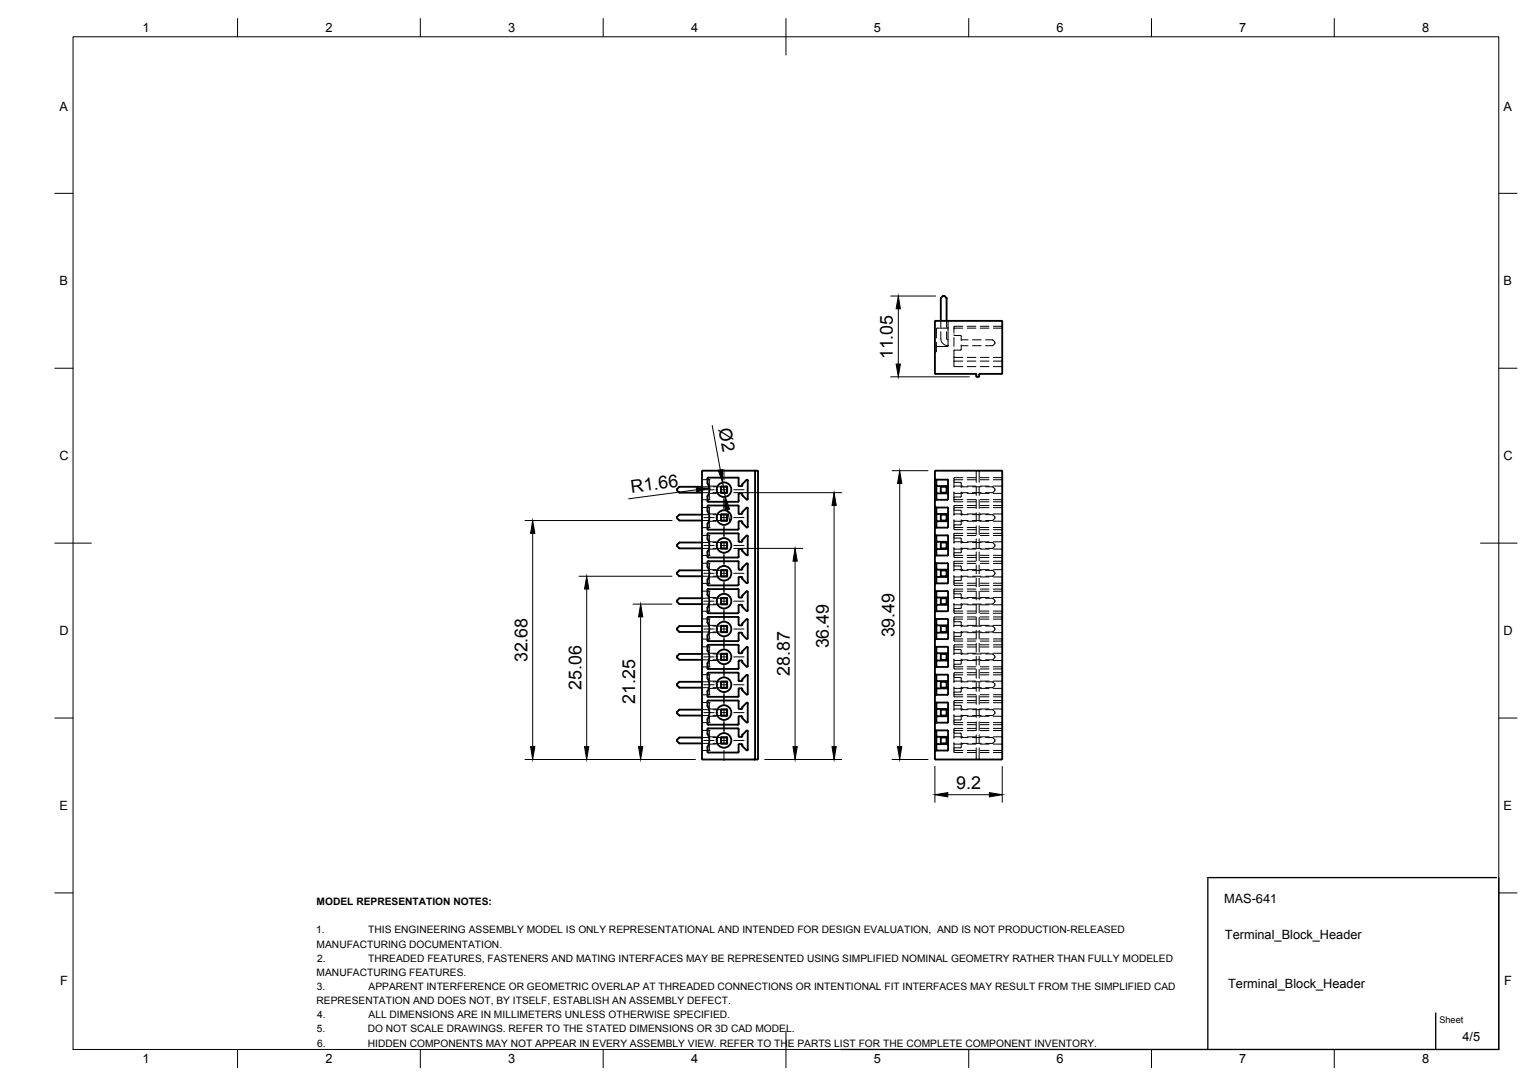
ISO-10303-21;
HEADER;
FILE_DESCRIPTION((''),'2;1');
FILE_NAME('Terminal_Block_Header.step','2026-10-09T09:55:32-07:00',(''),(''),'','','');
FILE_SCHEMA (('AUTOMOTIVE_DESIGN { 1 0 10303 214 3 1 1 }'));
ENDSEC;
DATA;
#10=MECHANICAL_DESIGN_GEOMETRIC_PRESENTATION_REPRESENTATION('',(#80780,#80781,#80782,#80783,#80784,#80785,#80786,#80787,#80788,#80789,#80790,#80791,#80792,#80793,#80794,#80795,#80796,#80797,#80798,#80799,#80800,#80801,#80802,#80803,#80804,#80805,#80806,#80807,#80808,#80809,#80810,#80811,#80812,#80813,#80814,#80815,#80816,#80817,#80818,#80819,#80820,#80821,#80822,#80823,#80824,#80825,#80826,#80827,#80828,#80829,#80830,#80831,#80832,#80833,#80834,#80835,#80836,#80837,#80838,#80839,#80840,#80841,#80842,#80843,#80844,#80845,#80846,#80847,#80848,#80849,#80850,#80851,#80852,#80853,#80854,#80855,#80856,#80857,#80858,#80859,#80860,#80861,#80862,#80863,#80864,#80865,#80866,#80867,#80868,#80869,#80870,#80871,#80872,#80873,#80874,#80875,#80876,#80877,#80878,#80879,#80880,#80881,#80882,#80883,#80884,#80885,#80886,#80887,#80888,#80889,#80890,#80891,#80892,#80893,#80894,#80895,#80896,#80897,#80898,#80899,#80900,#80901,#80902,#80903,#80904,#80905,#80906,#80907,#80908,#80909,#80910,#80911,#80912,#80913,#80914,#80915,#80916,#80917,#80918,#80919,#80920,#80921,#80922,#80923,#80924,#80925,#80926,#80927,#80928,#80929,#80930,#80931,#80932,#80933,#80934,#80935,#80936,#80937,#80938,#80939,#80940,#80941,#80942,#80943,#80944,#80945,#80946,#80947,#80948,#80949,#80950,#80951,#80952,#80953,#80954,#80955,#80956,#80957,#80958,#80959,#80960,#80961,#80962,#80963,#80964,#80965,#80966,#80967,#80968,#80969,#80970,#80971,#80972,#80973,#80974,#80975,#80976,#80977,#80978,#80979,#80980,#80981,#80982,#80983,#80984,#80985,#80986,#80987,#80988,#80989,#80990,#80991,#80992,#80993,#80994,#80995,#80996,#80997,#80998,#80999,#81000,#81001,#81002,#81003,#81004,#81005,#81006,#81007,#81008,#81009,#81010,#81011,#81012,#81013,#81014,#81015,#81016,#81017,#81018,#81019,#81020,#81021,#81022,#81023,#81024,#81025,#81026,#81027,#81028,#81029,#81030,#81031,#81032,#81033,#81034,#81035,#81036,#81037,#81038,#81039,#81040,#81041,#81042,#81043,#81044,#81045,#81046,#81047,#81048,#81049,#81050,#81051,#81052,#81053,#81054,#81055,#81056,#81057,#81058,#81059,#81060,#81061,#81062,#81063,#81064,#81065,#81066,#81067,#81068,#81069,#81070,#81071,#81072,#81073,#81074,#81075,#81076,#81077,#81078,#81079,#81080,#81081,#81082,#81083,#81084,#81085,#81086,#81087,#81088,#81089,#81090,#81091,#81092,#81093,#81094,#81095,#81096,#81097,#81098,#81099,#81100,#81101,#81102,#81103,#81104,#81105,#81106,#81107,#81108,#81109,#81110,#81111,#81112,#81113,#81114,#81115,#81116,#81117,#81118,#81119,#81120,#81121,#81122,#81123,#81124,#81125,#81126,#81127,#81128,#81129,#81130,#81131,#81132,#81133,#81134,#81135,#81136,#81137,#81138,#81139,#81140,#81141,#81142,#81143,#81144,#81145,#81146,#81147,#81148,#81149,#81150,#81151,#81152,#81153,#81154,#81155,#81156,#81157,#81158,#81159,#81160,#81161,#81162,#81163,#81164,#81165,#81166,#81167,#81168,#81169,#81170,#81171,#81172,#81173,#81174,#81175,#81176,#81177,#81178,#81179,#81180,#81181,#81182,#81183,#81184,#81185,#81186,#81187,#81188,#81189,#81190,#81191,#81192,#81193,#81194,#81195,#81196,#81197,#81198,#81199,#81200,#81201,#81202,#81203,#81204,#81205,#81206,#81207,#81208,#81209,#81210,#81211,#81212,#81213,#81214,#81215,#81216,#81217,#81218,#81219,#81220,#81221,#81222,#81223,#81224,#81225,#81226,#81227,#81228,#81229,#81230,#81231,#81232,#81233,#81234,#81235,#81236,#81237,#81238,#81239,#81240,#81241,#81242,#81243,#81244,#81245,#81246,#81247,#81248,#81249,#81250,#81251,#81252,#81253,#81254,#81255,#81256,#81257,#81258,#81259,#81260,#81261,#81262,#81263,#81264,#81265,#81266,#81267,#81268,#81269,#81270,#81271,#81272,#81273,#81274,#81275,#81276,#81277,#81278,#81279,#81280,#81281,#81282,#81283,#81284,#81285,#81286,#81287,#81288,#81289,#81290,#81291,#81292,#81293,#81294,#81295,#81296,#81297,#81298,#81299,#81300,#81301,#81302,#81303,#81304,#81305,#81306,#81307,#81308,#81309,#81310,#81311,#81312,#81313,#81314,#81315,#81316,#81317,#81318,#81319,#81320,#81321,#81322,#81323,#81324,#81325,#81326,#81327,#81328,#81329,#81330,#81331,#81332,#81333,#81334,#81335,#81336,#81337,#81338,#81339,#81340,#81341,#81342,#81343,#81344,#81345,#81346,#81347,#81348,#81349,#81350,#81351,#81352,#81353,#81354,#81355,#81356,#81357,#81358,#81359,#81360,#81361,#81362,#81363,#81364,#81365,#81366,#81367,#81368,#81369,#81370,#81371,#81372,#81373,#81374,#81375,#81376,#81377,#81378,#81379,#81380,#81381,#81382,#81383,#81384,#81385,#81386,#81387,#81388,#81389,#81390,#81391,#81392,#81393,#81394,#81395,#81396,#81397,#81398,#81399,#81400,#81401,#81402,#81403,#81404,#81405,#81406,#81407,#81408,#81409,#81410,#81411,#81412,#81413,#81414,#81415,#81416,#81417,#81418,#81419,#81420,#81421,#81422,#81423,#81424,#81425,#81426,#81427,#81428,#81429,#81430,#81431,#81432,#81433,#81434,#81435,#81436,#81437,#81438,#81439,#81440,#81441,#81442,#81443,#81444,#81445,#81446,#81447,#81448,#81449,#81450,#81451,#81452,#81453,#81454,#81455,#81456,#81457,#81458,#81459,#81460,#81461,#81462,#81463,#81464,#81465,#81466,#81467,#81468,#81469,#81470,#81471,#81472,#81473,#81474,#81475,#81476,#81477,#81478,#81479,#81480,#81481,#81482,#81483,#81484,#81485,#81486,#81487,#81488,#81489,#81490,#81491,#81492,#81493,#81494,#81495,#81496,#81497,#81498,#81499,#81500,#81501,#81502,#81503,#81504,#81505,#81506,#81507,#81508,#81509,#81510,#81511,#81512,#81513,#81514,#81515,#81516,#81517,#81518,#81519,#81520,#81521,#81522,#81523,#81524,#81525,#81526,#81527,#81528,#81529,#81530,#81531,#81532,#81533,#81534,#81535,#81536,#81537,#81538,#81539,#81540,#81541,#81542,#81543,#81544,#81545,#81546,#81547,#81548,#81549,#81550,#81551,#81552,#81553,#81554,#81555,#81556,#81557,#81558,#81559,#81560,#81561,#81562,#81563,#81564,#81565,#81566,#81567,#81568,#81569,#81570,#81571,#81572,#81573,#81574,#81575,#81576,#81577,#81578,#81579,#81580,#81581,#81582,#81583,#81584,#81585,#81586,#81587,#81588,#81589,#81590,#81591,#81592,#81593,#81594,#81595,#81596,#81597,#81598,#81599,#81600,#81601,#81602,#81603,#81604,#81605,#81606,#81607,#81608,#81609,#81610,#81611,#81612,#81613,#81614,#81615,#81616,#81617,#81618,#81619,#81620,#81621,#81622,#81623,#81624,#81625,#81626,#81627,#81628,#81629,#81630,#81631,#81632,#81633,#81634,#81635,#81636,#81637,#81638,#81639,#81640,#81641,#81642,#81643,#81644,#81645,#81646,#81647,#81648,#81649,#81650,#81651,#81652,#81653,#81654,#81655,#81656,#81657,#81658,#81659,#81660,#81661,#81662,#81663,#81664,#81665,#81666,#81667,#81668,#81669,#81670,#81671,#81672,#81673,#81674,#81675,#81676,#81677,#81678,#81679,#81680,#81681,#81682,#81683,#81684,#81685,#81686,#81687,#81688,#81689,#81690,#81691,#81692,#81693,#81694,#81695,#81696,#81697,#81698,#81699,#81700,#81701,#81702,#81703,#81704,#81705,#81706,#81707,#81708,#81709,#81710,#81711,#81712,#81713,#81714,#81715,#81716,#81717,#81718,#81719,#81720,#81721,#81722,#81723,#81724,#81725,#81726,#81727,#81728,#81729,#81730,#81731,#81732,#81733,#81734,#81735,#81736,#81737,#81738,#81739,#81740,#81741,#81742,#81743,#81744,#81745,#81746,#81747,#81748,#81749,#81750,#81751,#81752,#81753,#81754,#81755,#81756,#81757,#81758,#81759,#81760,#81761,#81762,#81763,#81764,#81765,#81766,#81767,#81768,#81769,#81770,#81771,#81772,#81773,#81774,#81775,#81776,#81777,#81778,#81779,#81780,#81781,#81782,#81783,#81784,#81785,#81786,#81787,#81788,#81789,#81790,#81791,#81792,#81793,#81794,#81795,#81796,#81797,#81798,#81799,#81800,#81801,#81802,#81803,#81804,#81805,#81806,#81807,#81808,#81809,#81810,#81811,#81812,#81813,#81814,#81815,#81816,#81817,#81818,#81819,#81820,#81821,#81822,#81823,#81824,#81825,#81826,#81827,#81828,#81829,#81830,#81831,#81832,#81833,#81834,#81835,#81836,#81837,#81838,#81839,#81840,#81841,#81842,#81843,#81844,#81845,#81846,#81847,#81848,#81849,#81850,#81851,#81852,#81853,#81854,#81855,#81856,#81857,#81858,#81859,#81860,#81861,#81862,#81863,#81864,#81865,#81866,#81867,#81868,#81869,#81870,#81871,#81872,#81873,#81874,#81875,#81876,#81877,#81878,#81879,#81880,#81881,#81882,#81883,#81884,#81885,#81886,#81887,#81888,#81889,#81890,#81891,#81892,#81893,#81894,#81895,#81896,#81897,#81898,#81899,#81900,#81901,#81902,#81903,#81904,#81905,#81906,#81907,#81908,#81909,#81910,#81911,#81912,#81913,#81914,#81915,#81916,#81917,#81918,#81919,#81920,#81921,#81922,#81923,#81924,#81925,#81926,#81927,#81928,#81929,#81930,#81931,#81932,#81933,#81934,#81935,#81936,#81937,#81938,#81939,#81940,#81941,#81942,#81943,#81944,#81945,#81946,#81947,#81948,#81949,#81950,#81951,#81952,#81953,#81954,#81955,#81956,#81957,#81958,#81959,#81960,#81961,#81962,#81963,#81964,#81965,#81966,#81967,#81968,#81969,#81970,#81971,#81972,#81973,#81974,#81975,#81976,#81977,#81978,#81979,#81980,#81981,#81982,#81983,#81984,#81985,#81986,#81987,#81988,#81989,#81990,#81991,#81992,#81993,#81994,#81995,#81996,#81997,#81998,#81999,#82000,#82001,#82002,#82003,#82004,#82005,#82006,#82007,#82008,#82009,#82010,#82011,#82012,#82013,#82014,#82015,#82016,#82017,#82018,#82019,#82020,#82021,#82022,#82023,#82024,#82025,#82026,#82027,#82028,#82029,#82030,#82031,#82032,#82033,#82034,#82035,#82036,#82037,#82038,#82039,#82040,#82041,#82042,#82043,#82044,#82045,#82046,#82047,#82048,#82049,#82050,#82051,#82052,#82053,#82054,#82055,#82056,#82057,#82058,#82059,#82060,#82061,#82062,#82063,#82064,#82065,#82066,#82067,#82068,#82069,#82070,#82071,#82072,#82073,#82074,#82075,#82076,#82077,#82078,#82079,#82080,#82081,#82082,#82083,#82084,#82085,#82086,#82087,#82088,#82089,#82090,#82091,#82092,#82093,#82094,#82095,#82096,#82097,#82098,#82099,#82100,#82101,#82102,#82103,#82104,#82105,#82106,#82107,#82108,#82109,#82110,#82111,#82112,#82113,#82114,#82115,#82116,#82117,#82118,#82119,#82120,#82121,#82122,#82123,#82124,#82125,#82126,#82127,#82128,#82129,#82130,#82131,#82132,#82133,#82134,#82135,#82136,#82137,#82138,#82139,#82140,#82141,#82142,#82143,#82144,#82145,#82146,#82147,#82148,#82149,#82150,#82151,#82152,#82153,#82154,#82155,#82156,#82157,#82158,#82159,#82160,#82161,#82162,#82163,#82164,#82165,#82166,#82167,#82168,#82169,#82170,#82171,#82172,#82173,#82174,#82175,#82176,#82177,#82178,#82179,#82180,#82181,#82182,#82183,#82184,#82185,#82186,#82187,#82188,#82189,#82190,#82191,#82192,#82193,#82194,#82195,#82196,#82197,#82198,#82199,#82200,#82201,#82202,#82203,#82204,#82205,#82206,#82207,#82208,#82209,#82210,#82211,#82212,#82213,#82214,#82215,#82216,#82217,#82218,#82219,#82220,#82221,#82222,#82223,#82224,#82225,#82226,#82227,#82228,#82229,#82230,#82231,#82232,#82233,#82234,#82235,#82236,#82237,#82238,#82239,#82240,#82241,#82242,#82243,#82244,#82245,#82246,#82247,#82248,#82249,#82250,#82251,#82252,#82253,#82254,#82255,#82256,#82257,#82258,#82259,#82260,#82261,#82262,#82263,#82264,#82265,#82266,#82267,#82268,#82269,#82270,#82271,#82272,#82273,#82274,#82275,#82276,#82277,#82278,#82279,#82280,#82281,#82282,#82283,#82284,#82285,#82286,#82287,#82288,#82289,#82290,#82291,#82292,#82293,#82294,#82295,#82296,#82297,#82298,#82299,#82300,#82301,#82302,#82303,#82304,#82305,#82306,#82307,#82308,#82309,#82310,#82311,#82312,#82313,#82314,#82315,#82316,#82317,#82318,#82319,#82320,#82321,#82322,#82323,#82324,#82325,#82326,#82327,#82328,#82329,#82330,#82331,#82332,#82333,#82334,#82335,#82336,#82337,#82338,#82339,#82340,#82341,#82342,#82343,#82344,#82345,#82346,#82347,#82348,#82349,#82350,#82351,#82352,#82353,#82354,#82355,#82356,#82357,#82358,#82359,#82360,#82361,#82362,#82363,#82364,#82365,#82366,#82367,#82368,#82369,#82370,#82371,#82372,#82373,#82374,#82375,#82376,#82377,#82378,#82379,#82380,#82381,#82382,#82383,#82384,#82385,#82386,#82387,#82388,#82389,#82390,#82391,#82392,#82393,#82394,#82395,#82396,#82397,#82398,#82399,#82400,#82401,#82402,#82403,#82404,#82405,#82406,#82407,#82408,#82409,#82410,#82411,#82412,#82413,#82414,#82415,#82416,#82417,#82418,#82419,#82420,#82421,#82422,#82423,#82424,#82425,#82426,#82427,#82428,#82429,#82430,#82431,#82432,#82433,#82434,#82435,#82436,#82437,#82438,#82439,#82440,#82441,#82442,#82443,#82444,#82445,#82446,#82447,#82448,#82449,#82450,#82451,#82452,#82453,#82454,#82455,#82456,#82457,#82458,#82459,#82460,#82461,#82462,#82463,#82464,#82465,#82466,#82467,#82468,#82469,#82470,#82471,#82472,#82473,#82474,#82475,#82476,#82477,#82478,#82479,#82480,#82481,#82482,#82483,#82484,#82485,#82486,#82487,#82488,#82489,#82490,#82491,#82492,#82493,#82494,#82495,#82496,#82497,#82498,#82499,#82500,#82501,#82502,#82503,#82504,#82505,#82506,#82507,#82508,#82509,#82510,#82511,#82512,#82513,#82514,#82515,#82516,#82517,#82518,#82519,#82520,#82521,#82522,#82523,#82524,#82525,#82526,#82527,#82528,#82529,#82530,#82531,#82532,#82533,#82534,#82535,#82536,#82537,#82538,#82539,#82540,#82541,#82542,#82543,#82544,#82545,#82546,#82547,#82548,#82549,#82550,#82551,#82552,#82553,#82554,#82555,#82556,#82557,#82558,#82559,#82560,#82561,#82562,#82563,#82564,#82565,#82566,#82567,#82568,#82569,#82570,#82571,#82572,#82573,#82574,#82575,#82576,#82577,#82578,#82579,#82580,#82581,#82582,#82583,#82584,#82585,#82586,#82587,#82588,#82589,#82590,#82591,#82592,#82593,#82594,#82595,#82596,#82597,#82598,#82599,#82600,#82601,#82602,#82603,#82604,#82605,#82606,#82607,#82608,#82609,#82610,#82611,#82612,#82613,#82614,#82615,#82616,#82617,#82618,#82619,#82620,#82621,#82622,#82623,#82624,#82625,#82626,#82627,#82628,#82629,#82630,#82631,#82632,#82633,#82634,#82635,#82636,#82637,#82638,#82639,#82640,#82641,#82642,#82643,#82644,#82645,#82646,#82647,#82648,#82649,#82650,#82651,#82652,#82653,#82654,#82655,#82656,#82657,#82658,#82659,#82660,#82661,#82662,#82663,#82664,#82665,#82666,#82667,#82668,#82669,#82670,#82671,#82672,#82673,#82674,#82675,#82676,#82677,#82678,#82679,#82680,#82681,#82682,#82683,#82684,#82685,#82686,#82687,#82688,#82689,#82690,#82691,#82692,#82693,#82694,#82695,#82696,#82697,#82698,#82699,#82700,#82701,#82702,#82703,#82704,#82705,#82706,#82707,#82708,#82709,#82710,#82711,#82712,#82713,#82714,#82715,#82716,#82717,#82718,#82719,#82720,#82721,#82722,#82723,#82724,#82725,#82726,#82727,#82728,#82729,#82730,#82731,#82732,#82733,#82734,#82735,#82736,#82737,#82738,#82739,#82740,#82741,#82742,#82743,#82744,#82745,#82746,#82747,#82748,#82749,#82750,#82751,#82752,#82753,#82754,#82755,#82756,#82757,#82758,#82759,#82760,#82761,#82762,#82763,#82764,#82765,#82766,#82767,#82768,#82769,#82770,#82771,#82772,#82773,#82774,#82775,#82776,#82777,#82778,#82779,#82780,#82781,#82782,#82783,#82784,#82785,#82786,#82787,#82788,#82789,#82790,#82791,#82792,#82793,#82794,#82795,#82796,#82797,#82798,#82799,#82800,#82801,#82802,#82803,#82804,#82805,#82806,#82807,#82808,#82809,#82810,#82811,#82812,#82813,#82814,#82815,#82816,#82817,#82818,#82819,#82820,#82821,#82822,#82823,#82824,#82825,#82826,#82827,#82828,#82829,#82830,#82831,#82832,#82833,#82834,#82835,#82836,#82837,#82838,#82839,#82840,#82841,#82842,#82843,#82844,#82845,#82846,#82847,#82848,#82849,#82850,#82851,#82852,#82853,#82854,#82855,#82856,#82857,#82858,#82859,#82860,#82861,#82862,#82863,#82864,#82865,#82866,#82867,#82868,#82869,#82870,#82871,#82872,#82873,#82874,#82875,#82876,#82877,#82878,#82879,#82880,#82881,#82882,#82883,#82884,#82885,#82886,#82887,#82888,#82889,#82890,#82891,#82892,#82893,#82894,#82895,#82896,#82897,#82898,#82899,#82900,#82901,#82902,#82903,#82904,#82905,#82906,#82907,#82908,#82909,#82910,#82911,#82912,#82913,#82914,#82915,#82916,#82917,#82918,#82919,#82920,#82921,#82922,#82923,#82924,#82925,#82926,#82927,#82928,#82929,#82930,#82931,#82932,#82933,#82934,#82935,#82936,#82937,#82938,#82939,#82940,#82941,#82942,#82943,#82944,#82945,#82946,#82947,#82948,#82949,#82950,#82951,#82952,#82953,#82954,#82955,#82956,#82957,#82958,#82959,#82960,#82961,#82962,#82963,#82964,#82965,#82966,#82967,#82968,#82969,#82970,#82971,#82972,#82973,#82974,#82975,#82976,#82977,#82978,#82979,#82980,#82981,#82982,#82983,#82984,#82985,#82986,#82987,#82988,#82989,#82990,#82991,#82992,#82993,#82994,#82995,#82996,#82997,#82998,#82999,#83000,#83001,#83002,#83003,#83004,#83005,#83006,#83007,#83008,#83009,#83010),#170127);
#24=SHAPE_REPRESENTATION_RELATIONSHIP('SRR','None',#170145,#27) ;
#27=ADVANCED_BREP_SHAPE_REPRESENTATION('',(#32),#170125) ;
#32=MANIFOLD_SOLID_BREP('Body1',#91086) ;
#357=ELLIPSE('',#93363,0.141421356226833,0.0999999999854714) ;
#358=ELLIPSE('',#93380,0.141421356205715,0.0999999999561054) ;
#359=ELLIPSE('',#93397,0.141421356206211,0.0999999999568741) ;
#360=ELLIPSE('',#93414,0.14142135619891,0.0999999999469108) ;
#361=ELLIPSE('',#93431,0.14142135620716,0.0999999999583245) ;
#362=ELLIPSE('',#93448,0.141421356264666,0.100000000037862) ;
#363=ELLIPSE('',#93465,0.141421356235352,0.0999999999972513) ;
#364=ELLIPSE('',#93482,0.141421356240128,0.100000000003844) ;
#365=ELLIPSE('',#93544,0.141421356242718,0.100000000007393) ;
#366=ELLIPSE('',#93593,0.141421356244824,0.100000000010334) ;
#684=FACE_BOUND('',#24047,.T.) ;
#685=FACE_BOUND('',#24048,.T.) ;
#686=FACE_BOUND('',#24049,.T.) ;
#687=FACE_BOUND('',#24050,.T.) ;
#688=FACE_BOUND('',#24051,.T.) ;
#689=FACE_BOUND('',#24052,.T.) ;
#690=FACE_BOUND('',#24053,.T.) ;
#691=FACE_BOUND('',#24054,.T.) ;
#692=FACE_BOUND('',#24055,.T.) ;
#693=FACE_BOUND('',#24056,.T.) ;
#694=FACE_BOUND('',#24093,.T.) ;
#695=FACE_BOUND('',#24095,.T.) ;
#696=FACE_BOUND('',#24382,.T.) ;
#697=FACE_BOUND('',#24411,.T.) ;
#698=FACE_BOUND('',#24440,.T.) ;
#699=FACE_BOUND('',#24469,.T.) ;
#700=FACE_BOUND('',#24498,.T.) ;
#701=FACE_BOUND('',#24527,.T.) ;
#702=FACE_BOUND('',#24556,.T.) ;
#703=FACE_BOUND('',#24585,.T.) ;
#704=FACE_BOUND('',#24614,.T.) ;
#705=FACE_BOUND('',#24616,.T.) ;
#706=FACE_BOUND('',#24618,.T.) ;
#707=FACE_BOUND('',#24620,.T.) ;
#708=FACE_BOUND('',#24622,.T.) ;
#709=FACE_BOUND('',#24624,.T.) ;
#710=FACE_BOUND('',#24626,.T.) ;
#711=FACE_BOUND('',#24628,.T.) ;
#712=FACE_BOUND('',#24630,.T.) ;
#713=FACE_BOUND('',#24632,.T.) ;
#1083=PLANE('',#93599) ;
#1084=PLANE('',#93604) ;
#1085=PLANE('',#93609) ;
#1086=PLANE('',#93614) ;
#1087=PLANE('',#93619) ;
#1088=PLANE('',#93624) ;
#1089=PLANE('',#93629) ;
#1090=PLANE('',#93634) ;
#1091=PLANE('',#93639) ;
#1092=PLANE('',#93644) ;
#1093=PLANE('',#93646) ;
#1094=PLANE('',#93648) ;
#1095=PLANE('',#93650) ;
#1096=PLANE('',#93652) ;
#1097=PLANE('',#93654) ;
#1098=PLANE('',#93656) ;
#1099=PLANE('',#93658) ;
#1100=PLANE('',#93660) ;
#1101=PLANE('',#93662) ;
#1102=PLANE('',#93664) ;
#1103=PLANE('',#93666) ;
#1104=PLANE('',#93668) ;
#1105=PLANE('',#93670) ;
#1106=PLANE('',#93672) ;
#1107=PLANE('',#93674) ;
#1108=PLANE('',#93676) ;
#1109=PLANE('',#93678) ;
#1110=PLANE('',#93707) ;
#1111=PLANE('',#93712) ;
#1112=PLANE('',#93714) ;
#1113=PLANE('',#93722) ;
#1114=PLANE('',#93746) ;
#1115=PLANE('',#93770) ;
#1116=PLANE('',#93774) ;
#1117=PLANE('',#93778) ;
#1118=PLANE('',#93782) ;
#1119=PLANE('',#93786) ;
#1120=PLANE('',#93790) ;
#1121=PLANE('',#93891) ;
#1122=PLANE('',#93894) ;
#1123=PLANE('',#93897) ;
#1124=PLANE('',#93900) ;
#1125=PLANE('',#93901) ;
#1126=PLANE('',#93902) ;
#1127=PLANE('',#93903) ;
#1128=PLANE('',#93904) ;
#1129=PLANE('',#93908) ;
#1130=PLANE('',#93912) ;
#1131=PLANE('',#93916) ;
#1132=PLANE('',#93919) ;
#1133=PLANE('',#93920) ;
#1134=PLANE('',#93924) ;
#1135=PLANE('',#93928) ;
#1136=PLANE('',#93932) ;
#1137=PLANE('',#93936) ;
#1138=PLANE('',#93940) ;
#1139=PLANE('',#93950) ;
#1140=PLANE('',#93954) ;
#1141=PLANE('',#93958) ;
#1142=PLANE('',#93959) ;
#1143=PLANE('',#93965) ;
#1144=PLANE('',#94240) ;
#1145=PLANE('',#94241) ;
#1146=PLANE('',#94242) ;
#1147=PLANE('',#94243) ;
#1148=PLANE('',#94244) ;
#1149=PLANE('',#94245) ;
#1150=PLANE('',#94248) ;
#1151=PLANE('',#94257) ;
#1152=PLANE('',#94258) ;
#1153=PLANE('',#94259) ;
#1154=PLANE('',#94260) ;
#1155=PLANE('',#94261) ;
#1156=PLANE('',#94262) ;
#1157=PLANE('',#94263) ;
#1158=PLANE('',#94264) ;
#1159=PLANE('',#94265) ;
#1160=PLANE('',#94266) ;
#1161=PLANE('',#94267) ;
#1162=PLANE('',#94380) ;
#1163=PLANE('',#94383) ;
#1164=PLANE('',#94386) ;
#1165=PLANE('',#94389) ;
#1166=PLANE('',#94392) ;
#1167=PLANE('',#94395) ;
#1168=PLANE('',#94398) ;
#1169=PLANE('',#94401) ;
#1170=PLANE('',#94404) ;
#1171=PLANE('',#94407) ;
#1172=PLANE('',#94408) ;
#1173=PLANE('',#94409) ;
#1174=PLANE('',#94410) ;
#1175=PLANE('',#94411) ;
#1176=PLANE('',#94412) ;
#1177=PLANE('',#94413) ;
#1178=PLANE('',#94414) ;
#1179=PLANE('',#94415) ;
#1180=PLANE('',#94416) ;
#1181=PLANE('',#94417) ;
#1182=PLANE('',#94418) ;
#1183=PLANE('',#94419) ;
#1184=PLANE('',#94420) ;
#1185=PLANE('',#94421) ;
#1186=PLANE('',#94422) ;
#1187=PLANE('',#94423) ;
#1188=PLANE('',#94424) ;
#1189=PLANE('',#94425) ;
#1190=PLANE('',#94426) ;
#1191=PLANE('',#94427) ;
#1192=PLANE('',#94428) ;
#1193=PLANE('',#94429) ;
#1194=PLANE('',#94430) ;
#1195=PLANE('',#94431) ;
#1196=PLANE('',#94432) ;
#1197=PLANE('',#94433) ;
#1198=PLANE('',#94434) ;
#1199=PLANE('',#94435) ;
#1200=PLANE('',#94436) ;
#1201=PLANE('',#94437) ;
#1202=PLANE('',#94438) ;
#1203=PLANE('',#94439) ;
#1204=PLANE('',#94440) ;
#1205=PLANE('',#94441) ;
#1206=PLANE('',#94442) ;
#1207=PLANE('',#94443) ;
#1208=PLANE('',#94444) ;
#1209=PLANE('',#94445) ;
#1210=PLANE('',#94446) ;
#1211=PLANE('',#94447) ;
#1212=PLANE('',#94448) ;
#1213=PLANE('',#94449) ;
#1214=PLANE('',#94450) ;
#1215=PLANE('',#94451) ;
#1216=PLANE('',#94455) ;
#1217=PLANE('',#94459) ;
#1218=PLANE('',#94463) ;
#1219=PLANE('',#94466) ;
#1220=PLANE('',#94467) ;
#1221=PLANE('',#94471) ;
#1222=PLANE('',#94475) ;
#1223=PLANE('',#94479) ;
#1224=PLANE('',#94483) ;
#1225=PLANE('',#94487) ;
#1226=PLANE('',#94497) ;
#1227=PLANE('',#94501) ;
#1228=PLANE('',#94505) ;
#1229=PLANE('',#94506) ;
#1230=PLANE('',#94515) ;
#1231=PLANE('',#94519) ;
#1232=PLANE('',#94523) ;
#1233=PLANE('',#94526) ;
#1234=PLANE('',#94527) ;
#1235=PLANE('',#94531) ;
#1236=PLANE('',#94535) ;
#1237=PLANE('',#94539) ;
#1238=PLANE('',#94543) ;
#1239=PLANE('',#94547) ;
#1240=PLANE('',#94557) ;
#1241=PLANE('',#94561) ;
#1242=PLANE('',#94565) ;
#1243=PLANE('',#94566) ;
#1244=PLANE('',#94575) ;
#1245=PLANE('',#94579) ;
#1246=PLANE('',#94583) ;
#1247=PLANE('',#94586) ;
#1248=PLANE('',#94587) ;
#1249=PLANE('',#94591) ;
#1250=PLANE('',#94595) ;
#1251=PLANE('',#94599) ;
#1252=PLANE('',#94603) ;
#1253=PLANE('',#94607) ;
#1254=PLANE('',#94617) ;
#1255=PLANE('',#94621) ;
#1256=PLANE('',#94625) ;
#1257=PLANE('',#94626) ;
#1258=PLANE('',#94635) ;
#1259=PLANE('',#94639) ;
#1260=PLANE('',#94643) ;
#1261=PLANE('',#94646) ;
#1262=PLANE('',#94647) ;
#1263=PLANE('',#94651) ;
#1264=PLANE('',#94655) ;
#1265=PLANE('',#94659) ;
#1266=PLANE('',#94663) ;
#1267=PLANE('',#94667) ;
#1268=PLANE('',#94677) ;
#1269=PLANE('',#94681) ;
#1270=PLANE('',#94685) ;
#1271=PLANE('',#94686) ;
#1272=PLANE('',#94695) ;
#1273=PLANE('',#94699) ;
#1274=PLANE('',#94703) ;
#1275=PLANE('',#94706) ;
#1276=PLANE('',#94707) ;
#1277=PLANE('',#94711) ;
#1278=PLANE('',#94715) ;
#1279=PLANE('',#94719) ;
#1280=PLANE('',#94723) ;
#1281=PLANE('',#94727) ;
#1282=PLANE('',#94737) ;
#1283=PLANE('',#94741) ;
#1284=PLANE('',#94745) ;
#1285=PLANE('',#94746) ;
#1286=PLANE('',#94755) ;
#1287=PLANE('',#94759) ;
#1288=PLANE('',#94763) ;
#1289=PLANE('',#94766) ;
#1290=PLANE('',#94767) ;
#1291=PLANE('',#94771) ;
#1292=PLANE('',#94775) ;
#1293=PLANE('',#94779) ;
#1294=PLANE('',#94783) ;
#1295=PLANE('',#94787) ;
#1296=PLANE('',#94797) ;
#1297=PLANE('',#94801) ;
#1298=PLANE('',#94805) ;
#1299=PLANE('',#94806) ;
#1300=PLANE('',#94815) ;
#1301=PLANE('',#94819) ;
#1302=PLANE('',#94823) ;
#1303=PLANE('',#94826) ;
#1304=PLANE('',#94827) ;
#1305=PLANE('',#94831) ;
#1306=PLANE('',#94835) ;
#1307=PLANE('',#94839) ;
#1308=PLANE('',#94843) ;
#1309=PLANE('',#94847) ;
#1310=PLANE('',#94857) ;
#1311=PLANE('',#94861) ;
#1312=PLANE('',#94865) ;
#1313=PLANE('',#94866) ;
#1314=PLANE('',#94875) ;
#1315=PLANE('',#94879) ;
#1316=PLANE('',#94883) ;
#1317=PLANE('',#94886) ;
#1318=PLANE('',#94887) ;
#1319=PLANE('',#94891) ;
#1320=PLANE('',#94895) ;
#1321=PLANE('',#94899) ;
#1322=PLANE('',#94903) ;
#1323=PLANE('',#94907) ;
#1324=PLANE('',#94917) ;
#1325=PLANE('',#94921) ;
#1326=PLANE('',#94925) ;
#1327=PLANE('',#94926) ;
#1328=PLANE('',#94935) ;
#1329=PLANE('',#94939) ;
#1330=PLANE('',#94943) ;
#1331=PLANE('',#94946) ;
#1332=PLANE('',#94947) ;
#1333=PLANE('',#94951) ;
#1334=PLANE('',#94955) ;
#1335=PLANE('',#94959) ;
#1336=PLANE('',#94963) ;
#1337=PLANE('',#94967) ;
#1338=PLANE('',#94977) ;
#1339=PLANE('',#94981) ;
#1340=PLANE('',#94985) ;
#1341=PLANE('',#94986) ;
#1342=PLANE('',#94992) ;
#1343=PLANE('',#94997) ;
#1344=PLANE('',#95002) ;
#1345=PLANE('',#95007) ;
#1346=PLANE('',#95012) ;
#1347=PLANE('',#95017) ;
#1348=PLANE('',#95022) ;
#1349=PLANE('',#95027) ;
#1350=PLANE('',#95032) ;
#1351=PLANE('',#96891) ;
#1352=PLANE('',#96892) ;
#1353=PLANE('',#96893) ;
#1354=PLANE('',#96894) ;
#1355=PLANE('',#96895) ;
#1356=PLANE('',#96896) ;
#1357=PLANE('',#96899) ;
#1358=PLANE('',#96908) ;
#1359=PLANE('',#96909) ;
#1360=PLANE('',#96910) ;
#1361=PLANE('',#96911) ;
#1362=PLANE('',#96912) ;
#1363=PLANE('',#96913) ;
#1364=PLANE('',#96914) ;
#1365=PLANE('',#96915) ;
#1366=PLANE('',#96916) ;
#1367=PLANE('',#96917) ;
#1368=PLANE('',#96918) ;
#1369=PLANE('',#96919) ;
#1370=PLANE('',#96920) ;
#1371=PLANE('',#96923) ;
#1372=PLANE('',#96932) ;
#1373=PLANE('',#96933) ;
#1374=PLANE('',#96934) ;
#1375=PLANE('',#96935) ;
#1376=PLANE('',#96936) ;
#1377=PLANE('',#96937) ;
#1378=PLANE('',#96938) ;
#1379=PLANE('',#96939) ;
#1380=PLANE('',#96940) ;
#1381=PLANE('',#96941) ;
#1382=PLANE('',#96942) ;
#1383=PLANE('',#96943) ;
#1384=PLANE('',#96944) ;
#1385=PLANE('',#96947) ;
#1386=PLANE('',#96956) ;
#1387=PLANE('',#96957) ;
#1388=PLANE('',#96958) ;
#1389=PLANE('',#96959) ;
#1390=PLANE('',#96960) ;
#1391=PLANE('',#96961) ;
#1392=PLANE('',#96962) ;
#1393=PLANE('',#96963) ;
#1394=PLANE('',#96964) ;
#1395=PLANE('',#96965) ;
#1396=PLANE('',#96966) ;
#1397=PLANE('',#96967) ;
#1398=PLANE('',#96968) ;
#1399=PLANE('',#96971) ;
#1400=PLANE('',#96980) ;
#1401=PLANE('',#96981) ;
#1402=PLANE('',#96982) ;
#1403=PLANE('',#96983) ;
#1404=PLANE('',#96984) ;
#1405=PLANE('',#96985) ;
#1406=PLANE('',#96986) ;
#1407=PLANE('',#96987) ;
#1408=PLANE('',#96988) ;
#1409=PLANE('',#96989) ;
#1410=PLANE('',#96990) ;
#1411=PLANE('',#96991) ;
#1412=PLANE('',#96992) ;
#1413=PLANE('',#96995) ;
#1414=PLANE('',#97004) ;
#1415=PLANE('',#97005) ;
#1416=PLANE('',#97006) ;
#1417=PLANE('',#97007) ;
#1418=PLANE('',#97008) ;
#1419=PLANE('',#97009) ;
#1420=PLANE('',#97010) ;
#1421=PLANE('',#97011) ;
#1422=PLANE('',#97012) ;
#1423=PLANE('',#97013) ;
#1424=PLANE('',#97014) ;
#1425=PLANE('',#97015) ;
#1426=PLANE('',#97016) ;
#1427=PLANE('',#97019) ;
#1428=PLANE('',#97028) ;
#1429=PLANE('',#97029) ;
#1430=PLANE('',#97030) ;
#1431=PLANE('',#97031) ;
#1432=PLANE('',#97032) ;
#1433=PLANE('',#97033) ;
#1434=PLANE('',#97034) ;
#1435=PLANE('',#97035) ;
#1436=PLANE('',#97036) ;
#1437=PLANE('',#97037) ;
#1438=PLANE('',#97038) ;
#1439=PLANE('',#97039) ;
#1440=PLANE('',#97040) ;
#1441=PLANE('',#97043) ;
#1442=PLANE('',#97052) ;
#1443=PLANE('',#97053) ;
#1444=PLANE('',#97054) ;
#1445=PLANE('',#97055) ;
#1446=PLANE('',#97056) ;
#1447=PLANE('',#97057) ;
#1448=PLANE('',#97058) ;
#1449=PLANE('',#97059) ;
#1450=PLANE('',#97060) ;
#1451=PLANE('',#97061) ;
#1452=PLANE('',#97062) ;
#1453=PLANE('',#97063) ;
#1454=PLANE('',#97064) ;
#1455=PLANE('',#97067) ;
#1456=PLANE('',#97076) ;
#1457=PLANE('',#97077) ;
#1458=PLANE('',#97078) ;
#1459=PLANE('',#97079) ;
#1460=PLANE('',#97080) ;
#1461=PLANE('',#97081) ;
#1462=PLANE('',#97082) ;
#1463=PLANE('',#97083) ;
#1464=PLANE('',#97084) ;
#1465=PLANE('',#97085) ;
#1466=PLANE('',#97086) ;
#1467=PLANE('',#97087) ;
#1468=PLANE('',#97088) ;
#1469=PLANE('',#97091) ;
#1470=PLANE('',#97100) ;
#1471=PLANE('',#97101) ;
#1472=PLANE('',#97102) ;
#1473=PLANE('',#97103) ;
#1474=PLANE('',#97104) ;
#1475=PLANE('',#97105) ;
#1476=PLANE('',#97106) ;
#1477=PLANE('',#97107) ;
#1478=PLANE('',#97108) ;
#1479=PLANE('',#97109) ;
#1480=PLANE('',#97110) ;
#1481=PLANE('',#97111) ;
#1482=PLANE('',#97112) ;
#1483=PLANE('',#97113) ;
#1484=PLANE('',#97114) ;
#1485=PLANE('',#97115) ;
#1486=PLANE('',#97116) ;
#1487=PLANE('',#97117) ;
#1488=PLANE('',#97118) ;
#1489=PLANE('',#97119) ;
#1490=PLANE('',#97120) ;
#1491=PLANE('',#97121) ;
#1492=PLANE('',#97122) ;
#1493=PLANE('',#97123) ;
#1494=PLANE('',#97124) ;
#1495=PLANE('',#97125) ;
#1496=PLANE('',#97126) ;
#1497=PLANE('',#97127) ;
#1498=PLANE('',#97128) ;
#1499=PLANE('',#97129) ;
#1500=PLANE('',#97130) ;
#1501=PLANE('',#97131) ;
#1502=PLANE('',#97132) ;
#1503=PLANE('',#97133) ;
#1504=PLANE('',#97134) ;
#1505=PLANE('',#97135) ;
#1506=PLANE('',#97136) ;
#1507=PLANE('',#97137) ;
#1508=PLANE('',#97138) ;
#1509=PLANE('',#97139) ;
#1510=PLANE('',#97140) ;
#1511=PLANE('',#97141) ;
#1512=PLANE('',#97142) ;
#2157=B_SPLINE_CURVE_WITH_KNOTS('',3,(#141862,#141863,#141864,#141865,#141866,
#141867,#141868,#141869),.UNSPECIFIED.,.F.,.F.,(4,2,2,4),(-0.0212593174733862,
-0.0176486602253693,-0.0143243289552082,-0.0134403252720105),
 .UNSPECIFIED.) ;
#2158=B_SPLINE_CURVE_WITH_KNOTS('',3,(#141905,#141906,#141907,#141908,#141909,
#141910,#141911,#141912),.UNSPECIFIED.,.F.,.F.,(4,2,2,4),(-0.021259317482921,
-0.0176486602328459,-0.0143243289609224,-0.0134403252772803),
 .UNSPECIFIED.) ;
#2159=B_SPLINE_CURVE_WITH_KNOTS('',3,(#141948,#141949,#141950,#141951,#141952,
#141953,#141954,#141955),.UNSPECIFIED.,.F.,.F.,(4,2,2,4),(-0.0212593174877944,
-0.0176486602368674,-0.0143243289641644,-0.0134403252803157),
 .UNSPECIFIED.) ;
#2160=B_SPLINE_CURVE_WITH_KNOTS('',3,(#141991,#141992,#141993,#141994,#141995,
#141996,#141997,#141998),.UNSPECIFIED.,.F.,.F.,(4,2,2,4),(-0.0212593174829433,
-0.0176486602328601,-0.014324328960934,-0.0134403252772914),
 .UNSPECIFIED.) ;
#2161=B_SPLINE_CURVE_WITH_KNOTS('',3,(#142034,#142035,#142036,#142037,#142038,
#142039,#142040,#142041),.UNSPECIFIED.,.F.,.F.,(4,2,2,4),(-0.0212593174732112,
-0.0176486602254681,-0.0143243289554829,-0.0134403252723181),
 .UNSPECIFIED.) ;
#2162=B_SPLINE_CURVE_WITH_KNOTS('',3,(#142077,#142078,#142079,#142080,#142081,
#142082,#142083,#142084),.UNSPECIFIED.,.F.,.F.,(4,2,2,4),(-0.0212593174781932,
-0.0176486602293651,-0.0143243289584549,-0.0134403252750573),
 .UNSPECIFIED.) ;
#2163=B_SPLINE_CURVE_WITH_KNOTS('',3,(#142120,#142121,#142122,#142123,#142124,
#142125,#142126,#142127),.UNSPECIFIED.,.F.,.F.,(4,2,2,4),(-0.0212593174830444,
-0.0176486602331658,-0.0143243289613579,-0.0134403252777338),
 .UNSPECIFIED.) ;
#2164=B_SPLINE_CURVE_WITH_KNOTS('',3,(#142163,#142164,#142165,#142166,#142167,
#142168,#142169,#142170),.UNSPECIFIED.,.F.,.F.,(4,2,2,4),(-0.021259317485983,
-0.017648660235379,-0.0143243289629727,-0.0134403252792024),
 .UNSPECIFIED.) ;
#2165=B_SPLINE_CURVE_WITH_KNOTS('',3,(#142287,#142288,#142289,#142290,#142291,
#142292,#142293,#142294),.UNSPECIFIED.,.F.,.F.,(4,2,2,4),(-0.0212593174838741,
-0.0176486602337396,-0.0143243289617316,-0.0134403252780616),
 .UNSPECIFIED.) ;
#2166=B_SPLINE_CURVE_WITH_KNOTS('',3,(#142411,#142412,#142413,#142414,#142415,
#142416,#142417,#142418),.UNSPECIFIED.,.F.,.F.,(4,2,2,4),(-0.021259317485706,
-0.0176486602351398,-0.0143243289627718,-0.013440325279013),
 .UNSPECIFIED.) ;
#2167=B_SPLINE_CURVE_WITH_KNOTS('',3,(#144015,#144016,#144017,#144018,#144019,
#144020,#144021,#144022),.UNSPECIFIED.,.F.,.F.,(4,2,2,4),(-0.052701717162025,
-0.0518504523811948,-0.0480303917439054,-0.04467544736819),
 .UNSPECIFIED.) ;
#2168=B_SPLINE_CURVE_WITH_KNOTS('',3,(#144026,#144027,#144028,#144029,#144030,
#144031,#144032,#144033,#144034,#144035,#144036,#144037,#144038,#144039,
#144040,#144041,#144042,#144043,#144044,#144045,#144046,#144047,#144048,
#144049,#144050,#144051,#144052,#144053,#144054,#144055,#144056),
 .UNSPECIFIED.,.F.,.F.,(4,3,3,3,3,3,3,3,3,3,4),(0.,1.7911486298437E-5,3.35636550441565E-5,
5.14128838689559E-5,6.71346369544057E-5,8.50076921954425E-5,0.000100614915215922,
0.000118595988596762,0.000134133865285036,0.000151845157316713,0.0001565184788544),
 .UNSPECIFIED.) ;
#2169=B_SPLINE_CURVE_WITH_KNOTS('',3,(#144058,#144059,#144060,#144061,#144062,
#144063,#144064,#144065,#144066,#144067,#144068,#144069,#144070,#144071,
#144072,#144073,#144074,#144075,#144076,#144077,#144078,#144079),
 .UNSPECIFIED.,.F.,.F.,(4,2,2,2,2,2,2,2,2,2,4),(-0.0842935807175857,-0.0841564124762399,
-0.0836958438579189,-0.0829341784875174,-0.0805923611130053,-0.0773601159115686,
-0.0742136752654363,-0.071123820447877,-0.0675672289498007,-0.0637829215046486,
-0.0629274139192696),.UNSPECIFIED.) ;
#2170=B_SPLINE_CURVE_WITH_KNOTS('',3,(#147077,#147078,#147079,#147080,#147081,
#147082,#147083,#147084),.UNSPECIFIED.,.F.,.F.,(4,2,2,4),(-0.0527017171620382,
-0.0518504523812081,-0.0480303917439178,-0.0446754473682008),
 .UNSPECIFIED.) ;
#2171=B_SPLINE_CURVE_WITH_KNOTS('',3,(#147088,#147089,#147090,#147091,#147092,
#147093,#147094,#147095,#147096,#147097,#147098,#147099,#147100,#147101,
#147102,#147103,#147104,#147105,#147106,#147107,#147108,#147109,#147110,
#147111,#147112,#147113,#147114,#147115,#147116,#147117,#147118),
 .UNSPECIFIED.,.F.,.F.,(4,3,3,3,3,3,3,3,3,3,4),(0.,1.79114862984415E-5,
3.35636550441565E-5,5.14128838689557E-5,6.7134636954406E-5,8.50076921954395E-5,
0.000100614915215921,0.000118595988596772,0.000134133865285036,0.000151845157316653,
0.0001565184788544),.UNSPECIFIED.) ;
#2172=B_SPLINE_CURVE_WITH_KNOTS('',3,(#147120,#147121,#147122,#147123,#147124,
#147125,#147126,#147127,#147128,#147129,#147130,#147131,#147132,#147133,
#147134,#147135,#147136,#147137,#147138,#147139,#147140,#147141),
 .UNSPECIFIED.,.F.,.F.,(4,2,2,2,2,2,2,2,2,2,4),(-0.0842935807153196,-0.0841564124739783,
-0.0836958438556783,-0.0829341784853091,-0.0805923611108952,-0.0773601159095917,
-0.0742136752635866,-0.0711238204461505,-0.0675672289482145,-0.0637829215032092,
-0.062927413917864),.UNSPECIFIED.) ;
#2173=B_SPLINE_CURVE_WITH_KNOTS('',3,(#147781,#147782,#147783,#147784,#147785,
#147786,#147787,#147788),.UNSPECIFIED.,.F.,.F.,(4,2,2,4),(-0.0527017171621304,
-0.0518504523813015,-0.0480303917440028,-0.0446754473682719),
 .UNSPECIFIED.) ;
#2174=B_SPLINE_CURVE_WITH_KNOTS('',3,(#147792,#147793,#147794,#147795,#147796,
#147797,#147798,#147799,#147800,#147801,#147802,#147803,#147804,#147805,
#147806,#147807,#147808,#147809,#147810,#147811,#147812,#147813,#147814,
#147815,#147816,#147817,#147818,#147819,#147820,#147821,#147822),
 .UNSPECIFIED.,.F.,.F.,(4,3,3,3,3,3,3,3,3,3,4),(0.,1.79114862984384E-5,
3.35636550441566E-5,5.14128838689606E-5,6.7134636954406E-5,8.50076921954722E-5,
0.000100614915215922,0.000118595988596755,0.000134133865285036,0.00015184515731678,
0.0001565184788544),.UNSPECIFIED.) ;
#2175=B_SPLINE_CURVE_WITH_KNOTS('',3,(#147824,#147825,#147826,#147827,#147828,
#147829,#147830,#147831,#147832,#147833,#147834,#147835,#147836,#147837,
#147838,#147839,#147840,#147841,#147842,#147843,#147844,#147845),
 .UNSPECIFIED.,.F.,.F.,(4,2,2,2,2,2,2,2,2,2,4),(-0.0842935807419127,-0.0841564125005222,
-0.0836958438819682,-0.082934178511186,-0.0805923611355419,-0.0773601159325885,
-0.0742136752850249,-0.0711238204661043,-0.0675672289665108,-0.0637829215197928,
-0.0629274139340661),.UNSPECIFIED.) ;
#2176=B_SPLINE_CURVE_WITH_KNOTS('',3,(#148008,#148009,#148010,#148011,#148012,
#148013,#148014,#148015),.UNSPECIFIED.,.F.,.F.,(4,2,2,4),(-0.0527017171621393,
-0.0518504523813096,-0.0480303917440155,-0.0446754473682944),
 .UNSPECIFIED.) ;
#2177=B_SPLINE_CURVE_WITH_KNOTS('',3,(#148019,#148020,#148021,#148022,#148023,
#148024,#148025,#148026,#148027,#148028,#148029,#148030,#148031,#148032,
#148033,#148034,#148035,#148036,#148037,#148038,#148039,#148040,#148041,
#148042,#148043,#148044,#148045,#148046,#148047,#148048,#148049),
 .UNSPECIFIED.,.F.,.F.,(4,3,3,3,3,3,3,3,3,3,4),(0.,1.7911486298444E-5,3.35636550441567E-5,
5.14128838689174E-5,6.71346369544062E-5,8.50076921954515E-5,0.000100614915215921,
0.000118595988596814,0.000134133865285036,0.000151845157316771,0.0001565184788544),
 .UNSPECIFIED.) ;
#2178=B_SPLINE_CURVE_WITH_KNOTS('',3,(#148051,#148052,#148053,#148054,#148055,
#148056,#148057,#148058,#148059,#148060,#148061,#148062,#148063,#148064,
#148065,#148066,#148067,#148068,#148069,#148070,#148071,#148072),
 .UNSPECIFIED.,.F.,.F.,(4,2,2,2,2,2,2,2,2,2,4),(-0.0842935808351552,-0.0841564125935704,
-0.0836958439740798,-0.0829341786018125,-0.0805923612217205,-0.077360116012801,
-0.0742136753596006,-0.0711238205353107,-0.0675672290297288,-0.0637829215768355,
-0.0629274139897445),.UNSPECIFIED.) ;
#2179=B_SPLINE_CURVE_WITH_KNOTS('',3,(#148235,#148236,#148237,#148238,#148239,
#148240,#148241,#148242),.UNSPECIFIED.,.F.,.F.,(4,2,2,4),(-0.0527017171620452,
-0.0518504523812172,-0.0480303917439374,-0.04467544736823),
 .UNSPECIFIED.) ;
#2180=B_SPLINE_CURVE_WITH_KNOTS('',3,(#148246,#148247,#148248,#148249,#148250,
#148251,#148252,#148253,#148254,#148255,#148256,#148257,#148258,#148259,
#148260,#148261,#148262,#148263,#148264,#148265,#148266,#148267,#148268,
#148269,#148270,#148271,#148272,#148273,#148274,#148275,#148276),
 .UNSPECIFIED.,.F.,.F.,(4,3,3,3,3,3,3,3,3,3,4),(0.,1.79114862984569E-5,
3.35636550441567E-5,5.14128838689565E-5,6.71346369544062E-5,8.50076921954284E-5,
0.000100614915215921,0.000118595988596684,0.000134133865285036,0.000151845157316633,
0.0001565184788544),.UNSPECIFIED.) ;
#2181=B_SPLINE_CURVE_WITH_KNOTS('',3,(#148278,#148279,#148280,#148281,#148282,
#148283,#148284,#148285,#148286,#148287,#148288,#148289,#148290,#148291,
#148292,#148293,#148294,#148295,#148296,#148297,#148298,#148299),
 .UNSPECIFIED.,.F.,.F.,(4,2,2,2,2,2,2,2,2,2,4),(-0.0842935807861705,-0.0841564125446822,
-0.08369584392567,-0.0829341785541707,-0.0805923611763772,-0.0773601159705437,
-0.0742136753202586,-0.0711238204987475,-0.0675672289962676,-0.0637829215465878,
-0.0629274139602073),.UNSPECIFIED.) ;
#2182=B_SPLINE_CURVE_WITH_KNOTS('',3,(#148462,#148463,#148464,#148465,#148466,
#148467,#148468,#148469),.UNSPECIFIED.,.F.,.F.,(4,2,2,4),(-0.0527017171621833,
-0.0518504523813524,-0.0480303917440445,-0.044675447368305),
 .UNSPECIFIED.) ;
#2183=B_SPLINE_CURVE_WITH_KNOTS('',3,(#148473,#148474,#148475,#148476,#148477,
#148478,#148479,#148480,#148481,#148482,#148483,#148484,#148485,#148486,
#148487,#148488,#148489,#148490,#148491,#148492,#148493,#148494,#148495,
#148496,#148497,#148498,#148499,#148500,#148501,#148502,#148503),
 .UNSPECIFIED.,.F.,.F.,(4,3,3,3,3,3,3,3,3,3,4),(0.,1.791148629847E-5,3.35636550441561E-5,
5.14128838689644E-5,6.71346369544058E-5,8.50076921954764E-5,0.000100614915215921,
0.000118595988596817,0.000134133865285032,0.000151845157316703,0.000156518478854398),
 .UNSPECIFIED.) ;
#2184=B_SPLINE_CURVE_WITH_KNOTS('',3,(#148505,#148506,#148507,#148508,#148509,
#148510,#148511,#148512,#148513,#148514,#148515,#148516,#148517,#148518,
#148519,#148520,#148521,#148522,#148523,#148524,#148525,#148526),
 .UNSPECIFIED.,.F.,.F.,(4,2,2,2,2,2,2,2,2,2,4),(-0.0842935807861705,-0.0841564125446822,
-0.08369584392567,-0.0829341785541707,-0.0805923611763772,-0.0773601159705437,
-0.0742136753202586,-0.0711238204987475,-0.0675672289962676,-0.0637829215465878,
-0.0629274139602073),.UNSPECIFIED.) ;
#2185=B_SPLINE_CURVE_WITH_KNOTS('',3,(#148689,#148690,#148691,#148692,#148693,
#148694,#148695,#148696),.UNSPECIFIED.,.F.,.F.,(4,2,2,4),(-0.0527017171619057,
-0.0518504523810739,-0.0480303917437878,-0.0446754473680843),
 .UNSPECIFIED.) ;
#2186=B_SPLINE_CURVE_WITH_KNOTS('',3,(#148700,#148701,#148702,#148703,#148704,
#148705,#148706,#148707,#148708,#148709,#148710,#148711,#148712,#148713,
#148714,#148715,#148716,#148717,#148718,#148719,#148720,#148721,#148722,
#148723,#148724,#148725,#148726,#148727,#148728,#148729,#148730),
 .UNSPECIFIED.,.F.,.F.,(4,3,3,3,3,3,3,3,3,3,4),(0.,1.79114862984022E-5,
3.35636550441561E-5,5.14128838690747E-5,6.71346369544058E-5,8.50076921955029E-5,
0.000100614915215921,0.000118595988596949,0.000134133865285032,0.000151845157316721,
0.000156518478854398),.UNSPECIFIED.) ;
#2187=B_SPLINE_CURVE_WITH_KNOTS('',3,(#148732,#148733,#148734,#148735,#148736,
#148737,#148738,#148739,#148740,#148741,#148742,#148743,#148744,#148745,
#148746,#148747,#148748,#148749,#148750,#148751,#148752,#148753),
 .UNSPECIFIED.,.F.,.F.,(4,2,2,2,2,2,2,2,2,2,4),(-0.0842935806846017,-0.0841564124433096,
-0.0836958438252493,-0.0829341784552694,-0.0805923610820353,-0.0773601158823278,
-0.0742136752378489,-0.07112382042188,-0.0675672289255957,-0.0637829214823062,
-0.0629274138973503),.UNSPECIFIED.) ;
#2188=B_SPLINE_CURVE_WITH_KNOTS('',3,(#148916,#148917,#148918,#148919,#148920,
#148921,#148922,#148923),.UNSPECIFIED.,.F.,.F.,(4,2,2,4),(-0.0527017171620534,
-0.0518504523812236,-0.0480303917439217,-0.0446754473681886),
 .UNSPECIFIED.) ;
#2189=B_SPLINE_CURVE_WITH_KNOTS('',3,(#148927,#148928,#148929,#148930,#148931,
#148932,#148933,#148934,#148935,#148936,#148937,#148938,#148939,#148940,
#148941,#148942,#148943,#148944,#148945,#148946,#148947,#148948,#148949,
#148950,#148951,#148952,#148953,#148954,#148955,#148956,#148957),
 .UNSPECIFIED.,.F.,.F.,(4,3,3,3,3,3,3,3,3,3,4),(0.,1.79114862984111E-5,
3.35636550441561E-5,5.1412883869035E-5,6.71346369544058E-5,8.50076921954072E-5,
0.000100614915215921,0.000118595988596959,0.000134133865285032,0.000151845157317271,
0.000156518478854398),.UNSPECIFIED.) ;
#2190=B_SPLINE_CURVE_WITH_KNOTS('',3,(#148959,#148960,#148961,#148962,#148963,
#148964,#148965,#148966,#148967,#148968,#148969,#148970,#148971,#148972,
#148973,#148974,#148975,#148976,#148977,#148978,#148979,#148980),
 .UNSPECIFIED.,.F.,.F.,(4,2,2,2,2,2,2,2,2,2,4),(-0.0842935807784001,-0.0841564125369118,
-0.0836958439179285,-0.0829341785465007,-0.080592361168928,-0.0773601159633862,
-0.0742136753133782,-0.071123820492143,-0.0675672289899856,-0.063782921540619,
-0.0629274139542864),.UNSPECIFIED.) ;
#2191=B_SPLINE_CURVE_WITH_KNOTS('',3,(#149143,#149144,#149145,#149146,#149147,
#149148,#149149,#149150),.UNSPECIFIED.,.F.,.F.,(4,2,2,4),(-0.0527017171619366,
-0.0518504523811075,-0.0480303917438238,-0.0446754473681228),
 .UNSPECIFIED.) ;
#2192=B_SPLINE_CURVE_WITH_KNOTS('',3,(#149154,#149155,#149156,#149157,#149158,
#149159,#149160,#149161,#149162,#149163,#149164,#149165,#149166,#149167,
#149168,#149169,#149170,#149171,#149172,#149173,#149174,#149175,#149176,
#149177,#149178,#149179,#149180,#149181,#149182,#149183,#149184),
 .UNSPECIFIED.,.F.,.F.,(4,3,3,3,3,3,3,3,3,3,4),(0.,1.7911486298388E-5,3.35636550441561E-5,
5.14128838690249E-5,6.71346369544058E-5,8.50076921954834E-5,0.000100614915215921,
0.000118595988596784,0.000134133865285032,0.000151845157317113,0.000156518478854398),
 .UNSPECIFIED.) ;
#2193=B_SPLINE_CURVE_WITH_KNOTS('',3,(#149186,#149187,#149188,#149189,#149190,
#149191,#149192,#149193,#149194,#149195,#149196,#149197,#149198,#149199,
#149200,#149201,#149202,#149203,#149204,#149205,#149206,#149207),
 .UNSPECIFIED.,.F.,.F.,(4,2,2,2,2,2,2,2,2,2,4),(-0.0842935807784001,-0.0841564125369118,
-0.0836958439179285,-0.0829341785465007,-0.080592361168928,-0.0773601159633862,
-0.0742136753133782,-0.071123820492143,-0.0675672289899856,-0.063782921540619,
-0.0629274139542864),.UNSPECIFIED.) ;
#2194=B_SPLINE_CURVE_WITH_KNOTS('',3,(#149370,#149371,#149372,#149373,#149374,
#149375,#149376,#149377),.UNSPECIFIED.,.F.,.F.,(4,2,2,4),(-0.0527017171617456,
-0.0518504523809185,-0.0480303917436524,-0.0446754473679689),
 .UNSPECIFIED.) ;
#2195=B_SPLINE_CURVE_WITH_KNOTS('',3,(#149381,#149382,#149383,#149384,#149385,
#149386,#149387,#149388,#149389,#149390,#149391,#149392,#149393,#149394,
#149395,#149396,#149397,#149398,#149399,#149400,#149401,#149402,#149403,
#149404,#149405,#149406,#149407,#149408,#149409,#149410,#149411),
 .UNSPECIFIED.,.F.,.F.,(4,3,3,3,3,3,3,3,3,3,4),(0.,1.79114862983986E-5,
3.35636550441583E-5,5.14128838688763E-5,6.71346369544075E-5,8.5007692195462E-5,
0.000100614915215918,0.000118595988596873,0.000134133865285036,0.000151845157315814,
0.000156518478854401),.UNSPECIFIED.) ;
#2196=B_SPLINE_CURVE_WITH_KNOTS('',3,(#149413,#149414,#149415,#149416,#149417,
#149418,#149419,#149420,#149421,#149422,#149423,#149424,#149425,#149426,
#149427,#149428,#149429,#149430,#149431,#149432,#149433,#149434),
 .UNSPECIFIED.,.F.,.F.,(4,2,2,2,2,2,2,2,2,2,4),(-0.0842935807784001,-0.0841564125369118,
-0.0836958439179285,-0.0829341785465007,-0.080592361168928,-0.0773601159633862,
-0.0742136753133782,-0.071123820492143,-0.0675672289899856,-0.063782921540619,
-0.0629274139542864),.UNSPECIFIED.) ;
#3629=LINE('',#141855,#9183) ;
#3630=LINE('',#141859,#9184) ;
#3631=LINE('',#141861,#9185) ;
#3632=LINE('',#141898,#9186) ;
#3633=LINE('',#141902,#9187) ;
#3634=LINE('',#141904,#9188) ;
#3635=LINE('',#141941,#9189) ;
#3636=LINE('',#141945,#9190) ;
#3637=LINE('',#141947,#9191) ;
#3638=LINE('',#141984,#9192) ;
#3639=LINE('',#141988,#9193) ;
#3640=LINE('',#141990,#9194) ;
#3641=LINE('',#142027,#9195) ;
#3642=LINE('',#142031,#9196) ;
#3643=LINE('',#142033,#9197) ;
#3644=LINE('',#142070,#9198) ;
#3645=LINE('',#142074,#9199) ;
#3646=LINE('',#142076,#9200) ;
#3647=LINE('',#142113,#9201) ;
#3648=LINE('',#142117,#9202) ;
#3649=LINE('',#142119,#9203) ;
#3650=LINE('',#142156,#9204) ;
#3651=LINE('',#142160,#9205) ;
#3652=LINE('',#142162,#9206) ;
#3653=LINE('',#142280,#9207) ;
#3654=LINE('',#142284,#9208) ;
#3655=LINE('',#142286,#9209) ;
#3656=LINE('',#142296,#9210) ;
#3657=LINE('',#142298,#9211) ;
#3658=LINE('',#142300,#9212) ;
#3659=LINE('',#142302,#9213) ;
#3660=LINE('',#142304,#9214) ;
#3661=LINE('',#142306,#9215) ;
#3662=LINE('',#142308,#9216) ;
#3663=LINE('',#142310,#9217) ;
#3664=LINE('',#142312,#9218) ;
#3665=LINE('',#142317,#9219) ;
#3666=LINE('',#142318,#9220) ;
#3667=LINE('',#142323,#9221) ;
#3668=LINE('',#142324,#9222) ;
#3669=LINE('',#142329,#9223) ;
#3670=LINE('',#142330,#9224) ;
#3671=LINE('',#142335,#9225) ;
#3672=LINE('',#142336,#9226) ;
#3673=LINE('',#142341,#9227) ;
#3674=LINE('',#142342,#9228) ;
#3675=LINE('',#142347,#9229) ;
#3676=LINE('',#142348,#9230) ;
#3677=LINE('',#142353,#9231) ;
#3678=LINE('',#142354,#9232) ;
#3679=LINE('',#142359,#9233) ;
#3680=LINE('',#142360,#9234) ;
#3681=LINE('',#142365,#9235) ;
#3682=LINE('',#142366,#9236) ;
#3683=LINE('',#142404,#9237) ;
#3684=LINE('',#142408,#9238) ;
#3685=LINE('',#142410,#9239) ;
#3686=LINE('',#142420,#9240) ;
#3687=LINE('',#142425,#9241) ;
#3688=LINE('',#142426,#9242) ;
#3689=LINE('',#142430,#9243) ;
#3690=LINE('',#142434,#9244) ;
#3691=LINE('',#142439,#9245) ;
#3692=LINE('',#142441,#9246) ;
#3693=LINE('',#142443,#9247) ;
#3694=LINE('',#142445,#9248) ;
#3695=LINE('',#142447,#9249) ;
#3696=LINE('',#142452,#9250) ;
#3697=LINE('',#142456,#9251) ;
#3698=LINE('',#142461,#9252) ;
#3699=LINE('',#142463,#9253) ;
#3700=LINE('',#142465,#9254) ;
#3701=LINE('',#142467,#9255) ;
#3702=LINE('',#142469,#9256) ;
#3703=LINE('',#142474,#9257) ;
#3704=LINE('',#142478,#9258) ;
#3705=LINE('',#142483,#9259) ;
#3706=LINE('',#142485,#9260) ;
#3707=LINE('',#142487,#9261) ;
#3708=LINE('',#142489,#9262) ;
#3709=LINE('',#142491,#9263) ;
#3710=LINE('',#142496,#9264) ;
#3711=LINE('',#142500,#9265) ;
#3712=LINE('',#142505,#9266) ;
#3713=LINE('',#142507,#9267) ;
#3714=LINE('',#142509,#9268) ;
#3715=LINE('',#142511,#9269) ;
#3716=LINE('',#142513,#9270) ;
#3717=LINE('',#142518,#9271) ;
#3718=LINE('',#142522,#9272) ;
#3719=LINE('',#142527,#9273) ;
#3720=LINE('',#142529,#9274) ;
#3721=LINE('',#142531,#9275) ;
#3722=LINE('',#142533,#9276) ;
#3723=LINE('',#142535,#9277) ;
#3724=LINE('',#142540,#9278) ;
#3725=LINE('',#142544,#9279) ;
#3726=LINE('',#142549,#9280) ;
#3727=LINE('',#142551,#9281) ;
#3728=LINE('',#142553,#9282) ;
#3729=LINE('',#142555,#9283) ;
#3730=LINE('',#142557,#9284) ;
#3731=LINE('',#142562,#9285) ;
#3732=LINE('',#142566,#9286) ;
#3733=LINE('',#142571,#9287) ;
#3734=LINE('',#142573,#9288) ;
#3735=LINE('',#142575,#9289) ;
#3736=LINE('',#142577,#9290) ;
#3737=LINE('',#142579,#9291) ;
#3738=LINE('',#142584,#9292) ;
#3739=LINE('',#142588,#9293) ;
#3740=LINE('',#142593,#9294) ;
#3741=LINE('',#142595,#9295) ;
#3742=LINE('',#142597,#9296) ;
#3743=LINE('',#142599,#9297) ;
#3744=LINE('',#142601,#9298) ;
#3745=LINE('',#142606,#9299) ;
#3746=LINE('',#142610,#9300) ;
#3747=LINE('',#142615,#9301) ;
#3748=LINE('',#142617,#9302) ;
#3749=LINE('',#142619,#9303) ;
#3750=LINE('',#142621,#9304) ;
#3751=LINE('',#142623,#9305) ;
#3752=LINE('',#142630,#9306) ;
#3753=LINE('',#142632,#9307) ;
#3754=LINE('',#142634,#9308) ;
#3755=LINE('',#142635,#9309) ;
#3756=LINE('',#142641,#9310) ;
#3757=LINE('',#142643,#9311) ;
#3758=LINE('',#142645,#9312) ;
#3759=LINE('',#142646,#9313) ;
#3760=LINE('',#142652,#9314) ;
#3761=LINE('',#142654,#9315) ;
#3762=LINE('',#142656,#9316) ;
#3763=LINE('',#142657,#9317) ;
#3764=LINE('',#142663,#9318) ;
#3765=LINE('',#142665,#9319) ;
#3766=LINE('',#142667,#9320) ;
#3767=LINE('',#142668,#9321) ;
#3768=LINE('',#142674,#9322) ;
#3769=LINE('',#142676,#9323) ;
#3770=LINE('',#142678,#9324) ;
#3771=LINE('',#142679,#9325) ;
#3772=LINE('',#142685,#9326) ;
#3773=LINE('',#142687,#9327) ;
#3774=LINE('',#142689,#9328) ;
#3775=LINE('',#142690,#9329) ;
#3776=LINE('',#142696,#9330) ;
#3777=LINE('',#142698,#9331) ;
#3778=LINE('',#142700,#9332) ;
#3779=LINE('',#142701,#9333) ;
#3780=LINE('',#142707,#9334) ;
#3781=LINE('',#142709,#9335) ;
#3782=LINE('',#142711,#9336) ;
#3783=LINE('',#142712,#9337) ;
#3784=LINE('',#142718,#9338) ;
#3785=LINE('',#142720,#9339) ;
#3786=LINE('',#142722,#9340) ;
#3787=LINE('',#142723,#9341) ;
#3788=LINE('',#142729,#9342) ;
#3789=LINE('',#142731,#9343) ;
#3790=LINE('',#142733,#9344) ;
#3791=LINE('',#142734,#9345) ;
#3792=LINE('',#142740,#9346) ;
#3793=LINE('',#142742,#9347) ;
#3794=LINE('',#142744,#9348) ;
#3795=LINE('',#142745,#9349) ;
#3796=LINE('',#142751,#9350) ;
#3797=LINE('',#142753,#9351) ;
#3798=LINE('',#142755,#9352) ;
#3799=LINE('',#142756,#9353) ;
#3800=LINE('',#142762,#9354) ;
#3801=LINE('',#142764,#9355) ;
#3802=LINE('',#142766,#9356) ;
#3803=LINE('',#142767,#9357) ;
#3804=LINE('',#142773,#9358) ;
#3805=LINE('',#142775,#9359) ;
#3806=LINE('',#142777,#9360) ;
#3807=LINE('',#142778,#9361) ;
#3808=LINE('',#142784,#9362) ;
#3809=LINE('',#142786,#9363) ;
#3810=LINE('',#142788,#9364) ;
#3811=LINE('',#142789,#9365) ;
#3812=LINE('',#142795,#9366) ;
#3813=LINE('',#142797,#9367) ;
#3814=LINE('',#142799,#9368) ;
#3815=LINE('',#142800,#9369) ;
#3816=LINE('',#142806,#9370) ;
#3817=LINE('',#142808,#9371) ;
#3818=LINE('',#142810,#9372) ;
#3819=LINE('',#142811,#9373) ;
#3820=LINE('',#142817,#9374) ;
#3821=LINE('',#142819,#9375) ;
#3822=LINE('',#142821,#9376) ;
#3823=LINE('',#142822,#9377) ;
#3824=LINE('',#142826,#9378) ;
#3825=LINE('',#142830,#9379) ;
#3826=LINE('',#142835,#9380) ;
#3827=LINE('',#142839,#9381) ;
#3828=LINE('',#142844,#9382) ;
#3829=LINE('',#142848,#9383) ;
#3830=LINE('',#142853,#9384) ;
#3831=LINE('',#142857,#9385) ;
#3832=LINE('',#142862,#9386) ;
#3833=LINE('',#142866,#9387) ;
#3834=LINE('',#142871,#9388) ;
#3835=LINE('',#142875,#9389) ;
#3836=LINE('',#142880,#9390) ;
#3837=LINE('',#142884,#9391) ;
#3838=LINE('',#142889,#9392) ;
#3839=LINE('',#142893,#9393) ;
#3840=LINE('',#142898,#9394) ;
#3841=LINE('',#142902,#9395) ;
#3842=LINE('',#142907,#9396) ;
#3843=LINE('',#142911,#9397) ;
#3844=LINE('',#142916,#9398) ;
#3845=LINE('',#142918,#9399) ;
#3846=LINE('',#142920,#9400) ;
#3847=LINE('',#142922,#9401) ;
#3848=LINE('',#142924,#9402) ;
#3849=LINE('',#142931,#9403) ;
#3850=LINE('',#142933,#9404) ;
#3851=LINE('',#142935,#9405) ;
#3852=LINE('',#142936,#9406) ;
#3853=LINE('',#142942,#9407) ;
#3854=LINE('',#142944,#9408) ;
#3855=LINE('',#142946,#9409) ;
#3856=LINE('',#142947,#9410) ;
#3857=LINE('',#142951,#9411) ;
#3858=LINE('',#142955,#9412) ;
#3859=LINE('',#142960,#9413) ;
#3860=LINE('',#142964,#9414) ;
#3861=LINE('',#142971,#9415) ;
#3862=LINE('',#142973,#9416) ;
#3863=LINE('',#142974,#9417) ;
#3864=LINE('',#142975,#9418) ;
#3865=LINE('',#142977,#9419) ;
#3866=LINE('',#142981,#9420) ;
#3867=LINE('',#142984,#9421) ;
#3868=LINE('',#142986,#9422) ;
#3869=LINE('',#142990,#9423) ;
#3870=LINE('',#142993,#9424) ;
#3871=LINE('',#142995,#9425) ;
#3872=LINE('',#142999,#9426) ;
#3873=LINE('',#143002,#9427) ;
#3874=LINE('',#143004,#9428) ;
#3875=LINE('',#143008,#9429) ;
#3876=LINE('',#143011,#9430) ;
#3877=LINE('',#143013,#9431) ;
#3878=LINE('',#143017,#9432) ;
#3879=LINE('',#143020,#9433) ;
#3880=LINE('',#143022,#9434) ;
#3881=LINE('',#143026,#9435) ;
#3882=LINE('',#143029,#9436) ;
#3883=LINE('',#143031,#9437) ;
#3884=LINE('',#143035,#9438) ;
#3885=LINE('',#143038,#9439) ;
#3886=LINE('',#143040,#9440) ;
#3887=LINE('',#143044,#9441) ;
#3888=LINE('',#143047,#9442) ;
#3889=LINE('',#143049,#9443) ;
#3890=LINE('',#143053,#9444) ;
#3891=LINE('',#143056,#9445) ;
#3892=LINE('',#143058,#9446) ;
#3893=LINE('',#143061,#9447) ;
#3894=LINE('',#143066,#9448) ;
#3895=LINE('',#143072,#9449) ;
#3896=LINE('',#143074,#9450) ;
#3897=LINE('',#143078,#9451) ;
#3898=LINE('',#143081,#9452) ;
#3899=LINE('',#143083,#9453) ;
#3900=LINE('',#143087,#9454) ;
#3901=LINE('',#143090,#9455) ;
#3902=LINE('',#143092,#9456) ;
#3903=LINE('',#143096,#9457) ;
#3904=LINE('',#143099,#9458) ;
#3905=LINE('',#143101,#9459) ;
#3906=LINE('',#143105,#9460) ;
#3907=LINE('',#143108,#9461) ;
#3908=LINE('',#143110,#9462) ;
#3909=LINE('',#143114,#9463) ;
#3910=LINE('',#143117,#9464) ;
#3911=LINE('',#143119,#9465) ;
#3912=LINE('',#143123,#9466) ;
#3913=LINE('',#143126,#9467) ;
#3914=LINE('',#143128,#9468) ;
#3915=LINE('',#143132,#9469) ;
#3916=LINE('',#143135,#9470) ;
#3917=LINE('',#143137,#9471) ;
#3918=LINE('',#143141,#9472) ;
#3919=LINE('',#143144,#9473) ;
#3920=LINE('',#143146,#9474) ;
#3921=LINE('',#143150,#9475) ;
#3922=LINE('',#143153,#9476) ;
#3923=LINE('',#143155,#9477) ;
#3924=LINE('',#143157,#9478) ;
#3925=LINE('',#143158,#9479) ;
#3926=LINE('',#143160,#9480) ;
#3927=LINE('',#143163,#9481) ;
#3928=LINE('',#143167,#9482) ;
#3929=LINE('',#143173,#9483) ;
#3930=LINE('',#143174,#9484) ;
#3931=LINE('',#143175,#9485) ;
#3932=LINE('',#143179,#9486) ;
#3933=LINE('',#143185,#9487) ;
#3934=LINE('',#143186,#9488) ;
#3935=LINE('',#143187,#9489) ;
#3936=LINE('',#143191,#9490) ;
#3937=LINE('',#143197,#9491) ;
#3938=LINE('',#143198,#9492) ;
#3939=LINE('',#143199,#9493) ;
#3940=LINE('',#143203,#9494) ;
#3941=LINE('',#143209,#9495) ;
#3942=LINE('',#143210,#9496) ;
#3943=LINE('',#143211,#9497) ;
#3944=LINE('',#143215,#9498) ;
#3945=LINE('',#143221,#9499) ;
#3946=LINE('',#143222,#9500) ;
#3947=LINE('',#143223,#9501) ;
#3948=LINE('',#143227,#9502) ;
#3949=LINE('',#143231,#9503) ;
#3950=LINE('',#143232,#9504) ;
#3951=LINE('',#143237,#9505) ;
#3952=LINE('',#143239,#9506) ;
#3953=LINE('',#143241,#9507) ;
#3954=LINE('',#143245,#9508) ;
#3955=LINE('',#143248,#9509) ;
#3956=LINE('',#143250,#9510) ;
#3957=LINE('',#143254,#9511) ;
#3958=LINE('',#143256,#9512) ;
#3959=LINE('',#143258,#9513) ;
#3960=LINE('',#143262,#9514) ;
#3961=LINE('',#143266,#9515) ;
#3962=LINE('',#143274,#9516) ;
#3963=LINE('',#143277,#9517) ;
#3964=LINE('',#143282,#9518) ;
#3965=LINE('',#143284,#9519) ;
#3966=LINE('',#143286,#9520) ;
#3967=LINE('',#143290,#9521) ;
#3968=LINE('',#143293,#9522) ;
#3969=LINE('',#143295,#9523) ;
#3970=LINE('',#143299,#9524) ;
#3971=LINE('',#143301,#9525) ;
#3972=LINE('',#143303,#9526) ;
#3973=LINE('',#143307,#9527) ;
#3974=LINE('',#143311,#9528) ;
#3975=LINE('',#143319,#9529) ;
#3976=LINE('',#143322,#9530) ;
#3977=LINE('',#143327,#9531) ;
#3978=LINE('',#143329,#9532) ;
#3979=LINE('',#143331,#9533) ;
#3980=LINE('',#143335,#9534) ;
#3981=LINE('',#143338,#9535) ;
#3982=LINE('',#143340,#9536) ;
#3983=LINE('',#143344,#9537) ;
#3984=LINE('',#143346,#9538) ;
#3985=LINE('',#143348,#9539) ;
#3986=LINE('',#143352,#9540) ;
#3987=LINE('',#143356,#9541) ;
#3988=LINE('',#143364,#9542) ;
#3989=LINE('',#143367,#9543) ;
#3990=LINE('',#143372,#9544) ;
#3991=LINE('',#143374,#9545) ;
#3992=LINE('',#143376,#9546) ;
#3993=LINE('',#143380,#9547) ;
#3994=LINE('',#143383,#9548) ;
#3995=LINE('',#143385,#9549) ;
#3996=LINE('',#143389,#9550) ;
#3997=LINE('',#143391,#9551) ;
#3998=LINE('',#143393,#9552) ;
#3999=LINE('',#143397,#9553) ;
#4000=LINE('',#143401,#9554) ;
#4001=LINE('',#143409,#9555) ;
#4002=LINE('',#143412,#9556) ;
#4003=LINE('',#143417,#9557) ;
#4004=LINE('',#143419,#9558) ;
#4005=LINE('',#143421,#9559) ;
#4006=LINE('',#143425,#9560) ;
#4007=LINE('',#143428,#9561) ;
#4008=LINE('',#143430,#9562) ;
#4009=LINE('',#143434,#9563) ;
#4010=LINE('',#143436,#9564) ;
#4011=LINE('',#143438,#9565) ;
#4012=LINE('',#143442,#9566) ;
#4013=LINE('',#143446,#9567) ;
#4014=LINE('',#143454,#9568) ;
#4015=LINE('',#143457,#9569) ;
#4016=LINE('',#143462,#9570) ;
#4017=LINE('',#143464,#9571) ;
#4018=LINE('',#143466,#9572) ;
#4019=LINE('',#143470,#9573) ;
#4020=LINE('',#143473,#9574) ;
#4021=LINE('',#143475,#9575) ;
#4022=LINE('',#143479,#9576) ;
#4023=LINE('',#143481,#9577) ;
#4024=LINE('',#143483,#9578) ;
#4025=LINE('',#143487,#9579) ;
#4026=LINE('',#143491,#9580) ;
#4027=LINE('',#143499,#9581) ;
#4028=LINE('',#143502,#9582) ;
#4029=LINE('',#143507,#9583) ;
#4030=LINE('',#143509,#9584) ;
#4031=LINE('',#143511,#9585) ;
#4032=LINE('',#143515,#9586) ;
#4033=LINE('',#143518,#9587) ;
#4034=LINE('',#143520,#9588) ;
#4035=LINE('',#143524,#9589) ;
#4036=LINE('',#143526,#9590) ;
#4037=LINE('',#143528,#9591) ;
#4038=LINE('',#143532,#9592) ;
#4039=LINE('',#143536,#9593) ;
#4040=LINE('',#143544,#9594) ;
#4041=LINE('',#143547,#9595) ;
#4042=LINE('',#143552,#9596) ;
#4043=LINE('',#143554,#9597) ;
#4044=LINE('',#143556,#9598) ;
#4045=LINE('',#143560,#9599) ;
#4046=LINE('',#143563,#9600) ;
#4047=LINE('',#143565,#9601) ;
#4048=LINE('',#143569,#9602) ;
#4049=LINE('',#143571,#9603) ;
#4050=LINE('',#143573,#9604) ;
#4051=LINE('',#143577,#9605) ;
#4052=LINE('',#143581,#9606) ;
#4053=LINE('',#143589,#9607) ;
#4054=LINE('',#143592,#9608) ;
#4055=LINE('',#143597,#9609) ;
#4056=LINE('',#143599,#9610) ;
#4057=LINE('',#143601,#9611) ;
#4058=LINE('',#143605,#9612) ;
#4059=LINE('',#143608,#9613) ;
#4060=LINE('',#143610,#9614) ;
#4061=LINE('',#143614,#9615) ;
#4062=LINE('',#143616,#9616) ;
#4063=LINE('',#143618,#9617) ;
#4064=LINE('',#143622,#9618) ;
#4065=LINE('',#143626,#9619) ;
#4066=LINE('',#143634,#9620) ;
#4067=LINE('',#143637,#9621) ;
#4068=LINE('',#143642,#9622) ;
#4069=LINE('',#143644,#9623) ;
#4070=LINE('',#143646,#9624) ;
#4071=LINE('',#143650,#9625) ;
#4072=LINE('',#143653,#9626) ;
#4073=LINE('',#143655,#9627) ;
#4074=LINE('',#143659,#9628) ;
#4075=LINE('',#143661,#9629) ;
#4076=LINE('',#143663,#9630) ;
#4077=LINE('',#143667,#9631) ;
#4078=LINE('',#143671,#9632) ;
#4079=LINE('',#143679,#9633) ;
#4080=LINE('',#143682,#9634) ;
#4081=LINE('',#143686,#9635) ;
#4082=LINE('',#143688,#9636) ;
#4083=LINE('',#143690,#9637) ;
#4084=LINE('',#143692,#9638) ;
#4085=LINE('',#143696,#9639) ;
#4086=LINE('',#143698,#9640) ;
#4087=LINE('',#143700,#9641) ;
#4088=LINE('',#143703,#9642) ;
#4089=LINE('',#143707,#9643) ;
#4090=LINE('',#143709,#9644) ;
#4091=LINE('',#143711,#9645) ;
#4092=LINE('',#143713,#9646) ;
#4093=LINE('',#143717,#9647) ;
#4094=LINE('',#143719,#9648) ;
#4095=LINE('',#143721,#9649) ;
#4096=LINE('',#143724,#9650) ;
#4097=LINE('',#143728,#9651) ;
#4098=LINE('',#143730,#9652) ;
#4099=LINE('',#143732,#9653) ;
#4100=LINE('',#143734,#9654) ;
#4101=LINE('',#143736,#9655) ;
#4102=LINE('',#143738,#9656) ;
#4103=LINE('',#143742,#9657) ;
#4104=LINE('',#143745,#9658) ;
#4105=LINE('',#143749,#9659) ;
#4106=LINE('',#143751,#9660) ;
#4107=LINE('',#143753,#9661) ;
#4108=LINE('',#143754,#9662) ;
#4109=LINE('',#143757,#9663) ;
#4110=LINE('',#143759,#9664) ;
#4111=LINE('',#143760,#9665) ;
#4112=LINE('',#143764,#9666) ;
#4113=LINE('',#143766,#9667) ;
#4114=LINE('',#143768,#9668) ;
#4115=LINE('',#143769,#9669) ;
#4116=LINE('',#143773,#9670) ;
#4117=LINE('',#143775,#9671) ;
#4118=LINE('',#143777,#9672) ;
#4119=LINE('',#143778,#9673) ;
#4120=LINE('',#143782,#9674) ;
#4121=LINE('',#143784,#9675) ;
#4122=LINE('',#143786,#9676) ;
#4123=LINE('',#143787,#9677) ;
#4124=LINE('',#143791,#9678) ;
#4125=LINE('',#143795,#9679) ;
#4126=LINE('',#143799,#9680) ;
#4127=LINE('',#143801,#9681) ;
#4128=LINE('',#143802,#9682) ;
#4129=LINE('',#143807,#9683) ;
#4130=LINE('',#143811,#9684) ;
#4131=LINE('',#143813,#9685) ;
#4132=LINE('',#143814,#9686) ;
#4133=LINE('',#143819,#9687) ;
#4134=LINE('',#143822,#9688) ;
#4135=LINE('',#143824,#9689) ;
#4136=LINE('',#143825,#9690) ;
#4137=LINE('',#143828,#9691) ;
#4138=LINE('',#143831,#9692) ;
#4139=LINE('',#143832,#9693) ;
#4140=LINE('',#143835,#9694) ;
#4141=LINE('',#143837,#9695) ;
#4142=LINE('',#143838,#9696) ;
#4143=LINE('',#143843,#9697) ;
#4144=LINE('',#143847,#9698) ;
#4145=LINE('',#143849,#9699) ;
#4146=LINE('',#143850,#9700) ;
#4147=LINE('',#143855,#9701) ;
#4148=LINE('',#143859,#9702) ;
#4149=LINE('',#143861,#9703) ;
#4150=LINE('',#143862,#9704) ;
#4151=LINE('',#143867,#9705) ;
#4152=LINE('',#143871,#9706) ;
#4153=LINE('',#143873,#9707) ;
#4154=LINE('',#143874,#9708) ;
#4155=LINE('',#143879,#9709) ;
#4156=LINE('',#143883,#9710) ;
#4157=LINE('',#143885,#9711) ;
#4158=LINE('',#143886,#9712) ;
#4159=LINE('',#143891,#9713) ;
#4160=LINE('',#143895,#9714) ;
#4161=LINE('',#143897,#9715) ;
#4162=LINE('',#143898,#9716) ;
#4163=LINE('',#143903,#9717) ;
#4164=LINE('',#143909,#9718) ;
#4165=LINE('',#143915,#9719) ;
#4166=LINE('',#143919,#9720) ;
#4167=LINE('',#143921,#9721) ;
#4168=LINE('',#143922,#9722) ;
#4169=LINE('',#143927,#9723) ;
#4170=LINE('',#143931,#9724) ;
#4171=LINE('',#143933,#9725) ;
#4172=LINE('',#143934,#9726) ;
#4173=LINE('',#143939,#9727) ;
#4174=LINE('',#143942,#9728) ;
#4175=LINE('',#143943,#9729) ;
#4176=LINE('',#143949,#9730) ;
#4177=LINE('',#143953,#9731) ;
#4178=LINE('',#143955,#9732) ;
#4179=LINE('',#143957,#9733) ;
#4180=LINE('',#143961,#9734) ;
#4181=LINE('',#143963,#9735) ;
#4182=LINE('',#143965,#9736) ;
#4183=LINE('',#143969,#9737) ;
#4184=LINE('',#143973,#9738) ;
#4185=LINE('',#143975,#9739) ;
#4186=LINE('',#143976,#9740) ;
#4187=LINE('',#143978,#9741) ;
#4188=LINE('',#143979,#9742) ;
#4189=LINE('',#143983,#9743) ;
#4190=LINE('',#143987,#9744) ;
#4191=LINE('',#143991,#9745) ;
#4192=LINE('',#143995,#9746) ;
#4193=LINE('',#144023,#9747) ;
#4194=LINE('',#144080,#9748) ;
#4195=LINE('',#144105,#9749) ;
#4196=LINE('',#144137,#9750) ;
#4197=LINE('',#144163,#9751) ;
#4198=LINE('',#144344,#9752) ;
#4199=LINE('',#144346,#9753) ;
#4200=LINE('',#144348,#9754) ;
#4201=LINE('',#144349,#9755) ;
#4202=LINE('',#144353,#9756) ;
#4203=LINE('',#144355,#9757) ;
#4204=LINE('',#144357,#9758) ;
#4205=LINE('',#144358,#9759) ;
#4206=LINE('',#144362,#9760) ;
#4207=LINE('',#144364,#9761) ;
#4208=LINE('',#144366,#9762) ;
#4209=LINE('',#144367,#9763) ;
#4210=LINE('',#144371,#9764) ;
#4211=LINE('',#144373,#9765) ;
#4212=LINE('',#144375,#9766) ;
#4213=LINE('',#144376,#9767) ;
#4214=LINE('',#144380,#9768) ;
#4215=LINE('',#144382,#9769) ;
#4216=LINE('',#144384,#9770) ;
#4217=LINE('',#144385,#9771) ;
#4218=LINE('',#144389,#9772) ;
#4219=LINE('',#144394,#9773) ;
#4220=LINE('',#144395,#9774) ;
#4221=LINE('',#144399,#9775) ;
#4222=LINE('',#144404,#9776) ;
#4223=LINE('',#144405,#9777) ;
#4224=LINE('',#144415,#9778) ;
#4225=LINE('',#144417,#9779) ;
#4226=LINE('',#144419,#9780) ;
#4227=LINE('',#144420,#9781) ;
#4228=LINE('',#144424,#9782) ;
#4229=LINE('',#144425,#9783) ;
#4230=LINE('',#144426,#9784) ;
#4231=LINE('',#144429,#9785) ;
#4232=LINE('',#144431,#9786) ;
#4233=LINE('',#144432,#9787) ;
#4234=LINE('',#144436,#9788) ;
#4235=LINE('',#144438,#9789) ;
#4236=LINE('',#144440,#9790) ;
#4237=LINE('',#144441,#9791) ;
#4238=LINE('',#144445,#9792) ;
#4239=LINE('',#144447,#9793) ;
#4240=LINE('',#144449,#9794) ;
#4241=LINE('',#144450,#9795) ;
#4242=LINE('',#144454,#9796) ;
#4243=LINE('',#144455,#9797) ;
#4244=LINE('',#144456,#9798) ;
#4245=LINE('',#144459,#9799) ;
#4246=LINE('',#144461,#9800) ;
#4247=LINE('',#144462,#9801) ;
#4248=LINE('',#144466,#9802) ;
#4249=LINE('',#144468,#9803) ;
#4250=LINE('',#144470,#9804) ;
#4251=LINE('',#144471,#9805) ;
#4252=LINE('',#144475,#9806) ;
#4253=LINE('',#144477,#9807) ;
#4254=LINE('',#144479,#9808) ;
#4255=LINE('',#144480,#9809) ;
#4256=LINE('',#144484,#9810) ;
#4257=LINE('',#144486,#9811) ;
#4258=LINE('',#144488,#9812) ;
#4259=LINE('',#144489,#9813) ;
#4260=LINE('',#144493,#9814) ;
#4261=LINE('',#144495,#9815) ;
#4262=LINE('',#144497,#9816) ;
#4263=LINE('',#144498,#9817) ;
#4264=LINE('',#144614,#9818) ;
#4265=LINE('',#144616,#9819) ;
#4266=LINE('',#144618,#9820) ;
#4267=LINE('',#144620,#9821) ;
#4268=LINE('',#144622,#9822) ;
#4269=LINE('',#144624,#9823) ;
#4270=LINE('',#144628,#9824) ;
#4271=LINE('',#144631,#9825) ;
#4272=LINE('',#144635,#9826) ;
#4273=LINE('',#144637,#9827) ;
#4274=LINE('',#144639,#9828) ;
#4275=LINE('',#144641,#9829) ;
#4276=LINE('',#144643,#9830) ;
#4277=LINE('',#144645,#9831) ;
#4278=LINE('',#144649,#9832) ;
#4279=LINE('',#144652,#9833) ;
#4280=LINE('',#144656,#9834) ;
#4281=LINE('',#144658,#9835) ;
#4282=LINE('',#144660,#9836) ;
#4283=LINE('',#144662,#9837) ;
#4284=LINE('',#144664,#9838) ;
#4285=LINE('',#144666,#9839) ;
#4286=LINE('',#144670,#9840) ;
#4287=LINE('',#144673,#9841) ;
#4288=LINE('',#144677,#9842) ;
#4289=LINE('',#144679,#9843) ;
#4290=LINE('',#144681,#9844) ;
#4291=LINE('',#144683,#9845) ;
#4292=LINE('',#144685,#9846) ;
#4293=LINE('',#144687,#9847) ;
#4294=LINE('',#144691,#9848) ;
#4295=LINE('',#144694,#9849) ;
#4296=LINE('',#144698,#9850) ;
#4297=LINE('',#144700,#9851) ;
#4298=LINE('',#144702,#9852) ;
#4299=LINE('',#144704,#9853) ;
#4300=LINE('',#144706,#9854) ;
#4301=LINE('',#144708,#9855) ;
#4302=LINE('',#144712,#9856) ;
#4303=LINE('',#144715,#9857) ;
#4304=LINE('',#144719,#9858) ;
#4305=LINE('',#144721,#9859) ;
#4306=LINE('',#144723,#9860) ;
#4307=LINE('',#144725,#9861) ;
#4308=LINE('',#144727,#9862) ;
#4309=LINE('',#144729,#9863) ;
#4310=LINE('',#144733,#9864) ;
#4311=LINE('',#144736,#9865) ;
#4312=LINE('',#144740,#9866) ;
#4313=LINE('',#144742,#9867) ;
#4314=LINE('',#144744,#9868) ;
#4315=LINE('',#144746,#9869) ;
#4316=LINE('',#144748,#9870) ;
#4317=LINE('',#144750,#9871) ;
#4318=LINE('',#144754,#9872) ;
#4319=LINE('',#144757,#9873) ;
#4320=LINE('',#144761,#9874) ;
#4321=LINE('',#144763,#9875) ;
#4322=LINE('',#144765,#9876) ;
#4323=LINE('',#144767,#9877) ;
#4324=LINE('',#144769,#9878) ;
#4325=LINE('',#144771,#9879) ;
#4326=LINE('',#144775,#9880) ;
#4327=LINE('',#144778,#9881) ;
#4328=LINE('',#144782,#9882) ;
#4329=LINE('',#144784,#9883) ;
#4330=LINE('',#144786,#9884) ;
#4331=LINE('',#144788,#9885) ;
#4332=LINE('',#144790,#9886) ;
#4333=LINE('',#144792,#9887) ;
#4334=LINE('',#144796,#9888) ;
#4335=LINE('',#144799,#9889) ;
#4336=LINE('',#144803,#9890) ;
#4337=LINE('',#144805,#9891) ;
#4338=LINE('',#144807,#9892) ;
#4339=LINE('',#144808,#9893) ;
#4340=LINE('',#144811,#9894) ;
#4341=LINE('',#144813,#9895) ;
#4342=LINE('',#144814,#9896) ;
#4343=LINE('',#144818,#9897) ;
#4344=LINE('',#144820,#9898) ;
#4345=LINE('',#144822,#9899) ;
#4346=LINE('',#144823,#9900) ;
#4347=LINE('',#144827,#9901) ;
#4348=LINE('',#144829,#9902) ;
#4349=LINE('',#144831,#9903) ;
#4350=LINE('',#144832,#9904) ;
#4351=LINE('',#144836,#9905) ;
#4352=LINE('',#144838,#9906) ;
#4353=LINE('',#144840,#9907) ;
#4354=LINE('',#144841,#9908) ;
#4355=LINE('',#144845,#9909) ;
#4356=LINE('',#144847,#9910) ;
#4357=LINE('',#144849,#9911) ;
#4358=LINE('',#144850,#9912) ;
#4359=LINE('',#144853,#9913) ;
#4360=LINE('',#144855,#9914) ;
#4361=LINE('',#144856,#9915) ;
#4362=LINE('',#144860,#9916) ;
#4363=LINE('',#144862,#9917) ;
#4364=LINE('',#144864,#9918) ;
#4365=LINE('',#144865,#9919) ;
#4366=LINE('',#144869,#9920) ;
#4367=LINE('',#144871,#9921) ;
#4368=LINE('',#144873,#9922) ;
#4369=LINE('',#144874,#9923) ;
#4370=LINE('',#144878,#9924) ;
#4371=LINE('',#144880,#9925) ;
#4372=LINE('',#144882,#9926) ;
#4373=LINE('',#144883,#9927) ;
#4374=LINE('',#144887,#9928) ;
#4375=LINE('',#144889,#9929) ;
#4376=LINE('',#144891,#9930) ;
#4377=LINE('',#144892,#9931) ;
#4378=LINE('',#144895,#9932) ;
#4379=LINE('',#144897,#9933) ;
#4380=LINE('',#144898,#9934) ;
#4381=LINE('',#144902,#9935) ;
#4382=LINE('',#144904,#9936) ;
#4383=LINE('',#144906,#9937) ;
#4384=LINE('',#144907,#9938) ;
#4385=LINE('',#144911,#9939) ;
#4386=LINE('',#144913,#9940) ;
#4387=LINE('',#144915,#9941) ;
#4388=LINE('',#144916,#9942) ;
#4389=LINE('',#144920,#9943) ;
#4390=LINE('',#144922,#9944) ;
#4391=LINE('',#144924,#9945) ;
#4392=LINE('',#144925,#9946) ;
#4393=LINE('',#144929,#9947) ;
#4394=LINE('',#144931,#9948) ;
#4395=LINE('',#144933,#9949) ;
#4396=LINE('',#144934,#9950) ;
#4397=LINE('',#144937,#9951) ;
#4398=LINE('',#144939,#9952) ;
#4399=LINE('',#144940,#9953) ;
#4400=LINE('',#144944,#9954) ;
#4401=LINE('',#144946,#9955) ;
#4402=LINE('',#144948,#9956) ;
#4403=LINE('',#144949,#9957) ;
#4404=LINE('',#144953,#9958) ;
#4405=LINE('',#144955,#9959) ;
#4406=LINE('',#144957,#9960) ;
#4407=LINE('',#144958,#9961) ;
#4408=LINE('',#144962,#9962) ;
#4409=LINE('',#144964,#9963) ;
#4410=LINE('',#144966,#9964) ;
#4411=LINE('',#144967,#9965) ;
#4412=LINE('',#144971,#9966) ;
#4413=LINE('',#144973,#9967) ;
#4414=LINE('',#144975,#9968) ;
#4415=LINE('',#144976,#9969) ;
#4416=LINE('',#144979,#9970) ;
#4417=LINE('',#144981,#9971) ;
#4418=LINE('',#144982,#9972) ;
#4419=LINE('',#144986,#9973) ;
#4420=LINE('',#144988,#9974) ;
#4421=LINE('',#144990,#9975) ;
#4422=LINE('',#144991,#9976) ;
#4423=LINE('',#144995,#9977) ;
#4424=LINE('',#144997,#9978) ;
#4425=LINE('',#144999,#9979) ;
#4426=LINE('',#145000,#9980) ;
#4427=LINE('',#145004,#9981) ;
#4428=LINE('',#145006,#9982) ;
#4429=LINE('',#145008,#9983) ;
#4430=LINE('',#145009,#9984) ;
#4431=LINE('',#145013,#9985) ;
#4432=LINE('',#145015,#9986) ;
#4433=LINE('',#145017,#9987) ;
#4434=LINE('',#145018,#9988) ;
#4435=LINE('',#145021,#9989) ;
#4436=LINE('',#145023,#9990) ;
#4437=LINE('',#145024,#9991) ;
#4438=LINE('',#145028,#9992) ;
#4439=LINE('',#145030,#9993) ;
#4440=LINE('',#145032,#9994) ;
#4441=LINE('',#145033,#9995) ;
#4442=LINE('',#145037,#9996) ;
#4443=LINE('',#145039,#9997) ;
#4444=LINE('',#145041,#9998) ;
#4445=LINE('',#145042,#9999) ;
#4446=LINE('',#145046,#10000) ;
#4447=LINE('',#145048,#10001) ;
#4448=LINE('',#145050,#10002) ;
#4449=LINE('',#145051,#10003) ;
#4450=LINE('',#145055,#10004) ;
#4451=LINE('',#145057,#10005) ;
#4452=LINE('',#145059,#10006) ;
#4453=LINE('',#145060,#10007) ;
#4454=LINE('',#145063,#10008) ;
#4455=LINE('',#145065,#10009) ;
#4456=LINE('',#145066,#10010) ;
#4457=LINE('',#145070,#10011) ;
#4458=LINE('',#145072,#10012) ;
#4459=LINE('',#145074,#10013) ;
#4460=LINE('',#145075,#10014) ;
#4461=LINE('',#145079,#10015) ;
#4462=LINE('',#145081,#10016) ;
#4463=LINE('',#145083,#10017) ;
#4464=LINE('',#145084,#10018) ;
#4465=LINE('',#145088,#10019) ;
#4466=LINE('',#145090,#10020) ;
#4467=LINE('',#145092,#10021) ;
#4468=LINE('',#145093,#10022) ;
#4469=LINE('',#145097,#10023) ;
#4470=LINE('',#145099,#10024) ;
#4471=LINE('',#145101,#10025) ;
#4472=LINE('',#145102,#10026) ;
#4473=LINE('',#145105,#10027) ;
#4474=LINE('',#145107,#10028) ;
#4475=LINE('',#145108,#10029) ;
#4476=LINE('',#145112,#10030) ;
#4477=LINE('',#145114,#10031) ;
#4478=LINE('',#145116,#10032) ;
#4479=LINE('',#145117,#10033) ;
#4480=LINE('',#145121,#10034) ;
#4481=LINE('',#145123,#10035) ;
#4482=LINE('',#145125,#10036) ;
#4483=LINE('',#145126,#10037) ;
#4484=LINE('',#145130,#10038) ;
#4485=LINE('',#145132,#10039) ;
#4486=LINE('',#145134,#10040) ;
#4487=LINE('',#145135,#10041) ;
#4488=LINE('',#145139,#10042) ;
#4489=LINE('',#145141,#10043) ;
#4490=LINE('',#145143,#10044) ;
#4491=LINE('',#145144,#10045) ;
#4492=LINE('',#145147,#10046) ;
#4493=LINE('',#145149,#10047) ;
#4494=LINE('',#145150,#10048) ;
#4495=LINE('',#145154,#10049) ;
#4496=LINE('',#145156,#10050) ;
#4497=LINE('',#145158,#10051) ;
#4498=LINE('',#145159,#10052) ;
#4499=LINE('',#145163,#10053) ;
#4500=LINE('',#145165,#10054) ;
#4501=LINE('',#145167,#10055) ;
#4502=LINE('',#145168,#10056) ;
#4503=LINE('',#145172,#10057) ;
#4504=LINE('',#145174,#10058) ;
#4505=LINE('',#145176,#10059) ;
#4506=LINE('',#145177,#10060) ;
#4507=LINE('',#145181,#10061) ;
#4508=LINE('',#145185,#10062) ;
#4509=LINE('',#145189,#10063) ;
#4510=LINE('',#145191,#10064) ;
#4511=LINE('',#145192,#10065) ;
#4512=LINE('',#145197,#10066) ;
#4513=LINE('',#145201,#10067) ;
#4514=LINE('',#145203,#10068) ;
#4515=LINE('',#145204,#10069) ;
#4516=LINE('',#145209,#10070) ;
#4517=LINE('',#145212,#10071) ;
#4518=LINE('',#145214,#10072) ;
#4519=LINE('',#145215,#10073) ;
#4520=LINE('',#145218,#10074) ;
#4521=LINE('',#145221,#10075) ;
#4522=LINE('',#145222,#10076) ;
#4523=LINE('',#145225,#10077) ;
#4524=LINE('',#145227,#10078) ;
#4525=LINE('',#145228,#10079) ;
#4526=LINE('',#145233,#10080) ;
#4527=LINE('',#145237,#10081) ;
#4528=LINE('',#145239,#10082) ;
#4529=LINE('',#145240,#10083) ;
#4530=LINE('',#145245,#10084) ;
#4531=LINE('',#145249,#10085) ;
#4532=LINE('',#145251,#10086) ;
#4533=LINE('',#145252,#10087) ;
#4534=LINE('',#145257,#10088) ;
#4535=LINE('',#145261,#10089) ;
#4536=LINE('',#145263,#10090) ;
#4537=LINE('',#145264,#10091) ;
#4538=LINE('',#145269,#10092) ;
#4539=LINE('',#145273,#10093) ;
#4540=LINE('',#145275,#10094) ;
#4541=LINE('',#145276,#10095) ;
#4542=LINE('',#145281,#10096) ;
#4543=LINE('',#145285,#10097) ;
#4544=LINE('',#145287,#10098) ;
#4545=LINE('',#145288,#10099) ;
#4546=LINE('',#145293,#10100) ;
#4547=LINE('',#145299,#10101) ;
#4548=LINE('',#145305,#10102) ;
#4549=LINE('',#145309,#10103) ;
#4550=LINE('',#145311,#10104) ;
#4551=LINE('',#145312,#10105) ;
#4552=LINE('',#145317,#10106) ;
#4553=LINE('',#145321,#10107) ;
#4554=LINE('',#145323,#10108) ;
#4555=LINE('',#145324,#10109) ;
#4556=LINE('',#145329,#10110) ;
#4557=LINE('',#145332,#10111) ;
#4558=LINE('',#145333,#10112) ;
#4559=LINE('',#145339,#10113) ;
#4560=LINE('',#145343,#10114) ;
#4561=LINE('',#145345,#10115) ;
#4562=LINE('',#145347,#10116) ;
#4563=LINE('',#145351,#10117) ;
#4564=LINE('',#145353,#10118) ;
#4565=LINE('',#145355,#10119) ;
#4566=LINE('',#145359,#10120) ;
#4567=LINE('',#145363,#10121) ;
#4568=LINE('',#145365,#10122) ;
#4569=LINE('',#145366,#10123) ;
#4570=LINE('',#145368,#10124) ;
#4571=LINE('',#145369,#10125) ;
#4572=LINE('',#145373,#10126) ;
#4573=LINE('',#145377,#10127) ;
#4574=LINE('',#145381,#10128) ;
#4575=LINE('',#145383,#10129) ;
#4576=LINE('',#145384,#10130) ;
#4577=LINE('',#145389,#10131) ;
#4578=LINE('',#145393,#10132) ;
#4579=LINE('',#145395,#10133) ;
#4580=LINE('',#145396,#10134) ;
#4581=LINE('',#145401,#10135) ;
#4582=LINE('',#145404,#10136) ;
#4583=LINE('',#145406,#10137) ;
#4584=LINE('',#145407,#10138) ;
#4585=LINE('',#145410,#10139) ;
#4586=LINE('',#145413,#10140) ;
#4587=LINE('',#145414,#10141) ;
#4588=LINE('',#145417,#10142) ;
#4589=LINE('',#145419,#10143) ;
#4590=LINE('',#145420,#10144) ;
#4591=LINE('',#145425,#10145) ;
#4592=LINE('',#145429,#10146) ;
#4593=LINE('',#145431,#10147) ;
#4594=LINE('',#145432,#10148) ;
#4595=LINE('',#145437,#10149) ;
#4596=LINE('',#145441,#10150) ;
#4597=LINE('',#145443,#10151) ;
#4598=LINE('',#145444,#10152) ;
#4599=LINE('',#145449,#10153) ;
#4600=LINE('',#145453,#10154) ;
#4601=LINE('',#145455,#10155) ;
#4602=LINE('',#145456,#10156) ;
#4603=LINE('',#145461,#10157) ;
#4604=LINE('',#145465,#10158) ;
#4605=LINE('',#145467,#10159) ;
#4606=LINE('',#145468,#10160) ;
#4607=LINE('',#145473,#10161) ;
#4608=LINE('',#145477,#10162) ;
#4609=LINE('',#145479,#10163) ;
#4610=LINE('',#145480,#10164) ;
#4611=LINE('',#145485,#10165) ;
#4612=LINE('',#145491,#10166) ;
#4613=LINE('',#145497,#10167) ;
#4614=LINE('',#145501,#10168) ;
#4615=LINE('',#145503,#10169) ;
#4616=LINE('',#145504,#10170) ;
#4617=LINE('',#145509,#10171) ;
#4618=LINE('',#145513,#10172) ;
#4619=LINE('',#145515,#10173) ;
#4620=LINE('',#145516,#10174) ;
#4621=LINE('',#145521,#10175) ;
#4622=LINE('',#145524,#10176) ;
#4623=LINE('',#145525,#10177) ;
#4624=LINE('',#145531,#10178) ;
#4625=LINE('',#145535,#10179) ;
#4626=LINE('',#145537,#10180) ;
#4627=LINE('',#145539,#10181) ;
#4628=LINE('',#145543,#10182) ;
#4629=LINE('',#145545,#10183) ;
#4630=LINE('',#145547,#10184) ;
#4631=LINE('',#145551,#10185) ;
#4632=LINE('',#145555,#10186) ;
#4633=LINE('',#145557,#10187) ;
#4634=LINE('',#145558,#10188) ;
#4635=LINE('',#145560,#10189) ;
#4636=LINE('',#145561,#10190) ;
#4637=LINE('',#145565,#10191) ;
#4638=LINE('',#145569,#10192) ;
#4639=LINE('',#145573,#10193) ;
#4640=LINE('',#145575,#10194) ;
#4641=LINE('',#145576,#10195) ;
#4642=LINE('',#145581,#10196) ;
#4643=LINE('',#145585,#10197) ;
#4644=LINE('',#145587,#10198) ;
#4645=LINE('',#145588,#10199) ;
#4646=LINE('',#145593,#10200) ;
#4647=LINE('',#145596,#10201) ;
#4648=LINE('',#145598,#10202) ;
#4649=LINE('',#145599,#10203) ;
#4650=LINE('',#145602,#10204) ;
#4651=LINE('',#145605,#10205) ;
#4652=LINE('',#145606,#10206) ;
#4653=LINE('',#145609,#10207) ;
#4654=LINE('',#145611,#10208) ;
#4655=LINE('',#145612,#10209) ;
#4656=LINE('',#145617,#10210) ;
#4657=LINE('',#145621,#10211) ;
#4658=LINE('',#145623,#10212) ;
#4659=LINE('',#145624,#10213) ;
#4660=LINE('',#145629,#10214) ;
#4661=LINE('',#145633,#10215) ;
#4662=LINE('',#145635,#10216) ;
#4663=LINE('',#145636,#10217) ;
#4664=LINE('',#145641,#10218) ;
#4665=LINE('',#145645,#10219) ;
#4666=LINE('',#145647,#10220) ;
#4667=LINE('',#145648,#10221) ;
#4668=LINE('',#145653,#10222) ;
#4669=LINE('',#145657,#10223) ;
#4670=LINE('',#145659,#10224) ;
#4671=LINE('',#145660,#10225) ;
#4672=LINE('',#145665,#10226) ;
#4673=LINE('',#145669,#10227) ;
#4674=LINE('',#145671,#10228) ;
#4675=LINE('',#145672,#10229) ;
#4676=LINE('',#145677,#10230) ;
#4677=LINE('',#145683,#10231) ;
#4678=LINE('',#145689,#10232) ;
#4679=LINE('',#145693,#10233) ;
#4680=LINE('',#145695,#10234) ;
#4681=LINE('',#145696,#10235) ;
#4682=LINE('',#145701,#10236) ;
#4683=LINE('',#145705,#10237) ;
#4684=LINE('',#145707,#10238) ;
#4685=LINE('',#145708,#10239) ;
#4686=LINE('',#145713,#10240) ;
#4687=LINE('',#145716,#10241) ;
#4688=LINE('',#145717,#10242) ;
#4689=LINE('',#145723,#10243) ;
#4690=LINE('',#145727,#10244) ;
#4691=LINE('',#145729,#10245) ;
#4692=LINE('',#145731,#10246) ;
#4693=LINE('',#145735,#10247) ;
#4694=LINE('',#145737,#10248) ;
#4695=LINE('',#145739,#10249) ;
#4696=LINE('',#145743,#10250) ;
#4697=LINE('',#145747,#10251) ;
#4698=LINE('',#145749,#10252) ;
#4699=LINE('',#145750,#10253) ;
#4700=LINE('',#145752,#10254) ;
#4701=LINE('',#145753,#10255) ;
#4702=LINE('',#145757,#10256) ;
#4703=LINE('',#145761,#10257) ;
#4704=LINE('',#145765,#10258) ;
#4705=LINE('',#145767,#10259) ;
#4706=LINE('',#145768,#10260) ;
#4707=LINE('',#145773,#10261) ;
#4708=LINE('',#145777,#10262) ;
#4709=LINE('',#145779,#10263) ;
#4710=LINE('',#145780,#10264) ;
#4711=LINE('',#145785,#10265) ;
#4712=LINE('',#145788,#10266) ;
#4713=LINE('',#145790,#10267) ;
#4714=LINE('',#145791,#10268) ;
#4715=LINE('',#145794,#10269) ;
#4716=LINE('',#145797,#10270) ;
#4717=LINE('',#145798,#10271) ;
#4718=LINE('',#145801,#10272) ;
#4719=LINE('',#145803,#10273) ;
#4720=LINE('',#145804,#10274) ;
#4721=LINE('',#145809,#10275) ;
#4722=LINE('',#145813,#10276) ;
#4723=LINE('',#145815,#10277) ;
#4724=LINE('',#145816,#10278) ;
#4725=LINE('',#145821,#10279) ;
#4726=LINE('',#145825,#10280) ;
#4727=LINE('',#145827,#10281) ;
#4728=LINE('',#145828,#10282) ;
#4729=LINE('',#145833,#10283) ;
#4730=LINE('',#145837,#10284) ;
#4731=LINE('',#145839,#10285) ;
#4732=LINE('',#145840,#10286) ;
#4733=LINE('',#145845,#10287) ;
#4734=LINE('',#145849,#10288) ;
#4735=LINE('',#145851,#10289) ;
#4736=LINE('',#145852,#10290) ;
#4737=LINE('',#145857,#10291) ;
#4738=LINE('',#145861,#10292) ;
#4739=LINE('',#145863,#10293) ;
#4740=LINE('',#145864,#10294) ;
#4741=LINE('',#145869,#10295) ;
#4742=LINE('',#145875,#10296) ;
#4743=LINE('',#145881,#10297) ;
#4744=LINE('',#145885,#10298) ;
#4745=LINE('',#145887,#10299) ;
#4746=LINE('',#145888,#10300) ;
#4747=LINE('',#145893,#10301) ;
#4748=LINE('',#145897,#10302) ;
#4749=LINE('',#145899,#10303) ;
#4750=LINE('',#145900,#10304) ;
#4751=LINE('',#145905,#10305) ;
#4752=LINE('',#145908,#10306) ;
#4753=LINE('',#145909,#10307) ;
#4754=LINE('',#145915,#10308) ;
#4755=LINE('',#145919,#10309) ;
#4756=LINE('',#145921,#10310) ;
#4757=LINE('',#145923,#10311) ;
#4758=LINE('',#145927,#10312) ;
#4759=LINE('',#145929,#10313) ;
#4760=LINE('',#145931,#10314) ;
#4761=LINE('',#145935,#10315) ;
#4762=LINE('',#145939,#10316) ;
#4763=LINE('',#145941,#10317) ;
#4764=LINE('',#145942,#10318) ;
#4765=LINE('',#145944,#10319) ;
#4766=LINE('',#145945,#10320) ;
#4767=LINE('',#145949,#10321) ;
#4768=LINE('',#145953,#10322) ;
#4769=LINE('',#145957,#10323) ;
#4770=LINE('',#145959,#10324) ;
#4771=LINE('',#145960,#10325) ;
#4772=LINE('',#145965,#10326) ;
#4773=LINE('',#145969,#10327) ;
#4774=LINE('',#145971,#10328) ;
#4775=LINE('',#145972,#10329) ;
#4776=LINE('',#145977,#10330) ;
#4777=LINE('',#145980,#10331) ;
#4778=LINE('',#145982,#10332) ;
#4779=LINE('',#145983,#10333) ;
#4780=LINE('',#145986,#10334) ;
#4781=LINE('',#145989,#10335) ;
#4782=LINE('',#145990,#10336) ;
#4783=LINE('',#145993,#10337) ;
#4784=LINE('',#145995,#10338) ;
#4785=LINE('',#145996,#10339) ;
#4786=LINE('',#146001,#10340) ;
#4787=LINE('',#146005,#10341) ;
#4788=LINE('',#146007,#10342) ;
#4789=LINE('',#146008,#10343) ;
#4790=LINE('',#146013,#10344) ;
#4791=LINE('',#146017,#10345) ;
#4792=LINE('',#146019,#10346) ;
#4793=LINE('',#146020,#10347) ;
#4794=LINE('',#146025,#10348) ;
#4795=LINE('',#146029,#10349) ;
#4796=LINE('',#146031,#10350) ;
#4797=LINE('',#146032,#10351) ;
#4798=LINE('',#146037,#10352) ;
#4799=LINE('',#146041,#10353) ;
#4800=LINE('',#146043,#10354) ;
#4801=LINE('',#146044,#10355) ;
#4802=LINE('',#146049,#10356) ;
#4803=LINE('',#146053,#10357) ;
#4804=LINE('',#146055,#10358) ;
#4805=LINE('',#146056,#10359) ;
#4806=LINE('',#146061,#10360) ;
#4807=LINE('',#146067,#10361) ;
#4808=LINE('',#146073,#10362) ;
#4809=LINE('',#146077,#10363) ;
#4810=LINE('',#146079,#10364) ;
#4811=LINE('',#146080,#10365) ;
#4812=LINE('',#146085,#10366) ;
#4813=LINE('',#146089,#10367) ;
#4814=LINE('',#146091,#10368) ;
#4815=LINE('',#146092,#10369) ;
#4816=LINE('',#146097,#10370) ;
#4817=LINE('',#146100,#10371) ;
#4818=LINE('',#146101,#10372) ;
#4819=LINE('',#146107,#10373) ;
#4820=LINE('',#146111,#10374) ;
#4821=LINE('',#146113,#10375) ;
#4822=LINE('',#146115,#10376) ;
#4823=LINE('',#146119,#10377) ;
#4824=LINE('',#146121,#10378) ;
#4825=LINE('',#146123,#10379) ;
#4826=LINE('',#146127,#10380) ;
#4827=LINE('',#146131,#10381) ;
#4828=LINE('',#146133,#10382) ;
#4829=LINE('',#146134,#10383) ;
#4830=LINE('',#146136,#10384) ;
#4831=LINE('',#146137,#10385) ;
#4832=LINE('',#146141,#10386) ;
#4833=LINE('',#146145,#10387) ;
#4834=LINE('',#146149,#10388) ;
#4835=LINE('',#146151,#10389) ;
#4836=LINE('',#146152,#10390) ;
#4837=LINE('',#146157,#10391) ;
#4838=LINE('',#146161,#10392) ;
#4839=LINE('',#146163,#10393) ;
#4840=LINE('',#146164,#10394) ;
#4841=LINE('',#146169,#10395) ;
#4842=LINE('',#146172,#10396) ;
#4843=LINE('',#146174,#10397) ;
#4844=LINE('',#146175,#10398) ;
#4845=LINE('',#146178,#10399) ;
#4846=LINE('',#146181,#10400) ;
#4847=LINE('',#146182,#10401) ;
#4848=LINE('',#146185,#10402) ;
#4849=LINE('',#146187,#10403) ;
#4850=LINE('',#146188,#10404) ;
#4851=LINE('',#146193,#10405) ;
#4852=LINE('',#146197,#10406) ;
#4853=LINE('',#146199,#10407) ;
#4854=LINE('',#146200,#10408) ;
#4855=LINE('',#146205,#10409) ;
#4856=LINE('',#146209,#10410) ;
#4857=LINE('',#146211,#10411) ;
#4858=LINE('',#146212,#10412) ;
#4859=LINE('',#146217,#10413) ;
#4860=LINE('',#146221,#10414) ;
#4861=LINE('',#146223,#10415) ;
#4862=LINE('',#146224,#10416) ;
#4863=LINE('',#146229,#10417) ;
#4864=LINE('',#146233,#10418) ;
#4865=LINE('',#146235,#10419) ;
#4866=LINE('',#146236,#10420) ;
#4867=LINE('',#146241,#10421) ;
#4868=LINE('',#146245,#10422) ;
#4869=LINE('',#146247,#10423) ;
#4870=LINE('',#146248,#10424) ;
#4871=LINE('',#146253,#10425) ;
#4872=LINE('',#146259,#10426) ;
#4873=LINE('',#146265,#10427) ;
#4874=LINE('',#146269,#10428) ;
#4875=LINE('',#146271,#10429) ;
#4876=LINE('',#146272,#10430) ;
#4877=LINE('',#146277,#10431) ;
#4878=LINE('',#146281,#10432) ;
#4879=LINE('',#146283,#10433) ;
#4880=LINE('',#146284,#10434) ;
#4881=LINE('',#146289,#10435) ;
#4882=LINE('',#146292,#10436) ;
#4883=LINE('',#146293,#10437) ;
#4884=LINE('',#146299,#10438) ;
#4885=LINE('',#146303,#10439) ;
#4886=LINE('',#146305,#10440) ;
#4887=LINE('',#146307,#10441) ;
#4888=LINE('',#146311,#10442) ;
#4889=LINE('',#146313,#10443) ;
#4890=LINE('',#146315,#10444) ;
#4891=LINE('',#146319,#10445) ;
#4892=LINE('',#146323,#10446) ;
#4893=LINE('',#146325,#10447) ;
#4894=LINE('',#146326,#10448) ;
#4895=LINE('',#146328,#10449) ;
#4896=LINE('',#146329,#10450) ;
#4897=LINE('',#146333,#10451) ;
#4898=LINE('',#146337,#10452) ;
#4899=LINE('',#146341,#10453) ;
#4900=LINE('',#146343,#10454) ;
#4901=LINE('',#146344,#10455) ;
#4902=LINE('',#146349,#10456) ;
#4903=LINE('',#146353,#10457) ;
#4904=LINE('',#146355,#10458) ;
#4905=LINE('',#146356,#10459) ;
#4906=LINE('',#146361,#10460) ;
#4907=LINE('',#146364,#10461) ;
#4908=LINE('',#146366,#10462) ;
#4909=LINE('',#146367,#10463) ;
#4910=LINE('',#146370,#10464) ;
#4911=LINE('',#146373,#10465) ;
#4912=LINE('',#146374,#10466) ;
#4913=LINE('',#146377,#10467) ;
#4914=LINE('',#146379,#10468) ;
#4915=LINE('',#146380,#10469) ;
#4916=LINE('',#146385,#10470) ;
#4917=LINE('',#146389,#10471) ;
#4918=LINE('',#146391,#10472) ;
#4919=LINE('',#146392,#10473) ;
#4920=LINE('',#146397,#10474) ;
#4921=LINE('',#146401,#10475) ;
#4922=LINE('',#146403,#10476) ;
#4923=LINE('',#146404,#10477) ;
#4924=LINE('',#146409,#10478) ;
#4925=LINE('',#146413,#10479) ;
#4926=LINE('',#146415,#10480) ;
#4927=LINE('',#146416,#10481) ;
#4928=LINE('',#146421,#10482) ;
#4929=LINE('',#146425,#10483) ;
#4930=LINE('',#146427,#10484) ;
#4931=LINE('',#146428,#10485) ;
#4932=LINE('',#146433,#10486) ;
#4933=LINE('',#146437,#10487) ;
#4934=LINE('',#146439,#10488) ;
#4935=LINE('',#146440,#10489) ;
#4936=LINE('',#146445,#10490) ;
#4937=LINE('',#146451,#10491) ;
#4938=LINE('',#146457,#10492) ;
#4939=LINE('',#146461,#10493) ;
#4940=LINE('',#146463,#10494) ;
#4941=LINE('',#146464,#10495) ;
#4942=LINE('',#146469,#10496) ;
#4943=LINE('',#146473,#10497) ;
#4944=LINE('',#146475,#10498) ;
#4945=LINE('',#146476,#10499) ;
#4946=LINE('',#146481,#10500) ;
#4947=LINE('',#146484,#10501) ;
#4948=LINE('',#146485,#10502) ;
#4949=LINE('',#146491,#10503) ;
#4950=LINE('',#146495,#10504) ;
#4951=LINE('',#146497,#10505) ;
#4952=LINE('',#146499,#10506) ;
#4953=LINE('',#146503,#10507) ;
#4954=LINE('',#146505,#10508) ;
#4955=LINE('',#146507,#10509) ;
#4956=LINE('',#146511,#10510) ;
#4957=LINE('',#146515,#10511) ;
#4958=LINE('',#146517,#10512) ;
#4959=LINE('',#146518,#10513) ;
#4960=LINE('',#146520,#10514) ;
#4961=LINE('',#146521,#10515) ;
#4962=LINE('',#146525,#10516) ;
#4963=LINE('',#146529,#10517) ;
#4964=LINE('',#146533,#10518) ;
#4965=LINE('',#146535,#10519) ;
#4966=LINE('',#146536,#10520) ;
#4967=LINE('',#146541,#10521) ;
#4968=LINE('',#146545,#10522) ;
#4969=LINE('',#146547,#10523) ;
#4970=LINE('',#146548,#10524) ;
#4971=LINE('',#146553,#10525) ;
#4972=LINE('',#146556,#10526) ;
#4973=LINE('',#146558,#10527) ;
#4974=LINE('',#146559,#10528) ;
#4975=LINE('',#146562,#10529) ;
#4976=LINE('',#146565,#10530) ;
#4977=LINE('',#146566,#10531) ;
#4978=LINE('',#146569,#10532) ;
#4979=LINE('',#146571,#10533) ;
#4980=LINE('',#146572,#10534) ;
#4981=LINE('',#146577,#10535) ;
#4982=LINE('',#146581,#10536) ;
#4983=LINE('',#146583,#10537) ;
#4984=LINE('',#146584,#10538) ;
#4985=LINE('',#146589,#10539) ;
#4986=LINE('',#146593,#10540) ;
#4987=LINE('',#146595,#10541) ;
#4988=LINE('',#146596,#10542) ;
#4989=LINE('',#146601,#10543) ;
#4990=LINE('',#146605,#10544) ;
#4991=LINE('',#146607,#10545) ;
#4992=LINE('',#146608,#10546) ;
#4993=LINE('',#146613,#10547) ;
#4994=LINE('',#146617,#10548) ;
#4995=LINE('',#146619,#10549) ;
#4996=LINE('',#146620,#10550) ;
#4997=LINE('',#146625,#10551) ;
#4998=LINE('',#146629,#10552) ;
#4999=LINE('',#146631,#10553) ;
#5000=LINE('',#146632,#10554) ;
#5001=LINE('',#146637,#10555) ;
#5002=LINE('',#146643,#10556) ;
#5003=LINE('',#146649,#10557) ;
#5004=LINE('',#146653,#10558) ;
#5005=LINE('',#146655,#10559) ;
#5006=LINE('',#146656,#10560) ;
#5007=LINE('',#146661,#10561) ;
#5008=LINE('',#146665,#10562) ;
#5009=LINE('',#146667,#10563) ;
#5010=LINE('',#146668,#10564) ;
#5011=LINE('',#146673,#10565) ;
#5012=LINE('',#146676,#10566) ;
#5013=LINE('',#146677,#10567) ;
#5014=LINE('',#146683,#10568) ;
#5015=LINE('',#146687,#10569) ;
#5016=LINE('',#146689,#10570) ;
#5017=LINE('',#146691,#10571) ;
#5018=LINE('',#146695,#10572) ;
#5019=LINE('',#146697,#10573) ;
#5020=LINE('',#146699,#10574) ;
#5021=LINE('',#146703,#10575) ;
#5022=LINE('',#146707,#10576) ;
#5023=LINE('',#146709,#10577) ;
#5024=LINE('',#146710,#10578) ;
#5025=LINE('',#146712,#10579) ;
#5026=LINE('',#146713,#10580) ;
#5027=LINE('',#146717,#10581) ;
#5028=LINE('',#146721,#10582) ;
#5029=LINE('',#146725,#10583) ;
#5030=LINE('',#146727,#10584) ;
#5031=LINE('',#146728,#10585) ;
#5032=LINE('',#146733,#10586) ;
#5033=LINE('',#146737,#10587) ;
#5034=LINE('',#146739,#10588) ;
#5035=LINE('',#146740,#10589) ;
#5036=LINE('',#146745,#10590) ;
#5037=LINE('',#146748,#10591) ;
#5038=LINE('',#146750,#10592) ;
#5039=LINE('',#146751,#10593) ;
#5040=LINE('',#146754,#10594) ;
#5041=LINE('',#146757,#10595) ;
#5042=LINE('',#146758,#10596) ;
#5043=LINE('',#146761,#10597) ;
#5044=LINE('',#146763,#10598) ;
#5045=LINE('',#146764,#10599) ;
#5046=LINE('',#146769,#10600) ;
#5047=LINE('',#146773,#10601) ;
#5048=LINE('',#146775,#10602) ;
#5049=LINE('',#146776,#10603) ;
#5050=LINE('',#146781,#10604) ;
#5051=LINE('',#146785,#10605) ;
#5052=LINE('',#146787,#10606) ;
#5053=LINE('',#146788,#10607) ;
#5054=LINE('',#146793,#10608) ;
#5055=LINE('',#146797,#10609) ;
#5056=LINE('',#146799,#10610) ;
#5057=LINE('',#146800,#10611) ;
#5058=LINE('',#146805,#10612) ;
#5059=LINE('',#146809,#10613) ;
#5060=LINE('',#146811,#10614) ;
#5061=LINE('',#146812,#10615) ;
#5062=LINE('',#146817,#10616) ;
#5063=LINE('',#146821,#10617) ;
#5064=LINE('',#146823,#10618) ;
#5065=LINE('',#146824,#10619) ;
#5066=LINE('',#146829,#10620) ;
#5067=LINE('',#146835,#10621) ;
#5068=LINE('',#146841,#10622) ;
#5069=LINE('',#146845,#10623) ;
#5070=LINE('',#146847,#10624) ;
#5071=LINE('',#146848,#10625) ;
#5072=LINE('',#146853,#10626) ;
#5073=LINE('',#146857,#10627) ;
#5074=LINE('',#146859,#10628) ;
#5075=LINE('',#146860,#10629) ;
#5076=LINE('',#146865,#10630) ;
#5077=LINE('',#146868,#10631) ;
#5078=LINE('',#146869,#10632) ;
#5079=LINE('',#146875,#10633) ;
#5080=LINE('',#146879,#10634) ;
#5081=LINE('',#146881,#10635) ;
#5082=LINE('',#146883,#10636) ;
#5083=LINE('',#146887,#10637) ;
#5084=LINE('',#146889,#10638) ;
#5085=LINE('',#146891,#10639) ;
#5086=LINE('',#146895,#10640) ;
#5087=LINE('',#146899,#10641) ;
#5088=LINE('',#146901,#10642) ;
#5089=LINE('',#146902,#10643) ;
#5090=LINE('',#146904,#10644) ;
#5091=LINE('',#146905,#10645) ;
#5092=LINE('',#146909,#10646) ;
#5093=LINE('',#146913,#10647) ;
#5094=LINE('',#146917,#10648) ;
#5095=LINE('',#146921,#10649) ;
#5096=LINE('',#146926,#10650) ;
#5097=LINE('',#146930,#10651) ;
#5098=LINE('',#146934,#10652) ;
#5099=LINE('',#146938,#10653) ;
#5100=LINE('',#146943,#10654) ;
#5101=LINE('',#146947,#10655) ;
#5102=LINE('',#146951,#10656) ;
#5103=LINE('',#146955,#10657) ;
#5104=LINE('',#146960,#10658) ;
#5105=LINE('',#146964,#10659) ;
#5106=LINE('',#146968,#10660) ;
#5107=LINE('',#146972,#10661) ;
#5108=LINE('',#146977,#10662) ;
#5109=LINE('',#146981,#10663) ;
#5110=LINE('',#146985,#10664) ;
#5111=LINE('',#146989,#10665) ;
#5112=LINE('',#146994,#10666) ;
#5113=LINE('',#146998,#10667) ;
#5114=LINE('',#147002,#10668) ;
#5115=LINE('',#147006,#10669) ;
#5116=LINE('',#147011,#10670) ;
#5117=LINE('',#147015,#10671) ;
#5118=LINE('',#147019,#10672) ;
#5119=LINE('',#147023,#10673) ;
#5120=LINE('',#147028,#10674) ;
#5121=LINE('',#147032,#10675) ;
#5122=LINE('',#147036,#10676) ;
#5123=LINE('',#147040,#10677) ;
#5124=LINE('',#147045,#10678) ;
#5125=LINE('',#147049,#10679) ;
#5126=LINE('',#147053,#10680) ;
#5127=LINE('',#147057,#10681) ;
#5128=LINE('',#147085,#10682) ;
#5129=LINE('',#147142,#10683) ;
#5130=LINE('',#147167,#10684) ;
#5131=LINE('',#147199,#10685) ;
#5132=LINE('',#147225,#10686) ;
#5133=LINE('',#147789,#10687) ;
#5134=LINE('',#147846,#10688) ;
#5135=LINE('',#147871,#10689) ;
#5136=LINE('',#147903,#10690) ;
#5137=LINE('',#147929,#10691) ;
#5138=LINE('',#148016,#10692) ;
#5139=LINE('',#148073,#10693) ;
#5140=LINE('',#148098,#10694) ;
#5141=LINE('',#148130,#10695) ;
#5142=LINE('',#148156,#10696) ;
#5143=LINE('',#148243,#10697) ;
#5144=LINE('',#148300,#10698) ;
#5145=LINE('',#148325,#10699) ;
#5146=LINE('',#148357,#10700) ;
#5147=LINE('',#148383,#10701) ;
#5148=LINE('',#148470,#10702) ;
#5149=LINE('',#148527,#10703) ;
#5150=LINE('',#148552,#10704) ;
#5151=LINE('',#148584,#10705) ;
#5152=LINE('',#148610,#10706) ;
#5153=LINE('',#148697,#10707) ;
#5154=LINE('',#148754,#10708) ;
#5155=LINE('',#148779,#10709) ;
#5156=LINE('',#148811,#10710) ;
#5157=LINE('',#148837,#10711) ;
#5158=LINE('',#148924,#10712) ;
#5159=LINE('',#148981,#10713) ;
#5160=LINE('',#149006,#10714) ;
#5161=LINE('',#149038,#10715) ;
#5162=LINE('',#149064,#10716) ;
#5163=LINE('',#149151,#10717) ;
#5164=LINE('',#149208,#10718) ;
#5165=LINE('',#149233,#10719) ;
#5166=LINE('',#149265,#10720) ;
#5167=LINE('',#149291,#10721) ;
#5168=LINE('',#149378,#10722) ;
#5169=LINE('',#149435,#10723) ;
#5170=LINE('',#149460,#10724) ;
#5171=LINE('',#149492,#10725) ;
#5172=LINE('',#149518,#10726) ;
#5173=LINE('',#149582,#10727) ;
#5174=LINE('',#149584,#10728) ;
#5175=LINE('',#149586,#10729) ;
#5176=LINE('',#149587,#10730) ;
#5177=LINE('',#149591,#10731) ;
#5178=LINE('',#149593,#10732) ;
#5179=LINE('',#149595,#10733) ;
#5180=LINE('',#149596,#10734) ;
#5181=LINE('',#149600,#10735) ;
#5182=LINE('',#149602,#10736) ;
#5183=LINE('',#149604,#10737) ;
#5184=LINE('',#149605,#10738) ;
#5185=LINE('',#149609,#10739) ;
#5186=LINE('',#149611,#10740) ;
#5187=LINE('',#149613,#10741) ;
#5188=LINE('',#149614,#10742) ;
#5189=LINE('',#149618,#10743) ;
#5190=LINE('',#149620,#10744) ;
#5191=LINE('',#149622,#10745) ;
#5192=LINE('',#149623,#10746) ;
#5193=LINE('',#149627,#10747) ;
#5194=LINE('',#149632,#10748) ;
#5195=LINE('',#149633,#10749) ;
#5196=LINE('',#149637,#10750) ;
#5197=LINE('',#149642,#10751) ;
#5198=LINE('',#149643,#10752) ;
#5199=LINE('',#149653,#10753) ;
#5200=LINE('',#149655,#10754) ;
#5201=LINE('',#149657,#10755) ;
#5202=LINE('',#149658,#10756) ;
#5203=LINE('',#149662,#10757) ;
#5204=LINE('',#149663,#10758) ;
#5205=LINE('',#149664,#10759) ;
#5206=LINE('',#149667,#10760) ;
#5207=LINE('',#149669,#10761) ;
#5208=LINE('',#149670,#10762) ;
#5209=LINE('',#149674,#10763) ;
#5210=LINE('',#149676,#10764) ;
#5211=LINE('',#149678,#10765) ;
#5212=LINE('',#149679,#10766) ;
#5213=LINE('',#149683,#10767) ;
#5214=LINE('',#149685,#10768) ;
#5215=LINE('',#149687,#10769) ;
#5216=LINE('',#149688,#10770) ;
#5217=LINE('',#149692,#10771) ;
#5218=LINE('',#149693,#10772) ;
#5219=LINE('',#149694,#10773) ;
#5220=LINE('',#149697,#10774) ;
#5221=LINE('',#149699,#10775) ;
#5222=LINE('',#149700,#10776) ;
#5223=LINE('',#149704,#10777) ;
#5224=LINE('',#149706,#10778) ;
#5225=LINE('',#149708,#10779) ;
#5226=LINE('',#149709,#10780) ;
#5227=LINE('',#149713,#10781) ;
#5228=LINE('',#149715,#10782) ;
#5229=LINE('',#149717,#10783) ;
#5230=LINE('',#149718,#10784) ;
#5231=LINE('',#149722,#10785) ;
#5232=LINE('',#149724,#10786) ;
#5233=LINE('',#149726,#10787) ;
#5234=LINE('',#149727,#10788) ;
#5235=LINE('',#149731,#10789) ;
#5236=LINE('',#149733,#10790) ;
#5237=LINE('',#149735,#10791) ;
#5238=LINE('',#149736,#10792) ;
#5239=LINE('',#149740,#10793) ;
#5240=LINE('',#149742,#10794) ;
#5241=LINE('',#149744,#10795) ;
#5242=LINE('',#149745,#10796) ;
#5243=LINE('',#149749,#10797) ;
#5244=LINE('',#149754,#10798) ;
#5245=LINE('',#149755,#10799) ;
#5246=LINE('',#149759,#10800) ;
#5247=LINE('',#149764,#10801) ;
#5248=LINE('',#149765,#10802) ;
#5249=LINE('',#149775,#10803) ;
#5250=LINE('',#149777,#10804) ;
#5251=LINE('',#149779,#10805) ;
#5252=LINE('',#149780,#10806) ;
#5253=LINE('',#149784,#10807) ;
#5254=LINE('',#149785,#10808) ;
#5255=LINE('',#149786,#10809) ;
#5256=LINE('',#149789,#10810) ;
#5257=LINE('',#149791,#10811) ;
#5258=LINE('',#149792,#10812) ;
#5259=LINE('',#149796,#10813) ;
#5260=LINE('',#149798,#10814) ;
#5261=LINE('',#149800,#10815) ;
#5262=LINE('',#149801,#10816) ;
#5263=LINE('',#149805,#10817) ;
#5264=LINE('',#149807,#10818) ;
#5265=LINE('',#149809,#10819) ;
#5266=LINE('',#149810,#10820) ;
#5267=LINE('',#149814,#10821) ;
#5268=LINE('',#149815,#10822) ;
#5269=LINE('',#149816,#10823) ;
#5270=LINE('',#149819,#10824) ;
#5271=LINE('',#149821,#10825) ;
#5272=LINE('',#149822,#10826) ;
#5273=LINE('',#149826,#10827) ;
#5274=LINE('',#149828,#10828) ;
#5275=LINE('',#149830,#10829) ;
#5276=LINE('',#149831,#10830) ;
#5277=LINE('',#149835,#10831) ;
#5278=LINE('',#149837,#10832) ;
#5279=LINE('',#149839,#10833) ;
#5280=LINE('',#149840,#10834) ;
#5281=LINE('',#149844,#10835) ;
#5282=LINE('',#149846,#10836) ;
#5283=LINE('',#149848,#10837) ;
#5284=LINE('',#149849,#10838) ;
#5285=LINE('',#149853,#10839) ;
#5286=LINE('',#149855,#10840) ;
#5287=LINE('',#149857,#10841) ;
#5288=LINE('',#149858,#10842) ;
#5289=LINE('',#149862,#10843) ;
#5290=LINE('',#149864,#10844) ;
#5291=LINE('',#149866,#10845) ;
#5292=LINE('',#149867,#10846) ;
#5293=LINE('',#149871,#10847) ;
#5294=LINE('',#149876,#10848) ;
#5295=LINE('',#149877,#10849) ;
#5296=LINE('',#149881,#10850) ;
#5297=LINE('',#149886,#10851) ;
#5298=LINE('',#149887,#10852) ;
#5299=LINE('',#149897,#10853) ;
#5300=LINE('',#149899,#10854) ;
#5301=LINE('',#149901,#10855) ;
#5302=LINE('',#149902,#10856) ;
#5303=LINE('',#149906,#10857) ;
#5304=LINE('',#149907,#10858) ;
#5305=LINE('',#149908,#10859) ;
#5306=LINE('',#149911,#10860) ;
#5307=LINE('',#149913,#10861) ;
#5308=LINE('',#149914,#10862) ;
#5309=LINE('',#149918,#10863) ;
#5310=LINE('',#149920,#10864) ;
#5311=LINE('',#149922,#10865) ;
#5312=LINE('',#149923,#10866) ;
#5313=LINE('',#149927,#10867) ;
#5314=LINE('',#149929,#10868) ;
#5315=LINE('',#149931,#10869) ;
#5316=LINE('',#149932,#10870) ;
#5317=LINE('',#149936,#10871) ;
#5318=LINE('',#149937,#10872) ;
#5319=LINE('',#149938,#10873) ;
#5320=LINE('',#149941,#10874) ;
#5321=LINE('',#149943,#10875) ;
#5322=LINE('',#149944,#10876) ;
#5323=LINE('',#149948,#10877) ;
#5324=LINE('',#149950,#10878) ;
#5325=LINE('',#149952,#10879) ;
#5326=LINE('',#149953,#10880) ;
#5327=LINE('',#149957,#10881) ;
#5328=LINE('',#149959,#10882) ;
#5329=LINE('',#149961,#10883) ;
#5330=LINE('',#149962,#10884) ;
#5331=LINE('',#149966,#10885) ;
#5332=LINE('',#149968,#10886) ;
#5333=LINE('',#149970,#10887) ;
#5334=LINE('',#149971,#10888) ;
#5335=LINE('',#149975,#10889) ;
#5336=LINE('',#149977,#10890) ;
#5337=LINE('',#149979,#10891) ;
#5338=LINE('',#149980,#10892) ;
#5339=LINE('',#149984,#10893) ;
#5340=LINE('',#149986,#10894) ;
#5341=LINE('',#149988,#10895) ;
#5342=LINE('',#149989,#10896) ;
#5343=LINE('',#149993,#10897) ;
#5344=LINE('',#149998,#10898) ;
#5345=LINE('',#149999,#10899) ;
#5346=LINE('',#150003,#10900) ;
#5347=LINE('',#150008,#10901) ;
#5348=LINE('',#150009,#10902) ;
#5349=LINE('',#150019,#10903) ;
#5350=LINE('',#150021,#10904) ;
#5351=LINE('',#150023,#10905) ;
#5352=LINE('',#150024,#10906) ;
#5353=LINE('',#150028,#10907) ;
#5354=LINE('',#150029,#10908) ;
#5355=LINE('',#150030,#10909) ;
#5356=LINE('',#150033,#10910) ;
#5357=LINE('',#150035,#10911) ;
#5358=LINE('',#150036,#10912) ;
#5359=LINE('',#150040,#10913) ;
#5360=LINE('',#150042,#10914) ;
#5361=LINE('',#150044,#10915) ;
#5362=LINE('',#150045,#10916) ;
#5363=LINE('',#150049,#10917) ;
#5364=LINE('',#150051,#10918) ;
#5365=LINE('',#150053,#10919) ;
#5366=LINE('',#150054,#10920) ;
#5367=LINE('',#150058,#10921) ;
#5368=LINE('',#150059,#10922) ;
#5369=LINE('',#150060,#10923) ;
#5370=LINE('',#150063,#10924) ;
#5371=LINE('',#150065,#10925) ;
#5372=LINE('',#150066,#10926) ;
#5373=LINE('',#150070,#10927) ;
#5374=LINE('',#150072,#10928) ;
#5375=LINE('',#150074,#10929) ;
#5376=LINE('',#150075,#10930) ;
#5377=LINE('',#150079,#10931) ;
#5378=LINE('',#150081,#10932) ;
#5379=LINE('',#150083,#10933) ;
#5380=LINE('',#150084,#10934) ;
#5381=LINE('',#150088,#10935) ;
#5382=LINE('',#150090,#10936) ;
#5383=LINE('',#150092,#10937) ;
#5384=LINE('',#150093,#10938) ;
#5385=LINE('',#150097,#10939) ;
#5386=LINE('',#150099,#10940) ;
#5387=LINE('',#150101,#10941) ;
#5388=LINE('',#150102,#10942) ;
#5389=LINE('',#150106,#10943) ;
#5390=LINE('',#150108,#10944) ;
#5391=LINE('',#150110,#10945) ;
#5392=LINE('',#150111,#10946) ;
#5393=LINE('',#150115,#10947) ;
#5394=LINE('',#150120,#10948) ;
#5395=LINE('',#150121,#10949) ;
#5396=LINE('',#150125,#10950) ;
#5397=LINE('',#150130,#10951) ;
#5398=LINE('',#150131,#10952) ;
#5399=LINE('',#150141,#10953) ;
#5400=LINE('',#150143,#10954) ;
#5401=LINE('',#150145,#10955) ;
#5402=LINE('',#150146,#10956) ;
#5403=LINE('',#150150,#10957) ;
#5404=LINE('',#150151,#10958) ;
#5405=LINE('',#150152,#10959) ;
#5406=LINE('',#150155,#10960) ;
#5407=LINE('',#150157,#10961) ;
#5408=LINE('',#150158,#10962) ;
#5409=LINE('',#150162,#10963) ;
#5410=LINE('',#150164,#10964) ;
#5411=LINE('',#150166,#10965) ;
#5412=LINE('',#150167,#10966) ;
#5413=LINE('',#150171,#10967) ;
#5414=LINE('',#150173,#10968) ;
#5415=LINE('',#150175,#10969) ;
#5416=LINE('',#150176,#10970) ;
#5417=LINE('',#150180,#10971) ;
#5418=LINE('',#150181,#10972) ;
#5419=LINE('',#150182,#10973) ;
#5420=LINE('',#150185,#10974) ;
#5421=LINE('',#150187,#10975) ;
#5422=LINE('',#150188,#10976) ;
#5423=LINE('',#150192,#10977) ;
#5424=LINE('',#150194,#10978) ;
#5425=LINE('',#150196,#10979) ;
#5426=LINE('',#150197,#10980) ;
#5427=LINE('',#150201,#10981) ;
#5428=LINE('',#150203,#10982) ;
#5429=LINE('',#150205,#10983) ;
#5430=LINE('',#150206,#10984) ;
#5431=LINE('',#150210,#10985) ;
#5432=LINE('',#150212,#10986) ;
#5433=LINE('',#150214,#10987) ;
#5434=LINE('',#150215,#10988) ;
#5435=LINE('',#150219,#10989) ;
#5436=LINE('',#150221,#10990) ;
#5437=LINE('',#150223,#10991) ;
#5438=LINE('',#150224,#10992) ;
#5439=LINE('',#150228,#10993) ;
#5440=LINE('',#150230,#10994) ;
#5441=LINE('',#150232,#10995) ;
#5442=LINE('',#150233,#10996) ;
#5443=LINE('',#150237,#10997) ;
#5444=LINE('',#150242,#10998) ;
#5445=LINE('',#150243,#10999) ;
#5446=LINE('',#150247,#11000) ;
#5447=LINE('',#150252,#11001) ;
#5448=LINE('',#150253,#11002) ;
#5449=LINE('',#150263,#11003) ;
#5450=LINE('',#150265,#11004) ;
#5451=LINE('',#150267,#11005) ;
#5452=LINE('',#150268,#11006) ;
#5453=LINE('',#150272,#11007) ;
#5454=LINE('',#150273,#11008) ;
#5455=LINE('',#150274,#11009) ;
#5456=LINE('',#150277,#11010) ;
#5457=LINE('',#150279,#11011) ;
#5458=LINE('',#150280,#11012) ;
#5459=LINE('',#150284,#11013) ;
#5460=LINE('',#150286,#11014) ;
#5461=LINE('',#150288,#11015) ;
#5462=LINE('',#150289,#11016) ;
#5463=LINE('',#150293,#11017) ;
#5464=LINE('',#150295,#11018) ;
#5465=LINE('',#150297,#11019) ;
#5466=LINE('',#150298,#11020) ;
#5467=LINE('',#150302,#11021) ;
#5468=LINE('',#150303,#11022) ;
#5469=LINE('',#150304,#11023) ;
#5470=LINE('',#150307,#11024) ;
#5471=LINE('',#150309,#11025) ;
#5472=LINE('',#150310,#11026) ;
#5473=LINE('',#150314,#11027) ;
#5474=LINE('',#150316,#11028) ;
#5475=LINE('',#150318,#11029) ;
#5476=LINE('',#150319,#11030) ;
#5477=LINE('',#150323,#11031) ;
#5478=LINE('',#150325,#11032) ;
#5479=LINE('',#150327,#11033) ;
#5480=LINE('',#150328,#11034) ;
#5481=LINE('',#150332,#11035) ;
#5482=LINE('',#150334,#11036) ;
#5483=LINE('',#150336,#11037) ;
#5484=LINE('',#150337,#11038) ;
#5485=LINE('',#150341,#11039) ;
#5486=LINE('',#150343,#11040) ;
#5487=LINE('',#150345,#11041) ;
#5488=LINE('',#150346,#11042) ;
#5489=LINE('',#150350,#11043) ;
#5490=LINE('',#150352,#11044) ;
#5491=LINE('',#150354,#11045) ;
#5492=LINE('',#150355,#11046) ;
#5493=LINE('',#150359,#11047) ;
#5494=LINE('',#150364,#11048) ;
#5495=LINE('',#150365,#11049) ;
#5496=LINE('',#150369,#11050) ;
#5497=LINE('',#150374,#11051) ;
#5498=LINE('',#150375,#11052) ;
#5499=LINE('',#150385,#11053) ;
#5500=LINE('',#150387,#11054) ;
#5501=LINE('',#150389,#11055) ;
#5502=LINE('',#150390,#11056) ;
#5503=LINE('',#150394,#11057) ;
#5504=LINE('',#150395,#11058) ;
#5505=LINE('',#150396,#11059) ;
#5506=LINE('',#150399,#11060) ;
#5507=LINE('',#150401,#11061) ;
#5508=LINE('',#150402,#11062) ;
#5509=LINE('',#150406,#11063) ;
#5510=LINE('',#150408,#11064) ;
#5511=LINE('',#150410,#11065) ;
#5512=LINE('',#150411,#11066) ;
#5513=LINE('',#150415,#11067) ;
#5514=LINE('',#150417,#11068) ;
#5515=LINE('',#150419,#11069) ;
#5516=LINE('',#150420,#11070) ;
#5517=LINE('',#150424,#11071) ;
#5518=LINE('',#150425,#11072) ;
#5519=LINE('',#150426,#11073) ;
#5520=LINE('',#150429,#11074) ;
#5521=LINE('',#150431,#11075) ;
#5522=LINE('',#150432,#11076) ;
#5523=LINE('',#150436,#11077) ;
#5524=LINE('',#150438,#11078) ;
#5525=LINE('',#150440,#11079) ;
#5526=LINE('',#150441,#11080) ;
#5527=LINE('',#150445,#11081) ;
#5528=LINE('',#150447,#11082) ;
#5529=LINE('',#150449,#11083) ;
#5530=LINE('',#150450,#11084) ;
#5531=LINE('',#150454,#11085) ;
#5532=LINE('',#150456,#11086) ;
#5533=LINE('',#150458,#11087) ;
#5534=LINE('',#150459,#11088) ;
#5535=LINE('',#150463,#11089) ;
#5536=LINE('',#150465,#11090) ;
#5537=LINE('',#150467,#11091) ;
#5538=LINE('',#150468,#11092) ;
#5539=LINE('',#150472,#11093) ;
#5540=LINE('',#150474,#11094) ;
#5541=LINE('',#150476,#11095) ;
#5542=LINE('',#150477,#11096) ;
#5543=LINE('',#150481,#11097) ;
#5544=LINE('',#150486,#11098) ;
#5545=LINE('',#150487,#11099) ;
#5546=LINE('',#150491,#11100) ;
#5547=LINE('',#150496,#11101) ;
#5548=LINE('',#150497,#11102) ;
#5549=LINE('',#150507,#11103) ;
#5550=LINE('',#150509,#11104) ;
#5551=LINE('',#150511,#11105) ;
#5552=LINE('',#150512,#11106) ;
#5553=LINE('',#150516,#11107) ;
#5554=LINE('',#150517,#11108) ;
#5555=LINE('',#150518,#11109) ;
#5556=LINE('',#150521,#11110) ;
#5557=LINE('',#150523,#11111) ;
#5558=LINE('',#150524,#11112) ;
#5559=LINE('',#150528,#11113) ;
#5560=LINE('',#150530,#11114) ;
#5561=LINE('',#150532,#11115) ;
#5562=LINE('',#150533,#11116) ;
#5563=LINE('',#150537,#11117) ;
#5564=LINE('',#150539,#11118) ;
#5565=LINE('',#150541,#11119) ;
#5566=LINE('',#150542,#11120) ;
#5567=LINE('',#150546,#11121) ;
#5568=LINE('',#150547,#11122) ;
#5569=LINE('',#150548,#11123) ;
#5570=LINE('',#150551,#11124) ;
#5571=LINE('',#150553,#11125) ;
#5572=LINE('',#150554,#11126) ;
#5573=LINE('',#150558,#11127) ;
#5574=LINE('',#150560,#11128) ;
#5575=LINE('',#150562,#11129) ;
#5576=LINE('',#150563,#11130) ;
#5577=LINE('',#150567,#11131) ;
#5578=LINE('',#150569,#11132) ;
#5579=LINE('',#150571,#11133) ;
#5580=LINE('',#150572,#11134) ;
#5581=LINE('',#150576,#11135) ;
#5582=LINE('',#150578,#11136) ;
#5583=LINE('',#150580,#11137) ;
#5584=LINE('',#150581,#11138) ;
#5585=LINE('',#150585,#11139) ;
#5586=LINE('',#150587,#11140) ;
#5587=LINE('',#150589,#11141) ;
#5588=LINE('',#150590,#11142) ;
#5589=LINE('',#150594,#11143) ;
#5590=LINE('',#150596,#11144) ;
#5591=LINE('',#150598,#11145) ;
#5592=LINE('',#150599,#11146) ;
#5593=LINE('',#150603,#11147) ;
#5594=LINE('',#150608,#11148) ;
#5595=LINE('',#150609,#11149) ;
#5596=LINE('',#150613,#11150) ;
#5597=LINE('',#150618,#11151) ;
#5598=LINE('',#150619,#11152) ;
#5599=LINE('',#150629,#11153) ;
#5600=LINE('',#150631,#11154) ;
#5601=LINE('',#150633,#11155) ;
#5602=LINE('',#150634,#11156) ;
#5603=LINE('',#150638,#11157) ;
#5604=LINE('',#150639,#11158) ;
#5605=LINE('',#150640,#11159) ;
#5606=LINE('',#150643,#11160) ;
#5607=LINE('',#150645,#11161) ;
#5608=LINE('',#150646,#11162) ;
#5609=LINE('',#150650,#11163) ;
#5610=LINE('',#150652,#11164) ;
#5611=LINE('',#150654,#11165) ;
#5612=LINE('',#150655,#11166) ;
#5613=LINE('',#150659,#11167) ;
#5614=LINE('',#150661,#11168) ;
#5615=LINE('',#150663,#11169) ;
#5616=LINE('',#150664,#11170) ;
#5617=LINE('',#150668,#11171) ;
#5618=LINE('',#150669,#11172) ;
#5619=LINE('',#150670,#11173) ;
#5620=LINE('',#150673,#11174) ;
#5621=LINE('',#150675,#11175) ;
#5622=LINE('',#150676,#11176) ;
#5623=LINE('',#150680,#11177) ;
#5624=LINE('',#150682,#11178) ;
#5625=LINE('',#150684,#11179) ;
#5626=LINE('',#150685,#11180) ;
#5627=LINE('',#150689,#11181) ;
#5628=LINE('',#150691,#11182) ;
#5629=LINE('',#150693,#11183) ;
#5630=LINE('',#150694,#11184) ;
#5631=LINE('',#150698,#11185) ;
#5632=LINE('',#150700,#11186) ;
#5633=LINE('',#150702,#11187) ;
#5634=LINE('',#150703,#11188) ;
#5635=LINE('',#150707,#11189) ;
#5636=LINE('',#150709,#11190) ;
#5637=LINE('',#150711,#11191) ;
#5638=LINE('',#150712,#11192) ;
#5639=LINE('',#150716,#11193) ;
#5640=LINE('',#150718,#11194) ;
#5641=LINE('',#150720,#11195) ;
#5642=LINE('',#150721,#11196) ;
#5643=LINE('',#150725,#11197) ;
#5644=LINE('',#150727,#11198) ;
#5645=LINE('',#150729,#11199) ;
#5646=LINE('',#150730,#11200) ;
#5647=LINE('',#150734,#11201) ;
#5648=LINE('',#150736,#11202) ;
#5649=LINE('',#150738,#11203) ;
#5650=LINE('',#150739,#11204) ;
#5651=LINE('',#150743,#11205) ;
#5652=LINE('',#150745,#11206) ;
#5653=LINE('',#150747,#11207) ;
#5654=LINE('',#150748,#11208) ;
#5655=LINE('',#150752,#11209) ;
#5656=LINE('',#150754,#11210) ;
#5657=LINE('',#150756,#11211) ;
#5658=LINE('',#150757,#11212) ;
#5659=LINE('',#150761,#11213) ;
#5660=LINE('',#150763,#11214) ;
#5661=LINE('',#150765,#11215) ;
#5662=LINE('',#150766,#11216) ;
#5663=LINE('',#150770,#11217) ;
#5664=LINE('',#150772,#11218) ;
#5665=LINE('',#150774,#11219) ;
#5666=LINE('',#150775,#11220) ;
#5667=LINE('',#150779,#11221) ;
#5668=LINE('',#150781,#11222) ;
#5669=LINE('',#150783,#11223) ;
#5670=LINE('',#150784,#11224) ;
#5671=LINE('',#150788,#11225) ;
#5672=LINE('',#150790,#11226) ;
#5673=LINE('',#150792,#11227) ;
#5674=LINE('',#150793,#11228) ;
#5675=LINE('',#150797,#11229) ;
#5676=LINE('',#150799,#11230) ;
#5677=LINE('',#150801,#11231) ;
#5678=LINE('',#150802,#11232) ;
#5679=LINE('',#150806,#11233) ;
#5680=LINE('',#150808,#11234) ;
#5681=LINE('',#150810,#11235) ;
#5682=LINE('',#150811,#11236) ;
#5683=LINE('',#150815,#11237) ;
#5684=LINE('',#150817,#11238) ;
#5685=LINE('',#150819,#11239) ;
#5686=LINE('',#150820,#11240) ;
#5687=LINE('',#150824,#11241) ;
#5688=LINE('',#150826,#11242) ;
#5689=LINE('',#150828,#11243) ;
#5690=LINE('',#150829,#11244) ;
#5691=LINE('',#150833,#11245) ;
#5692=LINE('',#150835,#11246) ;
#5693=LINE('',#150837,#11247) ;
#5694=LINE('',#150838,#11248) ;
#5695=LINE('',#150842,#11249) ;
#5696=LINE('',#150844,#11250) ;
#5697=LINE('',#150846,#11251) ;
#5698=LINE('',#150847,#11252) ;
#5699=LINE('',#150851,#11253) ;
#5700=LINE('',#150853,#11254) ;
#5701=LINE('',#150855,#11255) ;
#5702=LINE('',#150856,#11256) ;
#5703=LINE('',#150860,#11257) ;
#5704=LINE('',#150862,#11258) ;
#5705=LINE('',#150864,#11259) ;
#5706=LINE('',#150865,#11260) ;
#5707=LINE('',#150869,#11261) ;
#5708=LINE('',#150871,#11262) ;
#5709=LINE('',#150873,#11263) ;
#5710=LINE('',#150874,#11264) ;
#5711=LINE('',#150878,#11265) ;
#5712=LINE('',#150880,#11266) ;
#5713=LINE('',#150882,#11267) ;
#5714=LINE('',#150883,#11268) ;
#5715=LINE('',#150887,#11269) ;
#5716=LINE('',#150889,#11270) ;
#5717=LINE('',#150891,#11271) ;
#5718=LINE('',#150892,#11272) ;
#5719=LINE('',#150896,#11273) ;
#5720=LINE('',#150898,#11274) ;
#5721=LINE('',#150900,#11275) ;
#5722=LINE('',#150901,#11276) ;
#5723=LINE('',#150905,#11277) ;
#5724=LINE('',#150907,#11278) ;
#5725=LINE('',#150909,#11279) ;
#5726=LINE('',#150910,#11280) ;
#5727=LINE('',#150914,#11281) ;
#5728=LINE('',#150916,#11282) ;
#5729=LINE('',#150918,#11283) ;
#5730=LINE('',#150919,#11284) ;
#5731=LINE('',#150923,#11285) ;
#5732=LINE('',#150925,#11286) ;
#5733=LINE('',#150927,#11287) ;
#5734=LINE('',#150928,#11288) ;
#5735=LINE('',#150932,#11289) ;
#5736=LINE('',#150934,#11290) ;
#5737=LINE('',#150936,#11291) ;
#5738=LINE('',#150937,#11292) ;
#5739=LINE('',#150941,#11293) ;
#5740=LINE('',#150943,#11294) ;
#5741=LINE('',#150945,#11295) ;
#5742=LINE('',#150946,#11296) ;
#5743=LINE('',#150950,#11297) ;
#5744=LINE('',#150952,#11298) ;
#5745=LINE('',#150954,#11299) ;
#5746=LINE('',#150955,#11300) ;
#5747=LINE('',#150959,#11301) ;
#5748=LINE('',#150961,#11302) ;
#5749=LINE('',#150963,#11303) ;
#5750=LINE('',#150964,#11304) ;
#5751=LINE('',#150968,#11305) ;
#5752=LINE('',#150970,#11306) ;
#5753=LINE('',#150972,#11307) ;
#5754=LINE('',#150973,#11308) ;
#5755=LINE('',#150977,#11309) ;
#5756=LINE('',#150979,#11310) ;
#5757=LINE('',#150981,#11311) ;
#5758=LINE('',#150982,#11312) ;
#5759=LINE('',#150986,#11313) ;
#5760=LINE('',#150988,#11314) ;
#5761=LINE('',#150990,#11315) ;
#5762=LINE('',#150991,#11316) ;
#5763=LINE('',#150995,#11317) ;
#5764=LINE('',#150997,#11318) ;
#5765=LINE('',#150999,#11319) ;
#5766=LINE('',#151000,#11320) ;
#9183=VECTOR('',#108765,1000.) ;
#9184=VECTOR('',#108768,1000.) ;
#9185=VECTOR('',#108769,1000.) ;
#9186=VECTOR('',#108802,1000.) ;
#9187=VECTOR('',#108805,1000.) ;
#9188=VECTOR('',#108806,1000.) ;
#9189=VECTOR('',#108839,1000.) ;
#9190=VECTOR('',#108842,1000.) ;
#9191=VECTOR('',#108843,1000.) ;
#9192=VECTOR('',#108876,1000.) ;
#9193=VECTOR('',#108879,1000.) ;
#9194=VECTOR('',#108880,1000.) ;
#9195=VECTOR('',#108913,1000.) ;
#9196=VECTOR('',#108916,1000.) ;
#9197=VECTOR('',#108917,1000.) ;
#9198=VECTOR('',#108950,1000.) ;
#9199=VECTOR('',#108953,1000.) ;
#9200=VECTOR('',#108954,1000.) ;
#9201=VECTOR('',#108987,1000.) ;
#9202=VECTOR('',#108990,1000.) ;
#9203=VECTOR('',#108991,1000.) ;
#9204=VECTOR('',#109024,1000.) ;
#9205=VECTOR('',#109027,1000.) ;
#9206=VECTOR('',#109028,1000.) ;
#9207=VECTOR('',#109151,1000.) ;
#9208=VECTOR('',#109154,1000.) ;
#9209=VECTOR('',#109155,1000.) ;
#9210=VECTOR('',#109158,1.) ;
#9211=VECTOR('',#109161,1.) ;
#9212=VECTOR('',#109164,1.) ;
#9213=VECTOR('',#109167,1.) ;
#9214=VECTOR('',#109170,1.) ;
#9215=VECTOR('',#109173,0.999999999999999) ;
#9216=VECTOR('',#109176,0.999999999999999) ;
#9217=VECTOR('',#109179,1.) ;
#9218=VECTOR('',#109182,1.) ;
#9219=VECTOR('',#109187,1000.) ;
#9220=VECTOR('',#109188,1000.) ;
#9221=VECTOR('',#109193,1000.) ;
#9222=VECTOR('',#109194,1000.) ;
#9223=VECTOR('',#109199,1000.) ;
#9224=VECTOR('',#109200,1000.) ;
#9225=VECTOR('',#109205,1000.) ;
#9226=VECTOR('',#109206,1000.) ;
#9227=VECTOR('',#109211,1000.) ;
#9228=VECTOR('',#109212,1000.) ;
#9229=VECTOR('',#109217,1000.) ;
#9230=VECTOR('',#109218,1000.) ;
#9231=VECTOR('',#109223,1000.) ;
#9232=VECTOR('',#109224,1000.) ;
#9233=VECTOR('',#109229,1000.) ;
#9234=VECTOR('',#109230,1000.) ;
#9235=VECTOR('',#109235,1000.) ;
#9236=VECTOR('',#109236,1000.) ;
#9237=VECTOR('',#109279,1000.) ;
#9238=VECTOR('',#109282,1000.) ;
#9239=VECTOR('',#109283,1000.) ;
#9240=VECTOR('',#109286,1.) ;
#9241=VECTOR('',#109291,1000.) ;
#9242=VECTOR('',#109292,1000.) ;
#9243=VECTOR('',#109295,1000.) ;
#9244=VECTOR('',#109298,1000.) ;
#9245=VECTOR('',#109303,1000.) ;
#9246=VECTOR('',#109304,1000.) ;
#9247=VECTOR('',#109305,1000.) ;
#9248=VECTOR('',#109306,1000.) ;
#9249=VECTOR('',#109307,1000.) ;
#9250=VECTOR('',#109312,1000.) ;
#9251=VECTOR('',#109315,1000.) ;
#9252=VECTOR('',#109320,1000.) ;
#9253=VECTOR('',#109321,1000.) ;
#9254=VECTOR('',#109322,1000.) ;
#9255=VECTOR('',#109323,1000.) ;
#9256=VECTOR('',#109324,1000.) ;
#9257=VECTOR('',#109329,1000.) ;
#9258=VECTOR('',#109332,1000.) ;
#9259=VECTOR('',#109337,1000.) ;
#9260=VECTOR('',#109338,1000.) ;
#9261=VECTOR('',#109339,1000.) ;
#9262=VECTOR('',#109340,1000.) ;
#9263=VECTOR('',#109341,1000.) ;
#9264=VECTOR('',#109346,1000.) ;
#9265=VECTOR('',#109349,1000.) ;
#9266=VECTOR('',#109354,1000.) ;
#9267=VECTOR('',#109355,1000.) ;
#9268=VECTOR('',#109356,1000.) ;
#9269=VECTOR('',#109357,1000.) ;
#9270=VECTOR('',#109358,1000.) ;
#9271=VECTOR('',#109363,1000.) ;
#9272=VECTOR('',#109366,1000.) ;
#9273=VECTOR('',#109371,1000.) ;
#9274=VECTOR('',#109372,1000.) ;
#9275=VECTOR('',#109373,1000.) ;
#9276=VECTOR('',#109374,1000.) ;
#9277=VECTOR('',#109375,1000.) ;
#9278=VECTOR('',#109380,1000.) ;
#9279=VECTOR('',#109383,1000.) ;
#9280=VECTOR('',#109388,1000.) ;
#9281=VECTOR('',#109389,1000.) ;
#9282=VECTOR('',#109390,1000.) ;
#9283=VECTOR('',#109391,1000.) ;
#9284=VECTOR('',#109392,1000.) ;
#9285=VECTOR('',#109397,1000.) ;
#9286=VECTOR('',#109400,1000.) ;
#9287=VECTOR('',#109405,1000.) ;
#9288=VECTOR('',#109406,1000.) ;
#9289=VECTOR('',#109407,1000.) ;
#9290=VECTOR('',#109408,1000.) ;
#9291=VECTOR('',#109409,1000.) ;
#9292=VECTOR('',#109414,1000.) ;
#9293=VECTOR('',#109417,1000.) ;
#9294=VECTOR('',#109422,1000.) ;
#9295=VECTOR('',#109423,1000.) ;
#9296=VECTOR('',#109424,1000.) ;
#9297=VECTOR('',#109425,1000.) ;
#9298=VECTOR('',#109426,1000.) ;
#9299=VECTOR('',#109431,1000.) ;
#9300=VECTOR('',#109434,1000.) ;
#9301=VECTOR('',#109439,1000.) ;
#9302=VECTOR('',#109440,1000.) ;
#9303=VECTOR('',#109441,1000.) ;
#9304=VECTOR('',#109442,1000.) ;
#9305=VECTOR('',#109443,1000.) ;
#9306=VECTOR('',#109450,1000.) ;
#9307=VECTOR('',#109451,1000.) ;
#9308=VECTOR('',#109452,1000.) ;
#9309=VECTOR('',#109453,1000.) ;
#9310=VECTOR('',#109458,1000.) ;
#9311=VECTOR('',#109459,1000.) ;
#9312=VECTOR('',#109460,1000.) ;
#9313=VECTOR('',#109461,1000.) ;
#9314=VECTOR('',#109466,1000.) ;
#9315=VECTOR('',#109467,1000.) ;
#9316=VECTOR('',#109468,1000.) ;
#9317=VECTOR('',#109469,1000.) ;
#9318=VECTOR('',#109474,1000.) ;
#9319=VECTOR('',#109475,1000.) ;
#9320=VECTOR('',#109476,1000.) ;
#9321=VECTOR('',#109477,1000.) ;
#9322=VECTOR('',#109482,1000.) ;
#9323=VECTOR('',#109483,1000.) ;
#9324=VECTOR('',#109484,1000.) ;
#9325=VECTOR('',#109485,1000.) ;
#9326=VECTOR('',#109490,1000.) ;
#9327=VECTOR('',#109491,1000.) ;
#9328=VECTOR('',#109492,1000.) ;
#9329=VECTOR('',#109493,1000.) ;
#9330=VECTOR('',#109498,1000.) ;
#9331=VECTOR('',#109499,1000.) ;
#9332=VECTOR('',#109500,1000.) ;
#9333=VECTOR('',#109501,1000.) ;
#9334=VECTOR('',#109506,1000.) ;
#9335=VECTOR('',#109507,1000.) ;
#9336=VECTOR('',#109508,1000.) ;
#9337=VECTOR('',#109509,1000.) ;
#9338=VECTOR('',#109514,1000.) ;
#9339=VECTOR('',#109515,1000.) ;
#9340=VECTOR('',#109516,1000.) ;
#9341=VECTOR('',#109517,1000.) ;
#9342=VECTOR('',#109522,1000.) ;
#9343=VECTOR('',#109523,1000.) ;
#9344=VECTOR('',#109524,1000.) ;
#9345=VECTOR('',#109525,1000.) ;
#9346=VECTOR('',#109530,1000.) ;
#9347=VECTOR('',#109531,1000.) ;
#9348=VECTOR('',#109532,1000.) ;
#9349=VECTOR('',#109533,1000.) ;
#9350=VECTOR('',#109538,1000.) ;
#9351=VECTOR('',#109539,1000.) ;
#9352=VECTOR('',#109540,1000.) ;
#9353=VECTOR('',#109541,1000.) ;
#9354=VECTOR('',#109546,1000.) ;
#9355=VECTOR('',#109547,1000.) ;
#9356=VECTOR('',#109548,1000.) ;
#9357=VECTOR('',#109549,1000.) ;
#9358=VECTOR('',#109554,1000.) ;
#9359=VECTOR('',#109555,1000.) ;
#9360=VECTOR('',#109556,1000.) ;
#9361=VECTOR('',#109557,1000.) ;
#9362=VECTOR('',#109562,1000.) ;
#9363=VECTOR('',#109563,1000.) ;
#9364=VECTOR('',#109564,1000.) ;
#9365=VECTOR('',#109565,1000.) ;
#9366=VECTOR('',#109570,1000.) ;
#9367=VECTOR('',#109571,1000.) ;
#9368=VECTOR('',#109572,1000.) ;
#9369=VECTOR('',#109573,1000.) ;
#9370=VECTOR('',#109578,1000.) ;
#9371=VECTOR('',#109579,1000.) ;
#9372=VECTOR('',#109580,1000.) ;
#9373=VECTOR('',#109581,1000.) ;
#9374=VECTOR('',#109586,1000.) ;
#9375=VECTOR('',#109587,1000.) ;
#9376=VECTOR('',#109588,1000.) ;
#9377=VECTOR('',#109589,1000.) ;
#9378=VECTOR('',#109592,1000.) ;
#9379=VECTOR('',#109595,1000.) ;
#9380=VECTOR('',#109600,1000.) ;
#9381=VECTOR('',#109603,1000.) ;
#9382=VECTOR('',#109608,1000.) ;
#9383=VECTOR('',#109611,1000.) ;
#9384=VECTOR('',#109616,1000.) ;
#9385=VECTOR('',#109619,1000.) ;
#9386=VECTOR('',#109624,1000.) ;
#9387=VECTOR('',#109627,1000.) ;
#9388=VECTOR('',#109632,1000.) ;
#9389=VECTOR('',#109635,1000.) ;
#9390=VECTOR('',#109640,1000.) ;
#9391=VECTOR('',#109643,1000.) ;
#9392=VECTOR('',#109648,1000.) ;
#9393=VECTOR('',#109651,1000.) ;
#9394=VECTOR('',#109656,1000.) ;
#9395=VECTOR('',#109659,1000.) ;
#9396=VECTOR('',#109664,1000.) ;
#9397=VECTOR('',#109667,1000.) ;
#9398=VECTOR('',#109672,1000.) ;
#9399=VECTOR('',#109673,1000.) ;
#9400=VECTOR('',#109674,1000.) ;
#9401=VECTOR('',#109675,1000.) ;
#9402=VECTOR('',#109676,1000.) ;
#9403=VECTOR('',#109683,1000.) ;
#9404=VECTOR('',#109684,1000.) ;
#9405=VECTOR('',#109685,1000.) ;
#9406=VECTOR('',#109686,1000.) ;
#9407=VECTOR('',#109691,1000.) ;
#9408=VECTOR('',#109692,1000.) ;
#9409=VECTOR('',#109693,1000.) ;
#9410=VECTOR('',#109694,1000.) ;
#9411=VECTOR('',#109697,1000.) ;
#9412=VECTOR('',#109700,1000.) ;
#9413=VECTOR('',#109705,1000.) ;
#9414=VECTOR('',#109708,1000.) ;
#9415=VECTOR('',#109715,1000.) ;
#9416=VECTOR('',#109716,1000.) ;
#9417=VECTOR('',#109717,1000.) ;
#9418=VECTOR('',#109718,1000.) ;
#9419=VECTOR('',#109719,1000.) ;
#9420=VECTOR('',#109722,1000.) ;
#9421=VECTOR('',#109725,1000.) ;
#9422=VECTOR('',#109726,1000.) ;
#9423=VECTOR('',#109729,1000.) ;
#9424=VECTOR('',#109732,1000.) ;
#9425=VECTOR('',#109733,1000.) ;
#9426=VECTOR('',#109736,1000.) ;
#9427=VECTOR('',#109739,1000.) ;
#9428=VECTOR('',#109740,1000.) ;
#9429=VECTOR('',#109743,1000.) ;
#9430=VECTOR('',#109746,1000.) ;
#9431=VECTOR('',#109747,1000.) ;
#9432=VECTOR('',#109750,1000.) ;
#9433=VECTOR('',#109753,1000.) ;
#9434=VECTOR('',#109754,1000.) ;
#9435=VECTOR('',#109757,1000.) ;
#9436=VECTOR('',#109760,1000.) ;
#9437=VECTOR('',#109761,1000.) ;
#9438=VECTOR('',#109764,1000.) ;
#9439=VECTOR('',#109767,1000.) ;
#9440=VECTOR('',#109768,1000.) ;
#9441=VECTOR('',#109771,1000.) ;
#9442=VECTOR('',#109774,1000.) ;
#9443=VECTOR('',#109775,1000.) ;
#9444=VECTOR('',#109778,1000.) ;
#9445=VECTOR('',#109781,1000.) ;
#9446=VECTOR('',#109782,1000.) ;
#9447=VECTOR('',#109785,1000.) ;
#9448=VECTOR('',#109790,1000.) ;
#9449=VECTOR('',#109797,1000.) ;
#9450=VECTOR('',#109798,1000.) ;
#9451=VECTOR('',#109801,1000.) ;
#9452=VECTOR('',#109804,1000.) ;
#9453=VECTOR('',#109805,1000.) ;
#9454=VECTOR('',#109808,1000.) ;
#9455=VECTOR('',#109811,1000.) ;
#9456=VECTOR('',#109812,1000.) ;
#9457=VECTOR('',#109815,1000.) ;
#9458=VECTOR('',#109818,1000.) ;
#9459=VECTOR('',#109819,1000.) ;
#9460=VECTOR('',#109822,1000.) ;
#9461=VECTOR('',#109825,1000.) ;
#9462=VECTOR('',#109826,1000.) ;
#9463=VECTOR('',#109829,1000.) ;
#9464=VECTOR('',#109832,1000.) ;
#9465=VECTOR('',#109833,1000.) ;
#9466=VECTOR('',#109836,1000.) ;
#9467=VECTOR('',#109839,1000.) ;
#9468=VECTOR('',#109840,1000.) ;
#9469=VECTOR('',#109843,1000.) ;
#9470=VECTOR('',#109846,1000.) ;
#9471=VECTOR('',#109847,1000.) ;
#9472=VECTOR('',#109850,1000.) ;
#9473=VECTOR('',#109853,1000.) ;
#9474=VECTOR('',#109854,1000.) ;
#9475=VECTOR('',#109857,1000.) ;
#9476=VECTOR('',#109860,1000.) ;
#9477=VECTOR('',#109861,1000.) ;
#9478=VECTOR('',#109862,1000.) ;
#9479=VECTOR('',#109863,1000.) ;
#9480=VECTOR('',#109864,1000.) ;
#9481=VECTOR('',#109867,1000.) ;
#9482=VECTOR('',#109870,1000.) ;
#9483=VECTOR('',#109877,1000.) ;
#9484=VECTOR('',#109878,1000.) ;
#9485=VECTOR('',#109879,1000.) ;
#9486=VECTOR('',#109882,1000.) ;
#9487=VECTOR('',#109889,1000.) ;
#9488=VECTOR('',#109890,1000.) ;
#9489=VECTOR('',#109891,1000.) ;
#9490=VECTOR('',#109894,1000.) ;
#9491=VECTOR('',#109901,1000.) ;
#9492=VECTOR('',#109902,1000.) ;
#9493=VECTOR('',#109903,1000.) ;
#9494=VECTOR('',#109906,1000.) ;
#9495=VECTOR('',#109913,1000.) ;
#9496=VECTOR('',#109914,1000.) ;
#9497=VECTOR('',#109915,1000.) ;
#9498=VECTOR('',#109918,1000.) ;
#9499=VECTOR('',#109925,1000.) ;
#9500=VECTOR('',#109926,1000.) ;
#9501=VECTOR('',#109927,1000.) ;
#9502=VECTOR('',#109930,1000.) ;
#9503=VECTOR('',#109937,1000.) ;
#9504=VECTOR('',#109938,1000.) ;
#9505=VECTOR('',#109941,1000.) ;
#9506=VECTOR('',#109942,1000.) ;
#9507=VECTOR('',#109943,1000.) ;
#9508=VECTOR('',#109946,1000.) ;
#9509=VECTOR('',#109949,1000.) ;
#9510=VECTOR('',#109950,1000.) ;
#9511=VECTOR('',#109953,1000.) ;
#9512=VECTOR('',#109954,1000.) ;
#9513=VECTOR('',#109955,1000.) ;
#9514=VECTOR('',#109958,1000.) ;
#9515=VECTOR('',#109961,1000.) ;
#9516=VECTOR('',#109968,1000.) ;
#9517=VECTOR('',#109971,1000.) ;
#9518=VECTOR('',#109974,1000.) ;
#9519=VECTOR('',#109975,1000.) ;
#9520=VECTOR('',#109976,1000.) ;
#9521=VECTOR('',#109979,1000.) ;
#9522=VECTOR('',#109982,1000.) ;
#9523=VECTOR('',#109983,1000.) ;
#9524=VECTOR('',#109986,1000.) ;
#9525=VECTOR('',#109987,1000.) ;
#9526=VECTOR('',#109988,1000.) ;
#9527=VECTOR('',#109991,1000.) ;
#9528=VECTOR('',#109994,1000.) ;
#9529=VECTOR('',#110001,1000.) ;
#9530=VECTOR('',#110004,1000.) ;
#9531=VECTOR('',#110007,1000.) ;
#9532=VECTOR('',#110008,1000.) ;
#9533=VECTOR('',#110009,1000.) ;
#9534=VECTOR('',#110012,1000.) ;
#9535=VECTOR('',#110015,1000.) ;
#9536=VECTOR('',#110016,1000.) ;
#9537=VECTOR('',#110019,1000.) ;
#9538=VECTOR('',#110020,1000.) ;
#9539=VECTOR('',#110021,1000.) ;
#9540=VECTOR('',#110024,1000.) ;
#9541=VECTOR('',#110027,1000.) ;
#9542=VECTOR('',#110034,1000.) ;
#9543=VECTOR('',#110037,1000.) ;
#9544=VECTOR('',#110040,1000.) ;
#9545=VECTOR('',#110041,1000.) ;
#9546=VECTOR('',#110042,1000.) ;
#9547=VECTOR('',#110045,1000.) ;
#9548=VECTOR('',#110048,1000.) ;
#9549=VECTOR('',#110049,1000.) ;
#9550=VECTOR('',#110052,1000.) ;
#9551=VECTOR('',#110053,1000.) ;
#9552=VECTOR('',#110054,1000.) ;
#9553=VECTOR('',#110057,1000.) ;
#9554=VECTOR('',#110060,1000.) ;
#9555=VECTOR('',#110067,1000.) ;
#9556=VECTOR('',#110070,1000.) ;
#9557=VECTOR('',#110073,1000.) ;
#9558=VECTOR('',#110074,1000.) ;
#9559=VECTOR('',#110075,1000.) ;
#9560=VECTOR('',#110078,1000.) ;
#9561=VECTOR('',#110081,1000.) ;
#9562=VECTOR('',#110082,1000.) ;
#9563=VECTOR('',#110085,1000.) ;
#9564=VECTOR('',#110086,1000.) ;
#9565=VECTOR('',#110087,1000.) ;
#9566=VECTOR('',#110090,1000.) ;
#9567=VECTOR('',#110093,1000.) ;
#9568=VECTOR('',#110100,1000.) ;
#9569=VECTOR('',#110103,1000.) ;
#9570=VECTOR('',#110106,1000.) ;
#9571=VECTOR('',#110107,1000.) ;
#9572=VECTOR('',#110108,1000.) ;
#9573=VECTOR('',#110111,1000.) ;
#9574=VECTOR('',#110114,1000.) ;
#9575=VECTOR('',#110115,1000.) ;
#9576=VECTOR('',#110118,1000.) ;
#9577=VECTOR('',#110119,1000.) ;
#9578=VECTOR('',#110120,1000.) ;
#9579=VECTOR('',#110123,1000.) ;
#9580=VECTOR('',#110126,1000.) ;
#9581=VECTOR('',#110133,1000.) ;
#9582=VECTOR('',#110136,1000.) ;
#9583=VECTOR('',#110139,1000.) ;
#9584=VECTOR('',#110140,1000.) ;
#9585=VECTOR('',#110141,1000.) ;
#9586=VECTOR('',#110144,1000.) ;
#9587=VECTOR('',#110147,1000.) ;
#9588=VECTOR('',#110148,1000.) ;
#9589=VECTOR('',#110151,1000.) ;
#9590=VECTOR('',#110152,1000.) ;
#9591=VECTOR('',#110153,1000.) ;
#9592=VECTOR('',#110156,1000.) ;
#9593=VECTOR('',#110159,1000.) ;
#9594=VECTOR('',#110166,1000.) ;
#9595=VECTOR('',#110169,1000.) ;
#9596=VECTOR('',#110172,1000.) ;
#9597=VECTOR('',#110173,1000.) ;
#9598=VECTOR('',#110174,1000.) ;
#9599=VECTOR('',#110177,1000.) ;
#9600=VECTOR('',#110180,1000.) ;
#9601=VECTOR('',#110181,1000.) ;
#9602=VECTOR('',#110184,1000.) ;
#9603=VECTOR('',#110185,1000.) ;
#9604=VECTOR('',#110186,1000.) ;
#9605=VECTOR('',#110189,1000.) ;
#9606=VECTOR('',#110192,1000.) ;
#9607=VECTOR('',#110199,1000.) ;
#9608=VECTOR('',#110202,1000.) ;
#9609=VECTOR('',#110205,1000.) ;
#9610=VECTOR('',#110206,1000.) ;
#9611=VECTOR('',#110207,1000.) ;
#9612=VECTOR('',#110210,1000.) ;
#9613=VECTOR('',#110213,1000.) ;
#9614=VECTOR('',#110214,1000.) ;
#9615=VECTOR('',#110217,1000.) ;
#9616=VECTOR('',#110218,1000.) ;
#9617=VECTOR('',#110219,1000.) ;
#9618=VECTOR('',#110222,1000.) ;
#9619=VECTOR('',#110225,1000.) ;
#9620=VECTOR('',#110232,1000.) ;
#9621=VECTOR('',#110235,1000.) ;
#9622=VECTOR('',#110238,1000.) ;
#9623=VECTOR('',#110239,1000.) ;
#9624=VECTOR('',#110240,1000.) ;
#9625=VECTOR('',#110243,1000.) ;
#9626=VECTOR('',#110246,1000.) ;
#9627=VECTOR('',#110247,1000.) ;
#9628=VECTOR('',#110250,1000.) ;
#9629=VECTOR('',#110251,1000.) ;
#9630=VECTOR('',#110252,1000.) ;
#9631=VECTOR('',#110255,1000.) ;
#9632=VECTOR('',#110258,1000.) ;
#9633=VECTOR('',#110265,1000.) ;
#9634=VECTOR('',#110268,1000.) ;
#9635=VECTOR('',#110271,1000.) ;
#9636=VECTOR('',#110272,1000.) ;
#9637=VECTOR('',#110273,1000.) ;
#9638=VECTOR('',#110274,1000.) ;
#9639=VECTOR('',#110277,1000.) ;
#9640=VECTOR('',#110278,1000.) ;
#9641=VECTOR('',#110279,1000.) ;
#9642=VECTOR('',#110282,1000.) ;
#9643=VECTOR('',#110285,1000.) ;
#9644=VECTOR('',#110286,1000.) ;
#9645=VECTOR('',#110287,1000.) ;
#9646=VECTOR('',#110288,1000.) ;
#9647=VECTOR('',#110291,1000.) ;
#9648=VECTOR('',#110292,1000.) ;
#9649=VECTOR('',#110293,1000.) ;
#9650=VECTOR('',#110296,1000.) ;
#9651=VECTOR('',#110299,1000.) ;
#9652=VECTOR('',#110300,1000.) ;
#9653=VECTOR('',#110301,1000.) ;
#9654=VECTOR('',#110302,1000.) ;
#9655=VECTOR('',#110303,1000.) ;
#9656=VECTOR('',#110304,1000.) ;
#9657=VECTOR('',#110307,1000.) ;
#9658=VECTOR('',#110310,1000.) ;
#9659=VECTOR('',#110313,1000.) ;
#9660=VECTOR('',#110314,1000.) ;
#9661=VECTOR('',#110315,1000.) ;
#9662=VECTOR('',#110316,1000.) ;
#9663=VECTOR('',#110319,1000.) ;
#9664=VECTOR('',#110320,1000.) ;
#9665=VECTOR('',#110321,1000.) ;
#9666=VECTOR('',#110324,1000.) ;
#9667=VECTOR('',#110325,1000.) ;
#9668=VECTOR('',#110326,1000.) ;
#9669=VECTOR('',#110327,1000.) ;
#9670=VECTOR('',#110330,1000.) ;
#9671=VECTOR('',#110331,1000.) ;
#9672=VECTOR('',#110332,1000.) ;
#9673=VECTOR('',#110333,1000.) ;
#9674=VECTOR('',#110336,1000.) ;
#9675=VECTOR('',#110337,1000.) ;
#9676=VECTOR('',#110338,1000.) ;
#9677=VECTOR('',#110339,1000.) ;
#9678=VECTOR('',#110342,1000.) ;
#9679=VECTOR('',#110345,1000.) ;
#9680=VECTOR('',#110350,1000.) ;
#9681=VECTOR('',#110351,1000.) ;
#9682=VECTOR('',#110352,1000.) ;
#9683=VECTOR('',#110357,1000.) ;
#9684=VECTOR('',#110362,1000.) ;
#9685=VECTOR('',#110363,1000.) ;
#9686=VECTOR('',#110364,1000.) ;
#9687=VECTOR('',#110369,1000.) ;
#9688=VECTOR('',#110374,1000.) ;
#9689=VECTOR('',#110375,1000.) ;
#9690=VECTOR('',#110376,1000.) ;
#9691=VECTOR('',#110379,1000.) ;
#9692=VECTOR('',#110384,1000.) ;
#9693=VECTOR('',#110385,1000.) ;
#9694=VECTOR('',#110388,1000.) ;
#9695=VECTOR('',#110389,1000.) ;
#9696=VECTOR('',#110390,1000.) ;
#9697=VECTOR('',#110395,1000.) ;
#9698=VECTOR('',#110400,1000.) ;
#9699=VECTOR('',#110401,1000.) ;
#9700=VECTOR('',#110402,1000.) ;
#9701=VECTOR('',#110407,1000.) ;
#9702=VECTOR('',#110412,1000.) ;
#9703=VECTOR('',#110413,1000.) ;
#9704=VECTOR('',#110414,1000.) ;
#9705=VECTOR('',#110419,1000.) ;
#9706=VECTOR('',#110424,1000.) ;
#9707=VECTOR('',#110425,1000.) ;
#9708=VECTOR('',#110426,1000.) ;
#9709=VECTOR('',#110431,1000.) ;
#9710=VECTOR('',#110436,1000.) ;
#9711=VECTOR('',#110437,1000.) ;
#9712=VECTOR('',#110438,1000.) ;
#9713=VECTOR('',#110443,1000.) ;
#9714=VECTOR('',#110448,1000.) ;
#9715=VECTOR('',#110449,1000.) ;
#9716=VECTOR('',#110450,1000.) ;
#9717=VECTOR('',#110455,1000.) ;
#9718=VECTOR('',#110462,1000.) ;
#9719=VECTOR('',#110469,1000.) ;
#9720=VECTOR('',#110474,1000.) ;
#9721=VECTOR('',#110475,1000.) ;
#9722=VECTOR('',#110476,1000.) ;
#9723=VECTOR('',#110481,1000.) ;
#9724=VECTOR('',#110486,1000.) ;
#9725=VECTOR('',#110487,1000.) ;
#9726=VECTOR('',#110488,1000.) ;
#9727=VECTOR('',#110493,1000.) ;
#9728=VECTOR('',#110498,1000.) ;
#9729=VECTOR('',#110499,1000.) ;
#9730=VECTOR('',#110504,1000.) ;
#9731=VECTOR('',#110507,1000.) ;
#9732=VECTOR('',#110508,1000.) ;
#9733=VECTOR('',#110509,1000.) ;
#9734=VECTOR('',#110512,1000.) ;
#9735=VECTOR('',#110513,1000.) ;
#9736=VECTOR('',#110514,1000.) ;
#9737=VECTOR('',#110517,1000.) ;
#9738=VECTOR('',#110520,1000.) ;
#9739=VECTOR('',#110521,1000.) ;
#9740=VECTOR('',#110522,1000.) ;
#9741=VECTOR('',#110523,1000.) ;
#9742=VECTOR('',#110524,1000.) ;
#9743=VECTOR('',#110527,1000.) ;
#9744=VECTOR('',#110530,1000.) ;
#9745=VECTOR('',#110533,1000.) ;
#9746=VECTOR('',#110536,1000.) ;
#9747=VECTOR('',#110571,1000.) ;
#9748=VECTOR('',#110574,1000.) ;
#9749=VECTOR('',#110621,1000.) ;
#9750=VECTOR('',#110680,1000.) ;
#9751=VECTOR('',#110729,1000.) ;
#9752=VECTOR('',#111086,1000.) ;
#9753=VECTOR('',#111087,1000.) ;
#9754=VECTOR('',#111088,1000.) ;
#9755=VECTOR('',#111089,1000.) ;
#9756=VECTOR('',#111092,1000.) ;
#9757=VECTOR('',#111093,1000.) ;
#9758=VECTOR('',#111094,1000.) ;
#9759=VECTOR('',#111095,1000.) ;
#9760=VECTOR('',#111098,1000.) ;
#9761=VECTOR('',#111099,1000.) ;
#9762=VECTOR('',#111100,1000.) ;
#9763=VECTOR('',#111101,1000.) ;
#9764=VECTOR('',#111104,1000.) ;
#9765=VECTOR('',#111105,1000.) ;
#9766=VECTOR('',#111106,1000.) ;
#9767=VECTOR('',#111107,1000.) ;
#9768=VECTOR('',#111110,1000.) ;
#9769=VECTOR('',#111111,1000.) ;
#9770=VECTOR('',#111112,1000.) ;
#9771=VECTOR('',#111113,1000.) ;
#9772=VECTOR('',#111116,1000.) ;
#9773=VECTOR('',#111121,1000.) ;
#9774=VECTOR('',#111122,1000.) ;
#9775=VECTOR('',#111125,1000.) ;
#9776=VECTOR('',#111130,1000.) ;
#9777=VECTOR('',#111131,1000.) ;
#9778=VECTOR('',#111146,1000.) ;
#9779=VECTOR('',#111147,1000.) ;
#9780=VECTOR('',#111148,1000.) ;
#9781=VECTOR('',#111149,1000.) ;
#9782=VECTOR('',#111152,1000.) ;
#9783=VECTOR('',#111153,1000.) ;
#9784=VECTOR('',#111154,1000.) ;
#9785=VECTOR('',#111157,1000.) ;
#9786=VECTOR('',#111158,1000.) ;
#9787=VECTOR('',#111159,1000.) ;
#9788=VECTOR('',#111162,1000.) ;
#9789=VECTOR('',#111163,1000.) ;
#9790=VECTOR('',#111164,1000.) ;
#9791=VECTOR('',#111165,1000.) ;
#9792=VECTOR('',#111168,1000.) ;
#9793=VECTOR('',#111169,1000.) ;
#9794=VECTOR('',#111170,1000.) ;
#9795=VECTOR('',#111171,1000.) ;
#9796=VECTOR('',#111174,1000.) ;
#9797=VECTOR('',#111175,1000.) ;
#9798=VECTOR('',#111176,1000.) ;
#9799=VECTOR('',#111179,1000.) ;
#9800=VECTOR('',#111180,1000.) ;
#9801=VECTOR('',#111181,1000.) ;
#9802=VECTOR('',#111184,1000.) ;
#9803=VECTOR('',#111185,1000.) ;
#9804=VECTOR('',#111186,1000.) ;
#9805=VECTOR('',#111187,1000.) ;
#9806=VECTOR('',#111190,1000.) ;
#9807=VECTOR('',#111191,1000.) ;
#9808=VECTOR('',#111192,1000.) ;
#9809=VECTOR('',#111193,1000.) ;
#9810=VECTOR('',#111196,1000.) ;
#9811=VECTOR('',#111197,1000.) ;
#9812=VECTOR('',#111198,1000.) ;
#9813=VECTOR('',#111199,1000.) ;
#9814=VECTOR('',#111202,1000.) ;
#9815=VECTOR('',#111203,1000.) ;
#9816=VECTOR('',#111204,1000.) ;
#9817=VECTOR('',#111205,1000.) ;
#9818=VECTOR('',#111432,1000.) ;
#9819=VECTOR('',#111433,1000.) ;
#9820=VECTOR('',#111434,1000.) ;
#9821=VECTOR('',#111435,1000.) ;
#9822=VECTOR('',#111436,1000.) ;
#9823=VECTOR('',#111437,1000.) ;
#9824=VECTOR('',#111440,1000.) ;
#9825=VECTOR('',#111443,1000.) ;
#9826=VECTOR('',#111446,1000.) ;
#9827=VECTOR('',#111447,1000.) ;
#9828=VECTOR('',#111448,1000.) ;
#9829=VECTOR('',#111449,1000.) ;
#9830=VECTOR('',#111450,1000.) ;
#9831=VECTOR('',#111451,1000.) ;
#9832=VECTOR('',#111454,1000.) ;
#9833=VECTOR('',#111457,1000.) ;
#9834=VECTOR('',#111460,1000.) ;
#9835=VECTOR('',#111461,1000.) ;
#9836=VECTOR('',#111462,1000.) ;
#9837=VECTOR('',#111463,1000.) ;
#9838=VECTOR('',#111464,1000.) ;
#9839=VECTOR('',#111465,1000.) ;
#9840=VECTOR('',#111468,1000.) ;
#9841=VECTOR('',#111471,1000.) ;
#9842=VECTOR('',#111474,1000.) ;
#9843=VECTOR('',#111475,1000.) ;
#9844=VECTOR('',#111476,1000.) ;
#9845=VECTOR('',#111477,1000.) ;
#9846=VECTOR('',#111478,1000.) ;
#9847=VECTOR('',#111479,1000.) ;
#9848=VECTOR('',#111482,1000.) ;
#9849=VECTOR('',#111485,1000.) ;
#9850=VECTOR('',#111488,1000.) ;
#9851=VECTOR('',#111489,1000.) ;
#9852=VECTOR('',#111490,1000.) ;
#9853=VECTOR('',#111491,1000.) ;
#9854=VECTOR('',#111492,1000.) ;
#9855=VECTOR('',#111493,1000.) ;
#9856=VECTOR('',#111496,1000.) ;
#9857=VECTOR('',#111499,1000.) ;
#9858=VECTOR('',#111502,1000.) ;
#9859=VECTOR('',#111503,1000.) ;
#9860=VECTOR('',#111504,1000.) ;
#9861=VECTOR('',#111505,1000.) ;
#9862=VECTOR('',#111506,1000.) ;
#9863=VECTOR('',#111507,1000.) ;
#9864=VECTOR('',#111510,1000.) ;
#9865=VECTOR('',#111513,1000.) ;
#9866=VECTOR('',#111516,1000.) ;
#9867=VECTOR('',#111517,1000.) ;
#9868=VECTOR('',#111518,1000.) ;
#9869=VECTOR('',#111519,1000.) ;
#9870=VECTOR('',#111520,1000.) ;
#9871=VECTOR('',#111521,1000.) ;
#9872=VECTOR('',#111524,1000.) ;
#9873=VECTOR('',#111527,1000.) ;
#9874=VECTOR('',#111530,1000.) ;
#9875=VECTOR('',#111531,1000.) ;
#9876=VECTOR('',#111532,1000.) ;
#9877=VECTOR('',#111533,1000.) ;
#9878=VECTOR('',#111534,1000.) ;
#9879=VECTOR('',#111535,1000.) ;
#9880=VECTOR('',#111538,1000.) ;
#9881=VECTOR('',#111541,1000.) ;
#9882=VECTOR('',#111544,1000.) ;
#9883=VECTOR('',#111545,1000.) ;
#9884=VECTOR('',#111546,1000.) ;
#9885=VECTOR('',#111547,1000.) ;
#9886=VECTOR('',#111548,1000.) ;
#9887=VECTOR('',#111549,1000.) ;
#9888=VECTOR('',#111552,1000.) ;
#9889=VECTOR('',#111555,1000.) ;
#9890=VECTOR('',#111558,1000.) ;
#9891=VECTOR('',#111559,1000.) ;
#9892=VECTOR('',#111560,1000.) ;
#9893=VECTOR('',#111561,1000.) ;
#9894=VECTOR('',#111564,1000.) ;
#9895=VECTOR('',#111565,1000.) ;
#9896=VECTOR('',#111566,1000.) ;
#9897=VECTOR('',#111569,1000.) ;
#9898=VECTOR('',#111570,1000.) ;
#9899=VECTOR('',#111571,1000.) ;
#9900=VECTOR('',#111572,1000.) ;
#9901=VECTOR('',#111575,1000.) ;
#9902=VECTOR('',#111576,1000.) ;
#9903=VECTOR('',#111577,1000.) ;
#9904=VECTOR('',#111578,1000.) ;
#9905=VECTOR('',#111581,1000.) ;
#9906=VECTOR('',#111582,1000.) ;
#9907=VECTOR('',#111583,1000.) ;
#9908=VECTOR('',#111584,1000.) ;
#9909=VECTOR('',#111587,1000.) ;
#9910=VECTOR('',#111588,1000.) ;
#9911=VECTOR('',#111589,1000.) ;
#9912=VECTOR('',#111590,1000.) ;
#9913=VECTOR('',#111593,1000.) ;
#9914=VECTOR('',#111594,1000.) ;
#9915=VECTOR('',#111595,1000.) ;
#9916=VECTOR('',#111598,1000.) ;
#9917=VECTOR('',#111599,1000.) ;
#9918=VECTOR('',#111600,1000.) ;
#9919=VECTOR('',#111601,1000.) ;
#9920=VECTOR('',#111604,1000.) ;
#9921=VECTOR('',#111605,1000.) ;
#9922=VECTOR('',#111606,1000.) ;
#9923=VECTOR('',#111607,1000.) ;
#9924=VECTOR('',#111610,1000.) ;
#9925=VECTOR('',#111611,1000.) ;
#9926=VECTOR('',#111612,1000.) ;
#9927=VECTOR('',#111613,1000.) ;
#9928=VECTOR('',#111616,1000.) ;
#9929=VECTOR('',#111617,1000.) ;
#9930=VECTOR('',#111618,1000.) ;
#9931=VECTOR('',#111619,1000.) ;
#9932=VECTOR('',#111622,1000.) ;
#9933=VECTOR('',#111623,1000.) ;
#9934=VECTOR('',#111624,1000.) ;
#9935=VECTOR('',#111627,1000.) ;
#9936=VECTOR('',#111628,1000.) ;
#9937=VECTOR('',#111629,1000.) ;
#9938=VECTOR('',#111630,1000.) ;
#9939=VECTOR('',#111633,1000.) ;
#9940=VECTOR('',#111634,1000.) ;
#9941=VECTOR('',#111635,1000.) ;
#9942=VECTOR('',#111636,1000.) ;
#9943=VECTOR('',#111639,1000.) ;
#9944=VECTOR('',#111640,1000.) ;
#9945=VECTOR('',#111641,1000.) ;
#9946=VECTOR('',#111642,1000.) ;
#9947=VECTOR('',#111645,1000.) ;
#9948=VECTOR('',#111646,1000.) ;
#9949=VECTOR('',#111647,1000.) ;
#9950=VECTOR('',#111648,1000.) ;
#9951=VECTOR('',#111651,1000.) ;
#9952=VECTOR('',#111652,1000.) ;
#9953=VECTOR('',#111653,1000.) ;
#9954=VECTOR('',#111656,1000.) ;
#9955=VECTOR('',#111657,1000.) ;
#9956=VECTOR('',#111658,1000.) ;
#9957=VECTOR('',#111659,1000.) ;
#9958=VECTOR('',#111662,1000.) ;
#9959=VECTOR('',#111663,1000.) ;
#9960=VECTOR('',#111664,1000.) ;
#9961=VECTOR('',#111665,1000.) ;
#9962=VECTOR('',#111668,1000.) ;
#9963=VECTOR('',#111669,1000.) ;
#9964=VECTOR('',#111670,1000.) ;
#9965=VECTOR('',#111671,1000.) ;
#9966=VECTOR('',#111674,1000.) ;
#9967=VECTOR('',#111675,1000.) ;
#9968=VECTOR('',#111676,1000.) ;
#9969=VECTOR('',#111677,1000.) ;
#9970=VECTOR('',#111680,1000.) ;
#9971=VECTOR('',#111681,1000.) ;
#9972=VECTOR('',#111682,1000.) ;
#9973=VECTOR('',#111685,1000.) ;
#9974=VECTOR('',#111686,1000.) ;
#9975=VECTOR('',#111687,1000.) ;
#9976=VECTOR('',#111688,1000.) ;
#9977=VECTOR('',#111691,1000.) ;
#9978=VECTOR('',#111692,1000.) ;
#9979=VECTOR('',#111693,1000.) ;
#9980=VECTOR('',#111694,1000.) ;
#9981=VECTOR('',#111697,1000.) ;
#9982=VECTOR('',#111698,1000.) ;
#9983=VECTOR('',#111699,1000.) ;
#9984=VECTOR('',#111700,1000.) ;
#9985=VECTOR('',#111703,1000.) ;
#9986=VECTOR('',#111704,1000.) ;
#9987=VECTOR('',#111705,1000.) ;
#9988=VECTOR('',#111706,1000.) ;
#9989=VECTOR('',#111709,1000.) ;
#9990=VECTOR('',#111710,1000.) ;
#9991=VECTOR('',#111711,1000.) ;
#9992=VECTOR('',#111714,1000.) ;
#9993=VECTOR('',#111715,1000.) ;
#9994=VECTOR('',#111716,1000.) ;
#9995=VECTOR('',#111717,1000.) ;
#9996=VECTOR('',#111720,1000.) ;
#9997=VECTOR('',#111721,1000.) ;
#9998=VECTOR('',#111722,1000.) ;
#9999=VECTOR('',#111723,1000.) ;
#10000=VECTOR('',#111726,1000.) ;
#10001=VECTOR('',#111727,1000.) ;
#10002=VECTOR('',#111728,1000.) ;
#10003=VECTOR('',#111729,1000.) ;
#10004=VECTOR('',#111732,1000.) ;
#10005=VECTOR('',#111733,1000.) ;
#10006=VECTOR('',#111734,1000.) ;
#10007=VECTOR('',#111735,1000.) ;
#10008=VECTOR('',#111738,1000.) ;
#10009=VECTOR('',#111739,1000.) ;
#10010=VECTOR('',#111740,1000.) ;
#10011=VECTOR('',#111743,1000.) ;
#10012=VECTOR('',#111744,1000.) ;
#10013=VECTOR('',#111745,1000.) ;
#10014=VECTOR('',#111746,1000.) ;
#10015=VECTOR('',#111749,1000.) ;
#10016=VECTOR('',#111750,1000.) ;
#10017=VECTOR('',#111751,1000.) ;
#10018=VECTOR('',#111752,1000.) ;
#10019=VECTOR('',#111755,1000.) ;
#10020=VECTOR('',#111756,1000.) ;
#10021=VECTOR('',#111757,1000.) ;
#10022=VECTOR('',#111758,1000.) ;
#10023=VECTOR('',#111761,1000.) ;
#10024=VECTOR('',#111762,1000.) ;
#10025=VECTOR('',#111763,1000.) ;
#10026=VECTOR('',#111764,1000.) ;
#10027=VECTOR('',#111767,1000.) ;
#10028=VECTOR('',#111768,1000.) ;
#10029=VECTOR('',#111769,1000.) ;
#10030=VECTOR('',#111772,1000.) ;
#10031=VECTOR('',#111773,1000.) ;
#10032=VECTOR('',#111774,1000.) ;
#10033=VECTOR('',#111775,1000.) ;
#10034=VECTOR('',#111778,1000.) ;
#10035=VECTOR('',#111779,1000.) ;
#10036=VECTOR('',#111780,1000.) ;
#10037=VECTOR('',#111781,1000.) ;
#10038=VECTOR('',#111784,1000.) ;
#10039=VECTOR('',#111785,1000.) ;
#10040=VECTOR('',#111786,1000.) ;
#10041=VECTOR('',#111787,1000.) ;
#10042=VECTOR('',#111790,1000.) ;
#10043=VECTOR('',#111791,1000.) ;
#10044=VECTOR('',#111792,1000.) ;
#10045=VECTOR('',#111793,1000.) ;
#10046=VECTOR('',#111796,1000.) ;
#10047=VECTOR('',#111797,1000.) ;
#10048=VECTOR('',#111798,1000.) ;
#10049=VECTOR('',#111801,1000.) ;
#10050=VECTOR('',#111802,1000.) ;
#10051=VECTOR('',#111803,1000.) ;
#10052=VECTOR('',#111804,1000.) ;
#10053=VECTOR('',#111807,1000.) ;
#10054=VECTOR('',#111808,1000.) ;
#10055=VECTOR('',#111809,1000.) ;
#10056=VECTOR('',#111810,1000.) ;
#10057=VECTOR('',#111813,1000.) ;
#10058=VECTOR('',#111814,1000.) ;
#10059=VECTOR('',#111815,1000.) ;
#10060=VECTOR('',#111816,1000.) ;
#10061=VECTOR('',#111819,1000.) ;
#10062=VECTOR('',#111822,1000.) ;
#10063=VECTOR('',#111827,1000.) ;
#10064=VECTOR('',#111828,1000.) ;
#10065=VECTOR('',#111829,1000.) ;
#10066=VECTOR('',#111834,1000.) ;
#10067=VECTOR('',#111839,1000.) ;
#10068=VECTOR('',#111840,1000.) ;
#10069=VECTOR('',#111841,1000.) ;
#10070=VECTOR('',#111846,1000.) ;
#10071=VECTOR('',#111851,1000.) ;
#10072=VECTOR('',#111852,1000.) ;
#10073=VECTOR('',#111853,1000.) ;
#10074=VECTOR('',#111856,1000.) ;
#10075=VECTOR('',#111861,1000.) ;
#10076=VECTOR('',#111862,1000.) ;
#10077=VECTOR('',#111865,1000.) ;
#10078=VECTOR('',#111866,1000.) ;
#10079=VECTOR('',#111867,1000.) ;
#10080=VECTOR('',#111872,1000.) ;
#10081=VECTOR('',#111877,1000.) ;
#10082=VECTOR('',#111878,1000.) ;
#10083=VECTOR('',#111879,1000.) ;
#10084=VECTOR('',#111884,1000.) ;
#10085=VECTOR('',#111889,1000.) ;
#10086=VECTOR('',#111890,1000.) ;
#10087=VECTOR('',#111891,1000.) ;
#10088=VECTOR('',#111896,1000.) ;
#10089=VECTOR('',#111901,1000.) ;
#10090=VECTOR('',#111902,1000.) ;
#10091=VECTOR('',#111903,1000.) ;
#10092=VECTOR('',#111908,1000.) ;
#10093=VECTOR('',#111913,1000.) ;
#10094=VECTOR('',#111914,1000.) ;
#10095=VECTOR('',#111915,1000.) ;
#10096=VECTOR('',#111920,1000.) ;
#10097=VECTOR('',#111925,1000.) ;
#10098=VECTOR('',#111926,1000.) ;
#10099=VECTOR('',#111927,1000.) ;
#10100=VECTOR('',#111932,1000.) ;
#10101=VECTOR('',#111939,1000.) ;
#10102=VECTOR('',#111946,1000.) ;
#10103=VECTOR('',#111951,1000.) ;
#10104=VECTOR('',#111952,1000.) ;
#10105=VECTOR('',#111953,1000.) ;
#10106=VECTOR('',#111958,1000.) ;
#10107=VECTOR('',#111963,1000.) ;
#10108=VECTOR('',#111964,1000.) ;
#10109=VECTOR('',#111965,1000.) ;
#10110=VECTOR('',#111970,1000.) ;
#10111=VECTOR('',#111975,1000.) ;
#10112=VECTOR('',#111976,1000.) ;
#10113=VECTOR('',#111981,1000.) ;
#10114=VECTOR('',#111984,1000.) ;
#10115=VECTOR('',#111985,1000.) ;
#10116=VECTOR('',#111986,1000.) ;
#10117=VECTOR('',#111989,1000.) ;
#10118=VECTOR('',#111990,1000.) ;
#10119=VECTOR('',#111991,1000.) ;
#10120=VECTOR('',#111994,1000.) ;
#10121=VECTOR('',#111997,1000.) ;
#10122=VECTOR('',#111998,1000.) ;
#10123=VECTOR('',#111999,1000.) ;
#10124=VECTOR('',#112000,1000.) ;
#10125=VECTOR('',#112001,1000.) ;
#10126=VECTOR('',#112004,1000.) ;
#10127=VECTOR('',#112007,1000.) ;
#10128=VECTOR('',#112012,1000.) ;
#10129=VECTOR('',#112013,1000.) ;
#10130=VECTOR('',#112014,1000.) ;
#10131=VECTOR('',#112019,1000.) ;
#10132=VECTOR('',#112024,1000.) ;
#10133=VECTOR('',#112025,1000.) ;
#10134=VECTOR('',#112026,1000.) ;
#10135=VECTOR('',#112031,1000.) ;
#10136=VECTOR('',#112036,1000.) ;
#10137=VECTOR('',#112037,1000.) ;
#10138=VECTOR('',#112038,1000.) ;
#10139=VECTOR('',#112041,1000.) ;
#10140=VECTOR('',#112046,1000.) ;
#10141=VECTOR('',#112047,1000.) ;
#10142=VECTOR('',#112050,1000.) ;
#10143=VECTOR('',#112051,1000.) ;
#10144=VECTOR('',#112052,1000.) ;
#10145=VECTOR('',#112057,1000.) ;
#10146=VECTOR('',#112062,1000.) ;
#10147=VECTOR('',#112063,1000.) ;
#10148=VECTOR('',#112064,1000.) ;
#10149=VECTOR('',#112069,1000.) ;
#10150=VECTOR('',#112074,1000.) ;
#10151=VECTOR('',#112075,1000.) ;
#10152=VECTOR('',#112076,1000.) ;
#10153=VECTOR('',#112081,1000.) ;
#10154=VECTOR('',#112086,1000.) ;
#10155=VECTOR('',#112087,1000.) ;
#10156=VECTOR('',#112088,1000.) ;
#10157=VECTOR('',#112093,1000.) ;
#10158=VECTOR('',#112098,1000.) ;
#10159=VECTOR('',#112099,1000.) ;
#10160=VECTOR('',#112100,1000.) ;
#10161=VECTOR('',#112105,1000.) ;
#10162=VECTOR('',#112110,1000.) ;
#10163=VECTOR('',#112111,1000.) ;
#10164=VECTOR('',#112112,1000.) ;
#10165=VECTOR('',#112117,1000.) ;
#10166=VECTOR('',#112124,1000.) ;
#10167=VECTOR('',#112131,1000.) ;
#10168=VECTOR('',#112136,1000.) ;
#10169=VECTOR('',#112137,1000.) ;
#10170=VECTOR('',#112138,1000.) ;
#10171=VECTOR('',#112143,1000.) ;
#10172=VECTOR('',#112148,1000.) ;
#10173=VECTOR('',#112149,1000.) ;
#10174=VECTOR('',#112150,1000.) ;
#10175=VECTOR('',#112155,1000.) ;
#10176=VECTOR('',#112160,1000.) ;
#10177=VECTOR('',#112161,1000.) ;
#10178=VECTOR('',#112166,1000.) ;
#10179=VECTOR('',#112169,1000.) ;
#10180=VECTOR('',#112170,1000.) ;
#10181=VECTOR('',#112171,1000.) ;
#10182=VECTOR('',#112174,1000.) ;
#10183=VECTOR('',#112175,1000.) ;
#10184=VECTOR('',#112176,1000.) ;
#10185=VECTOR('',#112179,1000.) ;
#10186=VECTOR('',#112182,1000.) ;
#10187=VECTOR('',#112183,1000.) ;
#10188=VECTOR('',#112184,1000.) ;
#10189=VECTOR('',#112185,1000.) ;
#10190=VECTOR('',#112186,1000.) ;
#10191=VECTOR('',#112189,1000.) ;
#10192=VECTOR('',#112192,1000.) ;
#10193=VECTOR('',#112197,1000.) ;
#10194=VECTOR('',#112198,1000.) ;
#10195=VECTOR('',#112199,1000.) ;
#10196=VECTOR('',#112204,1000.) ;
#10197=VECTOR('',#112209,1000.) ;
#10198=VECTOR('',#112210,1000.) ;
#10199=VECTOR('',#112211,1000.) ;
#10200=VECTOR('',#112216,1000.) ;
#10201=VECTOR('',#112221,1000.) ;
#10202=VECTOR('',#112222,1000.) ;
#10203=VECTOR('',#112223,1000.) ;
#10204=VECTOR('',#112226,1000.) ;
#10205=VECTOR('',#112231,1000.) ;
#10206=VECTOR('',#112232,1000.) ;
#10207=VECTOR('',#112235,1000.) ;
#10208=VECTOR('',#112236,1000.) ;
#10209=VECTOR('',#112237,1000.) ;
#10210=VECTOR('',#112242,1000.) ;
#10211=VECTOR('',#112247,1000.) ;
#10212=VECTOR('',#112248,1000.) ;
#10213=VECTOR('',#112249,1000.) ;
#10214=VECTOR('',#112254,1000.) ;
#10215=VECTOR('',#112259,1000.) ;
#10216=VECTOR('',#112260,1000.) ;
#10217=VECTOR('',#112261,1000.) ;
#10218=VECTOR('',#112266,1000.) ;
#10219=VECTOR('',#112271,1000.) ;
#10220=VECTOR('',#112272,1000.) ;
#10221=VECTOR('',#112273,1000.) ;
#10222=VECTOR('',#112278,1000.) ;
#10223=VECTOR('',#112283,1000.) ;
#10224=VECTOR('',#112284,1000.) ;
#10225=VECTOR('',#112285,1000.) ;
#10226=VECTOR('',#112290,1000.) ;
#10227=VECTOR('',#112295,1000.) ;
#10228=VECTOR('',#112296,1000.) ;
#10229=VECTOR('',#112297,1000.) ;
#10230=VECTOR('',#112302,1000.) ;
#10231=VECTOR('',#112309,1000.) ;
#10232=VECTOR('',#112316,1000.) ;
#10233=VECTOR('',#112321,1000.) ;
#10234=VECTOR('',#112322,1000.) ;
#10235=VECTOR('',#112323,1000.) ;
#10236=VECTOR('',#112328,1000.) ;
#10237=VECTOR('',#112333,1000.) ;
#10238=VECTOR('',#112334,1000.) ;
#10239=VECTOR('',#112335,1000.) ;
#10240=VECTOR('',#112340,1000.) ;
#10241=VECTOR('',#112345,1000.) ;
#10242=VECTOR('',#112346,1000.) ;
#10243=VECTOR('',#112351,1000.) ;
#10244=VECTOR('',#112354,1000.) ;
#10245=VECTOR('',#112355,1000.) ;
#10246=VECTOR('',#112356,1000.) ;
#10247=VECTOR('',#112359,1000.) ;
#10248=VECTOR('',#112360,1000.) ;
#10249=VECTOR('',#112361,1000.) ;
#10250=VECTOR('',#112364,1000.) ;
#10251=VECTOR('',#112367,1000.) ;
#10252=VECTOR('',#112368,1000.) ;
#10253=VECTOR('',#112369,1000.) ;
#10254=VECTOR('',#112370,1000.) ;
#10255=VECTOR('',#112371,1000.) ;
#10256=VECTOR('',#112374,1000.) ;
#10257=VECTOR('',#112377,1000.) ;
#10258=VECTOR('',#112382,1000.) ;
#10259=VECTOR('',#112383,1000.) ;
#10260=VECTOR('',#112384,1000.) ;
#10261=VECTOR('',#112389,1000.) ;
#10262=VECTOR('',#112394,1000.) ;
#10263=VECTOR('',#112395,1000.) ;
#10264=VECTOR('',#112396,1000.) ;
#10265=VECTOR('',#112401,1000.) ;
#10266=VECTOR('',#112406,1000.) ;
#10267=VECTOR('',#112407,1000.) ;
#10268=VECTOR('',#112408,1000.) ;
#10269=VECTOR('',#112411,1000.) ;
#10270=VECTOR('',#112416,1000.) ;
#10271=VECTOR('',#112417,1000.) ;
#10272=VECTOR('',#112420,1000.) ;
#10273=VECTOR('',#112421,1000.) ;
#10274=VECTOR('',#112422,1000.) ;
#10275=VECTOR('',#112427,1000.) ;
#10276=VECTOR('',#112432,1000.) ;
#10277=VECTOR('',#112433,1000.) ;
#10278=VECTOR('',#112434,1000.) ;
#10279=VECTOR('',#112439,1000.) ;
#10280=VECTOR('',#112444,1000.) ;
#10281=VECTOR('',#112445,1000.) ;
#10282=VECTOR('',#112446,1000.) ;
#10283=VECTOR('',#112451,1000.) ;
#10284=VECTOR('',#112456,1000.) ;
#10285=VECTOR('',#112457,1000.) ;
#10286=VECTOR('',#112458,1000.) ;
#10287=VECTOR('',#112463,1000.) ;
#10288=VECTOR('',#112468,1000.) ;
#10289=VECTOR('',#112469,1000.) ;
#10290=VECTOR('',#112470,1000.) ;
#10291=VECTOR('',#112475,1000.) ;
#10292=VECTOR('',#112480,1000.) ;
#10293=VECTOR('',#112481,1000.) ;
#10294=VECTOR('',#112482,1000.) ;
#10295=VECTOR('',#112487,1000.) ;
#10296=VECTOR('',#112494,1000.) ;
#10297=VECTOR('',#112501,1000.) ;
#10298=VECTOR('',#112506,1000.) ;
#10299=VECTOR('',#112507,1000.) ;
#10300=VECTOR('',#112508,1000.) ;
#10301=VECTOR('',#112513,1000.) ;
#10302=VECTOR('',#112518,1000.) ;
#10303=VECTOR('',#112519,1000.) ;
#10304=VECTOR('',#112520,1000.) ;
#10305=VECTOR('',#112525,1000.) ;
#10306=VECTOR('',#112530,1000.) ;
#10307=VECTOR('',#112531,1000.) ;
#10308=VECTOR('',#112536,1000.) ;
#10309=VECTOR('',#112539,1000.) ;
#10310=VECTOR('',#112540,1000.) ;
#10311=VECTOR('',#112541,1000.) ;
#10312=VECTOR('',#112544,1000.) ;
#10313=VECTOR('',#112545,1000.) ;
#10314=VECTOR('',#112546,1000.) ;
#10315=VECTOR('',#112549,1000.) ;
#10316=VECTOR('',#112552,1000.) ;
#10317=VECTOR('',#112553,1000.) ;
#10318=VECTOR('',#112554,1000.) ;
#10319=VECTOR('',#112555,1000.) ;
#10320=VECTOR('',#112556,1000.) ;
#10321=VECTOR('',#112559,1000.) ;
#10322=VECTOR('',#112562,1000.) ;
#10323=VECTOR('',#112567,1000.) ;
#10324=VECTOR('',#112568,1000.) ;
#10325=VECTOR('',#112569,1000.) ;
#10326=VECTOR('',#112574,1000.) ;
#10327=VECTOR('',#112579,1000.) ;
#10328=VECTOR('',#112580,1000.) ;
#10329=VECTOR('',#112581,1000.) ;
#10330=VECTOR('',#112586,1000.) ;
#10331=VECTOR('',#112591,1000.) ;
#10332=VECTOR('',#112592,1000.) ;
#10333=VECTOR('',#112593,1000.) ;
#10334=VECTOR('',#112596,1000.) ;
#10335=VECTOR('',#112601,1000.) ;
#10336=VECTOR('',#112602,1000.) ;
#10337=VECTOR('',#112605,1000.) ;
#10338=VECTOR('',#112606,1000.) ;
#10339=VECTOR('',#112607,1000.) ;
#10340=VECTOR('',#112612,1000.) ;
#10341=VECTOR('',#112617,1000.) ;
#10342=VECTOR('',#112618,1000.) ;
#10343=VECTOR('',#112619,1000.) ;
#10344=VECTOR('',#112624,1000.) ;
#10345=VECTOR('',#112629,1000.) ;
#10346=VECTOR('',#112630,1000.) ;
#10347=VECTOR('',#112631,1000.) ;
#10348=VECTOR('',#112636,1000.) ;
#10349=VECTOR('',#112641,1000.) ;
#10350=VECTOR('',#112642,1000.) ;
#10351=VECTOR('',#112643,1000.) ;
#10352=VECTOR('',#112648,1000.) ;
#10353=VECTOR('',#112653,1000.) ;
#10354=VECTOR('',#112654,1000.) ;
#10355=VECTOR('',#112655,1000.) ;
#10356=VECTOR('',#112660,1000.) ;
#10357=VECTOR('',#112665,1000.) ;
#10358=VECTOR('',#112666,1000.) ;
#10359=VECTOR('',#112667,1000.) ;
#10360=VECTOR('',#112672,1000.) ;
#10361=VECTOR('',#112679,1000.) ;
#10362=VECTOR('',#112686,1000.) ;
#10363=VECTOR('',#112691,1000.) ;
#10364=VECTOR('',#112692,1000.) ;
#10365=VECTOR('',#112693,1000.) ;
#10366=VECTOR('',#112698,1000.) ;
#10367=VECTOR('',#112703,1000.) ;
#10368=VECTOR('',#112704,1000.) ;
#10369=VECTOR('',#112705,1000.) ;
#10370=VECTOR('',#112710,1000.) ;
#10371=VECTOR('',#112715,1000.) ;
#10372=VECTOR('',#112716,1000.) ;
#10373=VECTOR('',#112721,1000.) ;
#10374=VECTOR('',#112724,1000.) ;
#10375=VECTOR('',#112725,1000.) ;
#10376=VECTOR('',#112726,1000.) ;
#10377=VECTOR('',#112729,1000.) ;
#10378=VECTOR('',#112730,1000.) ;
#10379=VECTOR('',#112731,1000.) ;
#10380=VECTOR('',#112734,1000.) ;
#10381=VECTOR('',#112737,1000.) ;
#10382=VECTOR('',#112738,1000.) ;
#10383=VECTOR('',#112739,1000.) ;
#10384=VECTOR('',#112740,1000.) ;
#10385=VECTOR('',#112741,1000.) ;
#10386=VECTOR('',#112744,1000.) ;
#10387=VECTOR('',#112747,1000.) ;
#10388=VECTOR('',#112752,1000.) ;
#10389=VECTOR('',#112753,1000.) ;
#10390=VECTOR('',#112754,1000.) ;
#10391=VECTOR('',#112759,1000.) ;
#10392=VECTOR('',#112764,1000.) ;
#10393=VECTOR('',#112765,1000.) ;
#10394=VECTOR('',#112766,1000.) ;
#10395=VECTOR('',#112771,1000.) ;
#10396=VECTOR('',#112776,1000.) ;
#10397=VECTOR('',#112777,1000.) ;
#10398=VECTOR('',#112778,1000.) ;
#10399=VECTOR('',#112781,1000.) ;
#10400=VECTOR('',#112786,1000.) ;
#10401=VECTOR('',#112787,1000.) ;
#10402=VECTOR('',#112790,1000.) ;
#10403=VECTOR('',#112791,1000.) ;
#10404=VECTOR('',#112792,1000.) ;
#10405=VECTOR('',#112797,1000.) ;
#10406=VECTOR('',#112802,1000.) ;
#10407=VECTOR('',#112803,1000.) ;
#10408=VECTOR('',#112804,1000.) ;
#10409=VECTOR('',#112809,1000.) ;
#10410=VECTOR('',#112814,1000.) ;
#10411=VECTOR('',#112815,1000.) ;
#10412=VECTOR('',#112816,1000.) ;
#10413=VECTOR('',#112821,1000.) ;
#10414=VECTOR('',#112826,1000.) ;
#10415=VECTOR('',#112827,1000.) ;
#10416=VECTOR('',#112828,1000.) ;
#10417=VECTOR('',#112833,1000.) ;
#10418=VECTOR('',#112838,1000.) ;
#10419=VECTOR('',#112839,1000.) ;
#10420=VECTOR('',#112840,1000.) ;
#10421=VECTOR('',#112845,1000.) ;
#10422=VECTOR('',#112850,1000.) ;
#10423=VECTOR('',#112851,1000.) ;
#10424=VECTOR('',#112852,1000.) ;
#10425=VECTOR('',#112857,1000.) ;
#10426=VECTOR('',#112864,1000.) ;
#10427=VECTOR('',#112871,1000.) ;
#10428=VECTOR('',#112876,1000.) ;
#10429=VECTOR('',#112877,1000.) ;
#10430=VECTOR('',#112878,1000.) ;
#10431=VECTOR('',#112883,1000.) ;
#10432=VECTOR('',#112888,1000.) ;
#10433=VECTOR('',#112889,1000.) ;
#10434=VECTOR('',#112890,1000.) ;
#10435=VECTOR('',#112895,1000.) ;
#10436=VECTOR('',#112900,1000.) ;
#10437=VECTOR('',#112901,1000.) ;
#10438=VECTOR('',#112906,1000.) ;
#10439=VECTOR('',#112909,1000.) ;
#10440=VECTOR('',#112910,1000.) ;
#10441=VECTOR('',#112911,1000.) ;
#10442=VECTOR('',#112914,1000.) ;
#10443=VECTOR('',#112915,1000.) ;
#10444=VECTOR('',#112916,1000.) ;
#10445=VECTOR('',#112919,1000.) ;
#10446=VECTOR('',#112922,1000.) ;
#10447=VECTOR('',#112923,1000.) ;
#10448=VECTOR('',#112924,1000.) ;
#10449=VECTOR('',#112925,1000.) ;
#10450=VECTOR('',#112926,1000.) ;
#10451=VECTOR('',#112929,1000.) ;
#10452=VECTOR('',#112932,1000.) ;
#10453=VECTOR('',#112937,1000.) ;
#10454=VECTOR('',#112938,1000.) ;
#10455=VECTOR('',#112939,1000.) ;
#10456=VECTOR('',#112944,1000.) ;
#10457=VECTOR('',#112949,1000.) ;
#10458=VECTOR('',#112950,1000.) ;
#10459=VECTOR('',#112951,1000.) ;
#10460=VECTOR('',#112956,1000.) ;
#10461=VECTOR('',#112961,1000.) ;
#10462=VECTOR('',#112962,1000.) ;
#10463=VECTOR('',#112963,1000.) ;
#10464=VECTOR('',#112966,1000.) ;
#10465=VECTOR('',#112971,1000.) ;
#10466=VECTOR('',#112972,1000.) ;
#10467=VECTOR('',#112975,1000.) ;
#10468=VECTOR('',#112976,1000.) ;
#10469=VECTOR('',#112977,1000.) ;
#10470=VECTOR('',#112982,1000.) ;
#10471=VECTOR('',#112987,1000.) ;
#10472=VECTOR('',#112988,1000.) ;
#10473=VECTOR('',#112989,1000.) ;
#10474=VECTOR('',#112994,1000.) ;
#10475=VECTOR('',#112999,1000.) ;
#10476=VECTOR('',#113000,1000.) ;
#10477=VECTOR('',#113001,1000.) ;
#10478=VECTOR('',#113006,1000.) ;
#10479=VECTOR('',#113011,1000.) ;
#10480=VECTOR('',#113012,1000.) ;
#10481=VECTOR('',#113013,1000.) ;
#10482=VECTOR('',#113018,1000.) ;
#10483=VECTOR('',#113023,1000.) ;
#10484=VECTOR('',#113024,1000.) ;
#10485=VECTOR('',#113025,1000.) ;
#10486=VECTOR('',#113030,1000.) ;
#10487=VECTOR('',#113035,1000.) ;
#10488=VECTOR('',#113036,1000.) ;
#10489=VECTOR('',#113037,1000.) ;
#10490=VECTOR('',#113042,1000.) ;
#10491=VECTOR('',#113049,1000.) ;
#10492=VECTOR('',#113056,1000.) ;
#10493=VECTOR('',#113061,1000.) ;
#10494=VECTOR('',#113062,1000.) ;
#10495=VECTOR('',#113063,1000.) ;
#10496=VECTOR('',#113068,1000.) ;
#10497=VECTOR('',#113073,1000.) ;
#10498=VECTOR('',#113074,1000.) ;
#10499=VECTOR('',#113075,1000.) ;
#10500=VECTOR('',#113080,1000.) ;
#10501=VECTOR('',#113085,1000.) ;
#10502=VECTOR('',#113086,1000.) ;
#10503=VECTOR('',#113091,1000.) ;
#10504=VECTOR('',#113094,1000.) ;
#10505=VECTOR('',#113095,1000.) ;
#10506=VECTOR('',#113096,1000.) ;
#10507=VECTOR('',#113099,1000.) ;
#10508=VECTOR('',#113100,1000.) ;
#10509=VECTOR('',#113101,1000.) ;
#10510=VECTOR('',#113104,1000.) ;
#10511=VECTOR('',#113107,1000.) ;
#10512=VECTOR('',#113108,1000.) ;
#10513=VECTOR('',#113109,1000.) ;
#10514=VECTOR('',#113110,1000.) ;
#10515=VECTOR('',#113111,1000.) ;
#10516=VECTOR('',#113114,1000.) ;
#10517=VECTOR('',#113117,1000.) ;
#10518=VECTOR('',#113122,1000.) ;
#10519=VECTOR('',#113123,1000.) ;
#10520=VECTOR('',#113124,1000.) ;
#10521=VECTOR('',#113129,1000.) ;
#10522=VECTOR('',#113134,1000.) ;
#10523=VECTOR('',#113135,1000.) ;
#10524=VECTOR('',#113136,1000.) ;
#10525=VECTOR('',#113141,1000.) ;
#10526=VECTOR('',#113146,1000.) ;
#10527=VECTOR('',#113147,1000.) ;
#10528=VECTOR('',#113148,1000.) ;
#10529=VECTOR('',#113151,1000.) ;
#10530=VECTOR('',#113156,1000.) ;
#10531=VECTOR('',#113157,1000.) ;
#10532=VECTOR('',#113160,1000.) ;
#10533=VECTOR('',#113161,1000.) ;
#10534=VECTOR('',#113162,1000.) ;
#10535=VECTOR('',#113167,1000.) ;
#10536=VECTOR('',#113172,1000.) ;
#10537=VECTOR('',#113173,1000.) ;
#10538=VECTOR('',#113174,1000.) ;
#10539=VECTOR('',#113179,1000.) ;
#10540=VECTOR('',#113184,1000.) ;
#10541=VECTOR('',#113185,1000.) ;
#10542=VECTOR('',#113186,1000.) ;
#10543=VECTOR('',#113191,1000.) ;
#10544=VECTOR('',#113196,1000.) ;
#10545=VECTOR('',#113197,1000.) ;
#10546=VECTOR('',#113198,1000.) ;
#10547=VECTOR('',#113203,1000.) ;
#10548=VECTOR('',#113208,1000.) ;
#10549=VECTOR('',#113209,1000.) ;
#10550=VECTOR('',#113210,1000.) ;
#10551=VECTOR('',#113215,1000.) ;
#10552=VECTOR('',#113220,1000.) ;
#10553=VECTOR('',#113221,1000.) ;
#10554=VECTOR('',#113222,1000.) ;
#10555=VECTOR('',#113227,1000.) ;
#10556=VECTOR('',#113234,1000.) ;
#10557=VECTOR('',#113241,1000.) ;
#10558=VECTOR('',#113246,1000.) ;
#10559=VECTOR('',#113247,1000.) ;
#10560=VECTOR('',#113248,1000.) ;
#10561=VECTOR('',#113253,1000.) ;
#10562=VECTOR('',#113258,1000.) ;
#10563=VECTOR('',#113259,1000.) ;
#10564=VECTOR('',#113260,1000.) ;
#10565=VECTOR('',#113265,1000.) ;
#10566=VECTOR('',#113270,1000.) ;
#10567=VECTOR('',#113271,1000.) ;
#10568=VECTOR('',#113276,1000.) ;
#10569=VECTOR('',#113279,1000.) ;
#10570=VECTOR('',#113280,1000.) ;
#10571=VECTOR('',#113281,1000.) ;
#10572=VECTOR('',#113284,1000.) ;
#10573=VECTOR('',#113285,1000.) ;
#10574=VECTOR('',#113286,1000.) ;
#10575=VECTOR('',#113289,1000.) ;
#10576=VECTOR('',#113292,1000.) ;
#10577=VECTOR('',#113293,1000.) ;
#10578=VECTOR('',#113294,1000.) ;
#10579=VECTOR('',#113295,1000.) ;
#10580=VECTOR('',#113296,1000.) ;
#10581=VECTOR('',#113299,1000.) ;
#10582=VECTOR('',#113302,1000.) ;
#10583=VECTOR('',#113307,1000.) ;
#10584=VECTOR('',#113308,1000.) ;
#10585=VECTOR('',#113309,1000.) ;
#10586=VECTOR('',#113314,1000.) ;
#10587=VECTOR('',#113319,1000.) ;
#10588=VECTOR('',#113320,1000.) ;
#10589=VECTOR('',#113321,1000.) ;
#10590=VECTOR('',#113326,1000.) ;
#10591=VECTOR('',#113331,1000.) ;
#10592=VECTOR('',#113332,1000.) ;
#10593=VECTOR('',#113333,1000.) ;
#10594=VECTOR('',#113336,1000.) ;
#10595=VECTOR('',#113341,1000.) ;
#10596=VECTOR('',#113342,1000.) ;
#10597=VECTOR('',#113345,1000.) ;
#10598=VECTOR('',#113346,1000.) ;
#10599=VECTOR('',#113347,1000.) ;
#10600=VECTOR('',#113352,1000.) ;
#10601=VECTOR('',#113357,1000.) ;
#10602=VECTOR('',#113358,1000.) ;
#10603=VECTOR('',#113359,1000.) ;
#10604=VECTOR('',#113364,1000.) ;
#10605=VECTOR('',#113369,1000.) ;
#10606=VECTOR('',#113370,1000.) ;
#10607=VECTOR('',#113371,1000.) ;
#10608=VECTOR('',#113376,1000.) ;
#10609=VECTOR('',#113381,1000.) ;
#10610=VECTOR('',#113382,1000.) ;
#10611=VECTOR('',#113383,1000.) ;
#10612=VECTOR('',#113388,1000.) ;
#10613=VECTOR('',#113393,1000.) ;
#10614=VECTOR('',#113394,1000.) ;
#10615=VECTOR('',#113395,1000.) ;
#10616=VECTOR('',#113400,1000.) ;
#10617=VECTOR('',#113405,1000.) ;
#10618=VECTOR('',#113406,1000.) ;
#10619=VECTOR('',#113407,1000.) ;
#10620=VECTOR('',#113412,1000.) ;
#10621=VECTOR('',#113419,1000.) ;
#10622=VECTOR('',#113426,1000.) ;
#10623=VECTOR('',#113431,1000.) ;
#10624=VECTOR('',#113432,1000.) ;
#10625=VECTOR('',#113433,1000.) ;
#10626=VECTOR('',#113438,1000.) ;
#10627=VECTOR('',#113443,1000.) ;
#10628=VECTOR('',#113444,1000.) ;
#10629=VECTOR('',#113445,1000.) ;
#10630=VECTOR('',#113450,1000.) ;
#10631=VECTOR('',#113455,1000.) ;
#10632=VECTOR('',#113456,1000.) ;
#10633=VECTOR('',#113461,1000.) ;
#10634=VECTOR('',#113464,1000.) ;
#10635=VECTOR('',#113465,1000.) ;
#10636=VECTOR('',#113466,1000.) ;
#10637=VECTOR('',#113469,1000.) ;
#10638=VECTOR('',#113470,1000.) ;
#10639=VECTOR('',#113471,1000.) ;
#10640=VECTOR('',#113474,1000.) ;
#10641=VECTOR('',#113477,1000.) ;
#10642=VECTOR('',#113478,1000.) ;
#10643=VECTOR('',#113479,1000.) ;
#10644=VECTOR('',#113480,1000.) ;
#10645=VECTOR('',#113481,1000.) ;
#10646=VECTOR('',#113484,1000.) ;
#10647=VECTOR('',#113487,1000.) ;
#10648=VECTOR('',#113490,1000.) ;
#10649=VECTOR('',#113493,1000.) ;
#10650=VECTOR('',#113498,1000.) ;
#10651=VECTOR('',#113501,1000.) ;
#10652=VECTOR('',#113504,1000.) ;
#10653=VECTOR('',#113507,1000.) ;
#10654=VECTOR('',#113512,1000.) ;
#10655=VECTOR('',#113515,1000.) ;
#10656=VECTOR('',#113518,1000.) ;
#10657=VECTOR('',#113521,1000.) ;
#10658=VECTOR('',#113526,1000.) ;
#10659=VECTOR('',#113529,1000.) ;
#10660=VECTOR('',#113532,1000.) ;
#10661=VECTOR('',#113535,1000.) ;
#10662=VECTOR('',#113540,1000.) ;
#10663=VECTOR('',#113543,1000.) ;
#10664=VECTOR('',#113546,1000.) ;
#10665=VECTOR('',#113549,1000.) ;
#10666=VECTOR('',#113554,1000.) ;
#10667=VECTOR('',#113557,1000.) ;
#10668=VECTOR('',#113560,1000.) ;
#10669=VECTOR('',#113563,1000.) ;
#10670=VECTOR('',#113568,1000.) ;
#10671=VECTOR('',#113571,1000.) ;
#10672=VECTOR('',#113574,1000.) ;
#10673=VECTOR('',#113577,1000.) ;
#10674=VECTOR('',#113582,1000.) ;
#10675=VECTOR('',#113585,1000.) ;
#10676=VECTOR('',#113588,1000.) ;
#10677=VECTOR('',#113591,1000.) ;
#10678=VECTOR('',#113596,1000.) ;
#10679=VECTOR('',#113599,1000.) ;
#10680=VECTOR('',#113602,1000.) ;
#10681=VECTOR('',#113605,1000.) ;
#10682=VECTOR('',#113640,1000.) ;
#10683=VECTOR('',#113643,1000.) ;
#10684=VECTOR('',#113690,1000.) ;
#10685=VECTOR('',#113749,1000.) ;
#10686=VECTOR('',#113798,1000.) ;
#10687=VECTOR('',#114905,1000.) ;
#10688=VECTOR('',#114908,1000.) ;
#10689=VECTOR('',#114955,1000.) ;
#10690=VECTOR('',#115014,1000.) ;
#10691=VECTOR('',#115063,1000.) ;
#10692=VECTOR('',#115216,1000.) ;
#10693=VECTOR('',#115219,1000.) ;
#10694=VECTOR('',#115266,1000.) ;
#10695=VECTOR('',#115325,1000.) ;
#10696=VECTOR('',#115374,1000.) ;
#10697=VECTOR('',#115527,1000.) ;
#10698=VECTOR('',#115530,1000.) ;
#10699=VECTOR('',#115577,1000.) ;
#10700=VECTOR('',#115636,1000.) ;
#10701=VECTOR('',#115685,1000.) ;
#10702=VECTOR('',#115838,1000.) ;
#10703=VECTOR('',#115841,1000.) ;
#10704=VECTOR('',#115888,1000.) ;
#10705=VECTOR('',#115947,1000.) ;
#10706=VECTOR('',#115996,1000.) ;
#10707=VECTOR('',#116149,1000.) ;
#10708=VECTOR('',#116152,1000.) ;
#10709=VECTOR('',#116199,1000.) ;
#10710=VECTOR('',#116258,1000.) ;
#10711=VECTOR('',#116307,1000.) ;
#10712=VECTOR('',#116460,1000.) ;
#10713=VECTOR('',#116463,1000.) ;
#10714=VECTOR('',#116510,1000.) ;
#10715=VECTOR('',#116569,1000.) ;
#10716=VECTOR('',#116618,1000.) ;
#10717=VECTOR('',#116771,1000.) ;
#10718=VECTOR('',#116774,1000.) ;
#10719=VECTOR('',#116821,1000.) ;
#10720=VECTOR('',#116880,1000.) ;
#10721=VECTOR('',#116929,1000.) ;
#10722=VECTOR('',#117082,1000.) ;
#10723=VECTOR('',#117085,1000.) ;
#10724=VECTOR('',#117132,1000.) ;
#10725=VECTOR('',#117191,1000.) ;
#10726=VECTOR('',#117240,1000.) ;
#10727=VECTOR('',#117363,1000.) ;
#10728=VECTOR('',#117364,1000.) ;
#10729=VECTOR('',#117365,1000.) ;
#10730=VECTOR('',#117366,1000.) ;
#10731=VECTOR('',#117369,1000.) ;
#10732=VECTOR('',#117370,1000.) ;
#10733=VECTOR('',#117371,1000.) ;
#10734=VECTOR('',#117372,1000.) ;
#10735=VECTOR('',#117375,1000.) ;
#10736=VECTOR('',#117376,1000.) ;
#10737=VECTOR('',#117377,1000.) ;
#10738=VECTOR('',#117378,1000.) ;
#10739=VECTOR('',#117381,1000.) ;
#10740=VECTOR('',#117382,1000.) ;
#10741=VECTOR('',#117383,1000.) ;
#10742=VECTOR('',#117384,1000.) ;
#10743=VECTOR('',#117387,1000.) ;
#10744=VECTOR('',#117388,1000.) ;
#10745=VECTOR('',#117389,1000.) ;
#10746=VECTOR('',#117390,1000.) ;
#10747=VECTOR('',#117393,1000.) ;
#10748=VECTOR('',#117398,1000.) ;
#10749=VECTOR('',#117399,1000.) ;
#10750=VECTOR('',#117402,1000.) ;
#10751=VECTOR('',#117407,1000.) ;
#10752=VECTOR('',#117408,1000.) ;
#10753=VECTOR('',#117423,1000.) ;
#10754=VECTOR('',#117424,1000.) ;
#10755=VECTOR('',#117425,1000.) ;
#10756=VECTOR('',#117426,1000.) ;
#10757=VECTOR('',#117429,1000.) ;
#10758=VECTOR('',#117430,1000.) ;
#10759=VECTOR('',#117431,1000.) ;
#10760=VECTOR('',#117434,1000.) ;
#10761=VECTOR('',#117435,1000.) ;
#10762=VECTOR('',#117436,1000.) ;
#10763=VECTOR('',#117439,1000.) ;
#10764=VECTOR('',#117440,1000.) ;
#10765=VECTOR('',#117441,1000.) ;
#10766=VECTOR('',#117442,1000.) ;
#10767=VECTOR('',#117445,1000.) ;
#10768=VECTOR('',#117446,1000.) ;
#10769=VECTOR('',#117447,1000.) ;
#10770=VECTOR('',#117448,1000.) ;
#10771=VECTOR('',#117451,1000.) ;
#10772=VECTOR('',#117452,1000.) ;
#10773=VECTOR('',#117453,1000.) ;
#10774=VECTOR('',#117456,1000.) ;
#10775=VECTOR('',#117457,1000.) ;
#10776=VECTOR('',#117458,1000.) ;
#10777=VECTOR('',#117461,1000.) ;
#10778=VECTOR('',#117462,1000.) ;
#10779=VECTOR('',#117463,1000.) ;
#10780=VECTOR('',#117464,1000.) ;
#10781=VECTOR('',#117467,1000.) ;
#10782=VECTOR('',#117468,1000.) ;
#10783=VECTOR('',#117469,1000.) ;
#10784=VECTOR('',#117470,1000.) ;
#10785=VECTOR('',#117473,1000.) ;
#10786=VECTOR('',#117474,1000.) ;
#10787=VECTOR('',#117475,1000.) ;
#10788=VECTOR('',#117476,1000.) ;
#10789=VECTOR('',#117479,1000.) ;
#10790=VECTOR('',#117480,1000.) ;
#10791=VECTOR('',#117481,1000.) ;
#10792=VECTOR('',#117482,1000.) ;
#10793=VECTOR('',#117485,1000.) ;
#10794=VECTOR('',#117486,1000.) ;
#10795=VECTOR('',#117487,1000.) ;
#10796=VECTOR('',#117488,1000.) ;
#10797=VECTOR('',#117491,1000.) ;
#10798=VECTOR('',#117496,1000.) ;
#10799=VECTOR('',#117497,1000.) ;
#10800=VECTOR('',#117500,1000.) ;
#10801=VECTOR('',#117505,1000.) ;
#10802=VECTOR('',#117506,1000.) ;
#10803=VECTOR('',#117521,1000.) ;
#10804=VECTOR('',#117522,1000.) ;
#10805=VECTOR('',#117523,1000.) ;
#10806=VECTOR('',#117524,1000.) ;
#10807=VECTOR('',#117527,1000.) ;
#10808=VECTOR('',#117528,1000.) ;
#10809=VECTOR('',#117529,1000.) ;
#10810=VECTOR('',#117532,1000.) ;
#10811=VECTOR('',#117533,1000.) ;
#10812=VECTOR('',#117534,1000.) ;
#10813=VECTOR('',#117537,1000.) ;
#10814=VECTOR('',#117538,1000.) ;
#10815=VECTOR('',#117539,1000.) ;
#10816=VECTOR('',#117540,1000.) ;
#10817=VECTOR('',#117543,1000.) ;
#10818=VECTOR('',#117544,1000.) ;
#10819=VECTOR('',#117545,1000.) ;
#10820=VECTOR('',#117546,1000.) ;
#10821=VECTOR('',#117549,1000.) ;
#10822=VECTOR('',#117550,1000.) ;
#10823=VECTOR('',#117551,1000.) ;
#10824=VECTOR('',#117554,1000.) ;
#10825=VECTOR('',#117555,1000.) ;
#10826=VECTOR('',#117556,1000.) ;
#10827=VECTOR('',#117559,1000.) ;
#10828=VECTOR('',#117560,1000.) ;
#10829=VECTOR('',#117561,1000.) ;
#10830=VECTOR('',#117562,1000.) ;
#10831=VECTOR('',#117565,1000.) ;
#10832=VECTOR('',#117566,1000.) ;
#10833=VECTOR('',#117567,1000.) ;
#10834=VECTOR('',#117568,1000.) ;
#10835=VECTOR('',#117571,1000.) ;
#10836=VECTOR('',#117572,1000.) ;
#10837=VECTOR('',#117573,1000.) ;
#10838=VECTOR('',#117574,1000.) ;
#10839=VECTOR('',#117577,1000.) ;
#10840=VECTOR('',#117578,1000.) ;
#10841=VECTOR('',#117579,1000.) ;
#10842=VECTOR('',#117580,1000.) ;
#10843=VECTOR('',#117583,1000.) ;
#10844=VECTOR('',#117584,1000.) ;
#10845=VECTOR('',#117585,1000.) ;
#10846=VECTOR('',#117586,1000.) ;
#10847=VECTOR('',#117589,1000.) ;
#10848=VECTOR('',#117594,1000.) ;
#10849=VECTOR('',#117595,1000.) ;
#10850=VECTOR('',#117598,1000.) ;
#10851=VECTOR('',#117603,1000.) ;
#10852=VECTOR('',#117604,1000.) ;
#10853=VECTOR('',#117619,1000.) ;
#10854=VECTOR('',#117620,1000.) ;
#10855=VECTOR('',#117621,1000.) ;
#10856=VECTOR('',#117622,1000.) ;
#10857=VECTOR('',#117625,1000.) ;
#10858=VECTOR('',#117626,1000.) ;
#10859=VECTOR('',#117627,1000.) ;
#10860=VECTOR('',#117630,1000.) ;
#10861=VECTOR('',#117631,1000.) ;
#10862=VECTOR('',#117632,1000.) ;
#10863=VECTOR('',#117635,1000.) ;
#10864=VECTOR('',#117636,1000.) ;
#10865=VECTOR('',#117637,1000.) ;
#10866=VECTOR('',#117638,1000.) ;
#10867=VECTOR('',#117641,1000.) ;
#10868=VECTOR('',#117642,1000.) ;
#10869=VECTOR('',#117643,1000.) ;
#10870=VECTOR('',#117644,1000.) ;
#10871=VECTOR('',#117647,1000.) ;
#10872=VECTOR('',#117648,1000.) ;
#10873=VECTOR('',#117649,1000.) ;
#10874=VECTOR('',#117652,1000.) ;
#10875=VECTOR('',#117653,1000.) ;
#10876=VECTOR('',#117654,1000.) ;
#10877=VECTOR('',#117657,1000.) ;
#10878=VECTOR('',#117658,1000.) ;
#10879=VECTOR('',#117659,1000.) ;
#10880=VECTOR('',#117660,1000.) ;
#10881=VECTOR('',#117663,1000.) ;
#10882=VECTOR('',#117664,1000.) ;
#10883=VECTOR('',#117665,1000.) ;
#10884=VECTOR('',#117666,1000.) ;
#10885=VECTOR('',#117669,1000.) ;
#10886=VECTOR('',#117670,1000.) ;
#10887=VECTOR('',#117671,1000.) ;
#10888=VECTOR('',#117672,1000.) ;
#10889=VECTOR('',#117675,1000.) ;
#10890=VECTOR('',#117676,1000.) ;
#10891=VECTOR('',#117677,1000.) ;
#10892=VECTOR('',#117678,1000.) ;
#10893=VECTOR('',#117681,1000.) ;
#10894=VECTOR('',#117682,1000.) ;
#10895=VECTOR('',#117683,1000.) ;
#10896=VECTOR('',#117684,1000.) ;
#10897=VECTOR('',#117687,1000.) ;
#10898=VECTOR('',#117692,1000.) ;
#10899=VECTOR('',#117693,1000.) ;
#10900=VECTOR('',#117696,1000.) ;
#10901=VECTOR('',#117701,1000.) ;
#10902=VECTOR('',#117702,1000.) ;
#10903=VECTOR('',#117717,1000.) ;
#10904=VECTOR('',#117718,1000.) ;
#10905=VECTOR('',#117719,1000.) ;
#10906=VECTOR('',#117720,1000.) ;
#10907=VECTOR('',#117723,1000.) ;
#10908=VECTOR('',#117724,1000.) ;
#10909=VECTOR('',#117725,1000.) ;
#10910=VECTOR('',#117728,1000.) ;
#10911=VECTOR('',#117729,1000.) ;
#10912=VECTOR('',#117730,1000.) ;
#10913=VECTOR('',#117733,1000.) ;
#10914=VECTOR('',#117734,1000.) ;
#10915=VECTOR('',#117735,1000.) ;
#10916=VECTOR('',#117736,1000.) ;
#10917=VECTOR('',#117739,1000.) ;
#10918=VECTOR('',#117740,1000.) ;
#10919=VECTOR('',#117741,1000.) ;
#10920=VECTOR('',#117742,1000.) ;
#10921=VECTOR('',#117745,1000.) ;
#10922=VECTOR('',#117746,1000.) ;
#10923=VECTOR('',#117747,1000.) ;
#10924=VECTOR('',#117750,1000.) ;
#10925=VECTOR('',#117751,1000.) ;
#10926=VECTOR('',#117752,1000.) ;
#10927=VECTOR('',#117755,1000.) ;
#10928=VECTOR('',#117756,1000.) ;
#10929=VECTOR('',#117757,1000.) ;
#10930=VECTOR('',#117758,1000.) ;
#10931=VECTOR('',#117761,1000.) ;
#10932=VECTOR('',#117762,1000.) ;
#10933=VECTOR('',#117763,1000.) ;
#10934=VECTOR('',#117764,1000.) ;
#10935=VECTOR('',#117767,1000.) ;
#10936=VECTOR('',#117768,1000.) ;
#10937=VECTOR('',#117769,1000.) ;
#10938=VECTOR('',#117770,1000.) ;
#10939=VECTOR('',#117773,1000.) ;
#10940=VECTOR('',#117774,1000.) ;
#10941=VECTOR('',#117775,1000.) ;
#10942=VECTOR('',#117776,1000.) ;
#10943=VECTOR('',#117779,1000.) ;
#10944=VECTOR('',#117780,1000.) ;
#10945=VECTOR('',#117781,1000.) ;
#10946=VECTOR('',#117782,1000.) ;
#10947=VECTOR('',#117785,1000.) ;
#10948=VECTOR('',#117790,1000.) ;
#10949=VECTOR('',#117791,1000.) ;
#10950=VECTOR('',#117794,1000.) ;
#10951=VECTOR('',#117799,1000.) ;
#10952=VECTOR('',#117800,1000.) ;
#10953=VECTOR('',#117815,1000.) ;
#10954=VECTOR('',#117816,1000.) ;
#10955=VECTOR('',#117817,1000.) ;
#10956=VECTOR('',#117818,1000.) ;
#10957=VECTOR('',#117821,1000.) ;
#10958=VECTOR('',#117822,1000.) ;
#10959=VECTOR('',#117823,1000.) ;
#10960=VECTOR('',#117826,1000.) ;
#10961=VECTOR('',#117827,1000.) ;
#10962=VECTOR('',#117828,1000.) ;
#10963=VECTOR('',#117831,1000.) ;
#10964=VECTOR('',#117832,1000.) ;
#10965=VECTOR('',#117833,1000.) ;
#10966=VECTOR('',#117834,1000.) ;
#10967=VECTOR('',#117837,1000.) ;
#10968=VECTOR('',#117838,1000.) ;
#10969=VECTOR('',#117839,1000.) ;
#10970=VECTOR('',#117840,1000.) ;
#10971=VECTOR('',#117843,1000.) ;
#10972=VECTOR('',#117844,1000.) ;
#10973=VECTOR('',#117845,1000.) ;
#10974=VECTOR('',#117848,1000.) ;
#10975=VECTOR('',#117849,1000.) ;
#10976=VECTOR('',#117850,1000.) ;
#10977=VECTOR('',#117853,1000.) ;
#10978=VECTOR('',#117854,1000.) ;
#10979=VECTOR('',#117855,1000.) ;
#10980=VECTOR('',#117856,1000.) ;
#10981=VECTOR('',#117859,1000.) ;
#10982=VECTOR('',#117860,1000.) ;
#10983=VECTOR('',#117861,1000.) ;
#10984=VECTOR('',#117862,1000.) ;
#10985=VECTOR('',#117865,1000.) ;
#10986=VECTOR('',#117866,1000.) ;
#10987=VECTOR('',#117867,1000.) ;
#10988=VECTOR('',#117868,1000.) ;
#10989=VECTOR('',#117871,1000.) ;
#10990=VECTOR('',#117872,1000.) ;
#10991=VECTOR('',#117873,1000.) ;
#10992=VECTOR('',#117874,1000.) ;
#10993=VECTOR('',#117877,1000.) ;
#10994=VECTOR('',#117878,1000.) ;
#10995=VECTOR('',#117879,1000.) ;
#10996=VECTOR('',#117880,1000.) ;
#10997=VECTOR('',#117883,1000.) ;
#10998=VECTOR('',#117888,1000.) ;
#10999=VECTOR('',#117889,1000.) ;
#11000=VECTOR('',#117892,1000.) ;
#11001=VECTOR('',#117897,1000.) ;
#11002=VECTOR('',#117898,1000.) ;
#11003=VECTOR('',#117913,1000.) ;
#11004=VECTOR('',#117914,1000.) ;
#11005=VECTOR('',#117915,1000.) ;
#11006=VECTOR('',#117916,1000.) ;
#11007=VECTOR('',#117919,1000.) ;
#11008=VECTOR('',#117920,1000.) ;
#11009=VECTOR('',#117921,1000.) ;
#11010=VECTOR('',#117924,1000.) ;
#11011=VECTOR('',#117925,1000.) ;
#11012=VECTOR('',#117926,1000.) ;
#11013=VECTOR('',#117929,1000.) ;
#11014=VECTOR('',#117930,1000.) ;
#11015=VECTOR('',#117931,1000.) ;
#11016=VECTOR('',#117932,1000.) ;
#11017=VECTOR('',#117935,1000.) ;
#11018=VECTOR('',#117936,1000.) ;
#11019=VECTOR('',#117937,1000.) ;
#11020=VECTOR('',#117938,1000.) ;
#11021=VECTOR('',#117941,1000.) ;
#11022=VECTOR('',#117942,1000.) ;
#11023=VECTOR('',#117943,1000.) ;
#11024=VECTOR('',#117946,1000.) ;
#11025=VECTOR('',#117947,1000.) ;
#11026=VECTOR('',#117948,1000.) ;
#11027=VECTOR('',#117951,1000.) ;
#11028=VECTOR('',#117952,1000.) ;
#11029=VECTOR('',#117953,1000.) ;
#11030=VECTOR('',#117954,1000.) ;
#11031=VECTOR('',#117957,1000.) ;
#11032=VECTOR('',#117958,1000.) ;
#11033=VECTOR('',#117959,1000.) ;
#11034=VECTOR('',#117960,1000.) ;
#11035=VECTOR('',#117963,1000.) ;
#11036=VECTOR('',#117964,1000.) ;
#11037=VECTOR('',#117965,1000.) ;
#11038=VECTOR('',#117966,1000.) ;
#11039=VECTOR('',#117969,1000.) ;
#11040=VECTOR('',#117970,1000.) ;
#11041=VECTOR('',#117971,1000.) ;
#11042=VECTOR('',#117972,1000.) ;
#11043=VECTOR('',#117975,1000.) ;
#11044=VECTOR('',#117976,1000.) ;
#11045=VECTOR('',#117977,1000.) ;
#11046=VECTOR('',#117978,1000.) ;
#11047=VECTOR('',#117981,1000.) ;
#11048=VECTOR('',#117986,1000.) ;
#11049=VECTOR('',#117987,1000.) ;
#11050=VECTOR('',#117990,1000.) ;
#11051=VECTOR('',#117995,1000.) ;
#11052=VECTOR('',#117996,1000.) ;
#11053=VECTOR('',#118011,1000.) ;
#11054=VECTOR('',#118012,1000.) ;
#11055=VECTOR('',#118013,1000.) ;
#11056=VECTOR('',#118014,1000.) ;
#11057=VECTOR('',#118017,1000.) ;
#11058=VECTOR('',#118018,1000.) ;
#11059=VECTOR('',#118019,1000.) ;
#11060=VECTOR('',#118022,1000.) ;
#11061=VECTOR('',#118023,1000.) ;
#11062=VECTOR('',#118024,1000.) ;
#11063=VECTOR('',#118027,1000.) ;
#11064=VECTOR('',#118028,1000.) ;
#11065=VECTOR('',#118029,1000.) ;
#11066=VECTOR('',#118030,1000.) ;
#11067=VECTOR('',#118033,1000.) ;
#11068=VECTOR('',#118034,1000.) ;
#11069=VECTOR('',#118035,1000.) ;
#11070=VECTOR('',#118036,1000.) ;
#11071=VECTOR('',#118039,1000.) ;
#11072=VECTOR('',#118040,1000.) ;
#11073=VECTOR('',#118041,1000.) ;
#11074=VECTOR('',#118044,1000.) ;
#11075=VECTOR('',#118045,1000.) ;
#11076=VECTOR('',#118046,1000.) ;
#11077=VECTOR('',#118049,1000.) ;
#11078=VECTOR('',#118050,1000.) ;
#11079=VECTOR('',#118051,1000.) ;
#11080=VECTOR('',#118052,1000.) ;
#11081=VECTOR('',#118055,1000.) ;
#11082=VECTOR('',#118056,1000.) ;
#11083=VECTOR('',#118057,1000.) ;
#11084=VECTOR('',#118058,1000.) ;
#11085=VECTOR('',#118061,1000.) ;
#11086=VECTOR('',#118062,1000.) ;
#11087=VECTOR('',#118063,1000.) ;
#11088=VECTOR('',#118064,1000.) ;
#11089=VECTOR('',#118067,1000.) ;
#11090=VECTOR('',#118068,1000.) ;
#11091=VECTOR('',#118069,1000.) ;
#11092=VECTOR('',#118070,1000.) ;
#11093=VECTOR('',#118073,1000.) ;
#11094=VECTOR('',#118074,1000.) ;
#11095=VECTOR('',#118075,1000.) ;
#11096=VECTOR('',#118076,1000.) ;
#11097=VECTOR('',#118079,1000.) ;
#11098=VECTOR('',#118084,1000.) ;
#11099=VECTOR('',#118085,1000.) ;
#11100=VECTOR('',#118088,1000.) ;
#11101=VECTOR('',#118093,1000.) ;
#11102=VECTOR('',#118094,1000.) ;
#11103=VECTOR('',#118109,1000.) ;
#11104=VECTOR('',#118110,1000.) ;
#11105=VECTOR('',#118111,1000.) ;
#11106=VECTOR('',#118112,1000.) ;
#11107=VECTOR('',#118115,1000.) ;
#11108=VECTOR('',#118116,1000.) ;
#11109=VECTOR('',#118117,1000.) ;
#11110=VECTOR('',#118120,1000.) ;
#11111=VECTOR('',#118121,1000.) ;
#11112=VECTOR('',#118122,1000.) ;
#11113=VECTOR('',#118125,1000.) ;
#11114=VECTOR('',#118126,1000.) ;
#11115=VECTOR('',#118127,1000.) ;
#11116=VECTOR('',#118128,1000.) ;
#11117=VECTOR('',#118131,1000.) ;
#11118=VECTOR('',#118132,1000.) ;
#11119=VECTOR('',#118133,1000.) ;
#11120=VECTOR('',#118134,1000.) ;
#11121=VECTOR('',#118137,1000.) ;
#11122=VECTOR('',#118138,1000.) ;
#11123=VECTOR('',#118139,1000.) ;
#11124=VECTOR('',#118142,1000.) ;
#11125=VECTOR('',#118143,1000.) ;
#11126=VECTOR('',#118144,1000.) ;
#11127=VECTOR('',#118147,1000.) ;
#11128=VECTOR('',#118148,1000.) ;
#11129=VECTOR('',#118149,1000.) ;
#11130=VECTOR('',#118150,1000.) ;
#11131=VECTOR('',#118153,1000.) ;
#11132=VECTOR('',#118154,1000.) ;
#11133=VECTOR('',#118155,1000.) ;
#11134=VECTOR('',#118156,1000.) ;
#11135=VECTOR('',#118159,1000.) ;
#11136=VECTOR('',#118160,1000.) ;
#11137=VECTOR('',#118161,1000.) ;
#11138=VECTOR('',#118162,1000.) ;
#11139=VECTOR('',#118165,1000.) ;
#11140=VECTOR('',#118166,1000.) ;
#11141=VECTOR('',#118167,1000.) ;
#11142=VECTOR('',#118168,1000.) ;
#11143=VECTOR('',#118171,1000.) ;
#11144=VECTOR('',#118172,1000.) ;
#11145=VECTOR('',#118173,1000.) ;
#11146=VECTOR('',#118174,1000.) ;
#11147=VECTOR('',#118177,1000.) ;
#11148=VECTOR('',#118182,1000.) ;
#11149=VECTOR('',#118183,1000.) ;
#11150=VECTOR('',#118186,1000.) ;
#11151=VECTOR('',#118191,1000.) ;
#11152=VECTOR('',#118192,1000.) ;
#11153=VECTOR('',#118207,1000.) ;
#11154=VECTOR('',#118208,1000.) ;
#11155=VECTOR('',#118209,1000.) ;
#11156=VECTOR('',#118210,1000.) ;
#11157=VECTOR('',#118213,1000.) ;
#11158=VECTOR('',#118214,1000.) ;
#11159=VECTOR('',#118215,1000.) ;
#11160=VECTOR('',#118218,1000.) ;
#11161=VECTOR('',#118219,1000.) ;
#11162=VECTOR('',#118220,1000.) ;
#11163=VECTOR('',#118223,1000.) ;
#11164=VECTOR('',#118224,1000.) ;
#11165=VECTOR('',#118225,1000.) ;
#11166=VECTOR('',#118226,1000.) ;
#11167=VECTOR('',#118229,1000.) ;
#11168=VECTOR('',#118230,1000.) ;
#11169=VECTOR('',#118231,1000.) ;
#11170=VECTOR('',#118232,1000.) ;
#11171=VECTOR('',#118235,1000.) ;
#11172=VECTOR('',#118236,1000.) ;
#11173=VECTOR('',#118237,1000.) ;
#11174=VECTOR('',#118240,1000.) ;
#11175=VECTOR('',#118241,1000.) ;
#11176=VECTOR('',#118242,1000.) ;
#11177=VECTOR('',#118245,1000.) ;
#11178=VECTOR('',#118246,1000.) ;
#11179=VECTOR('',#118247,1000.) ;
#11180=VECTOR('',#118248,1000.) ;
#11181=VECTOR('',#118251,1000.) ;
#11182=VECTOR('',#118252,1000.) ;
#11183=VECTOR('',#118253,1000.) ;
#11184=VECTOR('',#118254,1000.) ;
#11185=VECTOR('',#118257,1000.) ;
#11186=VECTOR('',#118258,1000.) ;
#11187=VECTOR('',#118259,1000.) ;
#11188=VECTOR('',#118260,1000.) ;
#11189=VECTOR('',#118263,1000.) ;
#11190=VECTOR('',#118264,1000.) ;
#11191=VECTOR('',#118265,1000.) ;
#11192=VECTOR('',#118266,1000.) ;
#11193=VECTOR('',#118269,1000.) ;
#11194=VECTOR('',#118270,1000.) ;
#11195=VECTOR('',#118271,1000.) ;
#11196=VECTOR('',#118272,1000.) ;
#11197=VECTOR('',#118275,1000.) ;
#11198=VECTOR('',#118276,1000.) ;
#11199=VECTOR('',#118277,1000.) ;
#11200=VECTOR('',#118278,1000.) ;
#11201=VECTOR('',#118281,1000.) ;
#11202=VECTOR('',#118282,1000.) ;
#11203=VECTOR('',#118283,1000.) ;
#11204=VECTOR('',#118284,1000.) ;
#11205=VECTOR('',#118287,1000.) ;
#11206=VECTOR('',#118288,1000.) ;
#11207=VECTOR('',#118289,1000.) ;
#11208=VECTOR('',#118290,1000.) ;
#11209=VECTOR('',#118293,1000.) ;
#11210=VECTOR('',#118294,1000.) ;
#11211=VECTOR('',#118295,1000.) ;
#11212=VECTOR('',#118296,1000.) ;
#11213=VECTOR('',#118299,1000.) ;
#11214=VECTOR('',#118300,1000.) ;
#11215=VECTOR('',#118301,1000.) ;
#11216=VECTOR('',#118302,1000.) ;
#11217=VECTOR('',#118305,1000.) ;
#11218=VECTOR('',#118306,1000.) ;
#11219=VECTOR('',#118307,1000.) ;
#11220=VECTOR('',#118308,1000.) ;
#11221=VECTOR('',#118311,1000.) ;
#11222=VECTOR('',#118312,1000.) ;
#11223=VECTOR('',#118313,1000.) ;
#11224=VECTOR('',#118314,1000.) ;
#11225=VECTOR('',#118317,1000.) ;
#11226=VECTOR('',#118318,1000.) ;
#11227=VECTOR('',#118319,1000.) ;
#11228=VECTOR('',#118320,1000.) ;
#11229=VECTOR('',#118323,1000.) ;
#11230=VECTOR('',#118324,1000.) ;
#11231=VECTOR('',#118325,1000.) ;
#11232=VECTOR('',#118326,1000.) ;
#11233=VECTOR('',#118329,1000.) ;
#11234=VECTOR('',#118330,1000.) ;
#11235=VECTOR('',#118331,1000.) ;
#11236=VECTOR('',#118332,1000.) ;
#11237=VECTOR('',#118335,1000.) ;
#11238=VECTOR('',#118336,1000.) ;
#11239=VECTOR('',#118337,1000.) ;
#11240=VECTOR('',#118338,1000.) ;
#11241=VECTOR('',#118341,1000.) ;
#11242=VECTOR('',#118342,1000.) ;
#11243=VECTOR('',#118343,1000.) ;
#11244=VECTOR('',#118344,1000.) ;
#11245=VECTOR('',#118347,1000.) ;
#11246=VECTOR('',#118348,1000.) ;
#11247=VECTOR('',#118349,1000.) ;
#11248=VECTOR('',#118350,1000.) ;
#11249=VECTOR('',#118353,1000.) ;
#11250=VECTOR('',#118354,1000.) ;
#11251=VECTOR('',#118355,1000.) ;
#11252=VECTOR('',#118356,1000.) ;
#11253=VECTOR('',#118359,1000.) ;
#11254=VECTOR('',#118360,1000.) ;
#11255=VECTOR('',#118361,1000.) ;
#11256=VECTOR('',#118362,1000.) ;
#11257=VECTOR('',#118365,1000.) ;
#11258=VECTOR('',#118366,1000.) ;
#11259=VECTOR('',#118367,1000.) ;
#11260=VECTOR('',#118368,1000.) ;
#11261=VECTOR('',#118371,1000.) ;
#11262=VECTOR('',#118372,1000.) ;
#11263=VECTOR('',#118373,1000.) ;
#11264=VECTOR('',#118374,1000.) ;
#11265=VECTOR('',#118377,1000.) ;
#11266=VECTOR('',#118378,1000.) ;
#11267=VECTOR('',#118379,1000.) ;
#11268=VECTOR('',#118380,1000.) ;
#11269=VECTOR('',#118383,1000.) ;
#11270=VECTOR('',#118384,1000.) ;
#11271=VECTOR('',#118385,1000.) ;
#11272=VECTOR('',#118386,1000.) ;
#11273=VECTOR('',#118389,1000.) ;
#11274=VECTOR('',#118390,1000.) ;
#11275=VECTOR('',#118391,1000.) ;
#11276=VECTOR('',#118392,1000.) ;
#11277=VECTOR('',#118395,1000.) ;
#11278=VECTOR('',#118396,1000.) ;
#11279=VECTOR('',#118397,1000.) ;
#11280=VECTOR('',#118398,1000.) ;
#11281=VECTOR('',#118401,1000.) ;
#11282=VECTOR('',#118402,1000.) ;
#11283=VECTOR('',#118403,1000.) ;
#11284=VECTOR('',#118404,1000.) ;
#11285=VECTOR('',#118407,1000.) ;
#11286=VECTOR('',#118408,1000.) ;
#11287=VECTOR('',#118409,1000.) ;
#11288=VECTOR('',#118410,1000.) ;
#11289=VECTOR('',#118413,1000.) ;
#11290=VECTOR('',#118414,1000.) ;
#11291=VECTOR('',#118415,1000.) ;
#11292=VECTOR('',#118416,1000.) ;
#11293=VECTOR('',#118419,1000.) ;
#11294=VECTOR('',#118420,1000.) ;
#11295=VECTOR('',#118421,1000.) ;
#11296=VECTOR('',#118422,1000.) ;
#11297=VECTOR('',#118425,1000.) ;
#11298=VECTOR('',#118426,1000.) ;
#11299=VECTOR('',#118427,1000.) ;
#11300=VECTOR('',#118428,1000.) ;
#11301=VECTOR('',#118431,1000.) ;
#11302=VECTOR('',#118432,1000.) ;
#11303=VECTOR('',#118433,1000.) ;
#11304=VECTOR('',#118434,1000.) ;
#11305=VECTOR('',#118437,1000.) ;
#11306=VECTOR('',#118438,1000.) ;
#11307=VECTOR('',#118439,1000.) ;
#11308=VECTOR('',#118440,1000.) ;
#11309=VECTOR('',#118443,1000.) ;
#11310=VECTOR('',#118444,1000.) ;
#11311=VECTOR('',#118445,1000.) ;
#11312=VECTOR('',#118446,1000.) ;
#11313=VECTOR('',#118449,1000.) ;
#11314=VECTOR('',#118450,1000.) ;
#11315=VECTOR('',#118451,1000.) ;
#11316=VECTOR('',#118452,1000.) ;
#11317=VECTOR('',#118455,1000.) ;
#11318=VECTOR('',#118456,1000.) ;
#11319=VECTOR('',#118457,1000.) ;
#11320=VECTOR('',#118458,1000.) ;
#14036=CYLINDRICAL_SURFACE('',#93362,0.1) ;
#14037=CYLINDRICAL_SURFACE('',#93379,0.1) ;
#14038=CYLINDRICAL_SURFACE('',#93396,0.1) ;
#14039=CYLINDRICAL_SURFACE('',#93413,0.1) ;
#14040=CYLINDRICAL_SURFACE('',#93430,0.1) ;
#14041=CYLINDRICAL_SURFACE('',#93447,0.1) ;
#14042=CYLINDRICAL_SURFACE('',#93464,0.1) ;
#14043=CYLINDRICAL_SURFACE('',#93481,0.1) ;
#14044=CYLINDRICAL_SURFACE('',#93543,0.1) ;
#14045=CYLINDRICAL_SURFACE('',#93547,1.) ;
#14046=CYLINDRICAL_SURFACE('',#93548,1.) ;
#14047=CYLINDRICAL_SURFACE('',#93549,1.) ;
#14048=CYLINDRICAL_SURFACE('',#93550,1.) ;
#14049=CYLINDRICAL_SURFACE('',#93551,1.) ;
#14050=CYLINDRICAL_SURFACE('',#93552,0.999999999999999) ;
#14051=CYLINDRICAL_SURFACE('',#93553,0.999999999999999) ;
#14052=CYLINDRICAL_SURFACE('',#93554,1.) ;
#14053=CYLINDRICAL_SURFACE('',#93555,1.) ;
#14054=CYLINDRICAL_SURFACE('',#93556,0.1) ;
#14055=CYLINDRICAL_SURFACE('',#93558,0.100000000000001) ;
#14056=CYLINDRICAL_SURFACE('',#93560,0.100000000000001) ;
#14057=CYLINDRICAL_SURFACE('',#93562,0.0999999999999994) ;
#14058=CYLINDRICAL_SURFACE('',#93564,0.0999999999999994) ;
#14059=CYLINDRICAL_SURFACE('',#93566,0.0999999999999994) ;
#14060=CYLINDRICAL_SURFACE('',#93568,0.0999999999999994) ;
#14061=CYLINDRICAL_SURFACE('',#93570,0.100000000000003) ;
#14062=CYLINDRICAL_SURFACE('',#93572,0.100000000000003) ;
#14063=CYLINDRICAL_SURFACE('',#93592,0.1) ;
#14064=CYLINDRICAL_SURFACE('',#93596,1.) ;
#14065=CYLINDRICAL_SURFACE('',#93597,0.1) ;
#14066=CYLINDRICAL_SURFACE('',#93680,0.1) ;
#14067=CYLINDRICAL_SURFACE('',#93683,0.1) ;
#14068=CYLINDRICAL_SURFACE('',#93686,0.1) ;
#14069=CYLINDRICAL_SURFACE('',#93689,0.1) ;
#14070=CYLINDRICAL_SURFACE('',#93692,0.1) ;
#14071=CYLINDRICAL_SURFACE('',#93695,0.1) ;
#14072=CYLINDRICAL_SURFACE('',#93698,0.1) ;
#14073=CYLINDRICAL_SURFACE('',#93701,0.1) ;
#14074=CYLINDRICAL_SURFACE('',#93704,0.1) ;
#14075=CYLINDRICAL_SURFACE('',#93716,0.1) ;
#14076=CYLINDRICAL_SURFACE('',#93719,0.0999999999999994) ;
#14077=CYLINDRICAL_SURFACE('',#93743,0.1) ;
#14078=CYLINDRICAL_SURFACE('',#93767,0.1) ;
#14079=CYLINDRICAL_SURFACE('',#93771,0.1) ;
#14080=CYLINDRICAL_SURFACE('',#93775,0.1) ;
#14081=CYLINDRICAL_SURFACE('',#93779,0.100000000000001) ;
#14082=CYLINDRICAL_SURFACE('',#93783,0.1) ;
#14083=CYLINDRICAL_SURFACE('',#93787,0.0999999999999994) ;
#14084=CYLINDRICAL_SURFACE('',#93905,0.1) ;
#14085=CYLINDRICAL_SURFACE('',#93909,0.1) ;
#14086=CYLINDRICAL_SURFACE('',#93913,0.0999999999999994) ;
#14087=CYLINDRICAL_SURFACE('',#93917,0.1) ;
#14088=CYLINDRICAL_SURFACE('',#93921,0.1) ;
#14089=CYLINDRICAL_SURFACE('',#93925,0.1) ;
#14090=CYLINDRICAL_SURFACE('',#93929,0.1) ;
#14091=CYLINDRICAL_SURFACE('',#93933,0.1) ;
#14092=CYLINDRICAL_SURFACE('',#93937,0.1) ;
#14093=CYLINDRICAL_SURFACE('',#93941,0.1) ;
#14094=CYLINDRICAL_SURFACE('',#93944,1.65625) ;
#14095=CYLINDRICAL_SURFACE('',#93947,0.1) ;
#14096=CYLINDRICAL_SURFACE('',#93951,0.1) ;
#14097=CYLINDRICAL_SURFACE('',#93955,0.1) ;
#14098=CYLINDRICAL_SURFACE('',#93970,0.1) ;
#14099=CYLINDRICAL_SURFACE('',#93973,0.1) ;
#14100=CYLINDRICAL_SURFACE('',#93984,0.1) ;
#14101=CYLINDRICAL_SURFACE('',#93986,0.1) ;
#14102=CYLINDRICAL_SURFACE('',#93988,0.1) ;
#14103=CYLINDRICAL_SURFACE('',#93990,0.1) ;
#14104=CYLINDRICAL_SURFACE('',#93992,0.1) ;
#14105=CYLINDRICAL_SURFACE('',#93994,0.1) ;
#14106=CYLINDRICAL_SURFACE('',#94005,0.1) ;
#14107=CYLINDRICAL_SURFACE('',#94007,0.0999999999999998) ;
#14108=CYLINDRICAL_SURFACE('',#94009,0.1) ;
#14109=CYLINDRICAL_SURFACE('',#94011,0.1) ;
#14110=CYLINDRICAL_SURFACE('',#94013,0.1) ;
#14111=CYLINDRICAL_SURFACE('',#94023,0.1) ;
#14112=CYLINDRICAL_SURFACE('',#94030,0.1) ;
#14113=CYLINDRICAL_SURFACE('',#94032,0.1) ;
#14114=CYLINDRICAL_SURFACE('',#94034,0.1) ;
#14115=CYLINDRICAL_SURFACE('',#94038,0.1) ;
#14116=CYLINDRICAL_SURFACE('',#94040,0.1) ;
#14117=CYLINDRICAL_SURFACE('',#94042,0.0999999999999998) ;
#14118=CYLINDRICAL_SURFACE('',#94049,0.1) ;
#14119=CYLINDRICAL_SURFACE('',#94056,0.1) ;
#14120=CYLINDRICAL_SURFACE('',#94058,0.1) ;
#14121=CYLINDRICAL_SURFACE('',#94062,0.1) ;
#14122=CYLINDRICAL_SURFACE('',#94065,0.1) ;
#14123=CYLINDRICAL_SURFACE('',#94067,0.1) ;
#14124=CYLINDRICAL_SURFACE('',#94073,0.100000000000003) ;
#14125=CYLINDRICAL_SURFACE('',#94075,0.100000000000003) ;
#14126=CYLINDRICAL_SURFACE('',#94081,0.1) ;
#14127=CYLINDRICAL_SURFACE('',#94083,0.1) ;
#14128=CYLINDRICAL_SURFACE('',#94089,0.1) ;
#14129=CYLINDRICAL_SURFACE('',#94091,0.1) ;
#14130=CYLINDRICAL_SURFACE('',#94097,0.100000000000003) ;
#14131=CYLINDRICAL_SURFACE('',#94099,0.100000000000003) ;
#14132=CYLINDRICAL_SURFACE('',#94105,0.0999999999999998) ;
#14133=CYLINDRICAL_SURFACE('',#94107,0.0999999999999998) ;
#14134=CYLINDRICAL_SURFACE('',#94113,0.1) ;
#14135=CYLINDRICAL_SURFACE('',#94115,0.1) ;
#14136=CYLINDRICAL_SURFACE('',#94121,0.1) ;
#14137=CYLINDRICAL_SURFACE('',#94123,0.1) ;
#14138=CYLINDRICAL_SURFACE('',#94129,0.0999999999999998) ;
#14139=CYLINDRICAL_SURFACE('',#94131,0.0999999999999998) ;
#14140=CYLINDRICAL_SURFACE('',#94134,0.1) ;
#14141=CYLINDRICAL_SURFACE('',#94141,0.1) ;
#14142=CYLINDRICAL_SURFACE('',#94143,0.1) ;
#14143=CYLINDRICAL_SURFACE('',#94149,0.1) ;
#14144=CYLINDRICAL_SURFACE('',#94151,0.1) ;
#14145=CYLINDRICAL_SURFACE('',#94157,0.0999999999999999) ;
#14146=CYLINDRICAL_SURFACE('',#94165,0.1) ;
#14147=CYLINDRICAL_SURFACE('',#94166,0.1) ;
#14148=CYLINDRICAL_SURFACE('',#94170,0.1) ;
#14149=CYLINDRICAL_SURFACE('',#94172,0.1) ;
#14150=CYLINDRICAL_SURFACE('',#94178,0.0999999999999998) ;
#14151=CYLINDRICAL_SURFACE('',#94180,0.1) ;
#14152=CYLINDRICAL_SURFACE('',#94186,0.1) ;
#14153=CYLINDRICAL_SURFACE('',#94187,0.1) ;
#14154=CYLINDRICAL_SURFACE('',#94194,0.0999999999999994) ;
#14155=CYLINDRICAL_SURFACE('',#94196,0.1) ;
#14156=CYLINDRICAL_SURFACE('',#94202,0.1) ;
#14157=CYLINDRICAL_SURFACE('',#94203,0.1) ;
#14158=CYLINDRICAL_SURFACE('',#94207,0.1) ;
#14159=CYLINDRICAL_SURFACE('',#94209,0.0999999999999994) ;
#14160=CYLINDRICAL_SURFACE('',#94215,0.1) ;
#14161=CYLINDRICAL_SURFACE('',#94223,0.0999999999999998) ;
#14162=CYLINDRICAL_SURFACE('',#94225,0.0999999999999994) ;
#14163=CYLINDRICAL_SURFACE('',#94231,0.1) ;
#14164=CYLINDRICAL_SURFACE('',#94233,0.1) ;
#14165=CYLINDRICAL_SURFACE('',#94239,0.1) ;
#14166=CYLINDRICAL_SURFACE('',#94251,1.) ;
#14167=CYLINDRICAL_SURFACE('',#94254,0.2) ;
#14168=CYLINDRICAL_SURFACE('',#94268,0.1) ;
#14169=CYLINDRICAL_SURFACE('',#94271,0.1) ;
#14170=CYLINDRICAL_SURFACE('',#94277,0.1) ;
#14171=CYLINDRICAL_SURFACE('',#94280,0.1) ;
#14172=CYLINDRICAL_SURFACE('',#94282,0.1) ;
#14173=CYLINDRICAL_SURFACE('',#94289,0.1) ;
#14174=CYLINDRICAL_SURFACE('',#94291,0.1) ;
#14175=CYLINDRICAL_SURFACE('',#94293,0.1) ;
#14176=CYLINDRICAL_SURFACE('',#94297,0.1) ;
#14177=CYLINDRICAL_SURFACE('',#94300,0.1) ;
#14178=CYLINDRICAL_SURFACE('',#94302,0.1) ;
#14179=CYLINDRICAL_SURFACE('',#94305,0.1) ;
#14180=CYLINDRICAL_SURFACE('',#94311,0.1) ;
#14181=CYLINDRICAL_SURFACE('',#94314,0.1) ;
#14182=CYLINDRICAL_SURFACE('',#94316,0.1) ;
#14183=CYLINDRICAL_SURFACE('',#94323,0.1) ;
#14184=CYLINDRICAL_SURFACE('',#94325,0.1) ;
#14185=CYLINDRICAL_SURFACE('',#94327,0.1) ;
#14186=CYLINDRICAL_SURFACE('',#94331,0.1) ;
#14187=CYLINDRICAL_SURFACE('',#94334,0.1) ;
#14188=CYLINDRICAL_SURFACE('',#94338,0.1) ;
#14189=CYLINDRICAL_SURFACE('',#94342,0.1) ;
#14190=CYLINDRICAL_SURFACE('',#94346,0.1) ;
#14191=CYLINDRICAL_SURFACE('',#94351,0.1) ;
#14192=CYLINDRICAL_SURFACE('',#94355,0.1) ;
#14193=CYLINDRICAL_SURFACE('',#94359,0.1) ;
#14194=CYLINDRICAL_SURFACE('',#94362,0.1) ;
#14195=CYLINDRICAL_SURFACE('',#94366,0.1) ;
#14196=CYLINDRICAL_SURFACE('',#94370,0.1) ;
#14197=CYLINDRICAL_SURFACE('',#94371,0.1) ;
#14198=CYLINDRICAL_SURFACE('',#94375,0.1) ;
#14199=CYLINDRICAL_SURFACE('',#94377,0.1) ;
#14200=CYLINDRICAL_SURFACE('',#94452,0.100000000000003) ;
#14201=CYLINDRICAL_SURFACE('',#94456,0.100000000000003) ;
#14202=CYLINDRICAL_SURFACE('',#94460,0.0999999999999959) ;
#14203=CYLINDRICAL_SURFACE('',#94464,0.100000000000003) ;
#14204=CYLINDRICAL_SURFACE('',#94468,0.100000000000003) ;
#14205=CYLINDRICAL_SURFACE('',#94472,0.100000000000003) ;
#14206=CYLINDRICAL_SURFACE('',#94476,0.100000000000003) ;
#14207=CYLINDRICAL_SURFACE('',#94480,0.100000000000003) ;
#14208=CYLINDRICAL_SURFACE('',#94484,0.100000000000003) ;
#14209=CYLINDRICAL_SURFACE('',#94488,0.100000000000003) ;
#14210=CYLINDRICAL_SURFACE('',#94491,1.65625) ;
#14211=CYLINDRICAL_SURFACE('',#94494,0.100000000000003) ;
#14212=CYLINDRICAL_SURFACE('',#94498,0.100000000000003) ;
#14213=CYLINDRICAL_SURFACE('',#94502,0.100000000000003) ;
#14214=CYLINDRICAL_SURFACE('',#94512,0.0999999999999994) ;
#14215=CYLINDRICAL_SURFACE('',#94516,0.0999999999999994) ;
#14216=CYLINDRICAL_SURFACE('',#94520,0.0999999999999994) ;
#14217=CYLINDRICAL_SURFACE('',#94524,0.0999999999999994) ;
#14218=CYLINDRICAL_SURFACE('',#94528,0.100000000000003) ;
#14219=CYLINDRICAL_SURFACE('',#94532,0.0999999999999994) ;
#14220=CYLINDRICAL_SURFACE('',#94536,0.0999999999999994) ;
#14221=CYLINDRICAL_SURFACE('',#94540,0.100000000000003) ;
#14222=CYLINDRICAL_SURFACE('',#94544,0.100000000000003) ;
#14223=CYLINDRICAL_SURFACE('',#94548,0.100000000000003) ;
#14224=CYLINDRICAL_SURFACE('',#94551,1.65625) ;
#14225=CYLINDRICAL_SURFACE('',#94554,0.0999999999999994) ;
#14226=CYLINDRICAL_SURFACE('',#94558,0.0999999999999994) ;
#14227=CYLINDRICAL_SURFACE('',#94562,0.0999999999999994) ;
#14228=CYLINDRICAL_SURFACE('',#94572,0.0999999999999994) ;
#14229=CYLINDRICAL_SURFACE('',#94576,0.0999999999999994) ;
#14230=CYLINDRICAL_SURFACE('',#94580,0.0999999999999994) ;
#14231=CYLINDRICAL_SURFACE('',#94584,0.0999999999999994) ;
#14232=CYLINDRICAL_SURFACE('',#94588,0.0999999999999994) ;
#14233=CYLINDRICAL_SURFACE('',#94592,0.0999999999999994) ;
#14234=CYLINDRICAL_SURFACE('',#94596,0.0999999999999994) ;
#14235=CYLINDRICAL_SURFACE('',#94600,0.0999999999999994) ;
#14236=CYLINDRICAL_SURFACE('',#94604,0.0999999999999994) ;
#14237=CYLINDRICAL_SURFACE('',#94608,0.0999999999999994) ;
#14238=CYLINDRICAL_SURFACE('',#94611,1.65625) ;
#14239=CYLINDRICAL_SURFACE('',#94614,0.0999999999999994) ;
#14240=CYLINDRICAL_SURFACE('',#94618,0.0999999999999994) ;
#14241=CYLINDRICAL_SURFACE('',#94622,0.0999999999999994) ;
#14242=CYLINDRICAL_SURFACE('',#94632,0.0999999999999994) ;
#14243=CYLINDRICAL_SURFACE('',#94636,0.0999999999999994) ;
#14244=CYLINDRICAL_SURFACE('',#94640,0.0999999999999994) ;
#14245=CYLINDRICAL_SURFACE('',#94644,0.0999999999999994) ;
#14246=CYLINDRICAL_SURFACE('',#94648,0.0999999999999994) ;
#14247=CYLINDRICAL_SURFACE('',#94652,0.0999999999999994) ;
#14248=CYLINDRICAL_SURFACE('',#94656,0.0999999999999994) ;
#14249=CYLINDRICAL_SURFACE('',#94660,0.0999999999999994) ;
#14250=CYLINDRICAL_SURFACE('',#94664,0.0999999999999994) ;
#14251=CYLINDRICAL_SURFACE('',#94668,0.0999999999999994) ;
#14252=CYLINDRICAL_SURFACE('',#94671,1.65625) ;
#14253=CYLINDRICAL_SURFACE('',#94674,0.0999999999999994) ;
#14254=CYLINDRICAL_SURFACE('',#94678,0.0999999999999994) ;
#14255=CYLINDRICAL_SURFACE('',#94682,0.0999999999999994) ;
#14256=CYLINDRICAL_SURFACE('',#94692,0.0999999999999994) ;
#14257=CYLINDRICAL_SURFACE('',#94696,0.0999999999999994) ;
#14258=CYLINDRICAL_SURFACE('',#94700,0.0999999999999994) ;
#14259=CYLINDRICAL_SURFACE('',#94704,0.0999999999999994) ;
#14260=CYLINDRICAL_SURFACE('',#94708,0.0999999999999994) ;
#14261=CYLINDRICAL_SURFACE('',#94712,0.0999999999999994) ;
#14262=CYLINDRICAL_SURFACE('',#94716,0.0999999999999994) ;
#14263=CYLINDRICAL_SURFACE('',#94720,0.0999999999999994) ;
#14264=CYLINDRICAL_SURFACE('',#94724,0.0999999999999994) ;
#14265=CYLINDRICAL_SURFACE('',#94728,0.0999999999999994) ;
#14266=CYLINDRICAL_SURFACE('',#94731,1.65625) ;
#14267=CYLINDRICAL_SURFACE('',#94734,0.0999999999999994) ;
#14268=CYLINDRICAL_SURFACE('',#94738,0.0999999999999994) ;
#14269=CYLINDRICAL_SURFACE('',#94742,0.0999999999999994) ;
#14270=CYLINDRICAL_SURFACE('',#94752,0.0999999999999994) ;
#14271=CYLINDRICAL_SURFACE('',#94756,0.0999999999999994) ;
#14272=CYLINDRICAL_SURFACE('',#94760,0.0999999999999994) ;
#14273=CYLINDRICAL_SURFACE('',#94764,0.100000000000001) ;
#14274=CYLINDRICAL_SURFACE('',#94768,0.0999999999999994) ;
#14275=CYLINDRICAL_SURFACE('',#94772,0.0999999999999994) ;
#14276=CYLINDRICAL_SURFACE('',#94776,0.0999999999999994) ;
#14277=CYLINDRICAL_SURFACE('',#94780,0.0999999999999994) ;
#14278=CYLINDRICAL_SURFACE('',#94784,0.0999999999999994) ;
#14279=CYLINDRICAL_SURFACE('',#94788,0.0999999999999994) ;
#14280=CYLINDRICAL_SURFACE('',#94791,1.65625) ;
#14281=CYLINDRICAL_SURFACE('',#94794,0.0999999999999994) ;
#14282=CYLINDRICAL_SURFACE('',#94798,0.0999999999999994) ;
#14283=CYLINDRICAL_SURFACE('',#94802,0.0999999999999994) ;
#14284=CYLINDRICAL_SURFACE('',#94812,0.0999999999999994) ;
#14285=CYLINDRICAL_SURFACE('',#94816,0.0999999999999994) ;
#14286=CYLINDRICAL_SURFACE('',#94820,0.0999999999999994) ;
#14287=CYLINDRICAL_SURFACE('',#94824,0.100000000000001) ;
#14288=CYLINDRICAL_SURFACE('',#94828,0.100000000000001) ;
#14289=CYLINDRICAL_SURFACE('',#94832,0.0999999999999994) ;
#14290=CYLINDRICAL_SURFACE('',#94836,0.0999999999999994) ;
#14291=CYLINDRICAL_SURFACE('',#94840,0.0999999999999994) ;
#14292=CYLINDRICAL_SURFACE('',#94844,0.0999999999999994) ;
#14293=CYLINDRICAL_SURFACE('',#94848,0.0999999999999994) ;
#14294=CYLINDRICAL_SURFACE('',#94851,1.65625) ;
#14295=CYLINDRICAL_SURFACE('',#94854,0.0999999999999994) ;
#14296=CYLINDRICAL_SURFACE('',#94858,0.0999999999999994) ;
#14297=CYLINDRICAL_SURFACE('',#94862,0.0999999999999994) ;
#14298=CYLINDRICAL_SURFACE('',#94872,0.1) ;
#14299=CYLINDRICAL_SURFACE('',#94876,0.1) ;
#14300=CYLINDRICAL_SURFACE('',#94880,0.0999999999999994) ;
#14301=CYLINDRICAL_SURFACE('',#94884,0.1) ;
#14302=CYLINDRICAL_SURFACE('',#94888,0.100000000000001) ;
#14303=CYLINDRICAL_SURFACE('',#94892,0.0999999999999994) ;
#14304=CYLINDRICAL_SURFACE('',#94896,0.0999999999999994) ;
#14305=CYLINDRICAL_SURFACE('',#94900,0.0999999999999994) ;
#14306=CYLINDRICAL_SURFACE('',#94904,0.0999999999999994) ;
#14307=CYLINDRICAL_SURFACE('',#94908,0.0999999999999994) ;
#14308=CYLINDRICAL_SURFACE('',#94911,1.65625) ;
#14309=CYLINDRICAL_SURFACE('',#94914,0.1) ;
#14310=CYLINDRICAL_SURFACE('',#94918,0.1) ;
#14311=CYLINDRICAL_SURFACE('',#94922,0.1) ;
#14312=CYLINDRICAL_SURFACE('',#94932,0.0999999999999998) ;
#14313=CYLINDRICAL_SURFACE('',#94936,0.0999999999999998) ;
#14314=CYLINDRICAL_SURFACE('',#94940,0.0999999999999994) ;
#14315=CYLINDRICAL_SURFACE('',#94944,0.100000000000001) ;
#14316=CYLINDRICAL_SURFACE('',#94948,0.1) ;
#14317=CYLINDRICAL_SURFACE('',#94952,0.1) ;
#14318=CYLINDRICAL_SURFACE('',#94956,0.1) ;
#14319=CYLINDRICAL_SURFACE('',#94960,0.1) ;
#14320=CYLINDRICAL_SURFACE('',#94964,0.1) ;
#14321=CYLINDRICAL_SURFACE('',#94968,0.1) ;
#14322=CYLINDRICAL_SURFACE('',#94971,1.65625) ;
#14323=CYLINDRICAL_SURFACE('',#94974,0.0999999999999998) ;
#14324=CYLINDRICAL_SURFACE('',#94978,0.0999999999999998) ;
#14325=CYLINDRICAL_SURFACE('',#94982,0.1) ;
#14326=CYLINDRICAL_SURFACE('',#95037,0.1) ;
#14327=CYLINDRICAL_SURFACE('',#95040,0.1) ;
#14328=CYLINDRICAL_SURFACE('',#95051,0.1) ;
#14329=CYLINDRICAL_SURFACE('',#95053,0.1) ;
#14330=CYLINDRICAL_SURFACE('',#95055,0.1) ;
#14331=CYLINDRICAL_SURFACE('',#95057,0.1) ;
#14332=CYLINDRICAL_SURFACE('',#95059,0.1) ;
#14333=CYLINDRICAL_SURFACE('',#95061,0.1) ;
#14334=CYLINDRICAL_SURFACE('',#95072,0.1) ;
#14335=CYLINDRICAL_SURFACE('',#95074,0.0999999999999998) ;
#14336=CYLINDRICAL_SURFACE('',#95076,0.1) ;
#14337=CYLINDRICAL_SURFACE('',#95078,0.1) ;
#14338=CYLINDRICAL_SURFACE('',#95080,0.1) ;
#14339=CYLINDRICAL_SURFACE('',#95090,0.1) ;
#14340=CYLINDRICAL_SURFACE('',#95097,0.1) ;
#14341=CYLINDRICAL_SURFACE('',#95099,0.1) ;
#14342=CYLINDRICAL_SURFACE('',#95101,0.0999999999999998) ;
#14343=CYLINDRICAL_SURFACE('',#95105,0.1) ;
#14344=CYLINDRICAL_SURFACE('',#95107,0.1) ;
#14345=CYLINDRICAL_SURFACE('',#95109,0.0999999999999998) ;
#14346=CYLINDRICAL_SURFACE('',#95116,0.1) ;
#14347=CYLINDRICAL_SURFACE('',#95123,0.1) ;
#14348=CYLINDRICAL_SURFACE('',#95125,0.1) ;
#14349=CYLINDRICAL_SURFACE('',#95129,0.1) ;
#14350=CYLINDRICAL_SURFACE('',#95132,0.1) ;
#14351=CYLINDRICAL_SURFACE('',#95134,0.1) ;
#14352=CYLINDRICAL_SURFACE('',#95137,0.1) ;
#14353=CYLINDRICAL_SURFACE('',#95144,0.1) ;
#14354=CYLINDRICAL_SURFACE('',#95146,0.1) ;
#14355=CYLINDRICAL_SURFACE('',#95152,0.1) ;
#14356=CYLINDRICAL_SURFACE('',#95154,0.1) ;
#14357=CYLINDRICAL_SURFACE('',#95160,0.1) ;
#14358=CYLINDRICAL_SURFACE('',#95168,0.1) ;
#14359=CYLINDRICAL_SURFACE('',#95169,0.1) ;
#14360=CYLINDRICAL_SURFACE('',#95173,0.1) ;
#14361=CYLINDRICAL_SURFACE('',#95175,0.0999999999999998) ;
#14362=CYLINDRICAL_SURFACE('',#95181,0.0999999999999998) ;
#14363=CYLINDRICAL_SURFACE('',#95183,0.1) ;
#14364=CYLINDRICAL_SURFACE('',#95189,0.0999999999999998) ;
#14365=CYLINDRICAL_SURFACE('',#95190,0.100000000000003) ;
#14366=CYLINDRICAL_SURFACE('',#95197,0.0999999999999994) ;
#14367=CYLINDRICAL_SURFACE('',#95199,0.1) ;
#14368=CYLINDRICAL_SURFACE('',#95205,0.0999999999999989) ;
#14369=CYLINDRICAL_SURFACE('',#95206,0.100000000000003) ;
#14370=CYLINDRICAL_SURFACE('',#95210,0.1) ;
#14371=CYLINDRICAL_SURFACE('',#95212,0.0999999999999994) ;
#14372=CYLINDRICAL_SURFACE('',#95218,0.0999999999999989) ;
#14373=CYLINDRICAL_SURFACE('',#95226,0.0999999999999998) ;
#14374=CYLINDRICAL_SURFACE('',#95228,0.0999999999999994) ;
#14375=CYLINDRICAL_SURFACE('',#95234,0.100000000000003) ;
#14376=CYLINDRICAL_SURFACE('',#95236,0.100000000000003) ;
#14377=CYLINDRICAL_SURFACE('',#95242,0.1) ;
#14378=CYLINDRICAL_SURFACE('',#95243,0.0999999999999994) ;
#14379=CYLINDRICAL_SURFACE('',#95250,0.0999999999999994) ;
#14380=CYLINDRICAL_SURFACE('',#95252,0.1) ;
#14381=CYLINDRICAL_SURFACE('',#95258,0.0999999999999989) ;
#14382=CYLINDRICAL_SURFACE('',#95259,0.100000000000003) ;
#14383=CYLINDRICAL_SURFACE('',#95263,0.1) ;
#14384=CYLINDRICAL_SURFACE('',#95265,0.0999999999999994) ;
#14385=CYLINDRICAL_SURFACE('',#95271,0.0999999999999989) ;
#14386=CYLINDRICAL_SURFACE('',#95279,0.0999999999999998) ;
#14387=CYLINDRICAL_SURFACE('',#95281,0.0999999999999994) ;
#14388=CYLINDRICAL_SURFACE('',#95287,0.0999999999999994) ;
#14389=CYLINDRICAL_SURFACE('',#95289,0.0999999999999994) ;
#14390=CYLINDRICAL_SURFACE('',#95295,0.1) ;
#14391=CYLINDRICAL_SURFACE('',#95296,0.0999999999999994) ;
#14392=CYLINDRICAL_SURFACE('',#95303,0.0999999999999994) ;
#14393=CYLINDRICAL_SURFACE('',#95305,0.1) ;
#14394=CYLINDRICAL_SURFACE('',#95311,0.0999999999999989) ;
#14395=CYLINDRICAL_SURFACE('',#95312,0.0999999999999994) ;
#14396=CYLINDRICAL_SURFACE('',#95316,0.1) ;
#14397=CYLINDRICAL_SURFACE('',#95318,0.0999999999999994) ;
#14398=CYLINDRICAL_SURFACE('',#95324,0.0999999999999989) ;
#14399=CYLINDRICAL_SURFACE('',#95332,0.0999999999999998) ;
#14400=CYLINDRICAL_SURFACE('',#95334,0.0999999999999994) ;
#14401=CYLINDRICAL_SURFACE('',#95340,0.0999999999999994) ;
#14402=CYLINDRICAL_SURFACE('',#95342,0.0999999999999994) ;
#14403=CYLINDRICAL_SURFACE('',#95348,0.1) ;
#14404=CYLINDRICAL_SURFACE('',#95349,0.0999999999999994) ;
#14405=CYLINDRICAL_SURFACE('',#95356,0.0999999999999994) ;
#14406=CYLINDRICAL_SURFACE('',#95358,0.1) ;
#14407=CYLINDRICAL_SURFACE('',#95364,0.0999999999999989) ;
#14408=CYLINDRICAL_SURFACE('',#95365,0.0999999999999994) ;
#14409=CYLINDRICAL_SURFACE('',#95369,0.1) ;
#14410=CYLINDRICAL_SURFACE('',#95371,0.0999999999999994) ;
#14411=CYLINDRICAL_SURFACE('',#95377,0.0999999999999989) ;
#14412=CYLINDRICAL_SURFACE('',#95385,0.0999999999999998) ;
#14413=CYLINDRICAL_SURFACE('',#95387,0.0999999999999994) ;
#14414=CYLINDRICAL_SURFACE('',#95393,0.0999999999999994) ;
#14415=CYLINDRICAL_SURFACE('',#95395,0.0999999999999994) ;
#14416=CYLINDRICAL_SURFACE('',#95401,0.1) ;
#14417=CYLINDRICAL_SURFACE('',#95402,0.0999999999999994) ;
#14418=CYLINDRICAL_SURFACE('',#95409,0.0999999999999994) ;
#14419=CYLINDRICAL_SURFACE('',#95411,0.1) ;
#14420=CYLINDRICAL_SURFACE('',#95417,0.0999999999999989) ;
#14421=CYLINDRICAL_SURFACE('',#95418,0.0999999999999994) ;
#14422=CYLINDRICAL_SURFACE('',#95422,0.1) ;
#14423=CYLINDRICAL_SURFACE('',#95424,0.0999999999999994) ;
#14424=CYLINDRICAL_SURFACE('',#95430,0.0999999999999989) ;
#14425=CYLINDRICAL_SURFACE('',#95438,0.0999999999999998) ;
#14426=CYLINDRICAL_SURFACE('',#95440,0.0999999999999994) ;
#14427=CYLINDRICAL_SURFACE('',#95446,0.0999999999999994) ;
#14428=CYLINDRICAL_SURFACE('',#95448,0.0999999999999994) ;
#14429=CYLINDRICAL_SURFACE('',#95454,0.1) ;
#14430=CYLINDRICAL_SURFACE('',#95455,0.0999999999999994) ;
#14431=CYLINDRICAL_SURFACE('',#95462,0.0999999999999994) ;
#14432=CYLINDRICAL_SURFACE('',#95464,0.1) ;
#14433=CYLINDRICAL_SURFACE('',#95470,0.0999999999999989) ;
#14434=CYLINDRICAL_SURFACE('',#95471,0.0999999999999994) ;
#14435=CYLINDRICAL_SURFACE('',#95475,0.1) ;
#14436=CYLINDRICAL_SURFACE('',#95477,0.0999999999999994) ;
#14437=CYLINDRICAL_SURFACE('',#95483,0.1) ;
#14438=CYLINDRICAL_SURFACE('',#95491,0.0999999999999998) ;
#14439=CYLINDRICAL_SURFACE('',#95493,0.0999999999999994) ;
#14440=CYLINDRICAL_SURFACE('',#95499,0.0999999999999994) ;
#14441=CYLINDRICAL_SURFACE('',#95501,0.0999999999999994) ;
#14442=CYLINDRICAL_SURFACE('',#95507,0.1) ;
#14443=CYLINDRICAL_SURFACE('',#95508,0.0999999999999994) ;
#14444=CYLINDRICAL_SURFACE('',#95515,0.0999999999999994) ;
#14445=CYLINDRICAL_SURFACE('',#95517,0.1) ;
#14446=CYLINDRICAL_SURFACE('',#95523,0.1) ;
#14447=CYLINDRICAL_SURFACE('',#95524,0.0999999999999994) ;
#14448=CYLINDRICAL_SURFACE('',#95528,0.1) ;
#14449=CYLINDRICAL_SURFACE('',#95530,0.0999999999999994) ;
#14450=CYLINDRICAL_SURFACE('',#95536,0.1) ;
#14451=CYLINDRICAL_SURFACE('',#95544,0.0999999999999998) ;
#14452=CYLINDRICAL_SURFACE('',#95546,0.0999999999999994) ;
#14453=CYLINDRICAL_SURFACE('',#95552,0.0999999999999994) ;
#14454=CYLINDRICAL_SURFACE('',#95554,0.0999999999999994) ;
#14455=CYLINDRICAL_SURFACE('',#95560,0.1) ;
#14456=CYLINDRICAL_SURFACE('',#95561,0.0999999999999994) ;
#14457=CYLINDRICAL_SURFACE('',#95568,0.0999999999999994) ;
#14458=CYLINDRICAL_SURFACE('',#95570,0.1) ;
#14459=CYLINDRICAL_SURFACE('',#95576,0.1) ;
#14460=CYLINDRICAL_SURFACE('',#95577,0.0999999999999994) ;
#14461=CYLINDRICAL_SURFACE('',#95581,0.1) ;
#14462=CYLINDRICAL_SURFACE('',#95583,0.0999999999999994) ;
#14463=CYLINDRICAL_SURFACE('',#95589,0.1) ;
#14464=CYLINDRICAL_SURFACE('',#95597,0.0999999999999998) ;
#14465=CYLINDRICAL_SURFACE('',#95599,0.0999999999999994) ;
#14466=CYLINDRICAL_SURFACE('',#95605,0.1) ;
#14467=CYLINDRICAL_SURFACE('',#95607,0.1) ;
#14468=CYLINDRICAL_SURFACE('',#95613,0.1) ;
#14469=CYLINDRICAL_SURFACE('',#95614,0.1) ;
#14470=CYLINDRICAL_SURFACE('',#95621,0.0999999999999994) ;
#14471=CYLINDRICAL_SURFACE('',#95623,0.1) ;
#14472=CYLINDRICAL_SURFACE('',#95629,0.1) ;
#14473=CYLINDRICAL_SURFACE('',#95630,0.1) ;
#14474=CYLINDRICAL_SURFACE('',#95634,0.1) ;
#14475=CYLINDRICAL_SURFACE('',#95636,0.0999999999999994) ;
#14476=CYLINDRICAL_SURFACE('',#95642,0.1) ;
#14477=CYLINDRICAL_SURFACE('',#95650,0.0999999999999998) ;
#14478=CYLINDRICAL_SURFACE('',#95652,0.0999999999999994) ;
#14479=CYLINDRICAL_SURFACE('',#95658,0.0999999999999998) ;
#14480=CYLINDRICAL_SURFACE('',#95660,0.0999999999999998) ;
#14481=CYLINDRICAL_SURFACE('',#95666,0.1) ;
#14482=CYLINDRICAL_SURFACE('',#95667,0.1) ;
#14483=CYLINDRICAL_SURFACE('',#95670,0.1) ;
#14484=CYLINDRICAL_SURFACE('',#95681,0.1) ;
#14485=CYLINDRICAL_SURFACE('',#95683,0.1) ;
#14486=CYLINDRICAL_SURFACE('',#95685,0.1) ;
#14487=CYLINDRICAL_SURFACE('',#95687,0.1) ;
#14488=CYLINDRICAL_SURFACE('',#95689,0.1) ;
#14489=CYLINDRICAL_SURFACE('',#95691,0.1) ;
#14490=CYLINDRICAL_SURFACE('',#95702,0.1) ;
#14491=CYLINDRICAL_SURFACE('',#95704,0.0999999999999998) ;
#14492=CYLINDRICAL_SURFACE('',#95706,0.1) ;
#14493=CYLINDRICAL_SURFACE('',#95708,0.1) ;
#14494=CYLINDRICAL_SURFACE('',#95710,0.1) ;
#14495=CYLINDRICAL_SURFACE('',#95720,0.1) ;
#14496=CYLINDRICAL_SURFACE('',#95727,0.1) ;
#14497=CYLINDRICAL_SURFACE('',#95729,0.1) ;
#14498=CYLINDRICAL_SURFACE('',#95731,0.1) ;
#14499=CYLINDRICAL_SURFACE('',#95735,0.1) ;
#14500=CYLINDRICAL_SURFACE('',#95737,0.1) ;
#14501=CYLINDRICAL_SURFACE('',#95739,0.0999999999999998) ;
#14502=CYLINDRICAL_SURFACE('',#95746,0.1) ;
#14503=CYLINDRICAL_SURFACE('',#95753,0.1) ;
#14504=CYLINDRICAL_SURFACE('',#95755,0.1) ;
#14505=CYLINDRICAL_SURFACE('',#95759,0.1) ;
#14506=CYLINDRICAL_SURFACE('',#95762,0.1) ;
#14507=CYLINDRICAL_SURFACE('',#95764,0.0999999999999994) ;
#14508=CYLINDRICAL_SURFACE('',#95767,0.1) ;
#14509=CYLINDRICAL_SURFACE('',#95774,0.0999999999999994) ;
#14510=CYLINDRICAL_SURFACE('',#95776,0.0999999999999994) ;
#14511=CYLINDRICAL_SURFACE('',#95782,0.1) ;
#14512=CYLINDRICAL_SURFACE('',#95784,0.1) ;
#14513=CYLINDRICAL_SURFACE('',#95790,0.1) ;
#14514=CYLINDRICAL_SURFACE('',#95798,0.1) ;
#14515=CYLINDRICAL_SURFACE('',#95799,0.1) ;
#14516=CYLINDRICAL_SURFACE('',#95803,0.1) ;
#14517=CYLINDRICAL_SURFACE('',#95805,0.1) ;
#14518=CYLINDRICAL_SURFACE('',#95811,0.0999999999999998) ;
#14519=CYLINDRICAL_SURFACE('',#95813,0.1) ;
#14520=CYLINDRICAL_SURFACE('',#95819,0.1) ;
#14521=CYLINDRICAL_SURFACE('',#95820,0.1) ;
#14522=CYLINDRICAL_SURFACE('',#95823,0.1) ;
#14523=CYLINDRICAL_SURFACE('',#95834,0.1) ;
#14524=CYLINDRICAL_SURFACE('',#95836,0.1) ;
#14525=CYLINDRICAL_SURFACE('',#95838,0.1) ;
#14526=CYLINDRICAL_SURFACE('',#95840,0.1) ;
#14527=CYLINDRICAL_SURFACE('',#95842,0.1) ;
#14528=CYLINDRICAL_SURFACE('',#95844,0.1) ;
#14529=CYLINDRICAL_SURFACE('',#95855,0.1) ;
#14530=CYLINDRICAL_SURFACE('',#95857,0.0999999999999998) ;
#14531=CYLINDRICAL_SURFACE('',#95859,0.1) ;
#14532=CYLINDRICAL_SURFACE('',#95861,0.1) ;
#14533=CYLINDRICAL_SURFACE('',#95863,0.1) ;
#14534=CYLINDRICAL_SURFACE('',#95873,0.1) ;
#14535=CYLINDRICAL_SURFACE('',#95880,0.1) ;
#14536=CYLINDRICAL_SURFACE('',#95882,0.1) ;
#14537=CYLINDRICAL_SURFACE('',#95884,0.0999999999999994) ;
#14538=CYLINDRICAL_SURFACE('',#95888,0.1) ;
#14539=CYLINDRICAL_SURFACE('',#95890,0.1) ;
#14540=CYLINDRICAL_SURFACE('',#95892,0.0999999999999998) ;
#14541=CYLINDRICAL_SURFACE('',#95899,0.1) ;
#14542=CYLINDRICAL_SURFACE('',#95906,0.1) ;
#14543=CYLINDRICAL_SURFACE('',#95908,0.1) ;
#14544=CYLINDRICAL_SURFACE('',#95912,0.1) ;
#14545=CYLINDRICAL_SURFACE('',#95915,0.1) ;
#14546=CYLINDRICAL_SURFACE('',#95917,0.0999999999999994) ;
#14547=CYLINDRICAL_SURFACE('',#95920,0.1) ;
#14548=CYLINDRICAL_SURFACE('',#95927,0.0999999999999994) ;
#14549=CYLINDRICAL_SURFACE('',#95929,0.0999999999999994) ;
#14550=CYLINDRICAL_SURFACE('',#95935,0.1) ;
#14551=CYLINDRICAL_SURFACE('',#95937,0.1) ;
#14552=CYLINDRICAL_SURFACE('',#95943,0.1) ;
#14553=CYLINDRICAL_SURFACE('',#95951,0.1) ;
#14554=CYLINDRICAL_SURFACE('',#95952,0.1) ;
#14555=CYLINDRICAL_SURFACE('',#95956,0.1) ;
#14556=CYLINDRICAL_SURFACE('',#95958,0.0999999999999994) ;
#14557=CYLINDRICAL_SURFACE('',#95964,0.0999999999999998) ;
#14558=CYLINDRICAL_SURFACE('',#95966,0.1) ;
#14559=CYLINDRICAL_SURFACE('',#95972,0.0999999999999994) ;
#14560=CYLINDRICAL_SURFACE('',#95973,0.1) ;
#14561=CYLINDRICAL_SURFACE('',#95976,0.1) ;
#14562=CYLINDRICAL_SURFACE('',#95987,0.1) ;
#14563=CYLINDRICAL_SURFACE('',#95989,0.1) ;
#14564=CYLINDRICAL_SURFACE('',#95991,0.1) ;
#14565=CYLINDRICAL_SURFACE('',#95993,0.1) ;
#14566=CYLINDRICAL_SURFACE('',#95995,0.1) ;
#14567=CYLINDRICAL_SURFACE('',#95997,0.1) ;
#14568=CYLINDRICAL_SURFACE('',#96008,0.1) ;
#14569=CYLINDRICAL_SURFACE('',#96010,0.0999999999999998) ;
#14570=CYLINDRICAL_SURFACE('',#96012,0.1) ;
#14571=CYLINDRICAL_SURFACE('',#96014,0.1) ;
#14572=CYLINDRICAL_SURFACE('',#96016,0.1) ;
#14573=CYLINDRICAL_SURFACE('',#96026,0.1) ;
#14574=CYLINDRICAL_SURFACE('',#96033,0.1) ;
#14575=CYLINDRICAL_SURFACE('',#96035,0.1) ;
#14576=CYLINDRICAL_SURFACE('',#96037,0.0999999999999994) ;
#14577=CYLINDRICAL_SURFACE('',#96041,0.1) ;
#14578=CYLINDRICAL_SURFACE('',#96043,0.1) ;
#14579=CYLINDRICAL_SURFACE('',#96045,0.0999999999999998) ;
#14580=CYLINDRICAL_SURFACE('',#96052,0.1) ;
#14581=CYLINDRICAL_SURFACE('',#96059,0.1) ;
#14582=CYLINDRICAL_SURFACE('',#96061,0.1) ;
#14583=CYLINDRICAL_SURFACE('',#96065,0.1) ;
#14584=CYLINDRICAL_SURFACE('',#96068,0.1) ;
#14585=CYLINDRICAL_SURFACE('',#96070,0.0999999999999994) ;
#14586=CYLINDRICAL_SURFACE('',#96073,0.1) ;
#14587=CYLINDRICAL_SURFACE('',#96080,0.0999999999999994) ;
#14588=CYLINDRICAL_SURFACE('',#96082,0.0999999999999994) ;
#14589=CYLINDRICAL_SURFACE('',#96088,0.1) ;
#14590=CYLINDRICAL_SURFACE('',#96090,0.1) ;
#14591=CYLINDRICAL_SURFACE('',#96096,0.1) ;
#14592=CYLINDRICAL_SURFACE('',#96104,0.1) ;
#14593=CYLINDRICAL_SURFACE('',#96105,0.1) ;
#14594=CYLINDRICAL_SURFACE('',#96109,0.1) ;
#14595=CYLINDRICAL_SURFACE('',#96111,0.0999999999999994) ;
#14596=CYLINDRICAL_SURFACE('',#96117,0.0999999999999998) ;
#14597=CYLINDRICAL_SURFACE('',#96119,0.1) ;
#14598=CYLINDRICAL_SURFACE('',#96125,0.0999999999999994) ;
#14599=CYLINDRICAL_SURFACE('',#96126,0.1) ;
#14600=CYLINDRICAL_SURFACE('',#96129,0.1) ;
#14601=CYLINDRICAL_SURFACE('',#96140,0.1) ;
#14602=CYLINDRICAL_SURFACE('',#96142,0.1) ;
#14603=CYLINDRICAL_SURFACE('',#96144,0.1) ;
#14604=CYLINDRICAL_SURFACE('',#96146,0.1) ;
#14605=CYLINDRICAL_SURFACE('',#96148,0.1) ;
#14606=CYLINDRICAL_SURFACE('',#96150,0.1) ;
#14607=CYLINDRICAL_SURFACE('',#96161,0.1) ;
#14608=CYLINDRICAL_SURFACE('',#96163,0.0999999999999998) ;
#14609=CYLINDRICAL_SURFACE('',#96165,0.1) ;
#14610=CYLINDRICAL_SURFACE('',#96167,0.1) ;
#14611=CYLINDRICAL_SURFACE('',#96169,0.1) ;
#14612=CYLINDRICAL_SURFACE('',#96179,0.1) ;
#14613=CYLINDRICAL_SURFACE('',#96186,0.1) ;
#14614=CYLINDRICAL_SURFACE('',#96188,0.1) ;
#14615=CYLINDRICAL_SURFACE('',#96190,0.0999999999999994) ;
#14616=CYLINDRICAL_SURFACE('',#96194,0.1) ;
#14617=CYLINDRICAL_SURFACE('',#96196,0.1) ;
#14618=CYLINDRICAL_SURFACE('',#96198,0.0999999999999998) ;
#14619=CYLINDRICAL_SURFACE('',#96205,0.1) ;
#14620=CYLINDRICAL_SURFACE('',#96212,0.1) ;
#14621=CYLINDRICAL_SURFACE('',#96214,0.1) ;
#14622=CYLINDRICAL_SURFACE('',#96218,0.1) ;
#14623=CYLINDRICAL_SURFACE('',#96221,0.1) ;
#14624=CYLINDRICAL_SURFACE('',#96223,0.0999999999999994) ;
#14625=CYLINDRICAL_SURFACE('',#96226,0.1) ;
#14626=CYLINDRICAL_SURFACE('',#96233,0.0999999999999994) ;
#14627=CYLINDRICAL_SURFACE('',#96235,0.0999999999999994) ;
#14628=CYLINDRICAL_SURFACE('',#96241,0.1) ;
#14629=CYLINDRICAL_SURFACE('',#96243,0.1) ;
#14630=CYLINDRICAL_SURFACE('',#96249,0.0999999999999988) ;
#14631=CYLINDRICAL_SURFACE('',#96257,0.1) ;
#14632=CYLINDRICAL_SURFACE('',#96258,0.1) ;
#14633=CYLINDRICAL_SURFACE('',#96262,0.0999999999999989) ;
#14634=CYLINDRICAL_SURFACE('',#96264,0.0999999999999994) ;
#14635=CYLINDRICAL_SURFACE('',#96270,0.0999999999999998) ;
#14636=CYLINDRICAL_SURFACE('',#96272,0.1) ;
#14637=CYLINDRICAL_SURFACE('',#96278,0.0999999999999994) ;
#14638=CYLINDRICAL_SURFACE('',#96279,0.1) ;
#14639=CYLINDRICAL_SURFACE('',#96282,0.1) ;
#14640=CYLINDRICAL_SURFACE('',#96293,0.1) ;
#14641=CYLINDRICAL_SURFACE('',#96295,0.1) ;
#14642=CYLINDRICAL_SURFACE('',#96297,0.1) ;
#14643=CYLINDRICAL_SURFACE('',#96299,0.1) ;
#14644=CYLINDRICAL_SURFACE('',#96301,0.1) ;
#14645=CYLINDRICAL_SURFACE('',#96303,0.1) ;
#14646=CYLINDRICAL_SURFACE('',#96314,0.1) ;
#14647=CYLINDRICAL_SURFACE('',#96316,0.0999999999999998) ;
#14648=CYLINDRICAL_SURFACE('',#96318,0.1) ;
#14649=CYLINDRICAL_SURFACE('',#96320,0.1) ;
#14650=CYLINDRICAL_SURFACE('',#96322,0.1) ;
#14651=CYLINDRICAL_SURFACE('',#96332,0.1) ;
#14652=CYLINDRICAL_SURFACE('',#96339,0.1) ;
#14653=CYLINDRICAL_SURFACE('',#96341,0.1) ;
#14654=CYLINDRICAL_SURFACE('',#96343,0.0999999999999994) ;
#14655=CYLINDRICAL_SURFACE('',#96347,0.1) ;
#14656=CYLINDRICAL_SURFACE('',#96349,0.1) ;
#14657=CYLINDRICAL_SURFACE('',#96351,0.0999999999999998) ;
#14658=CYLINDRICAL_SURFACE('',#96358,0.1) ;
#14659=CYLINDRICAL_SURFACE('',#96365,0.1) ;
#14660=CYLINDRICAL_SURFACE('',#96367,0.1) ;
#14661=CYLINDRICAL_SURFACE('',#96371,0.1) ;
#14662=CYLINDRICAL_SURFACE('',#96374,0.1) ;
#14663=CYLINDRICAL_SURFACE('',#96376,0.0999999999999994) ;
#14664=CYLINDRICAL_SURFACE('',#96379,0.1) ;
#14665=CYLINDRICAL_SURFACE('',#96386,0.0999999999999994) ;
#14666=CYLINDRICAL_SURFACE('',#96388,0.0999999999999994) ;
#14667=CYLINDRICAL_SURFACE('',#96394,0.1) ;
#14668=CYLINDRICAL_SURFACE('',#96396,0.1) ;
#14669=CYLINDRICAL_SURFACE('',#96402,0.0999999999999988) ;
#14670=CYLINDRICAL_SURFACE('',#96410,0.1) ;
#14671=CYLINDRICAL_SURFACE('',#96411,0.1) ;
#14672=CYLINDRICAL_SURFACE('',#96415,0.0999999999999989) ;
#14673=CYLINDRICAL_SURFACE('',#96417,0.0999999999999994) ;
#14674=CYLINDRICAL_SURFACE('',#96423,0.0999999999999998) ;
#14675=CYLINDRICAL_SURFACE('',#96425,0.1) ;
#14676=CYLINDRICAL_SURFACE('',#96431,0.0999999999999994) ;
#14677=CYLINDRICAL_SURFACE('',#96432,0.1) ;
#14678=CYLINDRICAL_SURFACE('',#96435,0.1) ;
#14679=CYLINDRICAL_SURFACE('',#96446,0.1) ;
#14680=CYLINDRICAL_SURFACE('',#96448,0.1) ;
#14681=CYLINDRICAL_SURFACE('',#96450,0.1) ;
#14682=CYLINDRICAL_SURFACE('',#96452,0.1) ;
#14683=CYLINDRICAL_SURFACE('',#96454,0.1) ;
#14684=CYLINDRICAL_SURFACE('',#96456,0.1) ;
#14685=CYLINDRICAL_SURFACE('',#96467,0.1) ;
#14686=CYLINDRICAL_SURFACE('',#96469,0.0999999999999998) ;
#14687=CYLINDRICAL_SURFACE('',#96471,0.1) ;
#14688=CYLINDRICAL_SURFACE('',#96473,0.1) ;
#14689=CYLINDRICAL_SURFACE('',#96475,0.1) ;
#14690=CYLINDRICAL_SURFACE('',#96485,0.1) ;
#14691=CYLINDRICAL_SURFACE('',#96492,0.1) ;
#14692=CYLINDRICAL_SURFACE('',#96494,0.1) ;
#14693=CYLINDRICAL_SURFACE('',#96496,0.0999999999999994) ;
#14694=CYLINDRICAL_SURFACE('',#96500,0.1) ;
#14695=CYLINDRICAL_SURFACE('',#96502,0.1) ;
#14696=CYLINDRICAL_SURFACE('',#96504,0.0999999999999998) ;
#14697=CYLINDRICAL_SURFACE('',#96511,0.1) ;
#14698=CYLINDRICAL_SURFACE('',#96518,0.1) ;
#14699=CYLINDRICAL_SURFACE('',#96520,0.1) ;
#14700=CYLINDRICAL_SURFACE('',#96524,0.1) ;
#14701=CYLINDRICAL_SURFACE('',#96527,0.1) ;
#14702=CYLINDRICAL_SURFACE('',#96529,0.0999999999999994) ;
#14703=CYLINDRICAL_SURFACE('',#96532,0.1) ;
#14704=CYLINDRICAL_SURFACE('',#96539,0.0999999999999994) ;
#14705=CYLINDRICAL_SURFACE('',#96541,0.0999999999999994) ;
#14706=CYLINDRICAL_SURFACE('',#96547,0.1) ;
#14707=CYLINDRICAL_SURFACE('',#96549,0.1) ;
#14708=CYLINDRICAL_SURFACE('',#96555,0.0999999999999988) ;
#14709=CYLINDRICAL_SURFACE('',#96563,0.1) ;
#14710=CYLINDRICAL_SURFACE('',#96564,0.1) ;
#14711=CYLINDRICAL_SURFACE('',#96568,0.0999999999999989) ;
#14712=CYLINDRICAL_SURFACE('',#96570,0.0999999999999994) ;
#14713=CYLINDRICAL_SURFACE('',#96576,0.0999999999999998) ;
#14714=CYLINDRICAL_SURFACE('',#96578,0.1) ;
#14715=CYLINDRICAL_SURFACE('',#96584,0.0999999999999994) ;
#14716=CYLINDRICAL_SURFACE('',#96585,0.1) ;
#14717=CYLINDRICAL_SURFACE('',#96588,0.1) ;
#14718=CYLINDRICAL_SURFACE('',#96599,0.1) ;
#14719=CYLINDRICAL_SURFACE('',#96601,0.1) ;
#14720=CYLINDRICAL_SURFACE('',#96603,0.1) ;
#14721=CYLINDRICAL_SURFACE('',#96605,0.1) ;
#14722=CYLINDRICAL_SURFACE('',#96607,0.1) ;
#14723=CYLINDRICAL_SURFACE('',#96609,0.1) ;
#14724=CYLINDRICAL_SURFACE('',#96620,0.1) ;
#14725=CYLINDRICAL_SURFACE('',#96622,0.0999999999999998) ;
#14726=CYLINDRICAL_SURFACE('',#96624,0.1) ;
#14727=CYLINDRICAL_SURFACE('',#96626,0.1) ;
#14728=CYLINDRICAL_SURFACE('',#96628,0.1) ;
#14729=CYLINDRICAL_SURFACE('',#96638,0.1) ;
#14730=CYLINDRICAL_SURFACE('',#96645,0.1) ;
#14731=CYLINDRICAL_SURFACE('',#96647,0.1) ;
#14732=CYLINDRICAL_SURFACE('',#96649,0.0999999999999994) ;
#14733=CYLINDRICAL_SURFACE('',#96653,0.1) ;
#14734=CYLINDRICAL_SURFACE('',#96655,0.1) ;
#14735=CYLINDRICAL_SURFACE('',#96657,0.0999999999999998) ;
#14736=CYLINDRICAL_SURFACE('',#96664,0.1) ;
#14737=CYLINDRICAL_SURFACE('',#96671,0.1) ;
#14738=CYLINDRICAL_SURFACE('',#96673,0.1) ;
#14739=CYLINDRICAL_SURFACE('',#96677,0.1) ;
#14740=CYLINDRICAL_SURFACE('',#96680,0.1) ;
#14741=CYLINDRICAL_SURFACE('',#96682,0.100000000000003) ;
#14742=CYLINDRICAL_SURFACE('',#96685,0.1) ;
#14743=CYLINDRICAL_SURFACE('',#96692,0.0999999999999994) ;
#14744=CYLINDRICAL_SURFACE('',#96694,0.100000000000003) ;
#14745=CYLINDRICAL_SURFACE('',#96700,0.1) ;
#14746=CYLINDRICAL_SURFACE('',#96702,0.1) ;
#14747=CYLINDRICAL_SURFACE('',#96708,0.0999999999999988) ;
#14748=CYLINDRICAL_SURFACE('',#96716,0.1) ;
#14749=CYLINDRICAL_SURFACE('',#96717,0.1) ;
#14750=CYLINDRICAL_SURFACE('',#96721,0.0999999999999989) ;
#14751=CYLINDRICAL_SURFACE('',#96723,0.0999999999999994) ;
#14752=CYLINDRICAL_SURFACE('',#96729,0.0999999999999998) ;
#14753=CYLINDRICAL_SURFACE('',#96731,0.1) ;
#14754=CYLINDRICAL_SURFACE('',#96737,0.0999999999999994) ;
#14755=CYLINDRICAL_SURFACE('',#96738,0.1) ;
#14756=CYLINDRICAL_SURFACE('',#96741,0.1) ;
#14757=CYLINDRICAL_SURFACE('',#96752,0.1) ;
#14758=CYLINDRICAL_SURFACE('',#96754,0.1) ;
#14759=CYLINDRICAL_SURFACE('',#96756,0.1) ;
#14760=CYLINDRICAL_SURFACE('',#96758,0.1) ;
#14761=CYLINDRICAL_SURFACE('',#96760,0.1) ;
#14762=CYLINDRICAL_SURFACE('',#96762,0.1) ;
#14763=CYLINDRICAL_SURFACE('',#96773,0.1) ;
#14764=CYLINDRICAL_SURFACE('',#96775,0.0999999999999998) ;
#14765=CYLINDRICAL_SURFACE('',#96777,0.1) ;
#14766=CYLINDRICAL_SURFACE('',#96779,0.1) ;
#14767=CYLINDRICAL_SURFACE('',#96781,0.1) ;
#14768=CYLINDRICAL_SURFACE('',#96791,0.1) ;
#14769=CYLINDRICAL_SURFACE('',#96798,0.1) ;
#14770=CYLINDRICAL_SURFACE('',#96800,0.1) ;
#14771=CYLINDRICAL_SURFACE('',#96802,0.100000000000003) ;
#14772=CYLINDRICAL_SURFACE('',#96806,0.1) ;
#14773=CYLINDRICAL_SURFACE('',#96808,0.1) ;
#14774=CYLINDRICAL_SURFACE('',#96810,0.0999999999999998) ;
#14775=CYLINDRICAL_SURFACE('',#96817,0.1) ;
#14776=CYLINDRICAL_SURFACE('',#96824,0.1) ;
#14777=CYLINDRICAL_SURFACE('',#96826,0.1) ;
#14778=CYLINDRICAL_SURFACE('',#96830,0.1) ;
#14779=CYLINDRICAL_SURFACE('',#96833,0.1) ;
#14780=CYLINDRICAL_SURFACE('',#96835,0.100000000000003) ;
#14781=CYLINDRICAL_SURFACE('',#96838,0.1) ;
#14782=CYLINDRICAL_SURFACE('',#96845,0.100000000000003) ;
#14783=CYLINDRICAL_SURFACE('',#96847,0.100000000000003) ;
#14784=CYLINDRICAL_SURFACE('',#96853,0.1) ;
#14785=CYLINDRICAL_SURFACE('',#96855,0.1) ;
#14786=CYLINDRICAL_SURFACE('',#96861,0.0999999999999988) ;
#14787=CYLINDRICAL_SURFACE('',#96869,0.1) ;
#14788=CYLINDRICAL_SURFACE('',#96870,0.1) ;
#14789=CYLINDRICAL_SURFACE('',#96874,0.0999999999999989) ;
#14790=CYLINDRICAL_SURFACE('',#96876,0.100000000000003) ;
#14791=CYLINDRICAL_SURFACE('',#96882,0.0999999999999998) ;
#14792=CYLINDRICAL_SURFACE('',#96884,0.1) ;
#14793=CYLINDRICAL_SURFACE('',#96890,0.100000000000003) ;
#14794=CYLINDRICAL_SURFACE('',#96902,1.) ;
#14795=CYLINDRICAL_SURFACE('',#96905,0.2) ;
#14796=CYLINDRICAL_SURFACE('',#96926,1.) ;
#14797=CYLINDRICAL_SURFACE('',#96929,0.2) ;
#14798=CYLINDRICAL_SURFACE('',#96950,1.) ;
#14799=CYLINDRICAL_SURFACE('',#96953,0.2) ;
#14800=CYLINDRICAL_SURFACE('',#96974,1.) ;
#14801=CYLINDRICAL_SURFACE('',#96977,0.2) ;
#14802=CYLINDRICAL_SURFACE('',#96998,1.) ;
#14803=CYLINDRICAL_SURFACE('',#97001,0.2) ;
#14804=CYLINDRICAL_SURFACE('',#97022,1.) ;
#14805=CYLINDRICAL_SURFACE('',#97025,0.2) ;
#14806=CYLINDRICAL_SURFACE('',#97046,1.) ;
#14807=CYLINDRICAL_SURFACE('',#97049,0.2) ;
#14808=CYLINDRICAL_SURFACE('',#97070,1.) ;
#14809=CYLINDRICAL_SURFACE('',#97073,0.2) ;
#14810=CYLINDRICAL_SURFACE('',#97094,1.) ;
#14811=CYLINDRICAL_SURFACE('',#97097,0.2) ;
#14812=CYLINDRICAL_SURFACE('',#97143,0.0999999999999999) ;
#14813=CYLINDRICAL_SURFACE('',#97146,0.1) ;
#14814=CYLINDRICAL_SURFACE('',#97152,0.0999999999999999) ;
#14815=CYLINDRICAL_SURFACE('',#97155,0.1) ;
#14816=CYLINDRICAL_SURFACE('',#97157,0.0999999999999998) ;
#14817=CYLINDRICAL_SURFACE('',#97164,0.0999999999999998) ;
#14818=CYLINDRICAL_SURFACE('',#97166,0.1) ;
#14819=CYLINDRICAL_SURFACE('',#97168,0.1) ;
#14820=CYLINDRICAL_SURFACE('',#97172,0.1) ;
#14821=CYLINDRICAL_SURFACE('',#97175,0.0999999999999999) ;
#14822=CYLINDRICAL_SURFACE('',#97177,0.1) ;
#14823=CYLINDRICAL_SURFACE('',#97180,0.1) ;
#14824=CYLINDRICAL_SURFACE('',#97186,0.1) ;
#14825=CYLINDRICAL_SURFACE('',#97189,0.1) ;
#14826=CYLINDRICAL_SURFACE('',#97191,0.0999999999999998) ;
#14827=CYLINDRICAL_SURFACE('',#97198,0.0999999999999998) ;
#14828=CYLINDRICAL_SURFACE('',#97200,0.1) ;
#14829=CYLINDRICAL_SURFACE('',#97202,0.1) ;
#14830=CYLINDRICAL_SURFACE('',#97206,0.1) ;
#14831=CYLINDRICAL_SURFACE('',#97209,0.1) ;
#14832=CYLINDRICAL_SURFACE('',#97211,0.1) ;
#14833=CYLINDRICAL_SURFACE('',#97214,0.1) ;
#14834=CYLINDRICAL_SURFACE('',#97220,0.1) ;
#14835=CYLINDRICAL_SURFACE('',#97223,0.1) ;
#14836=CYLINDRICAL_SURFACE('',#97225,0.1) ;
#14837=CYLINDRICAL_SURFACE('',#97232,0.1) ;
#14838=CYLINDRICAL_SURFACE('',#97234,0.1) ;
#14839=CYLINDRICAL_SURFACE('',#97236,0.1) ;
#14840=CYLINDRICAL_SURFACE('',#97240,0.1) ;
#14841=CYLINDRICAL_SURFACE('',#97243,0.1) ;
#14842=CYLINDRICAL_SURFACE('',#97245,0.1) ;
#14843=CYLINDRICAL_SURFACE('',#97248,0.1) ;
#14844=CYLINDRICAL_SURFACE('',#97254,0.1) ;
#14845=CYLINDRICAL_SURFACE('',#97257,0.1) ;
#14846=CYLINDRICAL_SURFACE('',#97259,0.1) ;
#14847=CYLINDRICAL_SURFACE('',#97266,0.1) ;
#14848=CYLINDRICAL_SURFACE('',#97268,0.1) ;
#14849=CYLINDRICAL_SURFACE('',#97270,0.1) ;
#14850=CYLINDRICAL_SURFACE('',#97274,0.1) ;
#14851=CYLINDRICAL_SURFACE('',#97277,0.1) ;
#14852=CYLINDRICAL_SURFACE('',#97279,0.1) ;
#14853=CYLINDRICAL_SURFACE('',#97282,0.1) ;
#14854=CYLINDRICAL_SURFACE('',#97288,0.1) ;
#14855=CYLINDRICAL_SURFACE('',#97291,0.1) ;
#14856=CYLINDRICAL_SURFACE('',#97293,0.0999999999999994) ;
#14857=CYLINDRICAL_SURFACE('',#97300,0.0999999999999994) ;
#14858=CYLINDRICAL_SURFACE('',#97302,0.1) ;
#14859=CYLINDRICAL_SURFACE('',#97304,0.1) ;
#14860=CYLINDRICAL_SURFACE('',#97308,0.1) ;
#14861=CYLINDRICAL_SURFACE('',#97311,0.1) ;
#14862=CYLINDRICAL_SURFACE('',#97313,0.1) ;
#14863=CYLINDRICAL_SURFACE('',#97316,0.1) ;
#14864=CYLINDRICAL_SURFACE('',#97322,0.1) ;
#14865=CYLINDRICAL_SURFACE('',#97325,0.1) ;
#14866=CYLINDRICAL_SURFACE('',#97327,0.0999999999999994) ;
#14867=CYLINDRICAL_SURFACE('',#97334,0.0999999999999994) ;
#14868=CYLINDRICAL_SURFACE('',#97336,0.1) ;
#14869=CYLINDRICAL_SURFACE('',#97338,0.1) ;
#14870=CYLINDRICAL_SURFACE('',#97342,0.1) ;
#14871=CYLINDRICAL_SURFACE('',#97345,0.1) ;
#14872=CYLINDRICAL_SURFACE('',#97347,0.1) ;
#14873=CYLINDRICAL_SURFACE('',#97350,0.1) ;
#14874=CYLINDRICAL_SURFACE('',#97356,0.1) ;
#14875=CYLINDRICAL_SURFACE('',#97359,0.1) ;
#14876=CYLINDRICAL_SURFACE('',#97361,0.0999999999999994) ;
#14877=CYLINDRICAL_SURFACE('',#97368,0.0999999999999994) ;
#14878=CYLINDRICAL_SURFACE('',#97370,0.1) ;
#14879=CYLINDRICAL_SURFACE('',#97372,0.1) ;
#14880=CYLINDRICAL_SURFACE('',#97376,0.1) ;
#14881=CYLINDRICAL_SURFACE('',#97379,0.1) ;
#14882=CYLINDRICAL_SURFACE('',#97381,0.1) ;
#14883=CYLINDRICAL_SURFACE('',#97384,0.1) ;
#14884=CYLINDRICAL_SURFACE('',#97390,0.1) ;
#14885=CYLINDRICAL_SURFACE('',#97393,0.1) ;
#14886=CYLINDRICAL_SURFACE('',#97395,0.0999999999999994) ;
#14887=CYLINDRICAL_SURFACE('',#97402,0.0999999999999994) ;
#14888=CYLINDRICAL_SURFACE('',#97404,0.1) ;
#14889=CYLINDRICAL_SURFACE('',#97406,0.1) ;
#14890=CYLINDRICAL_SURFACE('',#97410,0.1) ;
#14891=CYLINDRICAL_SURFACE('',#97413,0.1) ;
#14892=CYLINDRICAL_SURFACE('',#97415,0.099999999999999) ;
#14893=CYLINDRICAL_SURFACE('',#97418,0.1) ;
#14894=CYLINDRICAL_SURFACE('',#97424,0.099999999999999) ;
#14895=CYLINDRICAL_SURFACE('',#97427,0.1) ;
#14896=CYLINDRICAL_SURFACE('',#97429,0.0999999999999994) ;
#14897=CYLINDRICAL_SURFACE('',#97436,0.0999999999999994) ;
#14898=CYLINDRICAL_SURFACE('',#97438,0.1) ;
#14899=CYLINDRICAL_SURFACE('',#97440,0.099999999999999) ;
#14900=CYLINDRICAL_SURFACE('',#97444,0.1) ;
#14901=CYLINDRICAL_SURFACE('',#97447,0.099999999999999) ;
#14902=CYLINDRICAL_SURFACE('',#97449,0.0999999999999989) ;
#14903=CYLINDRICAL_SURFACE('',#97452,0.1) ;
#14904=CYLINDRICAL_SURFACE('',#97458,0.0999999999999989) ;
#14905=CYLINDRICAL_SURFACE('',#97461,0.1) ;
#14906=CYLINDRICAL_SURFACE('',#97463,0.0999999999999994) ;
#14907=CYLINDRICAL_SURFACE('',#97470,0.0999999999999994) ;
#14908=CYLINDRICAL_SURFACE('',#97472,0.1) ;
#14909=CYLINDRICAL_SURFACE('',#97474,0.0999999999999989) ;
#14910=CYLINDRICAL_SURFACE('',#97478,0.1) ;
#14911=CYLINDRICAL_SURFACE('',#97481,0.0999999999999989) ;
#14912=CYLINDRICAL_SURFACE('',#97483,0.099999999999999) ;
#14913=CYLINDRICAL_SURFACE('',#97486,0.1) ;
#14914=CYLINDRICAL_SURFACE('',#97492,0.099999999999999) ;
#14915=CYLINDRICAL_SURFACE('',#97495,0.1) ;
#14916=CYLINDRICAL_SURFACE('',#97497,0.0999999999999994) ;
#14917=CYLINDRICAL_SURFACE('',#97504,0.0999999999999994) ;
#14918=CYLINDRICAL_SURFACE('',#97506,0.1) ;
#14919=CYLINDRICAL_SURFACE('',#97508,0.099999999999999) ;
#14920=CYLINDRICAL_SURFACE('',#97512,0.1) ;
#14921=CYLINDRICAL_SURFACE('',#97515,0.099999999999999) ;
#14922=CYLINDRICAL_SURFACE('',#97517,0.0999999999999989) ;
#14923=CYLINDRICAL_SURFACE('',#97520,0.1) ;
#14924=CYLINDRICAL_SURFACE('',#97526,0.0999999999999989) ;
#14925=CYLINDRICAL_SURFACE('',#97529,0.1) ;
#14926=CYLINDRICAL_SURFACE('',#97531,0.0999999999999994) ;
#14927=CYLINDRICAL_SURFACE('',#97538,0.0999999999999994) ;
#14928=CYLINDRICAL_SURFACE('',#97540,0.1) ;
#14929=CYLINDRICAL_SURFACE('',#97542,0.0999999999999989) ;
#14930=CYLINDRICAL_SURFACE('',#97546,0.1) ;
#14931=CYLINDRICAL_SURFACE('',#97549,0.0999999999999989) ;
#14932=CYLINDRICAL_SURFACE('',#97551,0.099999999999999) ;
#14933=CYLINDRICAL_SURFACE('',#97554,0.1) ;
#14934=CYLINDRICAL_SURFACE('',#97560,0.099999999999999) ;
#14935=CYLINDRICAL_SURFACE('',#97563,0.1) ;
#14936=CYLINDRICAL_SURFACE('',#97565,0.0999999999999994) ;
#14937=CYLINDRICAL_SURFACE('',#97572,0.0999999999999994) ;
#14938=CYLINDRICAL_SURFACE('',#97574,0.1) ;
#14939=CYLINDRICAL_SURFACE('',#97576,0.099999999999999) ;
#14940=CYLINDRICAL_SURFACE('',#97580,0.1) ;
#14941=CYLINDRICAL_SURFACE('',#97583,0.099999999999999) ;
#14942=CYLINDRICAL_SURFACE('',#97585,0.0999999999999989) ;
#14943=CYLINDRICAL_SURFACE('',#97588,0.1) ;
#14944=CYLINDRICAL_SURFACE('',#97594,0.0999999999999989) ;
#14945=CYLINDRICAL_SURFACE('',#97597,0.1) ;
#14946=CYLINDRICAL_SURFACE('',#97599,0.0999999999999994) ;
#14947=CYLINDRICAL_SURFACE('',#97606,0.0999999999999994) ;
#14948=CYLINDRICAL_SURFACE('',#97608,0.1) ;
#14949=CYLINDRICAL_SURFACE('',#97610,0.0999999999999989) ;
#14950=CYLINDRICAL_SURFACE('',#97614,0.1) ;
#14951=CYLINDRICAL_SURFACE('',#97617,0.0999999999999989) ;
#14952=CYLINDRICAL_SURFACE('',#97619,0.099999999999999) ;
#14953=CYLINDRICAL_SURFACE('',#97622,0.1) ;
#14954=CYLINDRICAL_SURFACE('',#97628,0.099999999999999) ;
#14955=CYLINDRICAL_SURFACE('',#97631,0.1) ;
#14956=CYLINDRICAL_SURFACE('',#97633,0.0999999999999994) ;
#14957=CYLINDRICAL_SURFACE('',#97640,0.0999999999999994) ;
#14958=CYLINDRICAL_SURFACE('',#97642,0.1) ;
#14959=CYLINDRICAL_SURFACE('',#97644,0.099999999999999) ;
#14960=CYLINDRICAL_SURFACE('',#97648,0.1) ;
#14961=CYLINDRICAL_SURFACE('',#97651,0.099999999999999) ;
#14962=CYLINDRICAL_SURFACE('',#97653,0.0999999999999989) ;
#14963=CYLINDRICAL_SURFACE('',#97656,0.1) ;
#14964=CYLINDRICAL_SURFACE('',#97662,0.0999999999999989) ;
#14965=CYLINDRICAL_SURFACE('',#97665,0.1) ;
#14966=CYLINDRICAL_SURFACE('',#97667,0.0999999999999994) ;
#14967=CYLINDRICAL_SURFACE('',#97674,0.0999999999999994) ;
#14968=CYLINDRICAL_SURFACE('',#97676,0.1) ;
#14969=CYLINDRICAL_SURFACE('',#97678,0.0999999999999989) ;
#14970=CYLINDRICAL_SURFACE('',#97682,0.1) ;
#14971=CYLINDRICAL_SURFACE('',#97685,0.0999999999999989) ;
#14972=CYLINDRICAL_SURFACE('',#97687,0.099999999999999) ;
#14973=CYLINDRICAL_SURFACE('',#97690,0.1) ;
#14974=CYLINDRICAL_SURFACE('',#97696,0.099999999999999) ;
#14975=CYLINDRICAL_SURFACE('',#97699,0.1) ;
#14976=CYLINDRICAL_SURFACE('',#97701,0.100000000000003) ;
#14977=CYLINDRICAL_SURFACE('',#97708,0.100000000000003) ;
#14978=CYLINDRICAL_SURFACE('',#97710,0.1) ;
#14979=CYLINDRICAL_SURFACE('',#97712,0.099999999999999) ;
#14980=CYLINDRICAL_SURFACE('',#97716,0.1) ;
#14981=CYLINDRICAL_SURFACE('',#97719,0.099999999999999) ;
#14982=CYLINDRICAL_SURFACE('',#97721,0.0999999999999989) ;
#14983=CYLINDRICAL_SURFACE('',#97724,0.1) ;
#14984=CYLINDRICAL_SURFACE('',#97730,0.0999999999999989) ;
#14985=CYLINDRICAL_SURFACE('',#97733,0.1) ;
#14986=CYLINDRICAL_SURFACE('',#97735,0.100000000000003) ;
#14987=CYLINDRICAL_SURFACE('',#97742,0.100000000000003) ;
#14988=CYLINDRICAL_SURFACE('',#97744,0.1) ;
#14989=CYLINDRICAL_SURFACE('',#97746,0.0999999999999989) ;
#14990=CYLINDRICAL_SURFACE('',#97750,0.1) ;
#14991=CYLINDRICAL_SURFACE('',#97753,0.0999999999999989) ;
#14992=CYLINDRICAL_SURFACE('',#97757,0.1) ;
#14993=CYLINDRICAL_SURFACE('',#97761,0.1) ;
#14994=CYLINDRICAL_SURFACE('',#97765,0.1) ;
#14995=CYLINDRICAL_SURFACE('',#97770,0.1) ;
#14996=CYLINDRICAL_SURFACE('',#97774,0.1) ;
#14997=CYLINDRICAL_SURFACE('',#97778,0.1) ;
#14998=CYLINDRICAL_SURFACE('',#97781,0.1) ;
#14999=CYLINDRICAL_SURFACE('',#97785,0.1) ;
#15000=CYLINDRICAL_SURFACE('',#97789,0.1) ;
#15001=CYLINDRICAL_SURFACE('',#97790,0.1) ;
#15002=CYLINDRICAL_SURFACE('',#97794,0.1) ;
#15003=CYLINDRICAL_SURFACE('',#97796,0.1) ;
#15004=CYLINDRICAL_SURFACE('',#97801,0.1) ;
#15005=CYLINDRICAL_SURFACE('',#97805,0.1) ;
#15006=CYLINDRICAL_SURFACE('',#97809,0.1) ;
#15007=CYLINDRICAL_SURFACE('',#97814,0.1) ;
#15008=CYLINDRICAL_SURFACE('',#97818,0.1) ;
#15009=CYLINDRICAL_SURFACE('',#97822,0.1) ;
#15010=CYLINDRICAL_SURFACE('',#97825,0.1) ;
#15011=CYLINDRICAL_SURFACE('',#97829,0.1) ;
#15012=CYLINDRICAL_SURFACE('',#97833,0.1) ;
#15013=CYLINDRICAL_SURFACE('',#97834,0.1) ;
#15014=CYLINDRICAL_SURFACE('',#97838,0.1) ;
#15015=CYLINDRICAL_SURFACE('',#97840,0.1) ;
#15016=CYLINDRICAL_SURFACE('',#97845,0.1) ;
#15017=CYLINDRICAL_SURFACE('',#97849,0.1) ;
#15018=CYLINDRICAL_SURFACE('',#97853,0.1) ;
#15019=CYLINDRICAL_SURFACE('',#97858,0.1) ;
#15020=CYLINDRICAL_SURFACE('',#97862,0.1) ;
#15021=CYLINDRICAL_SURFACE('',#97866,0.1) ;
#15022=CYLINDRICAL_SURFACE('',#97869,0.1) ;
#15023=CYLINDRICAL_SURFACE('',#97873,0.1) ;
#15024=CYLINDRICAL_SURFACE('',#97877,0.1) ;
#15025=CYLINDRICAL_SURFACE('',#97878,0.1) ;
#15026=CYLINDRICAL_SURFACE('',#97882,0.1) ;
#15027=CYLINDRICAL_SURFACE('',#97884,0.1) ;
#15028=CYLINDRICAL_SURFACE('',#97889,0.1) ;
#15029=CYLINDRICAL_SURFACE('',#97893,0.1) ;
#15030=CYLINDRICAL_SURFACE('',#97897,0.1) ;
#15031=CYLINDRICAL_SURFACE('',#97902,0.1) ;
#15032=CYLINDRICAL_SURFACE('',#97906,0.1) ;
#15033=CYLINDRICAL_SURFACE('',#97910,0.1) ;
#15034=CYLINDRICAL_SURFACE('',#97913,0.1) ;
#15035=CYLINDRICAL_SURFACE('',#97917,0.1) ;
#15036=CYLINDRICAL_SURFACE('',#97921,0.1) ;
#15037=CYLINDRICAL_SURFACE('',#97922,0.1) ;
#15038=CYLINDRICAL_SURFACE('',#97926,0.1) ;
#15039=CYLINDRICAL_SURFACE('',#97928,0.1) ;
#15040=CYLINDRICAL_SURFACE('',#97933,0.1) ;
#15041=CYLINDRICAL_SURFACE('',#97937,0.1) ;
#15042=CYLINDRICAL_SURFACE('',#97941,0.1) ;
#15043=CYLINDRICAL_SURFACE('',#97946,0.1) ;
#15044=CYLINDRICAL_SURFACE('',#97950,0.1) ;
#15045=CYLINDRICAL_SURFACE('',#97954,0.1) ;
#15046=CYLINDRICAL_SURFACE('',#97957,0.1) ;
#15047=CYLINDRICAL_SURFACE('',#97961,0.1) ;
#15048=CYLINDRICAL_SURFACE('',#97965,0.1) ;
#15049=CYLINDRICAL_SURFACE('',#97966,0.1) ;
#15050=CYLINDRICAL_SURFACE('',#97970,0.1) ;
#15051=CYLINDRICAL_SURFACE('',#97972,0.1) ;
#15052=CYLINDRICAL_SURFACE('',#97977,0.1) ;
#15053=CYLINDRICAL_SURFACE('',#97981,0.1) ;
#15054=CYLINDRICAL_SURFACE('',#97985,0.1) ;
#15055=CYLINDRICAL_SURFACE('',#97990,0.1) ;
#15056=CYLINDRICAL_SURFACE('',#97994,0.1) ;
#15057=CYLINDRICAL_SURFACE('',#97998,0.1) ;
#15058=CYLINDRICAL_SURFACE('',#98001,0.1) ;
#15059=CYLINDRICAL_SURFACE('',#98005,0.1) ;
#15060=CYLINDRICAL_SURFACE('',#98009,0.1) ;
#15061=CYLINDRICAL_SURFACE('',#98010,0.1) ;
#15062=CYLINDRICAL_SURFACE('',#98014,0.1) ;
#15063=CYLINDRICAL_SURFACE('',#98016,0.1) ;
#15064=CYLINDRICAL_SURFACE('',#98021,0.1) ;
#15065=CYLINDRICAL_SURFACE('',#98025,0.1) ;
#15066=CYLINDRICAL_SURFACE('',#98029,0.1) ;
#15067=CYLINDRICAL_SURFACE('',#98034,0.1) ;
#15068=CYLINDRICAL_SURFACE('',#98038,0.1) ;
#15069=CYLINDRICAL_SURFACE('',#98042,0.1) ;
#15070=CYLINDRICAL_SURFACE('',#98045,0.1) ;
#15071=CYLINDRICAL_SURFACE('',#98049,0.1) ;
#15072=CYLINDRICAL_SURFACE('',#98053,0.1) ;
#15073=CYLINDRICAL_SURFACE('',#98054,0.1) ;
#15074=CYLINDRICAL_SURFACE('',#98058,0.1) ;
#15075=CYLINDRICAL_SURFACE('',#98060,0.1) ;
#15076=CYLINDRICAL_SURFACE('',#98065,0.1) ;
#15077=CYLINDRICAL_SURFACE('',#98069,0.1) ;
#15078=CYLINDRICAL_SURFACE('',#98073,0.1) ;
#15079=CYLINDRICAL_SURFACE('',#98078,0.1) ;
#15080=CYLINDRICAL_SURFACE('',#98082,0.1) ;
#15081=CYLINDRICAL_SURFACE('',#98086,0.1) ;
#15082=CYLINDRICAL_SURFACE('',#98089,0.1) ;
#15083=CYLINDRICAL_SURFACE('',#98093,0.1) ;
#15084=CYLINDRICAL_SURFACE('',#98097,0.1) ;
#15085=CYLINDRICAL_SURFACE('',#98098,0.1) ;
#15086=CYLINDRICAL_SURFACE('',#98102,0.1) ;
#15087=CYLINDRICAL_SURFACE('',#98104,0.1) ;
#15088=CYLINDRICAL_SURFACE('',#98109,0.1) ;
#15089=CYLINDRICAL_SURFACE('',#98113,0.1) ;
#15090=CYLINDRICAL_SURFACE('',#98117,0.1) ;
#15091=CYLINDRICAL_SURFACE('',#98122,0.1) ;
#15092=CYLINDRICAL_SURFACE('',#98126,0.1) ;
#15093=CYLINDRICAL_SURFACE('',#98130,0.1) ;
#15094=CYLINDRICAL_SURFACE('',#98133,0.1) ;
#15095=CYLINDRICAL_SURFACE('',#98137,0.1) ;
#15096=CYLINDRICAL_SURFACE('',#98141,0.1) ;
#15097=CYLINDRICAL_SURFACE('',#98142,0.1) ;
#15098=CYLINDRICAL_SURFACE('',#98146,0.1) ;
#15099=CYLINDRICAL_SURFACE('',#98148,0.1) ;
#16277=SPHERICAL_SURFACE('',#93358,0.1) ;
#16278=SPHERICAL_SURFACE('',#93375,0.1) ;
#16279=SPHERICAL_SURFACE('',#93392,0.1) ;
#16280=SPHERICAL_SURFACE('',#93409,0.1) ;
#16281=SPHERICAL_SURFACE('',#93426,0.1) ;
#16282=SPHERICAL_SURFACE('',#93443,0.1) ;
#16283=SPHERICAL_SURFACE('',#93460,0.1) ;
#16284=SPHERICAL_SURFACE('',#93477,0.1) ;
#16285=SPHERICAL_SURFACE('',#93539,0.1) ;
#16286=SPHERICAL_SURFACE('',#93588,0.1) ;
#16287=SPHERICAL_SURFACE('',#93976,0.1) ;
#16288=SPHERICAL_SURFACE('',#93979,0.1) ;
#16289=SPHERICAL_SURFACE('',#93997,0.1) ;
#16290=SPHERICAL_SURFACE('',#94018,0.1) ;
#16291=SPHERICAL_SURFACE('',#94020,0.1) ;
#16292=SPHERICAL_SURFACE('',#94025,0.1) ;
#16293=SPHERICAL_SURFACE('',#94028,0.1) ;
#16294=SPHERICAL_SURFACE('',#94045,0.1) ;
#16295=SPHERICAL_SURFACE('',#94051,0.1) ;
#16296=SPHERICAL_SURFACE('',#94069,0.1) ;
#16297=SPHERICAL_SURFACE('',#94070,0.1) ;
#16298=SPHERICAL_SURFACE('',#94079,0.1) ;
#16299=SPHERICAL_SURFACE('',#94085,0.1) ;
#16300=SPHERICAL_SURFACE('',#94093,0.1) ;
#16301=SPHERICAL_SURFACE('',#94095,0.1) ;
#16302=SPHERICAL_SURFACE('',#94101,0.1) ;
#16303=SPHERICAL_SURFACE('',#94102,0.1) ;
#16304=SPHERICAL_SURFACE('',#94111,0.1) ;
#16305=SPHERICAL_SURFACE('',#94117,0.1) ;
#16306=SPHERICAL_SURFACE('',#94125,0.1) ;
#16307=SPHERICAL_SURFACE('',#94127,0.1) ;
#16308=SPHERICAL_SURFACE('',#94133,0.1) ;
#16309=SPHERICAL_SURFACE('',#94139,0.1) ;
#16310=SPHERICAL_SURFACE('',#94147,0.1) ;
#16311=SPHERICAL_SURFACE('',#94153,0.1) ;
#16312=SPHERICAL_SURFACE('',#94155,0.1) ;
#16313=SPHERICAL_SURFACE('',#94161,0.1) ;
#16314=SPHERICAL_SURFACE('',#94163,0.1) ;
#16315=SPHERICAL_SURFACE('',#94168,0.1) ;
#16316=SPHERICAL_SURFACE('',#94174,0.1) ;
#16317=SPHERICAL_SURFACE('',#94176,0.1) ;
#16318=SPHERICAL_SURFACE('',#94190,0.1) ;
#16319=SPHERICAL_SURFACE('',#94192,0.1) ;
#16320=SPHERICAL_SURFACE('',#94227,0.1) ;
#16321=SPHERICAL_SURFACE('',#94235,0.1) ;
#16322=SPHERICAL_SURFACE('',#94274,0.1) ;
#16323=SPHERICAL_SURFACE('',#94284,0.1) ;
#16324=SPHERICAL_SURFACE('',#94286,0.1) ;
#16325=SPHERICAL_SURFACE('',#94295,0.1) ;
#16326=SPHERICAL_SURFACE('',#94308,0.1) ;
#16327=SPHERICAL_SURFACE('',#94318,0.1) ;
#16328=SPHERICAL_SURFACE('',#94320,0.1) ;
#16329=SPHERICAL_SURFACE('',#94329,0.1) ;
#16330=SPHERICAL_SURFACE('',#94340,0.1) ;
#16331=SPHERICAL_SURFACE('',#94344,0.1) ;
#16332=SPHERICAL_SURFACE('',#94353,0.1) ;
#16333=SPHERICAL_SURFACE('',#94357,0.1) ;
#16334=SPHERICAL_SURFACE('',#94364,0.1) ;
#16335=SPHERICAL_SURFACE('',#94368,0.1) ;
#16336=SPHERICAL_SURFACE('',#94373,0.1) ;
#16337=SPHERICAL_SURFACE('',#94379,0.1) ;
#16338=SPHERICAL_SURFACE('',#95043,0.1) ;
#16339=SPHERICAL_SURFACE('',#95046,0.1) ;
#16340=SPHERICAL_SURFACE('',#95064,0.1) ;
#16341=SPHERICAL_SURFACE('',#95085,0.1) ;
#16342=SPHERICAL_SURFACE('',#95087,0.1) ;
#16343=SPHERICAL_SURFACE('',#95092,0.1) ;
#16344=SPHERICAL_SURFACE('',#95095,0.1) ;
#16345=SPHERICAL_SURFACE('',#95112,0.1) ;
#16346=SPHERICAL_SURFACE('',#95118,0.1) ;
#16347=SPHERICAL_SURFACE('',#95136,0.1) ;
#16348=SPHERICAL_SURFACE('',#95142,0.1) ;
#16349=SPHERICAL_SURFACE('',#95150,0.1) ;
#16350=SPHERICAL_SURFACE('',#95156,0.1) ;
#16351=SPHERICAL_SURFACE('',#95158,0.1) ;
#16352=SPHERICAL_SURFACE('',#95164,0.1) ;
#16353=SPHERICAL_SURFACE('',#95166,0.1) ;
#16354=SPHERICAL_SURFACE('',#95171,0.1) ;
#16355=SPHERICAL_SURFACE('',#95177,0.1) ;
#16356=SPHERICAL_SURFACE('',#95179,0.1) ;
#16357=SPHERICAL_SURFACE('',#95193,0.1) ;
#16358=SPHERICAL_SURFACE('',#95195,0.1) ;
#16359=SPHERICAL_SURFACE('',#95230,0.1) ;
#16360=SPHERICAL_SURFACE('',#95238,0.1) ;
#16361=SPHERICAL_SURFACE('',#95246,0.1) ;
#16362=SPHERICAL_SURFACE('',#95248,0.1) ;
#16363=SPHERICAL_SURFACE('',#95283,0.1) ;
#16364=SPHERICAL_SURFACE('',#95291,0.1) ;
#16365=SPHERICAL_SURFACE('',#95299,0.1) ;
#16366=SPHERICAL_SURFACE('',#95301,0.1) ;
#16367=SPHERICAL_SURFACE('',#95336,0.1) ;
#16368=SPHERICAL_SURFACE('',#95344,0.1) ;
#16369=SPHERICAL_SURFACE('',#95352,0.1) ;
#16370=SPHERICAL_SURFACE('',#95354,0.1) ;
#16371=SPHERICAL_SURFACE('',#95389,0.1) ;
#16372=SPHERICAL_SURFACE('',#95397,0.1) ;
#16373=SPHERICAL_SURFACE('',#95405,0.1) ;
#16374=SPHERICAL_SURFACE('',#95407,0.1) ;
#16375=SPHERICAL_SURFACE('',#95442,0.1) ;
#16376=SPHERICAL_SURFACE('',#95450,0.1) ;
#16377=SPHERICAL_SURFACE('',#95458,0.1) ;
#16378=SPHERICAL_SURFACE('',#95460,0.1) ;
#16379=SPHERICAL_SURFACE('',#95495,0.1) ;
#16380=SPHERICAL_SURFACE('',#95503,0.1) ;
#16381=SPHERICAL_SURFACE('',#95511,0.1) ;
#16382=SPHERICAL_SURFACE('',#95513,0.1) ;
#16383=SPHERICAL_SURFACE('',#95548,0.1) ;
#16384=SPHERICAL_SURFACE('',#95556,0.1) ;
#16385=SPHERICAL_SURFACE('',#95564,0.1) ;
#16386=SPHERICAL_SURFACE('',#95566,0.1) ;
#16387=SPHERICAL_SURFACE('',#95601,0.1) ;
#16388=SPHERICAL_SURFACE('',#95609,0.1) ;
#16389=SPHERICAL_SURFACE('',#95617,0.1) ;
#16390=SPHERICAL_SURFACE('',#95619,0.1) ;
#16391=SPHERICAL_SURFACE('',#95654,0.1) ;
#16392=SPHERICAL_SURFACE('',#95662,0.1) ;
#16393=SPHERICAL_SURFACE('',#95673,0.1) ;
#16394=SPHERICAL_SURFACE('',#95676,0.1) ;
#16395=SPHERICAL_SURFACE('',#95694,0.1) ;
#16396=SPHERICAL_SURFACE('',#95715,0.1) ;
#16397=SPHERICAL_SURFACE('',#95717,0.1) ;
#16398=SPHERICAL_SURFACE('',#95722,0.1) ;
#16399=SPHERICAL_SURFACE('',#95725,0.1) ;
#16400=SPHERICAL_SURFACE('',#95742,0.1) ;
#16401=SPHERICAL_SURFACE('',#95748,0.1) ;
#16402=SPHERICAL_SURFACE('',#95766,0.1) ;
#16403=SPHERICAL_SURFACE('',#95772,0.1) ;
#16404=SPHERICAL_SURFACE('',#95780,0.1) ;
#16405=SPHERICAL_SURFACE('',#95786,0.1) ;
#16406=SPHERICAL_SURFACE('',#95788,0.1) ;
#16407=SPHERICAL_SURFACE('',#95794,0.1) ;
#16408=SPHERICAL_SURFACE('',#95796,0.1) ;
#16409=SPHERICAL_SURFACE('',#95801,0.1) ;
#16410=SPHERICAL_SURFACE('',#95807,0.1) ;
#16411=SPHERICAL_SURFACE('',#95809,0.1) ;
#16412=SPHERICAL_SURFACE('',#95826,0.1) ;
#16413=SPHERICAL_SURFACE('',#95829,0.1) ;
#16414=SPHERICAL_SURFACE('',#95847,0.1) ;
#16415=SPHERICAL_SURFACE('',#95868,0.1) ;
#16416=SPHERICAL_SURFACE('',#95870,0.1) ;
#16417=SPHERICAL_SURFACE('',#95875,0.1) ;
#16418=SPHERICAL_SURFACE('',#95878,0.1) ;
#16419=SPHERICAL_SURFACE('',#95895,0.1) ;
#16420=SPHERICAL_SURFACE('',#95901,0.1) ;
#16421=SPHERICAL_SURFACE('',#95919,0.1) ;
#16422=SPHERICAL_SURFACE('',#95925,0.1) ;
#16423=SPHERICAL_SURFACE('',#95933,0.1) ;
#16424=SPHERICAL_SURFACE('',#95939,0.1) ;
#16425=SPHERICAL_SURFACE('',#95941,0.1) ;
#16426=SPHERICAL_SURFACE('',#95947,0.1) ;
#16427=SPHERICAL_SURFACE('',#95949,0.1) ;
#16428=SPHERICAL_SURFACE('',#95954,0.1) ;
#16429=SPHERICAL_SURFACE('',#95960,0.1) ;
#16430=SPHERICAL_SURFACE('',#95962,0.1) ;
#16431=SPHERICAL_SURFACE('',#95979,0.1) ;
#16432=SPHERICAL_SURFACE('',#95982,0.1) ;
#16433=SPHERICAL_SURFACE('',#96000,0.1) ;
#16434=SPHERICAL_SURFACE('',#96021,0.1) ;
#16435=SPHERICAL_SURFACE('',#96023,0.1) ;
#16436=SPHERICAL_SURFACE('',#96028,0.1) ;
#16437=SPHERICAL_SURFACE('',#96031,0.1) ;
#16438=SPHERICAL_SURFACE('',#96048,0.1) ;
#16439=SPHERICAL_SURFACE('',#96054,0.1) ;
#16440=SPHERICAL_SURFACE('',#96072,0.1) ;
#16441=SPHERICAL_SURFACE('',#96078,0.1) ;
#16442=SPHERICAL_SURFACE('',#96086,0.1) ;
#16443=SPHERICAL_SURFACE('',#96092,0.1) ;
#16444=SPHERICAL_SURFACE('',#96094,0.1) ;
#16445=SPHERICAL_SURFACE('',#96100,0.1) ;
#16446=SPHERICAL_SURFACE('',#96102,0.1) ;
#16447=SPHERICAL_SURFACE('',#96107,0.1) ;
#16448=SPHERICAL_SURFACE('',#96113,0.1) ;
#16449=SPHERICAL_SURFACE('',#96115,0.1) ;
#16450=SPHERICAL_SURFACE('',#96132,0.1) ;
#16451=SPHERICAL_SURFACE('',#96135,0.1) ;
#16452=SPHERICAL_SURFACE('',#96153,0.1) ;
#16453=SPHERICAL_SURFACE('',#96174,0.1) ;
#16454=SPHERICAL_SURFACE('',#96176,0.1) ;
#16455=SPHERICAL_SURFACE('',#96181,0.1) ;
#16456=SPHERICAL_SURFACE('',#96184,0.1) ;
#16457=SPHERICAL_SURFACE('',#96201,0.1) ;
#16458=SPHERICAL_SURFACE('',#96207,0.1) ;
#16459=SPHERICAL_SURFACE('',#96225,0.1) ;
#16460=SPHERICAL_SURFACE('',#96231,0.1) ;
#16461=SPHERICAL_SURFACE('',#96239,0.1) ;
#16462=SPHERICAL_SURFACE('',#96245,0.1) ;
#16463=SPHERICAL_SURFACE('',#96247,0.1) ;
#16464=SPHERICAL_SURFACE('',#96253,0.1) ;
#16465=SPHERICAL_SURFACE('',#96255,0.1) ;
#16466=SPHERICAL_SURFACE('',#96260,0.1) ;
#16467=SPHERICAL_SURFACE('',#96266,0.1) ;
#16468=SPHERICAL_SURFACE('',#96268,0.1) ;
#16469=SPHERICAL_SURFACE('',#96285,0.1) ;
#16470=SPHERICAL_SURFACE('',#96288,0.1) ;
#16471=SPHERICAL_SURFACE('',#96306,0.1) ;
#16472=SPHERICAL_SURFACE('',#96327,0.1) ;
#16473=SPHERICAL_SURFACE('',#96329,0.1) ;
#16474=SPHERICAL_SURFACE('',#96334,0.1) ;
#16475=SPHERICAL_SURFACE('',#96337,0.1) ;
#16476=SPHERICAL_SURFACE('',#96354,0.1) ;
#16477=SPHERICAL_SURFACE('',#96360,0.1) ;
#16478=SPHERICAL_SURFACE('',#96378,0.1) ;
#16479=SPHERICAL_SURFACE('',#96384,0.1) ;
#16480=SPHERICAL_SURFACE('',#96392,0.1) ;
#16481=SPHERICAL_SURFACE('',#96398,0.1) ;
#16482=SPHERICAL_SURFACE('',#96400,0.1) ;
#16483=SPHERICAL_SURFACE('',#96406,0.1) ;
#16484=SPHERICAL_SURFACE('',#96408,0.1) ;
#16485=SPHERICAL_SURFACE('',#96413,0.1) ;
#16486=SPHERICAL_SURFACE('',#96419,0.1) ;
#16487=SPHERICAL_SURFACE('',#96421,0.1) ;
#16488=SPHERICAL_SURFACE('',#96438,0.1) ;
#16489=SPHERICAL_SURFACE('',#96441,0.1) ;
#16490=SPHERICAL_SURFACE('',#96459,0.1) ;
#16491=SPHERICAL_SURFACE('',#96480,0.1) ;
#16492=SPHERICAL_SURFACE('',#96482,0.1) ;
#16493=SPHERICAL_SURFACE('',#96487,0.1) ;
#16494=SPHERICAL_SURFACE('',#96490,0.1) ;
#16495=SPHERICAL_SURFACE('',#96507,0.1) ;
#16496=SPHERICAL_SURFACE('',#96513,0.1) ;
#16497=SPHERICAL_SURFACE('',#96531,0.1) ;
#16498=SPHERICAL_SURFACE('',#96537,0.1) ;
#16499=SPHERICAL_SURFACE('',#96545,0.1) ;
#16500=SPHERICAL_SURFACE('',#96551,0.1) ;
#16501=SPHERICAL_SURFACE('',#96553,0.1) ;
#16502=SPHERICAL_SURFACE('',#96559,0.1) ;
#16503=SPHERICAL_SURFACE('',#96561,0.1) ;
#16504=SPHERICAL_SURFACE('',#96566,0.1) ;
#16505=SPHERICAL_SURFACE('',#96572,0.1) ;
#16506=SPHERICAL_SURFACE('',#96574,0.1) ;
#16507=SPHERICAL_SURFACE('',#96591,0.1) ;
#16508=SPHERICAL_SURFACE('',#96594,0.1) ;
#16509=SPHERICAL_SURFACE('',#96612,0.1) ;
#16510=SPHERICAL_SURFACE('',#96633,0.1) ;
#16511=SPHERICAL_SURFACE('',#96635,0.1) ;
#16512=SPHERICAL_SURFACE('',#96640,0.1) ;
#16513=SPHERICAL_SURFACE('',#96643,0.1) ;
#16514=SPHERICAL_SURFACE('',#96660,0.1) ;
#16515=SPHERICAL_SURFACE('',#96666,0.1) ;
#16516=SPHERICAL_SURFACE('',#96684,0.1) ;
#16517=SPHERICAL_SURFACE('',#96690,0.1) ;
#16518=SPHERICAL_SURFACE('',#96698,0.1) ;
#16519=SPHERICAL_SURFACE('',#96704,0.1) ;
#16520=SPHERICAL_SURFACE('',#96706,0.1) ;
#16521=SPHERICAL_SURFACE('',#96712,0.1) ;
#16522=SPHERICAL_SURFACE('',#96714,0.1) ;
#16523=SPHERICAL_SURFACE('',#96719,0.1) ;
#16524=SPHERICAL_SURFACE('',#96725,0.1) ;
#16525=SPHERICAL_SURFACE('',#96727,0.1) ;
#16526=SPHERICAL_SURFACE('',#96744,0.1) ;
#16527=SPHERICAL_SURFACE('',#96747,0.1) ;
#16528=SPHERICAL_SURFACE('',#96765,0.1) ;
#16529=SPHERICAL_SURFACE('',#96786,0.1) ;
#16530=SPHERICAL_SURFACE('',#96788,0.1) ;
#16531=SPHERICAL_SURFACE('',#96793,0.1) ;
#16532=SPHERICAL_SURFACE('',#96796,0.1) ;
#16533=SPHERICAL_SURFACE('',#96813,0.1) ;
#16534=SPHERICAL_SURFACE('',#96819,0.1) ;
#16535=SPHERICAL_SURFACE('',#96837,0.1) ;
#16536=SPHERICAL_SURFACE('',#96843,0.1) ;
#16537=SPHERICAL_SURFACE('',#96851,0.1) ;
#16538=SPHERICAL_SURFACE('',#96857,0.1) ;
#16539=SPHERICAL_SURFACE('',#96859,0.1) ;
#16540=SPHERICAL_SURFACE('',#96865,0.1) ;
#16541=SPHERICAL_SURFACE('',#96867,0.1) ;
#16542=SPHERICAL_SURFACE('',#96872,0.1) ;
#16543=SPHERICAL_SURFACE('',#96878,0.1) ;
#16544=SPHERICAL_SURFACE('',#96880,0.1) ;
#16545=SPHERICAL_SURFACE('',#97149,0.1) ;
#16546=SPHERICAL_SURFACE('',#97159,0.1) ;
#16547=SPHERICAL_SURFACE('',#97161,0.1) ;
#16548=SPHERICAL_SURFACE('',#97170,0.1) ;
#16549=SPHERICAL_SURFACE('',#97183,0.1) ;
#16550=SPHERICAL_SURFACE('',#97193,0.1) ;
#16551=SPHERICAL_SURFACE('',#97195,0.1) ;
#16552=SPHERICAL_SURFACE('',#97204,0.1) ;
#16553=SPHERICAL_SURFACE('',#97217,0.1) ;
#16554=SPHERICAL_SURFACE('',#97227,0.1) ;
#16555=SPHERICAL_SURFACE('',#97229,0.1) ;
#16556=SPHERICAL_SURFACE('',#97238,0.1) ;
#16557=SPHERICAL_SURFACE('',#97251,0.1) ;
#16558=SPHERICAL_SURFACE('',#97261,0.1) ;
#16559=SPHERICAL_SURFACE('',#97263,0.1) ;
#16560=SPHERICAL_SURFACE('',#97272,0.1) ;
#16561=SPHERICAL_SURFACE('',#97285,0.1) ;
#16562=SPHERICAL_SURFACE('',#97295,0.1) ;
#16563=SPHERICAL_SURFACE('',#97297,0.1) ;
#16564=SPHERICAL_SURFACE('',#97306,0.1) ;
#16565=SPHERICAL_SURFACE('',#97319,0.1) ;
#16566=SPHERICAL_SURFACE('',#97329,0.1) ;
#16567=SPHERICAL_SURFACE('',#97331,0.1) ;
#16568=SPHERICAL_SURFACE('',#97340,0.1) ;
#16569=SPHERICAL_SURFACE('',#97353,0.1) ;
#16570=SPHERICAL_SURFACE('',#97363,0.1) ;
#16571=SPHERICAL_SURFACE('',#97365,0.1) ;
#16572=SPHERICAL_SURFACE('',#97374,0.1) ;
#16573=SPHERICAL_SURFACE('',#97387,0.1) ;
#16574=SPHERICAL_SURFACE('',#97397,0.1) ;
#16575=SPHERICAL_SURFACE('',#97399,0.1) ;
#16576=SPHERICAL_SURFACE('',#97408,0.1) ;
#16577=SPHERICAL_SURFACE('',#97421,0.1) ;
#16578=SPHERICAL_SURFACE('',#97431,0.1) ;
#16579=SPHERICAL_SURFACE('',#97433,0.1) ;
#16580=SPHERICAL_SURFACE('',#97442,0.1) ;
#16581=SPHERICAL_SURFACE('',#97455,0.1) ;
#16582=SPHERICAL_SURFACE('',#97465,0.1) ;
#16583=SPHERICAL_SURFACE('',#97467,0.1) ;
#16584=SPHERICAL_SURFACE('',#97476,0.1) ;
#16585=SPHERICAL_SURFACE('',#97489,0.1) ;
#16586=SPHERICAL_SURFACE('',#97499,0.1) ;
#16587=SPHERICAL_SURFACE('',#97501,0.1) ;
#16588=SPHERICAL_SURFACE('',#97510,0.1) ;
#16589=SPHERICAL_SURFACE('',#97523,0.1) ;
#16590=SPHERICAL_SURFACE('',#97533,0.1) ;
#16591=SPHERICAL_SURFACE('',#97535,0.1) ;
#16592=SPHERICAL_SURFACE('',#97544,0.1) ;
#16593=SPHERICAL_SURFACE('',#97557,0.1) ;
#16594=SPHERICAL_SURFACE('',#97567,0.1) ;
#16595=SPHERICAL_SURFACE('',#97569,0.1) ;
#16596=SPHERICAL_SURFACE('',#97578,0.1) ;
#16597=SPHERICAL_SURFACE('',#97591,0.1) ;
#16598=SPHERICAL_SURFACE('',#97601,0.1) ;
#16599=SPHERICAL_SURFACE('',#97603,0.1) ;
#16600=SPHERICAL_SURFACE('',#97612,0.1) ;
#16601=SPHERICAL_SURFACE('',#97625,0.1) ;
#16602=SPHERICAL_SURFACE('',#97635,0.1) ;
#16603=SPHERICAL_SURFACE('',#97637,0.1) ;
#16604=SPHERICAL_SURFACE('',#97646,0.1) ;
#16605=SPHERICAL_SURFACE('',#97659,0.1) ;
#16606=SPHERICAL_SURFACE('',#97669,0.1) ;
#16607=SPHERICAL_SURFACE('',#97671,0.1) ;
#16608=SPHERICAL_SURFACE('',#97680,0.1) ;
#16609=SPHERICAL_SURFACE('',#97693,0.1) ;
#16610=SPHERICAL_SURFACE('',#97703,0.1) ;
#16611=SPHERICAL_SURFACE('',#97705,0.1) ;
#16612=SPHERICAL_SURFACE('',#97714,0.1) ;
#16613=SPHERICAL_SURFACE('',#97727,0.1) ;
#16614=SPHERICAL_SURFACE('',#97737,0.1) ;
#16615=SPHERICAL_SURFACE('',#97739,0.1) ;
#16616=SPHERICAL_SURFACE('',#97748,0.1) ;
#16617=SPHERICAL_SURFACE('',#97759,0.1) ;
#16618=SPHERICAL_SURFACE('',#97763,0.1) ;
#16619=SPHERICAL_SURFACE('',#97772,0.1) ;
#16620=SPHERICAL_SURFACE('',#97776,0.1) ;
#16621=SPHERICAL_SURFACE('',#97783,0.1) ;
#16622=SPHERICAL_SURFACE('',#97787,0.1) ;
#16623=SPHERICAL_SURFACE('',#97792,0.1) ;
#16624=SPHERICAL_SURFACE('',#97798,0.1) ;
#16625=SPHERICAL_SURFACE('',#97803,0.1) ;
#16626=SPHERICAL_SURFACE('',#97807,0.1) ;
#16627=SPHERICAL_SURFACE('',#97816,0.1) ;
#16628=SPHERICAL_SURFACE('',#97820,0.1) ;
#16629=SPHERICAL_SURFACE('',#97827,0.1) ;
#16630=SPHERICAL_SURFACE('',#97831,0.1) ;
#16631=SPHERICAL_SURFACE('',#97836,0.1) ;
#16632=SPHERICAL_SURFACE('',#97842,0.1) ;
#16633=SPHERICAL_SURFACE('',#97847,0.1) ;
#16634=SPHERICAL_SURFACE('',#97851,0.1) ;
#16635=SPHERICAL_SURFACE('',#97860,0.1) ;
#16636=SPHERICAL_SURFACE('',#97864,0.1) ;
#16637=SPHERICAL_SURFACE('',#97871,0.1) ;
#16638=SPHERICAL_SURFACE('',#97875,0.1) ;
#16639=SPHERICAL_SURFACE('',#97880,0.1) ;
#16640=SPHERICAL_SURFACE('',#97886,0.1) ;
#16641=SPHERICAL_SURFACE('',#97891,0.1) ;
#16642=SPHERICAL_SURFACE('',#97895,0.1) ;
#16643=SPHERICAL_SURFACE('',#97904,0.1) ;
#16644=SPHERICAL_SURFACE('',#97908,0.1) ;
#16645=SPHERICAL_SURFACE('',#97915,0.1) ;
#16646=SPHERICAL_SURFACE('',#97919,0.1) ;
#16647=SPHERICAL_SURFACE('',#97924,0.1) ;
#16648=SPHERICAL_SURFACE('',#97930,0.1) ;
#16649=SPHERICAL_SURFACE('',#97935,0.1) ;
#16650=SPHERICAL_SURFACE('',#97939,0.1) ;
#16651=SPHERICAL_SURFACE('',#97948,0.1) ;
#16652=SPHERICAL_SURFACE('',#97952,0.1) ;
#16653=SPHERICAL_SURFACE('',#97959,0.1) ;
#16654=SPHERICAL_SURFACE('',#97963,0.1) ;
#16655=SPHERICAL_SURFACE('',#97968,0.1) ;
#16656=SPHERICAL_SURFACE('',#97974,0.1) ;
#16657=SPHERICAL_SURFACE('',#97979,0.1) ;
#16658=SPHERICAL_SURFACE('',#97983,0.1) ;
#16659=SPHERICAL_SURFACE('',#97992,0.1) ;
#16660=SPHERICAL_SURFACE('',#97996,0.1) ;
#16661=SPHERICAL_SURFACE('',#98003,0.1) ;
#16662=SPHERICAL_SURFACE('',#98007,0.1) ;
#16663=SPHERICAL_SURFACE('',#98012,0.1) ;
#16664=SPHERICAL_SURFACE('',#98018,0.1) ;
#16665=SPHERICAL_SURFACE('',#98023,0.1) ;
#16666=SPHERICAL_SURFACE('',#98027,0.1) ;
#16667=SPHERICAL_SURFACE('',#98036,0.1) ;
#16668=SPHERICAL_SURFACE('',#98040,0.1) ;
#16669=SPHERICAL_SURFACE('',#98047,0.1) ;
#16670=SPHERICAL_SURFACE('',#98051,0.1) ;
#16671=SPHERICAL_SURFACE('',#98056,0.1) ;
#16672=SPHERICAL_SURFACE('',#98062,0.1) ;
#16673=SPHERICAL_SURFACE('',#98067,0.1) ;
#16674=SPHERICAL_SURFACE('',#98071,0.1) ;
#16675=SPHERICAL_SURFACE('',#98080,0.1) ;
#16676=SPHERICAL_SURFACE('',#98084,0.1) ;
#16677=SPHERICAL_SURFACE('',#98091,0.1) ;
#16678=SPHERICAL_SURFACE('',#98095,0.1) ;
#16679=SPHERICAL_SURFACE('',#98100,0.1) ;
#16680=SPHERICAL_SURFACE('',#98106,0.1) ;
#16681=SPHERICAL_SURFACE('',#98111,0.1) ;
#16682=SPHERICAL_SURFACE('',#98115,0.1) ;
#16683=SPHERICAL_SURFACE('',#98124,0.1) ;
#16684=SPHERICAL_SURFACE('',#98128,0.1) ;
#16685=SPHERICAL_SURFACE('',#98135,0.1) ;
#16686=SPHERICAL_SURFACE('',#98139,0.1) ;
#16687=SPHERICAL_SURFACE('',#98144,0.1) ;
#16688=SPHERICAL_SURFACE('',#98150,0.1) ;
#18168=FACE_OUTER_BOUND('',#23921,.T.) ;
#18169=FACE_OUTER_BOUND('',#23922,.T.) ;
#18170=FACE_OUTER_BOUND('',#23923,.T.) ;
#18171=FACE_OUTER_BOUND('',#23924,.T.) ;
#18172=FACE_OUTER_BOUND('',#23925,.T.) ;
#18173=FACE_OUTER_BOUND('',#23926,.T.) ;
#18174=FACE_OUTER_BOUND('',#23927,.T.) ;
#18175=FACE_OUTER_BOUND('',#23928,.T.) ;
#18176=FACE_OUTER_BOUND('',#23929,.T.) ;
#18177=FACE_OUTER_BOUND('',#23930,.T.) ;
#18178=FACE_OUTER_BOUND('',#23931,.T.) ;
#18179=FACE_OUTER_BOUND('',#23932,.T.) ;
#18180=FACE_OUTER_BOUND('',#23933,.T.) ;
#18181=FACE_OUTER_BOUND('',#23934,.T.) ;
#18182=FACE_OUTER_BOUND('',#23935,.T.) ;
#18183=FACE_OUTER_BOUND('',#23936,.T.) ;
#18184=FACE_OUTER_BOUND('',#23937,.T.) ;
#18185=FACE_OUTER_BOUND('',#23938,.T.) ;
#18186=FACE_OUTER_BOUND('',#23939,.T.) ;
#18187=FACE_OUTER_BOUND('',#23940,.T.) ;
#18188=FACE_OUTER_BOUND('',#23941,.T.) ;
#18189=FACE_OUTER_BOUND('',#23942,.T.) ;
#18190=FACE_OUTER_BOUND('',#23943,.T.) ;
#18191=FACE_OUTER_BOUND('',#23944,.T.) ;
#18192=FACE_OUTER_BOUND('',#23945,.T.) ;
#18193=FACE_OUTER_BOUND('',#23946,.T.) ;
#18194=FACE_OUTER_BOUND('',#23947,.T.) ;
#18195=FACE_OUTER_BOUND('',#23948,.T.) ;
#18196=FACE_OUTER_BOUND('',#23949,.T.) ;
#18197=FACE_OUTER_BOUND('',#23950,.T.) ;
#18198=FACE_OUTER_BOUND('',#23951,.T.) ;
#18199=FACE_OUTER_BOUND('',#23952,.T.) ;
#18200=FACE_OUTER_BOUND('',#23953,.T.) ;
#18201=FACE_OUTER_BOUND('',#23954,.T.) ;
#18202=FACE_OUTER_BOUND('',#23955,.T.) ;
#18203=FACE_OUTER_BOUND('',#23956,.T.) ;
#18204=FACE_OUTER_BOUND('',#23957,.T.) ;
#18205=FACE_OUTER_BOUND('',#23958,.T.) ;
#18206=FACE_OUTER_BOUND('',#23959,.T.) ;
#18207=FACE_OUTER_BOUND('',#23960,.T.) ;
#18208=FACE_OUTER_BOUND('',#23961,.T.) ;
#18209=FACE_OUTER_BOUND('',#23962,.T.) ;
#18210=FACE_OUTER_BOUND('',#23963,.T.) ;
#18211=FACE_OUTER_BOUND('',#23964,.T.) ;
#18212=FACE_OUTER_BOUND('',#23965,.T.) ;
#18213=FACE_OUTER_BOUND('',#23966,.T.) ;
#18214=FACE_OUTER_BOUND('',#23967,.T.) ;
#18215=FACE_OUTER_BOUND('',#23968,.T.) ;
#18216=FACE_OUTER_BOUND('',#23969,.T.) ;
#18217=FACE_OUTER_BOUND('',#23970,.T.) ;
#18218=FACE_OUTER_BOUND('',#23971,.T.) ;
#18219=FACE_OUTER_BOUND('',#23972,.T.) ;
#18220=FACE_OUTER_BOUND('',#23973,.T.) ;
#18221=FACE_OUTER_BOUND('',#23974,.T.) ;
#18222=FACE_OUTER_BOUND('',#23975,.T.) ;
#18223=FACE_OUTER_BOUND('',#23976,.T.) ;
#18224=FACE_OUTER_BOUND('',#23977,.T.) ;
#18225=FACE_OUTER_BOUND('',#23978,.T.) ;
#18226=FACE_OUTER_BOUND('',#23979,.T.) ;
#18227=FACE_OUTER_BOUND('',#23980,.T.) ;
#18228=FACE_OUTER_BOUND('',#23981,.T.) ;
#18229=FACE_OUTER_BOUND('',#23982,.T.) ;
#18230=FACE_OUTER_BOUND('',#23983,.T.) ;
#18231=FACE_OUTER_BOUND('',#23984,.T.) ;
#18232=FACE_OUTER_BOUND('',#23985,.T.) ;
#18233=FACE_OUTER_BOUND('',#23986,.T.) ;
#18234=FACE_OUTER_BOUND('',#23987,.T.) ;
#18235=FACE_OUTER_BOUND('',#23988,.T.) ;
#18236=FACE_OUTER_BOUND('',#23989,.T.) ;
#18237=FACE_OUTER_BOUND('',#23990,.T.) ;
#18238=FACE_OUTER_BOUND('',#23991,.T.) ;
#18239=FACE_OUTER_BOUND('',#23992,.T.) ;
#18240=FACE_OUTER_BOUND('',#23993,.T.) ;
#18241=FACE_OUTER_BOUND('',#23994,.T.) ;
#18242=FACE_OUTER_BOUND('',#23995,.T.) ;
#18243=FACE_OUTER_BOUND('',#23996,.T.) ;
#18244=FACE_OUTER_BOUND('',#23997,.T.) ;
#18245=FACE_OUTER_BOUND('',#23998,.T.) ;
#18246=FACE_OUTER_BOUND('',#23999,.T.) ;
#18247=FACE_OUTER_BOUND('',#24000,.T.) ;
#18248=FACE_OUTER_BOUND('',#24001,.T.) ;
#18249=FACE_OUTER_BOUND('',#24002,.T.) ;
#18250=FACE_OUTER_BOUND('',#24003,.T.) ;
#18251=FACE_OUTER_BOUND('',#24004,.T.) ;
#18252=FACE_OUTER_BOUND('',#24005,.T.) ;
#18253=FACE_OUTER_BOUND('',#24006,.T.) ;
#18254=FACE_OUTER_BOUND('',#24007,.T.) ;
#18255=FACE_OUTER_BOUND('',#24008,.T.) ;
#18256=FACE_OUTER_BOUND('',#24009,.T.) ;
#18257=FACE_OUTER_BOUND('',#24010,.T.) ;
#18258=FACE_OUTER_BOUND('',#24011,.T.) ;
#18259=FACE_OUTER_BOUND('',#24012,.T.) ;
#18260=FACE_OUTER_BOUND('',#24013,.T.) ;
#18261=FACE_OUTER_BOUND('',#24014,.T.) ;
#18262=FACE_OUTER_BOUND('',#24015,.T.) ;
#18263=FACE_OUTER_BOUND('',#24016,.T.) ;
#18264=FACE_OUTER_BOUND('',#24017,.T.) ;
#18265=FACE_OUTER_BOUND('',#24018,.T.) ;
#18266=FACE_OUTER_BOUND('',#24019,.T.) ;
#18267=FACE_OUTER_BOUND('',#24020,.T.) ;
#18268=FACE_OUTER_BOUND('',#24021,.T.) ;
#18269=FACE_OUTER_BOUND('',#24022,.T.) ;
#18270=FACE_OUTER_BOUND('',#24023,.T.) ;
#18271=FACE_OUTER_BOUND('',#24024,.T.) ;
#18272=FACE_OUTER_BOUND('',#24025,.T.) ;
#18273=FACE_OUTER_BOUND('',#24026,.T.) ;
#18274=FACE_OUTER_BOUND('',#24027,.T.) ;
#18275=FACE_OUTER_BOUND('',#24028,.T.) ;
#18276=FACE_OUTER_BOUND('',#24029,.T.) ;
#18277=FACE_OUTER_BOUND('',#24030,.T.) ;
#18278=FACE_OUTER_BOUND('',#24031,.T.) ;
#18279=FACE_OUTER_BOUND('',#24032,.T.) ;
#18280=FACE_OUTER_BOUND('',#24033,.T.) ;
#18281=FACE_OUTER_BOUND('',#24034,.T.) ;
#18282=FACE_OUTER_BOUND('',#24035,.T.) ;
#18283=FACE_OUTER_BOUND('',#24036,.T.) ;
#18284=FACE_OUTER_BOUND('',#24037,.T.) ;
#18285=FACE_OUTER_BOUND('',#24038,.T.) ;
#18286=FACE_OUTER_BOUND('',#24039,.T.) ;
#18287=FACE_OUTER_BOUND('',#24040,.T.) ;
#18288=FACE_OUTER_BOUND('',#24041,.T.) ;
#18289=FACE_OUTER_BOUND('',#24042,.T.) ;
#18290=FACE_OUTER_BOUND('',#24043,.T.) ;
#18291=FACE_OUTER_BOUND('',#24044,.T.) ;
#18292=FACE_OUTER_BOUND('',#24045,.T.) ;
#18293=FACE_OUTER_BOUND('',#24046,.T.) ;
#18294=FACE_OUTER_BOUND('',#24057,.T.) ;
#18295=FACE_OUTER_BOUND('',#24058,.T.) ;
#18296=FACE_OUTER_BOUND('',#24059,.T.) ;
#18297=FACE_OUTER_BOUND('',#24060,.T.) ;
#18298=FACE_OUTER_BOUND('',#24061,.T.) ;
#18299=FACE_OUTER_BOUND('',#24062,.T.) ;
#18300=FACE_OUTER_BOUND('',#24063,.T.) ;
#18301=FACE_OUTER_BOUND('',#24064,.T.) ;
#18302=FACE_OUTER_BOUND('',#24065,.T.) ;
#18303=FACE_OUTER_BOUND('',#24066,.T.) ;
#18304=FACE_OUTER_BOUND('',#24067,.T.) ;
#18305=FACE_OUTER_BOUND('',#24068,.T.) ;
#18306=FACE_OUTER_BOUND('',#24069,.T.) ;
#18307=FACE_OUTER_BOUND('',#24070,.T.) ;
#18308=FACE_OUTER_BOUND('',#24071,.T.) ;
#18309=FACE_OUTER_BOUND('',#24072,.T.) ;
#18310=FACE_OUTER_BOUND('',#24073,.T.) ;
#18311=FACE_OUTER_BOUND('',#24074,.T.) ;
#18312=FACE_OUTER_BOUND('',#24075,.T.) ;
#18313=FACE_OUTER_BOUND('',#24076,.T.) ;
#18314=FACE_OUTER_BOUND('',#24077,.T.) ;
#18315=FACE_OUTER_BOUND('',#24078,.T.) ;
#18316=FACE_OUTER_BOUND('',#24079,.T.) ;
#18317=FACE_OUTER_BOUND('',#24080,.T.) ;
#18318=FACE_OUTER_BOUND('',#24081,.T.) ;
#18319=FACE_OUTER_BOUND('',#24082,.T.) ;
#18320=FACE_OUTER_BOUND('',#24083,.T.) ;
#18321=FACE_OUTER_BOUND('',#24084,.T.) ;
#18322=FACE_OUTER_BOUND('',#24085,.T.) ;
#18323=FACE_OUTER_BOUND('',#24086,.T.) ;
#18324=FACE_OUTER_BOUND('',#24087,.T.) ;
#18325=FACE_OUTER_BOUND('',#24088,.T.) ;
#18326=FACE_OUTER_BOUND('',#24089,.T.) ;
#18327=FACE_OUTER_BOUND('',#24090,.T.) ;
#18328=FACE_OUTER_BOUND('',#24091,.T.) ;
#18329=FACE_OUTER_BOUND('',#24092,.T.) ;
#18330=FACE_OUTER_BOUND('',#24094,.T.) ;
#18331=FACE_OUTER_BOUND('',#24096,.T.) ;
#18332=FACE_OUTER_BOUND('',#24097,.T.) ;
#18333=FACE_OUTER_BOUND('',#24098,.T.) ;
#18334=FACE_OUTER_BOUND('',#24099,.T.) ;
#18335=FACE_OUTER_BOUND('',#24100,.T.) ;
#18336=FACE_OUTER_BOUND('',#24101,.T.) ;
#18337=FACE_OUTER_BOUND('',#24102,.T.) ;
#18338=FACE_OUTER_BOUND('',#24103,.T.) ;
#18339=FACE_OUTER_BOUND('',#24104,.T.) ;
#18340=FACE_OUTER_BOUND('',#24105,.T.) ;
#18341=FACE_OUTER_BOUND('',#24106,.T.) ;
#18342=FACE_OUTER_BOUND('',#24107,.T.) ;
#18343=FACE_OUTER_BOUND('',#24108,.T.) ;
#18344=FACE_OUTER_BOUND('',#24109,.T.) ;
#18345=FACE_OUTER_BOUND('',#24110,.T.) ;
#18346=FACE_OUTER_BOUND('',#24111,.T.) ;
#18347=FACE_OUTER_BOUND('',#24112,.T.) ;
#18348=FACE_OUTER_BOUND('',#24113,.T.) ;
#18349=FACE_OUTER_BOUND('',#24114,.T.) ;
#18350=FACE_OUTER_BOUND('',#24115,.T.) ;
#18351=FACE_OUTER_BOUND('',#24116,.T.) ;
#18352=FACE_OUTER_BOUND('',#24117,.T.) ;
#18353=FACE_OUTER_BOUND('',#24118,.T.) ;
#18354=FACE_OUTER_BOUND('',#24119,.T.) ;
#18355=FACE_OUTER_BOUND('',#24120,.T.) ;
#18356=FACE_OUTER_BOUND('',#24121,.T.) ;
#18357=FACE_OUTER_BOUND('',#24122,.T.) ;
#18358=FACE_OUTER_BOUND('',#24123,.T.) ;
#18359=FACE_OUTER_BOUND('',#24124,.T.) ;
#18360=FACE_OUTER_BOUND('',#24125,.T.) ;
#18361=FACE_OUTER_BOUND('',#24126,.T.) ;
#18362=FACE_OUTER_BOUND('',#24127,.T.) ;
#18363=FACE_OUTER_BOUND('',#24128,.T.) ;
#18364=FACE_OUTER_BOUND('',#24129,.T.) ;
#18365=FACE_OUTER_BOUND('',#24130,.T.) ;
#18366=FACE_OUTER_BOUND('',#24131,.T.) ;
#18367=FACE_OUTER_BOUND('',#24132,.T.) ;
#18368=FACE_OUTER_BOUND('',#24133,.T.) ;
#18369=FACE_OUTER_BOUND('',#24134,.T.) ;
#18370=FACE_OUTER_BOUND('',#24135,.T.) ;
#18371=FACE_OUTER_BOUND('',#24136,.T.) ;
#18372=FACE_OUTER_BOUND('',#24137,.T.) ;
#18373=FACE_OUTER_BOUND('',#24138,.T.) ;
#18374=FACE_OUTER_BOUND('',#24139,.T.) ;
#18375=FACE_OUTER_BOUND('',#24140,.T.) ;
#18376=FACE_OUTER_BOUND('',#24141,.T.) ;
#18377=FACE_OUTER_BOUND('',#24142,.T.) ;
#18378=FACE_OUTER_BOUND('',#24143,.T.) ;
#18379=FACE_OUTER_BOUND('',#24144,.T.) ;
#18380=FACE_OUTER_BOUND('',#24145,.T.) ;
#18381=FACE_OUTER_BOUND('',#24146,.T.) ;
#18382=FACE_OUTER_BOUND('',#24147,.T.) ;
#18383=FACE_OUTER_BOUND('',#24148,.T.) ;
#18384=FACE_OUTER_BOUND('',#24149,.T.) ;
#18385=FACE_OUTER_BOUND('',#24150,.T.) ;
#18386=FACE_OUTER_BOUND('',#24151,.T.) ;
#18387=FACE_OUTER_BOUND('',#24152,.T.) ;
#18388=FACE_OUTER_BOUND('',#24153,.T.) ;
#18389=FACE_OUTER_BOUND('',#24154,.T.) ;
#18390=FACE_OUTER_BOUND('',#24155,.T.) ;
#18391=FACE_OUTER_BOUND('',#24156,.T.) ;
#18392=FACE_OUTER_BOUND('',#24157,.T.) ;
#18393=FACE_OUTER_BOUND('',#24158,.T.) ;
#18394=FACE_OUTER_BOUND('',#24159,.T.) ;
#18395=FACE_OUTER_BOUND('',#24160,.T.) ;
#18396=FACE_OUTER_BOUND('',#24161,.T.) ;
#18397=FACE_OUTER_BOUND('',#24162,.T.) ;
#18398=FACE_OUTER_BOUND('',#24163,.T.) ;
#18399=FACE_OUTER_BOUND('',#24164,.T.) ;
#18400=FACE_OUTER_BOUND('',#24165,.T.) ;
#18401=FACE_OUTER_BOUND('',#24166,.T.) ;
#18402=FACE_OUTER_BOUND('',#24167,.T.) ;
#18403=FACE_OUTER_BOUND('',#24168,.T.) ;
#18404=FACE_OUTER_BOUND('',#24169,.T.) ;
#18405=FACE_OUTER_BOUND('',#24170,.T.) ;
#18406=FACE_OUTER_BOUND('',#24171,.T.) ;
#18407=FACE_OUTER_BOUND('',#24172,.T.) ;
#18408=FACE_OUTER_BOUND('',#24173,.T.) ;
#18409=FACE_OUTER_BOUND('',#24174,.T.) ;
#18410=FACE_OUTER_BOUND('',#24175,.T.) ;
#18411=FACE_OUTER_BOUND('',#24176,.T.) ;
#18412=FACE_OUTER_BOUND('',#24177,.T.) ;
#18413=FACE_OUTER_BOUND('',#24178,.T.) ;
#18414=FACE_OUTER_BOUND('',#24179,.T.) ;
#18415=FACE_OUTER_BOUND('',#24180,.T.) ;
#18416=FACE_OUTER_BOUND('',#24181,.T.) ;
#18417=FACE_OUTER_BOUND('',#24182,.T.) ;
#18418=FACE_OUTER_BOUND('',#24183,.T.) ;
#18419=FACE_OUTER_BOUND('',#24184,.T.) ;
#18420=FACE_OUTER_BOUND('',#24185,.T.) ;
#18421=FACE_OUTER_BOUND('',#24186,.T.) ;
#18422=FACE_OUTER_BOUND('',#24187,.T.) ;
#18423=FACE_OUTER_BOUND('',#24188,.T.) ;
#18424=FACE_OUTER_BOUND('',#24189,.T.) ;
#18425=FACE_OUTER_BOUND('',#24190,.T.) ;
#18426=FACE_OUTER_BOUND('',#24191,.T.) ;
#18427=FACE_OUTER_BOUND('',#24192,.T.) ;
#18428=FACE_OUTER_BOUND('',#24193,.T.) ;
#18429=FACE_OUTER_BOUND('',#24194,.T.) ;
#18430=FACE_OUTER_BOUND('',#24195,.T.) ;
#18431=FACE_OUTER_BOUND('',#24196,.T.) ;
#18432=FACE_OUTER_BOUND('',#24197,.T.) ;
#18433=FACE_OUTER_BOUND('',#24198,.T.) ;
#18434=FACE_OUTER_BOUND('',#24199,.T.) ;
#18435=FACE_OUTER_BOUND('',#24200,.T.) ;
#18436=FACE_OUTER_BOUND('',#24201,.T.) ;
#18437=FACE_OUTER_BOUND('',#24202,.T.) ;
#18438=FACE_OUTER_BOUND('',#24203,.T.) ;
#18439=FACE_OUTER_BOUND('',#24204,.T.) ;
#18440=FACE_OUTER_BOUND('',#24205,.T.) ;
#18441=FACE_OUTER_BOUND('',#24206,.T.) ;
#18442=FACE_OUTER_BOUND('',#24207,.T.) ;
#18443=FACE_OUTER_BOUND('',#24208,.T.) ;
#18444=FACE_OUTER_BOUND('',#24209,.T.) ;
#18445=FACE_OUTER_BOUND('',#24210,.T.) ;
#18446=FACE_OUTER_BOUND('',#24211,.T.) ;
#18447=FACE_OUTER_BOUND('',#24212,.T.) ;
#18448=FACE_OUTER_BOUND('',#24213,.T.) ;
#18449=FACE_OUTER_BOUND('',#24214,.T.) ;
#18450=FACE_OUTER_BOUND('',#24215,.T.) ;
#18451=FACE_OUTER_BOUND('',#24216,.T.) ;
#18452=FACE_OUTER_BOUND('',#24217,.T.) ;
#18453=FACE_OUTER_BOUND('',#24218,.T.) ;
#18454=FACE_OUTER_BOUND('',#24219,.T.) ;
#18455=FACE_OUTER_BOUND('',#24220,.T.) ;
#18456=FACE_OUTER_BOUND('',#24221,.T.) ;
#18457=FACE_OUTER_BOUND('',#24222,.T.) ;
#18458=FACE_OUTER_BOUND('',#24223,.T.) ;
#18459=FACE_OUTER_BOUND('',#24224,.T.) ;
#18460=FACE_OUTER_BOUND('',#24225,.T.) ;
#18461=FACE_OUTER_BOUND('',#24226,.T.) ;
#18462=FACE_OUTER_BOUND('',#24227,.T.) ;
#18463=FACE_OUTER_BOUND('',#24228,.T.) ;
#18464=FACE_OUTER_BOUND('',#24229,.T.) ;
#18465=FACE_OUTER_BOUND('',#24230,.T.) ;
#18466=FACE_OUTER_BOUND('',#24231,.T.) ;
#18467=FACE_OUTER_BOUND('',#24232,.T.) ;
#18468=FACE_OUTER_BOUND('',#24233,.T.) ;
#18469=FACE_OUTER_BOUND('',#24234,.T.) ;
#18470=FACE_OUTER_BOUND('',#24235,.T.) ;
#18471=FACE_OUTER_BOUND('',#24236,.T.) ;
#18472=FACE_OUTER_BOUND('',#24237,.T.) ;
#18473=FACE_OUTER_BOUND('',#24238,.T.) ;
#18474=FACE_OUTER_BOUND('',#24239,.T.) ;
#18475=FACE_OUTER_BOUND('',#24240,.T.) ;
#18476=FACE_OUTER_BOUND('',#24241,.T.) ;
#18477=FACE_OUTER_BOUND('',#24242,.T.) ;
#18478=FACE_OUTER_BOUND('',#24243,.T.) ;
#18479=FACE_OUTER_BOUND('',#24244,.T.) ;
#18480=FACE_OUTER_BOUND('',#24245,.T.) ;
#18481=FACE_OUTER_BOUND('',#24246,.T.) ;
#18482=FACE_OUTER_BOUND('',#24247,.T.) ;
#18483=FACE_OUTER_BOUND('',#24248,.T.) ;
#18484=FACE_OUTER_BOUND('',#24249,.T.) ;
#18485=FACE_OUTER_BOUND('',#24250,.T.) ;
#18486=FACE_OUTER_BOUND('',#24251,.T.) ;
#18487=FACE_OUTER_BOUND('',#24252,.T.) ;
#18488=FACE_OUTER_BOUND('',#24253,.T.) ;
#18489=FACE_OUTER_BOUND('',#24254,.T.) ;
#18490=FACE_OUTER_BOUND('',#24255,.T.) ;
#18491=FACE_OUTER_BOUND('',#24256,.T.) ;
#18492=FACE_OUTER_BOUND('',#24257,.T.) ;
#18493=FACE_OUTER_BOUND('',#24258,.T.) ;
#18494=FACE_OUTER_BOUND('',#24259,.T.) ;
#18495=FACE_OUTER_BOUND('',#24260,.T.) ;
#18496=FACE_OUTER_BOUND('',#24261,.T.) ;
#18497=FACE_OUTER_BOUND('',#24262,.T.) ;
#18498=FACE_OUTER_BOUND('',#24263,.T.) ;
#18499=FACE_OUTER_BOUND('',#24264,.T.) ;
#18500=FACE_OUTER_BOUND('',#24265,.T.) ;
#18501=FACE_OUTER_BOUND('',#24266,.T.) ;
#18502=FACE_OUTER_BOUND('',#24267,.T.) ;
#18503=FACE_OUTER_BOUND('',#24268,.T.) ;
#18504=FACE_OUTER_BOUND('',#24269,.T.) ;
#18505=FACE_OUTER_BOUND('',#24270,.T.) ;
#18506=FACE_OUTER_BOUND('',#24271,.T.) ;
#18507=FACE_OUTER_BOUND('',#24272,.T.) ;
#18508=FACE_OUTER_BOUND('',#24273,.T.) ;
#18509=FACE_OUTER_BOUND('',#24274,.T.) ;
#18510=FACE_OUTER_BOUND('',#24275,.T.) ;
#18511=FACE_OUTER_BOUND('',#24276,.T.) ;
#18512=FACE_OUTER_BOUND('',#24277,.T.) ;
#18513=FACE_OUTER_BOUND('',#24278,.T.) ;
#18514=FACE_OUTER_BOUND('',#24279,.T.) ;
#18515=FACE_OUTER_BOUND('',#24280,.T.) ;
#18516=FACE_OUTER_BOUND('',#24281,.T.) ;
#18517=FACE_OUTER_BOUND('',#24282,.T.) ;
#18518=FACE_OUTER_BOUND('',#24283,.T.) ;
#18519=FACE_OUTER_BOUND('',#24284,.T.) ;
#18520=FACE_OUTER_BOUND('',#24285,.T.) ;
#18521=FACE_OUTER_BOUND('',#24286,.T.) ;
#18522=FACE_OUTER_BOUND('',#24287,.T.) ;
#18523=FACE_OUTER_BOUND('',#24288,.T.) ;
#18524=FACE_OUTER_BOUND('',#24289,.T.) ;
#18525=FACE_OUTER_BOUND('',#24290,.T.) ;
#18526=FACE_OUTER_BOUND('',#24291,.T.) ;
#18527=FACE_OUTER_BOUND('',#24292,.T.) ;
#18528=FACE_OUTER_BOUND('',#24293,.T.) ;
#18529=FACE_OUTER_BOUND('',#24294,.T.) ;
#18530=FACE_OUTER_BOUND('',#24295,.T.) ;
#18531=FACE_OUTER_BOUND('',#24296,.T.) ;
#18532=FACE_OUTER_BOUND('',#24297,.T.) ;
#18533=FACE_OUTER_BOUND('',#24298,.T.) ;
#18534=FACE_OUTER_BOUND('',#24299,.T.) ;
#18535=FACE_OUTER_BOUND('',#24300,.T.) ;
#18536=FACE_OUTER_BOUND('',#24301,.T.) ;
#18537=FACE_OUTER_BOUND('',#24302,.T.) ;
#18538=FACE_OUTER_BOUND('',#24303,.T.) ;
#18539=FACE_OUTER_BOUND('',#24304,.T.) ;
#18540=FACE_OUTER_BOUND('',#24305,.T.) ;
#18541=FACE_OUTER_BOUND('',#24306,.T.) ;
#18542=FACE_OUTER_BOUND('',#24307,.T.) ;
#18543=FACE_OUTER_BOUND('',#24308,.T.) ;
#18544=FACE_OUTER_BOUND('',#24309,.T.) ;
#18545=FACE_OUTER_BOUND('',#24310,.T.) ;
#18546=FACE_OUTER_BOUND('',#24311,.T.) ;
#18547=FACE_OUTER_BOUND('',#24312,.T.) ;
#18548=FACE_OUTER_BOUND('',#24313,.T.) ;
#18549=FACE_OUTER_BOUND('',#24314,.T.) ;
#18550=FACE_OUTER_BOUND('',#24315,.T.) ;
#18551=FACE_OUTER_BOUND('',#24316,.T.) ;
#18552=FACE_OUTER_BOUND('',#24317,.T.) ;
#18553=FACE_OUTER_BOUND('',#24318,.T.) ;
#18554=FACE_OUTER_BOUND('',#24319,.T.) ;
#18555=FACE_OUTER_BOUND('',#24320,.T.) ;
#18556=FACE_OUTER_BOUND('',#24321,.T.) ;
#18557=FACE_OUTER_BOUND('',#24322,.T.) ;
#18558=FACE_OUTER_BOUND('',#24323,.T.) ;
#18559=FACE_OUTER_BOUND('',#24324,.T.) ;
#18560=FACE_OUTER_BOUND('',#24325,.T.) ;
#18561=FACE_OUTER_BOUND('',#24326,.T.) ;
#18562=FACE_OUTER_BOUND('',#24327,.T.) ;
#18563=FACE_OUTER_BOUND('',#24328,.T.) ;
#18564=FACE_OUTER_BOUND('',#24329,.T.) ;
#18565=FACE_OUTER_BOUND('',#24330,.T.) ;
#18566=FACE_OUTER_BOUND('',#24331,.T.) ;
#18567=FACE_OUTER_BOUND('',#24332,.T.) ;
#18568=FACE_OUTER_BOUND('',#24333,.T.) ;
#18569=FACE_OUTER_BOUND('',#24334,.T.) ;
#18570=FACE_OUTER_BOUND('',#24335,.T.) ;
#18571=FACE_OUTER_BOUND('',#24336,.T.) ;
#18572=FACE_OUTER_BOUND('',#24337,.T.) ;
#18573=FACE_OUTER_BOUND('',#24338,.T.) ;
#18574=FACE_OUTER_BOUND('',#24339,.T.) ;
#18575=FACE_OUTER_BOUND('',#24340,.T.) ;
#18576=FACE_OUTER_BOUND('',#24341,.T.) ;
#18577=FACE_OUTER_BOUND('',#24342,.T.) ;
#18578=FACE_OUTER_BOUND('',#24343,.T.) ;
#18579=FACE_OUTER_BOUND('',#24344,.T.) ;
#18580=FACE_OUTER_BOUND('',#24345,.T.) ;
#18581=FACE_OUTER_BOUND('',#24346,.T.) ;
#18582=FACE_OUTER_BOUND('',#24347,.T.) ;
#18583=FACE_OUTER_BOUND('',#24348,.T.) ;
#18584=FACE_OUTER_BOUND('',#24349,.T.) ;
#18585=FACE_OUTER_BOUND('',#24350,.T.) ;
#18586=FACE_OUTER_BOUND('',#24351,.T.) ;
#18587=FACE_OUTER_BOUND('',#24352,.T.) ;
#18588=FACE_OUTER_BOUND('',#24353,.T.) ;
#18589=FACE_OUTER_BOUND('',#24354,.T.) ;
#18590=FACE_OUTER_BOUND('',#24355,.T.) ;
#18591=FACE_OUTER_BOUND('',#24356,.T.) ;
#18592=FACE_OUTER_BOUND('',#24357,.T.) ;
#18593=FACE_OUTER_BOUND('',#24358,.T.) ;
#18594=FACE_OUTER_BOUND('',#24359,.T.) ;
#18595=FACE_OUTER_BOUND('',#24360,.T.) ;
#18596=FACE_OUTER_BOUND('',#24361,.T.) ;
#18597=FACE_OUTER_BOUND('',#24362,.T.) ;
#18598=FACE_OUTER_BOUND('',#24363,.T.) ;
#18599=FACE_OUTER_BOUND('',#24364,.T.) ;
#18600=FACE_OUTER_BOUND('',#24365,.T.) ;
#18601=FACE_OUTER_BOUND('',#24366,.T.) ;
#18602=FACE_OUTER_BOUND('',#24367,.T.) ;
#18603=FACE_OUTER_BOUND('',#24368,.T.) ;
#18604=FACE_OUTER_BOUND('',#24369,.T.) ;
#18605=FACE_OUTER_BOUND('',#24370,.T.) ;
#18606=FACE_OUTER_BOUND('',#24371,.T.) ;
#18607=FACE_OUTER_BOUND('',#24372,.T.) ;
#18608=FACE_OUTER_BOUND('',#24373,.T.) ;
#18609=FACE_OUTER_BOUND('',#24374,.T.) ;
#18610=FACE_OUTER_BOUND('',#24375,.T.) ;
#18611=FACE_OUTER_BOUND('',#24376,.T.) ;
#18612=FACE_OUTER_BOUND('',#24377,.T.) ;
#18613=FACE_OUTER_BOUND('',#24378,.T.) ;
#18614=FACE_OUTER_BOUND('',#24379,.T.) ;
#18615=FACE_OUTER_BOUND('',#24380,.T.) ;
#18616=FACE_OUTER_BOUND('',#24381,.T.) ;
#18617=FACE_OUTER_BOUND('',#24383,.T.) ;
#18618=FACE_OUTER_BOUND('',#24384,.T.) ;
#18619=FACE_OUTER_BOUND('',#24385,.T.) ;
#18620=FACE_OUTER_BOUND('',#24386,.T.) ;
#18621=FACE_OUTER_BOUND('',#24387,.T.) ;
#18622=FACE_OUTER_BOUND('',#24388,.T.) ;
#18623=FACE_OUTER_BOUND('',#24389,.T.) ;
#18624=FACE_OUTER_BOUND('',#24390,.T.) ;
#18625=FACE_OUTER_BOUND('',#24391,.T.) ;
#18626=FACE_OUTER_BOUND('',#24392,.T.) ;
#18627=FACE_OUTER_BOUND('',#24393,.T.) ;
#18628=FACE_OUTER_BOUND('',#24394,.T.) ;
#18629=FACE_OUTER_BOUND('',#24395,.T.) ;
#18630=FACE_OUTER_BOUND('',#24396,.T.) ;
#18631=FACE_OUTER_BOUND('',#24397,.T.) ;
#18632=FACE_OUTER_BOUND('',#24398,.T.) ;
#18633=FACE_OUTER_BOUND('',#24399,.T.) ;
#18634=FACE_OUTER_BOUND('',#24400,.T.) ;
#18635=FACE_OUTER_BOUND('',#24401,.T.) ;
#18636=FACE_OUTER_BOUND('',#24402,.T.) ;
#18637=FACE_OUTER_BOUND('',#24403,.T.) ;
#18638=FACE_OUTER_BOUND('',#24404,.T.) ;
#18639=FACE_OUTER_BOUND('',#24405,.T.) ;
#18640=FACE_OUTER_BOUND('',#24406,.T.) ;
#18641=FACE_OUTER_BOUND('',#24407,.T.) ;
#18642=FACE_OUTER_BOUND('',#24408,.T.) ;
#18643=FACE_OUTER_BOUND('',#24409,.T.) ;
#18644=FACE_OUTER_BOUND('',#24410,.T.) ;
#18645=FACE_OUTER_BOUND('',#24412,.T.) ;
#18646=FACE_OUTER_BOUND('',#24413,.T.) ;
#18647=FACE_OUTER_BOUND('',#24414,.T.) ;
#18648=FACE_OUTER_BOUND('',#24415,.T.) ;
#18649=FACE_OUTER_BOUND('',#24416,.T.) ;
#18650=FACE_OUTER_BOUND('',#24417,.T.) ;
#18651=FACE_OUTER_BOUND('',#24418,.T.) ;
#18652=FACE_OUTER_BOUND('',#24419,.T.) ;
#18653=FACE_OUTER_BOUND('',#24420,.T.) ;
#18654=FACE_OUTER_BOUND('',#24421,.T.) ;
#18655=FACE_OUTER_BOUND('',#24422,.T.) ;
#18656=FACE_OUTER_BOUND('',#24423,.T.) ;
#18657=FACE_OUTER_BOUND('',#24424,.T.) ;
#18658=FACE_OUTER_BOUND('',#24425,.T.) ;
#18659=FACE_OUTER_BOUND('',#24426,.T.) ;
#18660=FACE_OUTER_BOUND('',#24427,.T.) ;
#18661=FACE_OUTER_BOUND('',#24428,.T.) ;
#18662=FACE_OUTER_BOUND('',#24429,.T.) ;
#18663=FACE_OUTER_BOUND('',#24430,.T.) ;
#18664=FACE_OUTER_BOUND('',#24431,.T.) ;
#18665=FACE_OUTER_BOUND('',#24432,.T.) ;
#18666=FACE_OUTER_BOUND('',#24433,.T.) ;
#18667=FACE_OUTER_BOUND('',#24434,.T.) ;
#18668=FACE_OUTER_BOUND('',#24435,.T.) ;
#18669=FACE_OUTER_BOUND('',#24436,.T.) ;
#18670=FACE_OUTER_BOUND('',#24437,.T.) ;
#18671=FACE_OUTER_BOUND('',#24438,.T.) ;
#18672=FACE_OUTER_BOUND('',#24439,.T.) ;
#18673=FACE_OUTER_BOUND('',#24441,.T.) ;
#18674=FACE_OUTER_BOUND('',#24442,.T.) ;
#18675=FACE_OUTER_BOUND('',#24443,.T.) ;
#18676=FACE_OUTER_BOUND('',#24444,.T.) ;
#18677=FACE_OUTER_BOUND('',#24445,.T.) ;
#18678=FACE_OUTER_BOUND('',#24446,.T.) ;
#18679=FACE_OUTER_BOUND('',#24447,.T.) ;
#18680=FACE_OUTER_BOUND('',#24448,.T.) ;
#18681=FACE_OUTER_BOUND('',#24449,.T.) ;
#18682=FACE_OUTER_BOUND('',#24450,.T.) ;
#18683=FACE_OUTER_BOUND('',#24451,.T.) ;
#18684=FACE_OUTER_BOUND('',#24452,.T.) ;
#18685=FACE_OUTER_BOUND('',#24453,.T.) ;
#18686=FACE_OUTER_BOUND('',#24454,.T.) ;
#18687=FACE_OUTER_BOUND('',#24455,.T.) ;
#18688=FACE_OUTER_BOUND('',#24456,.T.) ;
#18689=FACE_OUTER_BOUND('',#24457,.T.) ;
#18690=FACE_OUTER_BOUND('',#24458,.T.) ;
#18691=FACE_OUTER_BOUND('',#24459,.T.) ;
#18692=FACE_OUTER_BOUND('',#24460,.T.) ;
#18693=FACE_OUTER_BOUND('',#24461,.T.) ;
#18694=FACE_OUTER_BOUND('',#24462,.T.) ;
#18695=FACE_OUTER_BOUND('',#24463,.T.) ;
#18696=FACE_OUTER_BOUND('',#24464,.T.) ;
#18697=FACE_OUTER_BOUND('',#24465,.T.) ;
#18698=FACE_OUTER_BOUND('',#24466,.T.) ;
#18699=FACE_OUTER_BOUND('',#24467,.T.) ;
#18700=FACE_OUTER_BOUND('',#24468,.T.) ;
#18701=FACE_OUTER_BOUND('',#24470,.T.) ;
#18702=FACE_OUTER_BOUND('',#24471,.T.) ;
#18703=FACE_OUTER_BOUND('',#24472,.T.) ;
#18704=FACE_OUTER_BOUND('',#24473,.T.) ;
#18705=FACE_OUTER_BOUND('',#24474,.T.) ;
#18706=FACE_OUTER_BOUND('',#24475,.T.) ;
#18707=FACE_OUTER_BOUND('',#24476,.T.) ;
#18708=FACE_OUTER_BOUND('',#24477,.T.) ;
#18709=FACE_OUTER_BOUND('',#24478,.T.) ;
#18710=FACE_OUTER_BOUND('',#24479,.T.) ;
#18711=FACE_OUTER_BOUND('',#24480,.T.) ;
#18712=FACE_OUTER_BOUND('',#24481,.T.) ;
#18713=FACE_OUTER_BOUND('',#24482,.T.) ;
#18714=FACE_OUTER_BOUND('',#24483,.T.) ;
#18715=FACE_OUTER_BOUND('',#24484,.T.) ;
#18716=FACE_OUTER_BOUND('',#24485,.T.) ;
#18717=FACE_OUTER_BOUND('',#24486,.T.) ;
#18718=FACE_OUTER_BOUND('',#24487,.T.) ;
#18719=FACE_OUTER_BOUND('',#24488,.T.) ;
#18720=FACE_OUTER_BOUND('',#24489,.T.) ;
#18721=FACE_OUTER_BOUND('',#24490,.T.) ;
#18722=FACE_OUTER_BOUND('',#24491,.T.) ;
#18723=FACE_OUTER_BOUND('',#24492,.T.) ;
#18724=FACE_OUTER_BOUND('',#24493,.T.) ;
#18725=FACE_OUTER_BOUND('',#24494,.T.) ;
#18726=FACE_OUTER_BOUND('',#24495,.T.) ;
#18727=FACE_OUTER_BOUND('',#24496,.T.) ;
#18728=FACE_OUTER_BOUND('',#24497,.T.) ;
#18729=FACE_OUTER_BOUND('',#24499,.T.) ;
#18730=FACE_OUTER_BOUND('',#24500,.T.) ;
#18731=FACE_OUTER_BOUND('',#24501,.T.) ;
#18732=FACE_OUTER_BOUND('',#24502,.T.) ;
#18733=FACE_OUTER_BOUND('',#24503,.T.) ;
#18734=FACE_OUTER_BOUND('',#24504,.T.) ;
#18735=FACE_OUTER_BOUND('',#24505,.T.) ;
#18736=FACE_OUTER_BOUND('',#24506,.T.) ;
#18737=FACE_OUTER_BOUND('',#24507,.T.) ;
#18738=FACE_OUTER_BOUND('',#24508,.T.) ;
#18739=FACE_OUTER_BOUND('',#24509,.T.) ;
#18740=FACE_OUTER_BOUND('',#24510,.T.) ;
#18741=FACE_OUTER_BOUND('',#24511,.T.) ;
#18742=FACE_OUTER_BOUND('',#24512,.T.) ;
#18743=FACE_OUTER_BOUND('',#24513,.T.) ;
#18744=FACE_OUTER_BOUND('',#24514,.T.) ;
#18745=FACE_OUTER_BOUND('',#24515,.T.) ;
#18746=FACE_OUTER_BOUND('',#24516,.T.) ;
#18747=FACE_OUTER_BOUND('',#24517,.T.) ;
#18748=FACE_OUTER_BOUND('',#24518,.T.) ;
#18749=FACE_OUTER_BOUND('',#24519,.T.) ;
#18750=FACE_OUTER_BOUND('',#24520,.T.) ;
#18751=FACE_OUTER_BOUND('',#24521,.T.) ;
#18752=FACE_OUTER_BOUND('',#24522,.T.) ;
#18753=FACE_OUTER_BOUND('',#24523,.T.) ;
#18754=FACE_OUTER_BOUND('',#24524,.T.) ;
#18755=FACE_OUTER_BOUND('',#24525,.T.) ;
#18756=FACE_OUTER_BOUND('',#24526,.T.) ;
#18757=FACE_OUTER_BOUND('',#24528,.T.) ;
#18758=FACE_OUTER_BOUND('',#24529,.T.) ;
#18759=FACE_OUTER_BOUND('',#24530,.T.) ;
#18760=FACE_OUTER_BOUND('',#24531,.T.) ;
#18761=FACE_OUTER_BOUND('',#24532,.T.) ;
#18762=FACE_OUTER_BOUND('',#24533,.T.) ;
#18763=FACE_OUTER_BOUND('',#24534,.T.) ;
#18764=FACE_OUTER_BOUND('',#24535,.T.) ;
#18765=FACE_OUTER_BOUND('',#24536,.T.) ;
#18766=FACE_OUTER_BOUND('',#24537,.T.) ;
#18767=FACE_OUTER_BOUND('',#24538,.T.) ;
#18768=FACE_OUTER_BOUND('',#24539,.T.) ;
#18769=FACE_OUTER_BOUND('',#24540,.T.) ;
#18770=FACE_OUTER_BOUND('',#24541,.T.) ;
#18771=FACE_OUTER_BOUND('',#24542,.T.) ;
#18772=FACE_OUTER_BOUND('',#24543,.T.) ;
#18773=FACE_OUTER_BOUND('',#24544,.T.) ;
#18774=FACE_OUTER_BOUND('',#24545,.T.) ;
#18775=FACE_OUTER_BOUND('',#24546,.T.) ;
#18776=FACE_OUTER_BOUND('',#24547,.T.) ;
#18777=FACE_OUTER_BOUND('',#24548,.T.) ;
#18778=FACE_OUTER_BOUND('',#24549,.T.) ;
#18779=FACE_OUTER_BOUND('',#24550,.T.) ;
#18780=FACE_OUTER_BOUND('',#24551,.T.) ;
#18781=FACE_OUTER_BOUND('',#24552,.T.) ;
#18782=FACE_OUTER_BOUND('',#24553,.T.) ;
#18783=FACE_OUTER_BOUND('',#24554,.T.) ;
#18784=FACE_OUTER_BOUND('',#24555,.T.) ;
#18785=FACE_OUTER_BOUND('',#24557,.T.) ;
#18786=FACE_OUTER_BOUND('',#24558,.T.) ;
#18787=FACE_OUTER_BOUND('',#24559,.T.) ;
#18788=FACE_OUTER_BOUND('',#24560,.T.) ;
#18789=FACE_OUTER_BOUND('',#24561,.T.) ;
#18790=FACE_OUTER_BOUND('',#24562,.T.) ;
#18791=FACE_OUTER_BOUND('',#24563,.T.) ;
#18792=FACE_OUTER_BOUND('',#24564,.T.) ;
#18793=FACE_OUTER_BOUND('',#24565,.T.) ;
#18794=FACE_OUTER_BOUND('',#24566,.T.) ;
#18795=FACE_OUTER_BOUND('',#24567,.T.) ;
#18796=FACE_OUTER_BOUND('',#24568,.T.) ;
#18797=FACE_OUTER_BOUND('',#24569,.T.) ;
#18798=FACE_OUTER_BOUND('',#24570,.T.) ;
#18799=FACE_OUTER_BOUND('',#24571,.T.) ;
#18800=FACE_OUTER_BOUND('',#24572,.T.) ;
#18801=FACE_OUTER_BOUND('',#24573,.T.) ;
#18802=FACE_OUTER_BOUND('',#24574,.T.) ;
#18803=FACE_OUTER_BOUND('',#24575,.T.) ;
#18804=FACE_OUTER_BOUND('',#24576,.T.) ;
#18805=FACE_OUTER_BOUND('',#24577,.T.) ;
#18806=FACE_OUTER_BOUND('',#24578,.T.) ;
#18807=FACE_OUTER_BOUND('',#24579,.T.) ;
#18808=FACE_OUTER_BOUND('',#24580,.T.) ;
#18809=FACE_OUTER_BOUND('',#24581,.T.) ;
#18810=FACE_OUTER_BOUND('',#24582,.T.) ;
#18811=FACE_OUTER_BOUND('',#24583,.T.) ;
#18812=FACE_OUTER_BOUND('',#24584,.T.) ;
#18813=FACE_OUTER_BOUND('',#24586,.T.) ;
#18814=FACE_OUTER_BOUND('',#24587,.T.) ;
#18815=FACE_OUTER_BOUND('',#24588,.T.) ;
#18816=FACE_OUTER_BOUND('',#24589,.T.) ;
#18817=FACE_OUTER_BOUND('',#24590,.T.) ;
#18818=FACE_OUTER_BOUND('',#24591,.T.) ;
#18819=FACE_OUTER_BOUND('',#24592,.T.) ;
#18820=FACE_OUTER_BOUND('',#24593,.T.) ;
#18821=FACE_OUTER_BOUND('',#24594,.T.) ;
#18822=FACE_OUTER_BOUND('',#24595,.T.) ;
#18823=FACE_OUTER_BOUND('',#24596,.T.) ;
#18824=FACE_OUTER_BOUND('',#24597,.T.) ;
#18825=FACE_OUTER_BOUND('',#24598,.T.) ;
#18826=FACE_OUTER_BOUND('',#24599,.T.) ;
#18827=FACE_OUTER_BOUND('',#24600,.T.) ;
#18828=FACE_OUTER_BOUND('',#24601,.T.) ;
#18829=FACE_OUTER_BOUND('',#24602,.T.) ;
#18830=FACE_OUTER_BOUND('',#24603,.T.) ;
#18831=FACE_OUTER_BOUND('',#24604,.T.) ;
#18832=FACE_OUTER_BOUND('',#24605,.T.) ;
#18833=FACE_OUTER_BOUND('',#24606,.T.) ;
#18834=FACE_OUTER_BOUND('',#24607,.T.) ;
#18835=FACE_OUTER_BOUND('',#24608,.T.) ;
#18836=FACE_OUTER_BOUND('',#24609,.T.) ;
#18837=FACE_OUTER_BOUND('',#24610,.T.) ;
#18838=FACE_OUTER_BOUND('',#24611,.T.) ;
#18839=FACE_OUTER_BOUND('',#24612,.T.) ;
#18840=FACE_OUTER_BOUND('',#24613,.T.) ;
#18841=FACE_OUTER_BOUND('',#24615,.T.) ;
#18842=FACE_OUTER_BOUND('',#24617,.T.) ;
#18843=FACE_OUTER_BOUND('',#24619,.T.) ;
#18844=FACE_OUTER_BOUND('',#24621,.T.) ;
#18845=FACE_OUTER_BOUND('',#24623,.T.) ;
#18846=FACE_OUTER_BOUND('',#24625,.T.) ;
#18847=FACE_OUTER_BOUND('',#24627,.T.) ;
#18848=FACE_OUTER_BOUND('',#24629,.T.) ;
#18849=FACE_OUTER_BOUND('',#24631,.T.) ;
#18850=FACE_OUTER_BOUND('',#24633,.T.) ;
#18851=FACE_OUTER_BOUND('',#24634,.T.) ;
#18852=FACE_OUTER_BOUND('',#24635,.T.) ;
#18853=FACE_OUTER_BOUND('',#24636,.T.) ;
#18854=FACE_OUTER_BOUND('',#24637,.T.) ;
#18855=FACE_OUTER_BOUND('',#24638,.T.) ;
#18856=FACE_OUTER_BOUND('',#24639,.T.) ;
#18857=FACE_OUTER_BOUND('',#24640,.T.) ;
#18858=FACE_OUTER_BOUND('',#24641,.T.) ;
#18859=FACE_OUTER_BOUND('',#24642,.T.) ;
#18860=FACE_OUTER_BOUND('',#24643,.T.) ;
#18861=FACE_OUTER_BOUND('',#24644,.T.) ;
#18862=FACE_OUTER_BOUND('',#24645,.T.) ;
#18863=FACE_OUTER_BOUND('',#24646,.T.) ;
#18864=FACE_OUTER_BOUND('',#24647,.T.) ;
#18865=FACE_OUTER_BOUND('',#24648,.T.) ;
#18866=FACE_OUTER_BOUND('',#24649,.T.) ;
#18867=FACE_OUTER_BOUND('',#24650,.T.) ;
#18868=FACE_OUTER_BOUND('',#24651,.T.) ;
#18869=FACE_OUTER_BOUND('',#24652,.T.) ;
#18870=FACE_OUTER_BOUND('',#24653,.T.) ;
#18871=FACE_OUTER_BOUND('',#24654,.T.) ;
#18872=FACE_OUTER_BOUND('',#24655,.T.) ;
#18873=FACE_OUTER_BOUND('',#24656,.T.) ;
#18874=FACE_OUTER_BOUND('',#24657,.T.) ;
#18875=FACE_OUTER_BOUND('',#24658,.T.) ;
#18876=FACE_OUTER_BOUND('',#24659,.T.) ;
#18877=FACE_OUTER_BOUND('',#24660,.T.) ;
#18878=FACE_OUTER_BOUND('',#24661,.T.) ;
#18879=FACE_OUTER_BOUND('',#24662,.T.) ;
#18880=FACE_OUTER_BOUND('',#24663,.T.) ;
#18881=FACE_OUTER_BOUND('',#24664,.T.) ;
#18882=FACE_OUTER_BOUND('',#24665,.T.) ;
#18883=FACE_OUTER_BOUND('',#24666,.T.) ;
#18884=FACE_OUTER_BOUND('',#24667,.T.) ;
#18885=FACE_OUTER_BOUND('',#24668,.T.) ;
#18886=FACE_OUTER_BOUND('',#24669,.T.) ;
#18887=FACE_OUTER_BOUND('',#24670,.T.) ;
#18888=FACE_OUTER_BOUND('',#24671,.T.) ;
#18889=FACE_OUTER_BOUND('',#24672,.T.) ;
#18890=FACE_OUTER_BOUND('',#24673,.T.) ;
#18891=FACE_OUTER_BOUND('',#24674,.T.) ;
#18892=FACE_OUTER_BOUND('',#24675,.T.) ;
#18893=FACE_OUTER_BOUND('',#24676,.T.) ;
#18894=FACE_OUTER_BOUND('',#24677,.T.) ;
#18895=FACE_OUTER_BOUND('',#24678,.T.) ;
#18896=FACE_OUTER_BOUND('',#24679,.T.) ;
#18897=FACE_OUTER_BOUND('',#24680,.T.) ;
#18898=FACE_OUTER_BOUND('',#24681,.T.) ;
#18899=FACE_OUTER_BOUND('',#24682,.T.) ;
#18900=FACE_OUTER_BOUND('',#24683,.T.) ;
#18901=FACE_OUTER_BOUND('',#24684,.T.) ;
#18902=FACE_OUTER_BOUND('',#24685,.T.) ;
#18903=FACE_OUTER_BOUND('',#24686,.T.) ;
#18904=FACE_OUTER_BOUND('',#24687,.T.) ;
#18905=FACE_OUTER_BOUND('',#24688,.T.) ;
#18906=FACE_OUTER_BOUND('',#24689,.T.) ;
#18907=FACE_OUTER_BOUND('',#24690,.T.) ;
#18908=FACE_OUTER_BOUND('',#24691,.T.) ;
#18909=FACE_OUTER_BOUND('',#24692,.T.) ;
#18910=FACE_OUTER_BOUND('',#24693,.T.) ;
#18911=FACE_OUTER_BOUND('',#24694,.T.) ;
#18912=FACE_OUTER_BOUND('',#24695,.T.) ;
#18913=FACE_OUTER_BOUND('',#24696,.T.) ;
#18914=FACE_OUTER_BOUND('',#24697,.T.) ;
#18915=FACE_OUTER_BOUND('',#24698,.T.) ;
#18916=FACE_OUTER_BOUND('',#24699,.T.) ;
#18917=FACE_OUTER_BOUND('',#24700,.T.) ;
#18918=FACE_OUTER_BOUND('',#24701,.T.) ;
#18919=FACE_OUTER_BOUND('',#24702,.T.) ;
#18920=FACE_OUTER_BOUND('',#24703,.T.) ;
#18921=FACE_OUTER_BOUND('',#24704,.T.) ;
#18922=FACE_OUTER_BOUND('',#24705,.T.) ;
#18923=FACE_OUTER_BOUND('',#24706,.T.) ;
#18924=FACE_OUTER_BOUND('',#24707,.T.) ;
#18925=FACE_OUTER_BOUND('',#24708,.T.) ;
#18926=FACE_OUTER_BOUND('',#24709,.T.) ;
#18927=FACE_OUTER_BOUND('',#24710,.T.) ;
#18928=FACE_OUTER_BOUND('',#24711,.T.) ;
#18929=FACE_OUTER_BOUND('',#24712,.T.) ;
#18930=FACE_OUTER_BOUND('',#24713,.T.) ;
#18931=FACE_OUTER_BOUND('',#24714,.T.) ;
#18932=FACE_OUTER_BOUND('',#24715,.T.) ;
#18933=FACE_OUTER_BOUND('',#24716,.T.) ;
#18934=FACE_OUTER_BOUND('',#24717,.T.) ;
#18935=FACE_OUTER_BOUND('',#24718,.T.) ;
#18936=FACE_OUTER_BOUND('',#24719,.T.) ;
#18937=FACE_OUTER_BOUND('',#24720,.T.) ;
#18938=FACE_OUTER_BOUND('',#24721,.T.) ;
#18939=FACE_OUTER_BOUND('',#24722,.T.) ;
#18940=FACE_OUTER_BOUND('',#24723,.T.) ;
#18941=FACE_OUTER_BOUND('',#24724,.T.) ;
#18942=FACE_OUTER_BOUND('',#24725,.T.) ;
#18943=FACE_OUTER_BOUND('',#24726,.T.) ;
#18944=FACE_OUTER_BOUND('',#24727,.T.) ;
#18945=FACE_OUTER_BOUND('',#24728,.T.) ;
#18946=FACE_OUTER_BOUND('',#24729,.T.) ;
#18947=FACE_OUTER_BOUND('',#24730,.T.) ;
#18948=FACE_OUTER_BOUND('',#24731,.T.) ;
#18949=FACE_OUTER_BOUND('',#24732,.T.) ;
#18950=FACE_OUTER_BOUND('',#24733,.T.) ;
#18951=FACE_OUTER_BOUND('',#24734,.T.) ;
#18952=FACE_OUTER_BOUND('',#24735,.T.) ;
#18953=FACE_OUTER_BOUND('',#24736,.T.) ;
#18954=FACE_OUTER_BOUND('',#24737,.T.) ;
#18955=FACE_OUTER_BOUND('',#24738,.T.) ;
#18956=FACE_OUTER_BOUND('',#24739,.T.) ;
#18957=FACE_OUTER_BOUND('',#24740,.T.) ;
#18958=FACE_OUTER_BOUND('',#24741,.T.) ;
#18959=FACE_OUTER_BOUND('',#24742,.T.) ;
#18960=FACE_OUTER_BOUND('',#24743,.T.) ;
#18961=FACE_OUTER_BOUND('',#24744,.T.) ;
#18962=FACE_OUTER_BOUND('',#24745,.T.) ;
#18963=FACE_OUTER_BOUND('',#24746,.T.) ;
#18964=FACE_OUTER_BOUND('',#24747,.T.) ;
#18965=FACE_OUTER_BOUND('',#24748,.T.) ;
#18966=FACE_OUTER_BOUND('',#24749,.T.) ;
#18967=FACE_OUTER_BOUND('',#24750,.T.) ;
#18968=FACE_OUTER_BOUND('',#24751,.T.) ;
#18969=FACE_OUTER_BOUND('',#24752,.T.) ;
#18970=FACE_OUTER_BOUND('',#24753,.T.) ;
#18971=FACE_OUTER_BOUND('',#24754,.T.) ;
#18972=FACE_OUTER_BOUND('',#24755,.T.) ;
#18973=FACE_OUTER_BOUND('',#24756,.T.) ;
#18974=FACE_OUTER_BOUND('',#24757,.T.) ;
#18975=FACE_OUTER_BOUND('',#24758,.T.) ;
#18976=FACE_OUTER_BOUND('',#24759,.T.) ;
#18977=FACE_OUTER_BOUND('',#24760,.T.) ;
#18978=FACE_OUTER_BOUND('',#24761,.T.) ;
#18979=FACE_OUTER_BOUND('',#24762,.T.) ;
#18980=FACE_OUTER_BOUND('',#24763,.T.) ;
#18981=FACE_OUTER_BOUND('',#24764,.T.) ;
#18982=FACE_OUTER_BOUND('',#24765,.T.) ;
#18983=FACE_OUTER_BOUND('',#24766,.T.) ;
#18984=FACE_OUTER_BOUND('',#24767,.T.) ;
#18985=FACE_OUTER_BOUND('',#24768,.T.) ;
#18986=FACE_OUTER_BOUND('',#24769,.T.) ;
#18987=FACE_OUTER_BOUND('',#24770,.T.) ;
#18988=FACE_OUTER_BOUND('',#24771,.T.) ;
#18989=FACE_OUTER_BOUND('',#24772,.T.) ;
#18990=FACE_OUTER_BOUND('',#24773,.T.) ;
#18991=FACE_OUTER_BOUND('',#24774,.T.) ;
#18992=FACE_OUTER_BOUND('',#24775,.T.) ;
#18993=FACE_OUTER_BOUND('',#24776,.T.) ;
#18994=FACE_OUTER_BOUND('',#24777,.T.) ;
#18995=FACE_OUTER_BOUND('',#24778,.T.) ;
#18996=FACE_OUTER_BOUND('',#24779,.T.) ;
#18997=FACE_OUTER_BOUND('',#24780,.T.) ;
#18998=FACE_OUTER_BOUND('',#24781,.T.) ;
#18999=FACE_OUTER_BOUND('',#24782,.T.) ;
#19000=FACE_OUTER_BOUND('',#24783,.T.) ;
#19001=FACE_OUTER_BOUND('',#24784,.T.) ;
#19002=FACE_OUTER_BOUND('',#24785,.T.) ;
#19003=FACE_OUTER_BOUND('',#24786,.T.) ;
#19004=FACE_OUTER_BOUND('',#24787,.T.) ;
#19005=FACE_OUTER_BOUND('',#24788,.T.) ;
#19006=FACE_OUTER_BOUND('',#24789,.T.) ;
#19007=FACE_OUTER_BOUND('',#24790,.T.) ;
#19008=FACE_OUTER_BOUND('',#24791,.T.) ;
#19009=FACE_OUTER_BOUND('',#24792,.T.) ;
#19010=FACE_OUTER_BOUND('',#24793,.T.) ;
#19011=FACE_OUTER_BOUND('',#24794,.T.) ;
#19012=FACE_OUTER_BOUND('',#24795,.T.) ;
#19013=FACE_OUTER_BOUND('',#24796,.T.) ;
#19014=FACE_OUTER_BOUND('',#24797,.T.) ;
#19015=FACE_OUTER_BOUND('',#24798,.T.) ;
#19016=FACE_OUTER_BOUND('',#24799,.T.) ;
#19017=FACE_OUTER_BOUND('',#24800,.T.) ;
#19018=FACE_OUTER_BOUND('',#24801,.T.) ;
#19019=FACE_OUTER_BOUND('',#24802,.T.) ;
#19020=FACE_OUTER_BOUND('',#24803,.T.) ;
#19021=FACE_OUTER_BOUND('',#24804,.T.) ;
#19022=FACE_OUTER_BOUND('',#24805,.T.) ;
#19023=FACE_OUTER_BOUND('',#24806,.T.) ;
#19024=FACE_OUTER_BOUND('',#24807,.T.) ;
#19025=FACE_OUTER_BOUND('',#24808,.T.) ;
#19026=FACE_OUTER_BOUND('',#24809,.T.) ;
#19027=FACE_OUTER_BOUND('',#24810,.T.) ;
#19028=FACE_OUTER_BOUND('',#24811,.T.) ;
#19029=FACE_OUTER_BOUND('',#24812,.T.) ;
#19030=FACE_OUTER_BOUND('',#24813,.T.) ;
#19031=FACE_OUTER_BOUND('',#24814,.T.) ;
#19032=FACE_OUTER_BOUND('',#24815,.T.) ;
#19033=FACE_OUTER_BOUND('',#24816,.T.) ;
#19034=FACE_OUTER_BOUND('',#24817,.T.) ;
#19035=FACE_OUTER_BOUND('',#24818,.T.) ;
#19036=FACE_OUTER_BOUND('',#24819,.T.) ;
#19037=FACE_OUTER_BOUND('',#24820,.T.) ;
#19038=FACE_OUTER_BOUND('',#24821,.T.) ;
#19039=FACE_OUTER_BOUND('',#24822,.T.) ;
#19040=FACE_OUTER_BOUND('',#24823,.T.) ;
#19041=FACE_OUTER_BOUND('',#24824,.T.) ;
#19042=FACE_OUTER_BOUND('',#24825,.T.) ;
#19043=FACE_OUTER_BOUND('',#24826,.T.) ;
#19044=FACE_OUTER_BOUND('',#24827,.T.) ;
#19045=FACE_OUTER_BOUND('',#24828,.T.) ;
#19046=FACE_OUTER_BOUND('',#24829,.T.) ;
#19047=FACE_OUTER_BOUND('',#24830,.T.) ;
#19048=FACE_OUTER_BOUND('',#24831,.T.) ;
#19049=FACE_OUTER_BOUND('',#24832,.T.) ;
#19050=FACE_OUTER_BOUND('',#24833,.T.) ;
#19051=FACE_OUTER_BOUND('',#24834,.T.) ;
#19052=FACE_OUTER_BOUND('',#24835,.T.) ;
#19053=FACE_OUTER_BOUND('',#24836,.T.) ;
#19054=FACE_OUTER_BOUND('',#24837,.T.) ;
#19055=FACE_OUTER_BOUND('',#24838,.T.) ;
#19056=FACE_OUTER_BOUND('',#24839,.T.) ;
#19057=FACE_OUTER_BOUND('',#24840,.T.) ;
#19058=FACE_OUTER_BOUND('',#24841,.T.) ;
#19059=FACE_OUTER_BOUND('',#24842,.T.) ;
#19060=FACE_OUTER_BOUND('',#24843,.T.) ;
#19061=FACE_OUTER_BOUND('',#24844,.T.) ;
#19062=FACE_OUTER_BOUND('',#24845,.T.) ;
#19063=FACE_OUTER_BOUND('',#24846,.T.) ;
#19064=FACE_OUTER_BOUND('',#24847,.T.) ;
#19065=FACE_OUTER_BOUND('',#24848,.T.) ;
#19066=FACE_OUTER_BOUND('',#24849,.T.) ;
#19067=FACE_OUTER_BOUND('',#24850,.T.) ;
#19068=FACE_OUTER_BOUND('',#24851,.T.) ;
#19069=FACE_OUTER_BOUND('',#24852,.T.) ;
#19070=FACE_OUTER_BOUND('',#24853,.T.) ;
#19071=FACE_OUTER_BOUND('',#24854,.T.) ;
#19072=FACE_OUTER_BOUND('',#24855,.T.) ;
#19073=FACE_OUTER_BOUND('',#24856,.T.) ;
#19074=FACE_OUTER_BOUND('',#24857,.T.) ;
#19075=FACE_OUTER_BOUND('',#24858,.T.) ;
#19076=FACE_OUTER_BOUND('',#24859,.T.) ;
#19077=FACE_OUTER_BOUND('',#24860,.T.) ;
#19078=FACE_OUTER_BOUND('',#24861,.T.) ;
#19079=FACE_OUTER_BOUND('',#24862,.T.) ;
#19080=FACE_OUTER_BOUND('',#24863,.T.) ;
#19081=FACE_OUTER_BOUND('',#24864,.T.) ;
#19082=FACE_OUTER_BOUND('',#24865,.T.) ;
#19083=FACE_OUTER_BOUND('',#24866,.T.) ;
#19084=FACE_OUTER_BOUND('',#24867,.T.) ;
#19085=FACE_OUTER_BOUND('',#24868,.T.) ;
#19086=FACE_OUTER_BOUND('',#24869,.T.) ;
#19087=FACE_OUTER_BOUND('',#24870,.T.) ;
#19088=FACE_OUTER_BOUND('',#24871,.T.) ;
#19089=FACE_OUTER_BOUND('',#24872,.T.) ;
#19090=FACE_OUTER_BOUND('',#24873,.T.) ;
#19091=FACE_OUTER_BOUND('',#24874,.T.) ;
#19092=FACE_OUTER_BOUND('',#24875,.T.) ;
#19093=FACE_OUTER_BOUND('',#24876,.T.) ;
#19094=FACE_OUTER_BOUND('',#24877,.T.) ;
#19095=FACE_OUTER_BOUND('',#24878,.T.) ;
#19096=FACE_OUTER_BOUND('',#24879,.T.) ;
#19097=FACE_OUTER_BOUND('',#24880,.T.) ;
#19098=FACE_OUTER_BOUND('',#24881,.T.) ;
#19099=FACE_OUTER_BOUND('',#24882,.T.) ;
#19100=FACE_OUTER_BOUND('',#24883,.T.) ;
#19101=FACE_OUTER_BOUND('',#24884,.T.) ;
#19102=FACE_OUTER_BOUND('',#24885,.T.) ;
#19103=FACE_OUTER_BOUND('',#24886,.T.) ;
#19104=FACE_OUTER_BOUND('',#24887,.T.) ;
#19105=FACE_OUTER_BOUND('',#24888,.T.) ;
#19106=FACE_OUTER_BOUND('',#24889,.T.) ;
#19107=FACE_OUTER_BOUND('',#24890,.T.) ;
#19108=FACE_OUTER_BOUND('',#24891,.T.) ;
#19109=FACE_OUTER_BOUND('',#24892,.T.) ;
#19110=FACE_OUTER_BOUND('',#24893,.T.) ;
#19111=FACE_OUTER_BOUND('',#24894,.T.) ;
#19112=FACE_OUTER_BOUND('',#24895,.T.) ;
#19113=FACE_OUTER_BOUND('',#24896,.T.) ;
#19114=FACE_OUTER_BOUND('',#24897,.T.) ;
#19115=FACE_OUTER_BOUND('',#24898,.T.) ;
#19116=FACE_OUTER_BOUND('',#24899,.T.) ;
#19117=FACE_OUTER_BOUND('',#24900,.T.) ;
#19118=FACE_OUTER_BOUND('',#24901,.T.) ;
#19119=FACE_OUTER_BOUND('',#24902,.T.) ;
#19120=FACE_OUTER_BOUND('',#24903,.T.) ;
#19121=FACE_OUTER_BOUND('',#24904,.T.) ;
#19122=FACE_OUTER_BOUND('',#24905,.T.) ;
#19123=FACE_OUTER_BOUND('',#24906,.T.) ;
#19124=FACE_OUTER_BOUND('',#24907,.T.) ;
#19125=FACE_OUTER_BOUND('',#24908,.T.) ;
#19126=FACE_OUTER_BOUND('',#24909,.T.) ;
#19127=FACE_OUTER_BOUND('',#24910,.T.) ;
#19128=FACE_OUTER_BOUND('',#24911,.T.) ;
#19129=FACE_OUTER_BOUND('',#24912,.T.) ;
#19130=FACE_OUTER_BOUND('',#24913,.T.) ;
#19131=FACE_OUTER_BOUND('',#24914,.T.) ;
#19132=FACE_OUTER_BOUND('',#24915,.T.) ;
#19133=FACE_OUTER_BOUND('',#24916,.T.) ;
#19134=FACE_OUTER_BOUND('',#24917,.T.) ;
#19135=FACE_OUTER_BOUND('',#24918,.T.) ;
#19136=FACE_OUTER_BOUND('',#24919,.T.) ;
#19137=FACE_OUTER_BOUND('',#24920,.T.) ;
#19138=FACE_OUTER_BOUND('',#24921,.T.) ;
#19139=FACE_OUTER_BOUND('',#24922,.T.) ;
#19140=FACE_OUTER_BOUND('',#24923,.T.) ;
#19141=FACE_OUTER_BOUND('',#24924,.T.) ;
#19142=FACE_OUTER_BOUND('',#24925,.T.) ;
#19143=FACE_OUTER_BOUND('',#24926,.T.) ;
#19144=FACE_OUTER_BOUND('',#24927,.T.) ;
#19145=FACE_OUTER_BOUND('',#24928,.T.) ;
#19146=FACE_OUTER_BOUND('',#24929,.T.) ;
#19147=FACE_OUTER_BOUND('',#24930,.T.) ;
#19148=FACE_OUTER_BOUND('',#24931,.T.) ;
#19149=FACE_OUTER_BOUND('',#24932,.T.) ;
#19150=FACE_OUTER_BOUND('',#24933,.T.) ;
#19151=FACE_OUTER_BOUND('',#24934,.T.) ;
#19152=FACE_OUTER_BOUND('',#24935,.T.) ;
#19153=FACE_OUTER_BOUND('',#24936,.T.) ;
#19154=FACE_OUTER_BOUND('',#24937,.T.) ;
#19155=FACE_OUTER_BOUND('',#24938,.T.) ;
#19156=FACE_OUTER_BOUND('',#24939,.T.) ;
#19157=FACE_OUTER_BOUND('',#24940,.T.) ;
#19158=FACE_OUTER_BOUND('',#24941,.T.) ;
#19159=FACE_OUTER_BOUND('',#24942,.T.) ;
#19160=FACE_OUTER_BOUND('',#24943,.T.) ;
#19161=FACE_OUTER_BOUND('',#24944,.T.) ;
#19162=FACE_OUTER_BOUND('',#24945,.T.) ;
#19163=FACE_OUTER_BOUND('',#24946,.T.) ;
#19164=FACE_OUTER_BOUND('',#24947,.T.) ;
#19165=FACE_OUTER_BOUND('',#24948,.T.) ;
#19166=FACE_OUTER_BOUND('',#24949,.T.) ;
#19167=FACE_OUTER_BOUND('',#24950,.T.) ;
#19168=FACE_OUTER_BOUND('',#24951,.T.) ;
#19169=FACE_OUTER_BOUND('',#24952,.T.) ;
#19170=FACE_OUTER_BOUND('',#24953,.T.) ;
#19171=FACE_OUTER_BOUND('',#24954,.T.) ;
#19172=FACE_OUTER_BOUND('',#24955,.T.) ;
#19173=FACE_OUTER_BOUND('',#24956,.T.) ;
#19174=FACE_OUTER_BOUND('',#24957,.T.) ;
#19175=FACE_OUTER_BOUND('',#24958,.T.) ;
#19176=FACE_OUTER_BOUND('',#24959,.T.) ;
#19177=FACE_OUTER_BOUND('',#24960,.T.) ;
#19178=FACE_OUTER_BOUND('',#24961,.T.) ;
#19179=FACE_OUTER_BOUND('',#24962,.T.) ;
#19180=FACE_OUTER_BOUND('',#24963,.T.) ;
#19181=FACE_OUTER_BOUND('',#24964,.T.) ;
#19182=FACE_OUTER_BOUND('',#24965,.T.) ;
#19183=FACE_OUTER_BOUND('',#24966,.T.) ;
#19184=FACE_OUTER_BOUND('',#24967,.T.) ;
#19185=FACE_OUTER_BOUND('',#24968,.T.) ;
#19186=FACE_OUTER_BOUND('',#24969,.T.) ;
#19187=FACE_OUTER_BOUND('',#24970,.T.) ;
#19188=FACE_OUTER_BOUND('',#24971,.T.) ;
#19189=FACE_OUTER_BOUND('',#24972,.T.) ;
#19190=FACE_OUTER_BOUND('',#24973,.T.) ;
#19191=FACE_OUTER_BOUND('',#24974,.T.) ;
#19192=FACE_OUTER_BOUND('',#24975,.T.) ;
#19193=FACE_OUTER_BOUND('',#24976,.T.) ;
#19194=FACE_OUTER_BOUND('',#24977,.T.) ;
#19195=FACE_OUTER_BOUND('',#24978,.T.) ;
#19196=FACE_OUTER_BOUND('',#24979,.T.) ;
#19197=FACE_OUTER_BOUND('',#24980,.T.) ;
#19198=FACE_OUTER_BOUND('',#24981,.T.) ;
#19199=FACE_OUTER_BOUND('',#24982,.T.) ;
#19200=FACE_OUTER_BOUND('',#24983,.T.) ;
#19201=FACE_OUTER_BOUND('',#24984,.T.) ;
#19202=FACE_OUTER_BOUND('',#24985,.T.) ;
#19203=FACE_OUTER_BOUND('',#24986,.T.) ;
#19204=FACE_OUTER_BOUND('',#24987,.T.) ;
#19205=FACE_OUTER_BOUND('',#24988,.T.) ;
#19206=FACE_OUTER_BOUND('',#24989,.T.) ;
#19207=FACE_OUTER_BOUND('',#24990,.T.) ;
#19208=FACE_OUTER_BOUND('',#24991,.T.) ;
#19209=FACE_OUTER_BOUND('',#24992,.T.) ;
#19210=FACE_OUTER_BOUND('',#24993,.T.) ;
#19211=FACE_OUTER_BOUND('',#24994,.T.) ;
#19212=FACE_OUTER_BOUND('',#24995,.T.) ;
#19213=FACE_OUTER_BOUND('',#24996,.T.) ;
#19214=FACE_OUTER_BOUND('',#24997,.T.) ;
#19215=FACE_OUTER_BOUND('',#24998,.T.) ;
#19216=FACE_OUTER_BOUND('',#24999,.T.) ;
#19217=FACE_OUTER_BOUND('',#25000,.T.) ;
#19218=FACE_OUTER_BOUND('',#25001,.T.) ;
#19219=FACE_OUTER_BOUND('',#25002,.T.) ;
#19220=FACE_OUTER_BOUND('',#25003,.T.) ;
#19221=FACE_OUTER_BOUND('',#25004,.T.) ;
#19222=FACE_OUTER_BOUND('',#25005,.T.) ;
#19223=FACE_OUTER_BOUND('',#25006,.T.) ;
#19224=FACE_OUTER_BOUND('',#25007,.T.) ;
#19225=FACE_OUTER_BOUND('',#25008,.T.) ;
#19226=FACE_OUTER_BOUND('',#25009,.T.) ;
#19227=FACE_OUTER_BOUND('',#25010,.T.) ;
#19228=FACE_OUTER_BOUND('',#25011,.T.) ;
#19229=FACE_OUTER_BOUND('',#25012,.T.) ;
#19230=FACE_OUTER_BOUND('',#25013,.T.) ;
#19231=FACE_OUTER_BOUND('',#25014,.T.) ;
#19232=FACE_OUTER_BOUND('',#25015,.T.) ;
#19233=FACE_OUTER_BOUND('',#25016,.T.) ;
#19234=FACE_OUTER_BOUND('',#25017,.T.) ;
#19235=FACE_OUTER_BOUND('',#25018,.T.) ;
#19236=FACE_OUTER_BOUND('',#25019,.T.) ;
#19237=FACE_OUTER_BOUND('',#25020,.T.) ;
#19238=FACE_OUTER_BOUND('',#25021,.T.) ;
#19239=FACE_OUTER_BOUND('',#25022,.T.) ;
#19240=FACE_OUTER_BOUND('',#25023,.T.) ;
#19241=FACE_OUTER_BOUND('',#25024,.T.) ;
#19242=FACE_OUTER_BOUND('',#25025,.T.) ;
#19243=FACE_OUTER_BOUND('',#25026,.T.) ;
#19244=FACE_OUTER_BOUND('',#25027,.T.) ;
#19245=FACE_OUTER_BOUND('',#25028,.T.) ;
#19246=FACE_OUTER_BOUND('',#25029,.T.) ;
#19247=FACE_OUTER_BOUND('',#25030,.T.) ;
#19248=FACE_OUTER_BOUND('',#25031,.T.) ;
#19249=FACE_OUTER_BOUND('',#25032,.T.) ;
#19250=FACE_OUTER_BOUND('',#25033,.T.) ;
#19251=FACE_OUTER_BOUND('',#25034,.T.) ;
#19252=FACE_OUTER_BOUND('',#25035,.T.) ;
#19253=FACE_OUTER_BOUND('',#25036,.T.) ;
#19254=FACE_OUTER_BOUND('',#25037,.T.) ;
#19255=FACE_OUTER_BOUND('',#25038,.T.) ;
#19256=FACE_OUTER_BOUND('',#25039,.T.) ;
#19257=FACE_OUTER_BOUND('',#25040,.T.) ;
#19258=FACE_OUTER_BOUND('',#25041,.T.) ;
#19259=FACE_OUTER_BOUND('',#25042,.T.) ;
#19260=FACE_OUTER_BOUND('',#25043,.T.) ;
#19261=FACE_OUTER_BOUND('',#25044,.T.) ;
#19262=FACE_OUTER_BOUND('',#25045,.T.) ;
#19263=FACE_OUTER_BOUND('',#25046,.T.) ;
#19264=FACE_OUTER_BOUND('',#25047,.T.) ;
#19265=FACE_OUTER_BOUND('',#25048,.T.) ;
#19266=FACE_OUTER_BOUND('',#25049,.T.) ;
#19267=FACE_OUTER_BOUND('',#25050,.T.) ;
#19268=FACE_OUTER_BOUND('',#25051,.T.) ;
#19269=FACE_OUTER_BOUND('',#25052,.T.) ;
#19270=FACE_OUTER_BOUND('',#25053,.T.) ;
#19271=FACE_OUTER_BOUND('',#25054,.T.) ;
#19272=FACE_OUTER_BOUND('',#25055,.T.) ;
#19273=FACE_OUTER_BOUND('',#25056,.T.) ;
#19274=FACE_OUTER_BOUND('',#25057,.T.) ;
#19275=FACE_OUTER_BOUND('',#25058,.T.) ;
#19276=FACE_OUTER_BOUND('',#25059,.T.) ;
#19277=FACE_OUTER_BOUND('',#25060,.T.) ;
#19278=FACE_OUTER_BOUND('',#25061,.T.) ;
#19279=FACE_OUTER_BOUND('',#25062,.T.) ;
#19280=FACE_OUTER_BOUND('',#25063,.T.) ;
#19281=FACE_OUTER_BOUND('',#25064,.T.) ;
#19282=FACE_OUTER_BOUND('',#25065,.T.) ;
#19283=FACE_OUTER_BOUND('',#25066,.T.) ;
#19284=FACE_OUTER_BOUND('',#25067,.T.) ;
#19285=FACE_OUTER_BOUND('',#25068,.T.) ;
#19286=FACE_OUTER_BOUND('',#25069,.T.) ;
#19287=FACE_OUTER_BOUND('',#25070,.T.) ;
#19288=FACE_OUTER_BOUND('',#25071,.T.) ;
#19289=FACE_OUTER_BOUND('',#25072,.T.) ;
#19290=FACE_OUTER_BOUND('',#25073,.T.) ;
#19291=FACE_OUTER_BOUND('',#25074,.T.) ;
#19292=FACE_OUTER_BOUND('',#25075,.T.) ;
#19293=FACE_OUTER_BOUND('',#25076,.T.) ;
#19294=FACE_OUTER_BOUND('',#25077,.T.) ;
#19295=FACE_OUTER_BOUND('',#25078,.T.) ;
#19296=FACE_OUTER_BOUND('',#25079,.T.) ;
#19297=FACE_OUTER_BOUND('',#25080,.T.) ;
#19298=FACE_OUTER_BOUND('',#25081,.T.) ;
#19299=FACE_OUTER_BOUND('',#25082,.T.) ;
#19300=FACE_OUTER_BOUND('',#25083,.T.) ;
#19301=FACE_OUTER_BOUND('',#25084,.T.) ;
#19302=FACE_OUTER_BOUND('',#25085,.T.) ;
#19303=FACE_OUTER_BOUND('',#25086,.T.) ;
#19304=FACE_OUTER_BOUND('',#25087,.T.) ;
#19305=FACE_OUTER_BOUND('',#25088,.T.) ;
#19306=FACE_OUTER_BOUND('',#25089,.T.) ;
#19307=FACE_OUTER_BOUND('',#25090,.T.) ;
#19308=FACE_OUTER_BOUND('',#25091,.T.) ;
#19309=FACE_OUTER_BOUND('',#25092,.T.) ;
#19310=FACE_OUTER_BOUND('',#25093,.T.) ;
#19311=FACE_OUTER_BOUND('',#25094,.T.) ;
#19312=FACE_OUTER_BOUND('',#25095,.T.) ;
#19313=FACE_OUTER_BOUND('',#25096,.T.) ;
#19314=FACE_OUTER_BOUND('',#25097,.T.) ;
#19315=FACE_OUTER_BOUND('',#25098,.T.) ;
#19316=FACE_OUTER_BOUND('',#25099,.T.) ;
#19317=FACE_OUTER_BOUND('',#25100,.T.) ;
#19318=FACE_OUTER_BOUND('',#25101,.T.) ;
#19319=FACE_OUTER_BOUND('',#25102,.T.) ;
#19320=FACE_OUTER_BOUND('',#25103,.T.) ;
#19321=FACE_OUTER_BOUND('',#25104,.T.) ;
#19322=FACE_OUTER_BOUND('',#25105,.T.) ;
#19323=FACE_OUTER_BOUND('',#25106,.T.) ;
#19324=FACE_OUTER_BOUND('',#25107,.T.) ;
#19325=FACE_OUTER_BOUND('',#25108,.T.) ;
#19326=FACE_OUTER_BOUND('',#25109,.T.) ;
#19327=FACE_OUTER_BOUND('',#25110,.T.) ;
#19328=FACE_OUTER_BOUND('',#25111,.T.) ;
#19329=FACE_OUTER_BOUND('',#25112,.T.) ;
#19330=FACE_OUTER_BOUND('',#25113,.T.) ;
#19331=FACE_OUTER_BOUND('',#25114,.T.) ;
#19332=FACE_OUTER_BOUND('',#25115,.T.) ;
#19333=FACE_OUTER_BOUND('',#25116,.T.) ;
#19334=FACE_OUTER_BOUND('',#25117,.T.) ;
#19335=FACE_OUTER_BOUND('',#25118,.T.) ;
#19336=FACE_OUTER_BOUND('',#25119,.T.) ;
#19337=FACE_OUTER_BOUND('',#25120,.T.) ;
#19338=FACE_OUTER_BOUND('',#25121,.T.) ;
#19339=FACE_OUTER_BOUND('',#25122,.T.) ;
#19340=FACE_OUTER_BOUND('',#25123,.T.) ;
#19341=FACE_OUTER_BOUND('',#25124,.T.) ;
#19342=FACE_OUTER_BOUND('',#25125,.T.) ;
#19343=FACE_OUTER_BOUND('',#25126,.T.) ;
#19344=FACE_OUTER_BOUND('',#25127,.T.) ;
#19345=FACE_OUTER_BOUND('',#25128,.T.) ;
#19346=FACE_OUTER_BOUND('',#25129,.T.) ;
#19347=FACE_OUTER_BOUND('',#25130,.T.) ;
#19348=FACE_OUTER_BOUND('',#25131,.T.) ;
#19349=FACE_OUTER_BOUND('',#25132,.T.) ;
#19350=FACE_OUTER_BOUND('',#25133,.T.) ;
#19351=FACE_OUTER_BOUND('',#25134,.T.) ;
#19352=FACE_OUTER_BOUND('',#25135,.T.) ;
#19353=FACE_OUTER_BOUND('',#25136,.T.) ;
#19354=FACE_OUTER_BOUND('',#25137,.T.) ;
#19355=FACE_OUTER_BOUND('',#25138,.T.) ;
#19356=FACE_OUTER_BOUND('',#25139,.T.) ;
#19357=FACE_OUTER_BOUND('',#25140,.T.) ;
#19358=FACE_OUTER_BOUND('',#25141,.T.) ;
#19359=FACE_OUTER_BOUND('',#25142,.T.) ;
#19360=FACE_OUTER_BOUND('',#25143,.T.) ;
#19361=FACE_OUTER_BOUND('',#25144,.T.) ;
#19362=FACE_OUTER_BOUND('',#25145,.T.) ;
#19363=FACE_OUTER_BOUND('',#25146,.T.) ;
#19364=FACE_OUTER_BOUND('',#25147,.T.) ;
#19365=FACE_OUTER_BOUND('',#25148,.T.) ;
#19366=FACE_OUTER_BOUND('',#25149,.T.) ;
#19367=FACE_OUTER_BOUND('',#25150,.T.) ;
#19368=FACE_OUTER_BOUND('',#25151,.T.) ;
#19369=FACE_OUTER_BOUND('',#25152,.T.) ;
#19370=FACE_OUTER_BOUND('',#25153,.T.) ;
#19371=FACE_OUTER_BOUND('',#25154,.T.) ;
#19372=FACE_OUTER_BOUND('',#25155,.T.) ;
#19373=FACE_OUTER_BOUND('',#25156,.T.) ;
#19374=FACE_OUTER_BOUND('',#25157,.T.) ;
#19375=FACE_OUTER_BOUND('',#25158,.T.) ;
#19376=FACE_OUTER_BOUND('',#25159,.T.) ;
#19377=FACE_OUTER_BOUND('',#25160,.T.) ;
#19378=FACE_OUTER_BOUND('',#25161,.T.) ;
#19379=FACE_OUTER_BOUND('',#25162,.T.) ;
#19380=FACE_OUTER_BOUND('',#25163,.T.) ;
#19381=FACE_OUTER_BOUND('',#25164,.T.) ;
#19382=FACE_OUTER_BOUND('',#25165,.T.) ;
#19383=FACE_OUTER_BOUND('',#25166,.T.) ;
#19384=FACE_OUTER_BOUND('',#25167,.T.) ;
#19385=FACE_OUTER_BOUND('',#25168,.T.) ;
#19386=FACE_OUTER_BOUND('',#25169,.T.) ;
#19387=FACE_OUTER_BOUND('',#25170,.T.) ;
#19388=FACE_OUTER_BOUND('',#25171,.T.) ;
#19389=FACE_OUTER_BOUND('',#25172,.T.) ;
#19390=FACE_OUTER_BOUND('',#25173,.T.) ;
#19391=FACE_OUTER_BOUND('',#25174,.T.) ;
#19392=FACE_OUTER_BOUND('',#25175,.T.) ;
#19393=FACE_OUTER_BOUND('',#25176,.T.) ;
#19394=FACE_OUTER_BOUND('',#25177,.T.) ;
#19395=FACE_OUTER_BOUND('',#25178,.T.) ;
#19396=FACE_OUTER_BOUND('',#25179,.T.) ;
#19397=FACE_OUTER_BOUND('',#25180,.T.) ;
#19398=FACE_OUTER_BOUND('',#25181,.T.) ;
#19399=FACE_OUTER_BOUND('',#25182,.T.) ;
#19400=FACE_OUTER_BOUND('',#25183,.T.) ;
#19401=FACE_OUTER_BOUND('',#25184,.T.) ;
#19402=FACE_OUTER_BOUND('',#25185,.T.) ;
#19403=FACE_OUTER_BOUND('',#25186,.T.) ;
#19404=FACE_OUTER_BOUND('',#25187,.T.) ;
#19405=FACE_OUTER_BOUND('',#25188,.T.) ;
#19406=FACE_OUTER_BOUND('',#25189,.T.) ;
#19407=FACE_OUTER_BOUND('',#25190,.T.) ;
#19408=FACE_OUTER_BOUND('',#25191,.T.) ;
#19409=FACE_OUTER_BOUND('',#25192,.T.) ;
#19410=FACE_OUTER_BOUND('',#25193,.T.) ;
#19411=FACE_OUTER_BOUND('',#25194,.T.) ;
#19412=FACE_OUTER_BOUND('',#25195,.T.) ;
#19413=FACE_OUTER_BOUND('',#25196,.T.) ;
#19414=FACE_OUTER_BOUND('',#25197,.T.) ;
#19415=FACE_OUTER_BOUND('',#25198,.T.) ;
#19416=FACE_OUTER_BOUND('',#25199,.T.) ;
#19417=FACE_OUTER_BOUND('',#25200,.T.) ;
#19418=FACE_OUTER_BOUND('',#25201,.T.) ;
#19419=FACE_OUTER_BOUND('',#25202,.T.) ;
#19420=FACE_OUTER_BOUND('',#25203,.T.) ;
#19421=FACE_OUTER_BOUND('',#25204,.T.) ;
#19422=FACE_OUTER_BOUND('',#25205,.T.) ;
#19423=FACE_OUTER_BOUND('',#25206,.T.) ;
#19424=FACE_OUTER_BOUND('',#25207,.T.) ;
#19425=FACE_OUTER_BOUND('',#25208,.T.) ;
#19426=FACE_OUTER_BOUND('',#25209,.T.) ;
#19427=FACE_OUTER_BOUND('',#25210,.T.) ;
#19428=FACE_OUTER_BOUND('',#25211,.T.) ;
#19429=FACE_OUTER_BOUND('',#25212,.T.) ;
#19430=FACE_OUTER_BOUND('',#25213,.T.) ;
#19431=FACE_OUTER_BOUND('',#25214,.T.) ;
#19432=FACE_OUTER_BOUND('',#25215,.T.) ;
#19433=FACE_OUTER_BOUND('',#25216,.T.) ;
#19434=FACE_OUTER_BOUND('',#25217,.T.) ;
#19435=FACE_OUTER_BOUND('',#25218,.T.) ;
#19436=FACE_OUTER_BOUND('',#25219,.T.) ;
#19437=FACE_OUTER_BOUND('',#25220,.T.) ;
#19438=FACE_OUTER_BOUND('',#25221,.T.) ;
#19439=FACE_OUTER_BOUND('',#25222,.T.) ;
#19440=FACE_OUTER_BOUND('',#25223,.T.) ;
#19441=FACE_OUTER_BOUND('',#25224,.T.) ;
#19442=FACE_OUTER_BOUND('',#25225,.T.) ;
#19443=FACE_OUTER_BOUND('',#25226,.T.) ;
#19444=FACE_OUTER_BOUND('',#25227,.T.) ;
#19445=FACE_OUTER_BOUND('',#25228,.T.) ;
#19446=FACE_OUTER_BOUND('',#25229,.T.) ;
#19447=FACE_OUTER_BOUND('',#25230,.T.) ;
#19448=FACE_OUTER_BOUND('',#25231,.T.) ;
#19449=FACE_OUTER_BOUND('',#25232,.T.) ;
#19450=FACE_OUTER_BOUND('',#25233,.T.) ;
#19451=FACE_OUTER_BOUND('',#25234,.T.) ;
#19452=FACE_OUTER_BOUND('',#25235,.T.) ;
#19453=FACE_OUTER_BOUND('',#25236,.T.) ;
#19454=FACE_OUTER_BOUND('',#25237,.T.) ;
#19455=FACE_OUTER_BOUND('',#25238,.T.) ;
#19456=FACE_OUTER_BOUND('',#25239,.T.) ;
#19457=FACE_OUTER_BOUND('',#25240,.T.) ;
#19458=FACE_OUTER_BOUND('',#25241,.T.) ;
#19459=FACE_OUTER_BOUND('',#25242,.T.) ;
#19460=FACE_OUTER_BOUND('',#25243,.T.) ;
#19461=FACE_OUTER_BOUND('',#25244,.T.) ;
#19462=FACE_OUTER_BOUND('',#25245,.T.) ;
#19463=FACE_OUTER_BOUND('',#25246,.T.) ;
#19464=FACE_OUTER_BOUND('',#25247,.T.) ;
#19465=FACE_OUTER_BOUND('',#25248,.T.) ;
#19466=FACE_OUTER_BOUND('',#25249,.T.) ;
#19467=FACE_OUTER_BOUND('',#25250,.T.) ;
#19468=FACE_OUTER_BOUND('',#25251,.T.) ;
#19469=FACE_OUTER_BOUND('',#25252,.T.) ;
#19470=FACE_OUTER_BOUND('',#25253,.T.) ;
#19471=FACE_OUTER_BOUND('',#25254,.T.) ;
#19472=FACE_OUTER_BOUND('',#25255,.T.) ;
#19473=FACE_OUTER_BOUND('',#25256,.T.) ;
#19474=FACE_OUTER_BOUND('',#25257,.T.) ;
#19475=FACE_OUTER_BOUND('',#25258,.T.) ;
#19476=FACE_OUTER_BOUND('',#25259,.T.) ;
#19477=FACE_OUTER_BOUND('',#25260,.T.) ;
#19478=FACE_OUTER_BOUND('',#25261,.T.) ;
#19479=FACE_OUTER_BOUND('',#25262,.T.) ;
#19480=FACE_OUTER_BOUND('',#25263,.T.) ;
#19481=FACE_OUTER_BOUND('',#25264,.T.) ;
#19482=FACE_OUTER_BOUND('',#25265,.T.) ;
#19483=FACE_OUTER_BOUND('',#25266,.T.) ;
#19484=FACE_OUTER_BOUND('',#25267,.T.) ;
#19485=FACE_OUTER_BOUND('',#25268,.T.) ;
#19486=FACE_OUTER_BOUND('',#25269,.T.) ;
#19487=FACE_OUTER_BOUND('',#25270,.T.) ;
#19488=FACE_OUTER_BOUND('',#25271,.T.) ;
#19489=FACE_OUTER_BOUND('',#25272,.T.) ;
#19490=FACE_OUTER_BOUND('',#25273,.T.) ;
#19491=FACE_OUTER_BOUND('',#25274,.T.) ;
#19492=FACE_OUTER_BOUND('',#25275,.T.) ;
#19493=FACE_OUTER_BOUND('',#25276,.T.) ;
#19494=FACE_OUTER_BOUND('',#25277,.T.) ;
#19495=FACE_OUTER_BOUND('',#25278,.T.) ;
#19496=FACE_OUTER_BOUND('',#25279,.T.) ;
#19497=FACE_OUTER_BOUND('',#25280,.T.) ;
#19498=FACE_OUTER_BOUND('',#25281,.T.) ;
#19499=FACE_OUTER_BOUND('',#25282,.T.) ;
#19500=FACE_OUTER_BOUND('',#25283,.T.) ;
#19501=FACE_OUTER_BOUND('',#25284,.T.) ;
#19502=FACE_OUTER_BOUND('',#25285,.T.) ;
#19503=FACE_OUTER_BOUND('',#25286,.T.) ;
#19504=FACE_OUTER_BOUND('',#25287,.T.) ;
#19505=FACE_OUTER_BOUND('',#25288,.T.) ;
#19506=FACE_OUTER_BOUND('',#25289,.T.) ;
#19507=FACE_OUTER_BOUND('',#25290,.T.) ;
#19508=FACE_OUTER_BOUND('',#25291,.T.) ;
#19509=FACE_OUTER_BOUND('',#25292,.T.) ;
#19510=FACE_OUTER_BOUND('',#25293,.T.) ;
#19511=FACE_OUTER_BOUND('',#25294,.T.) ;
#19512=FACE_OUTER_BOUND('',#25295,.T.) ;
#19513=FACE_OUTER_BOUND('',#25296,.T.) ;
#19514=FACE_OUTER_BOUND('',#25297,.T.) ;
#19515=FACE_OUTER_BOUND('',#25298,.T.) ;
#19516=FACE_OUTER_BOUND('',#25299,.T.) ;
#19517=FACE_OUTER_BOUND('',#25300,.T.) ;
#19518=FACE_OUTER_BOUND('',#25301,.T.) ;
#19519=FACE_OUTER_BOUND('',#25302,.T.) ;
#19520=FACE_OUTER_BOUND('',#25303,.T.) ;
#19521=FACE_OUTER_BOUND('',#25304,.T.) ;
#19522=FACE_OUTER_BOUND('',#25305,.T.) ;
#19523=FACE_OUTER_BOUND('',#25306,.T.) ;
#19524=FACE_OUTER_BOUND('',#25307,.T.) ;
#19525=FACE_OUTER_BOUND('',#25308,.T.) ;
#19526=FACE_OUTER_BOUND('',#25309,.T.) ;
#19527=FACE_OUTER_BOUND('',#25310,.T.) ;
#19528=FACE_OUTER_BOUND('',#25311,.T.) ;
#19529=FACE_OUTER_BOUND('',#25312,.T.) ;
#19530=FACE_OUTER_BOUND('',#25313,.T.) ;
#19531=FACE_OUTER_BOUND('',#25314,.T.) ;
#19532=FACE_OUTER_BOUND('',#25315,.T.) ;
#19533=FACE_OUTER_BOUND('',#25316,.T.) ;
#19534=FACE_OUTER_BOUND('',#25317,.T.) ;
#19535=FACE_OUTER_BOUND('',#25318,.T.) ;
#19536=FACE_OUTER_BOUND('',#25319,.T.) ;
#19537=FACE_OUTER_BOUND('',#25320,.T.) ;
#19538=FACE_OUTER_BOUND('',#25321,.T.) ;
#19539=FACE_OUTER_BOUND('',#25322,.T.) ;
#19540=FACE_OUTER_BOUND('',#25323,.T.) ;
#19541=FACE_OUTER_BOUND('',#25324,.T.) ;
#19542=FACE_OUTER_BOUND('',#25325,.T.) ;
#19543=FACE_OUTER_BOUND('',#25326,.T.) ;
#19544=FACE_OUTER_BOUND('',#25327,.T.) ;
#19545=FACE_OUTER_BOUND('',#25328,.T.) ;
#19546=FACE_OUTER_BOUND('',#25329,.T.) ;
#19547=FACE_OUTER_BOUND('',#25330,.T.) ;
#19548=FACE_OUTER_BOUND('',#25331,.T.) ;
#19549=FACE_OUTER_BOUND('',#25332,.T.) ;
#19550=FACE_OUTER_BOUND('',#25333,.T.) ;
#19551=FACE_OUTER_BOUND('',#25334,.T.) ;
#19552=FACE_OUTER_BOUND('',#25335,.T.) ;
#19553=FACE_OUTER_BOUND('',#25336,.T.) ;
#19554=FACE_OUTER_BOUND('',#25337,.T.) ;
#19555=FACE_OUTER_BOUND('',#25338,.T.) ;
#19556=FACE_OUTER_BOUND('',#25339,.T.) ;
#19557=FACE_OUTER_BOUND('',#25340,.T.) ;
#19558=FACE_OUTER_BOUND('',#25341,.T.) ;
#19559=FACE_OUTER_BOUND('',#25342,.T.) ;
#19560=FACE_OUTER_BOUND('',#25343,.T.) ;
#19561=FACE_OUTER_BOUND('',#25344,.T.) ;
#19562=FACE_OUTER_BOUND('',#25345,.T.) ;
#19563=FACE_OUTER_BOUND('',#25346,.T.) ;
#19564=FACE_OUTER_BOUND('',#25347,.T.) ;
#19565=FACE_OUTER_BOUND('',#25348,.T.) ;
#19566=FACE_OUTER_BOUND('',#25349,.T.) ;
#19567=FACE_OUTER_BOUND('',#25350,.T.) ;
#19568=FACE_OUTER_BOUND('',#25351,.T.) ;
#19569=FACE_OUTER_BOUND('',#25352,.T.) ;
#19570=FACE_OUTER_BOUND('',#25353,.T.) ;
#19571=FACE_OUTER_BOUND('',#25354,.T.) ;
#19572=FACE_OUTER_BOUND('',#25355,.T.) ;
#19573=FACE_OUTER_BOUND('',#25356,.T.) ;
#19574=FACE_OUTER_BOUND('',#25357,.T.) ;
#19575=FACE_OUTER_BOUND('',#25358,.T.) ;
#19576=FACE_OUTER_BOUND('',#25359,.T.) ;
#19577=FACE_OUTER_BOUND('',#25360,.T.) ;
#19578=FACE_OUTER_BOUND('',#25361,.T.) ;
#19579=FACE_OUTER_BOUND('',#25362,.T.) ;
#19580=FACE_OUTER_BOUND('',#25363,.T.) ;
#19581=FACE_OUTER_BOUND('',#25364,.T.) ;
#19582=FACE_OUTER_BOUND('',#25365,.T.) ;
#19583=FACE_OUTER_BOUND('',#25366,.T.) ;
#19584=FACE_OUTER_BOUND('',#25367,.T.) ;
#19585=FACE_OUTER_BOUND('',#25368,.T.) ;
#19586=FACE_OUTER_BOUND('',#25369,.T.) ;
#19587=FACE_OUTER_BOUND('',#25370,.T.) ;
#19588=FACE_OUTER_BOUND('',#25371,.T.) ;
#19589=FACE_OUTER_BOUND('',#25372,.T.) ;
#19590=FACE_OUTER_BOUND('',#25373,.T.) ;
#19591=FACE_OUTER_BOUND('',#25374,.T.) ;
#19592=FACE_OUTER_BOUND('',#25375,.T.) ;
#19593=FACE_OUTER_BOUND('',#25376,.T.) ;
#19594=FACE_OUTER_BOUND('',#25377,.T.) ;
#19595=FACE_OUTER_BOUND('',#25378,.T.) ;
#19596=FACE_OUTER_BOUND('',#25379,.T.) ;
#19597=FACE_OUTER_BOUND('',#25380,.T.) ;
#19598=FACE_OUTER_BOUND('',#25381,.T.) ;
#19599=FACE_OUTER_BOUND('',#25382,.T.) ;
#19600=FACE_OUTER_BOUND('',#25383,.T.) ;
#19601=FACE_OUTER_BOUND('',#25384,.T.) ;
#19602=FACE_OUTER_BOUND('',#25385,.T.) ;
#19603=FACE_OUTER_BOUND('',#25386,.T.) ;
#19604=FACE_OUTER_BOUND('',#25387,.T.) ;
#19605=FACE_OUTER_BOUND('',#25388,.T.) ;
#19606=FACE_OUTER_BOUND('',#25389,.T.) ;
#19607=FACE_OUTER_BOUND('',#25390,.T.) ;
#19608=FACE_OUTER_BOUND('',#25391,.T.) ;
#19609=FACE_OUTER_BOUND('',#25392,.T.) ;
#19610=FACE_OUTER_BOUND('',#25393,.T.) ;
#19611=FACE_OUTER_BOUND('',#25394,.T.) ;
#19612=FACE_OUTER_BOUND('',#25395,.T.) ;
#19613=FACE_OUTER_BOUND('',#25396,.T.) ;
#19614=FACE_OUTER_BOUND('',#25397,.T.) ;
#19615=FACE_OUTER_BOUND('',#25398,.T.) ;
#19616=FACE_OUTER_BOUND('',#25399,.T.) ;
#19617=FACE_OUTER_BOUND('',#25400,.T.) ;
#19618=FACE_OUTER_BOUND('',#25401,.T.) ;
#19619=FACE_OUTER_BOUND('',#25402,.T.) ;
#19620=FACE_OUTER_BOUND('',#25403,.T.) ;
#19621=FACE_OUTER_BOUND('',#25404,.T.) ;
#19622=FACE_OUTER_BOUND('',#25405,.T.) ;
#19623=FACE_OUTER_BOUND('',#25406,.T.) ;
#19624=FACE_OUTER_BOUND('',#25407,.T.) ;
#19625=FACE_OUTER_BOUND('',#25408,.T.) ;
#19626=FACE_OUTER_BOUND('',#25409,.T.) ;
#19627=FACE_OUTER_BOUND('',#25410,.T.) ;
#19628=FACE_OUTER_BOUND('',#25411,.T.) ;
#19629=FACE_OUTER_BOUND('',#25412,.T.) ;
#19630=FACE_OUTER_BOUND('',#25413,.T.) ;
#19631=FACE_OUTER_BOUND('',#25414,.T.) ;
#19632=FACE_OUTER_BOUND('',#25415,.T.) ;
#19633=FACE_OUTER_BOUND('',#25416,.T.) ;
#19634=FACE_OUTER_BOUND('',#25417,.T.) ;
#19635=FACE_OUTER_BOUND('',#25418,.T.) ;
#19636=FACE_OUTER_BOUND('',#25419,.T.) ;
#19637=FACE_OUTER_BOUND('',#25420,.T.) ;
#19638=FACE_OUTER_BOUND('',#25421,.T.) ;
#19639=FACE_OUTER_BOUND('',#25422,.T.) ;
#19640=FACE_OUTER_BOUND('',#25423,.T.) ;
#19641=FACE_OUTER_BOUND('',#25424,.T.) ;
#19642=FACE_OUTER_BOUND('',#25425,.T.) ;
#19643=FACE_OUTER_BOUND('',#25426,.T.) ;
#19644=FACE_OUTER_BOUND('',#25427,.T.) ;
#19645=FACE_OUTER_BOUND('',#25428,.T.) ;
#19646=FACE_OUTER_BOUND('',#25429,.T.) ;
#19647=FACE_OUTER_BOUND('',#25430,.T.) ;
#19648=FACE_OUTER_BOUND('',#25431,.T.) ;
#19649=FACE_OUTER_BOUND('',#25432,.T.) ;
#19650=FACE_OUTER_BOUND('',#25433,.T.) ;
#19651=FACE_OUTER_BOUND('',#25434,.T.) ;
#19652=FACE_OUTER_BOUND('',#25435,.T.) ;
#19653=FACE_OUTER_BOUND('',#25436,.T.) ;
#19654=FACE_OUTER_BOUND('',#25437,.T.) ;
#19655=FACE_OUTER_BOUND('',#25438,.T.) ;
#19656=FACE_OUTER_BOUND('',#25439,.T.) ;
#19657=FACE_OUTER_BOUND('',#25440,.T.) ;
#19658=FACE_OUTER_BOUND('',#25441,.T.) ;
#19659=FACE_OUTER_BOUND('',#25442,.T.) ;
#19660=FACE_OUTER_BOUND('',#25443,.T.) ;
#19661=FACE_OUTER_BOUND('',#25444,.T.) ;
#19662=FACE_OUTER_BOUND('',#25445,.T.) ;
#19663=FACE_OUTER_BOUND('',#25446,.T.) ;
#19664=FACE_OUTER_BOUND('',#25447,.T.) ;
#19665=FACE_OUTER_BOUND('',#25448,.T.) ;
#19666=FACE_OUTER_BOUND('',#25449,.T.) ;
#19667=FACE_OUTER_BOUND('',#25450,.T.) ;
#19668=FACE_OUTER_BOUND('',#25451,.T.) ;
#19669=FACE_OUTER_BOUND('',#25452,.T.) ;
#19670=FACE_OUTER_BOUND('',#25453,.T.) ;
#19671=FACE_OUTER_BOUND('',#25454,.T.) ;
#19672=FACE_OUTER_BOUND('',#25455,.T.) ;
#19673=FACE_OUTER_BOUND('',#25456,.T.) ;
#19674=FACE_OUTER_BOUND('',#25457,.T.) ;
#19675=FACE_OUTER_BOUND('',#25458,.T.) ;
#19676=FACE_OUTER_BOUND('',#25459,.T.) ;
#19677=FACE_OUTER_BOUND('',#25460,.T.) ;
#19678=FACE_OUTER_BOUND('',#25461,.T.) ;
#19679=FACE_OUTER_BOUND('',#25462,.T.) ;
#19680=FACE_OUTER_BOUND('',#25463,.T.) ;
#19681=FACE_OUTER_BOUND('',#25464,.T.) ;
#19682=FACE_OUTER_BOUND('',#25465,.T.) ;
#19683=FACE_OUTER_BOUND('',#25466,.T.) ;
#19684=FACE_OUTER_BOUND('',#25467,.T.) ;
#19685=FACE_OUTER_BOUND('',#25468,.T.) ;
#19686=FACE_OUTER_BOUND('',#25469,.T.) ;
#19687=FACE_OUTER_BOUND('',#25470,.T.) ;
#19688=FACE_OUTER_BOUND('',#25471,.T.) ;
#19689=FACE_OUTER_BOUND('',#25472,.T.) ;
#19690=FACE_OUTER_BOUND('',#25473,.T.) ;
#19691=FACE_OUTER_BOUND('',#25474,.T.) ;
#19692=FACE_OUTER_BOUND('',#25475,.T.) ;
#19693=FACE_OUTER_BOUND('',#25476,.T.) ;
#19694=FACE_OUTER_BOUND('',#25477,.T.) ;
#19695=FACE_OUTER_BOUND('',#25478,.T.) ;
#19696=FACE_OUTER_BOUND('',#25479,.T.) ;
#19697=FACE_OUTER_BOUND('',#25480,.T.) ;
#19698=FACE_OUTER_BOUND('',#25481,.T.) ;
#19699=FACE_OUTER_BOUND('',#25482,.T.) ;
#19700=FACE_OUTER_BOUND('',#25483,.T.) ;
#19701=FACE_OUTER_BOUND('',#25484,.T.) ;
#19702=FACE_OUTER_BOUND('',#25485,.T.) ;
#19703=FACE_OUTER_BOUND('',#25486,.T.) ;
#19704=FACE_OUTER_BOUND('',#25487,.T.) ;
#19705=FACE_OUTER_BOUND('',#25488,.T.) ;
#19706=FACE_OUTER_BOUND('',#25489,.T.) ;
#19707=FACE_OUTER_BOUND('',#25490,.T.) ;
#19708=FACE_OUTER_BOUND('',#25491,.T.) ;
#19709=FACE_OUTER_BOUND('',#25492,.T.) ;
#19710=FACE_OUTER_BOUND('',#25493,.T.) ;
#19711=FACE_OUTER_BOUND('',#25494,.T.) ;
#19712=FACE_OUTER_BOUND('',#25495,.T.) ;
#19713=FACE_OUTER_BOUND('',#25496,.T.) ;
#19714=FACE_OUTER_BOUND('',#25497,.T.) ;
#19715=FACE_OUTER_BOUND('',#25498,.T.) ;
#19716=FACE_OUTER_BOUND('',#25499,.T.) ;
#19717=FACE_OUTER_BOUND('',#25500,.T.) ;
#19718=FACE_OUTER_BOUND('',#25501,.T.) ;
#19719=FACE_OUTER_BOUND('',#25502,.T.) ;
#19720=FACE_OUTER_BOUND('',#25503,.T.) ;
#19721=FACE_OUTER_BOUND('',#25504,.T.) ;
#19722=FACE_OUTER_BOUND('',#25505,.T.) ;
#19723=FACE_OUTER_BOUND('',#25506,.T.) ;
#19724=FACE_OUTER_BOUND('',#25507,.T.) ;
#19725=FACE_OUTER_BOUND('',#25508,.T.) ;
#19726=FACE_OUTER_BOUND('',#25509,.T.) ;
#19727=FACE_OUTER_BOUND('',#25510,.T.) ;
#19728=FACE_OUTER_BOUND('',#25511,.T.) ;
#19729=FACE_OUTER_BOUND('',#25512,.T.) ;
#19730=FACE_OUTER_BOUND('',#25513,.T.) ;
#19731=FACE_OUTER_BOUND('',#25514,.T.) ;
#19732=FACE_OUTER_BOUND('',#25515,.T.) ;
#19733=FACE_OUTER_BOUND('',#25516,.T.) ;
#19734=FACE_OUTER_BOUND('',#25517,.T.) ;
#19735=FACE_OUTER_BOUND('',#25518,.T.) ;
#19736=FACE_OUTER_BOUND('',#25519,.T.) ;
#19737=FACE_OUTER_BOUND('',#25520,.T.) ;
#19738=FACE_OUTER_BOUND('',#25521,.T.) ;
#19739=FACE_OUTER_BOUND('',#25522,.T.) ;
#19740=FACE_OUTER_BOUND('',#25523,.T.) ;
#19741=FACE_OUTER_BOUND('',#25524,.T.) ;
#19742=FACE_OUTER_BOUND('',#25525,.T.) ;
#19743=FACE_OUTER_BOUND('',#25526,.T.) ;
#19744=FACE_OUTER_BOUND('',#25527,.T.) ;
#19745=FACE_OUTER_BOUND('',#25528,.T.) ;
#19746=FACE_OUTER_BOUND('',#25529,.T.) ;
#19747=FACE_OUTER_BOUND('',#25530,.T.) ;
#19748=FACE_OUTER_BOUND('',#25531,.T.) ;
#19749=FACE_OUTER_BOUND('',#25532,.T.) ;
#19750=FACE_OUTER_BOUND('',#25533,.T.) ;
#19751=FACE_OUTER_BOUND('',#25534,.T.) ;
#19752=FACE_OUTER_BOUND('',#25535,.T.) ;
#19753=FACE_OUTER_BOUND('',#25536,.T.) ;
#19754=FACE_OUTER_BOUND('',#25537,.T.) ;
#19755=FACE_OUTER_BOUND('',#25538,.T.) ;
#19756=FACE_OUTER_BOUND('',#25539,.T.) ;
#19757=FACE_OUTER_BOUND('',#25540,.T.) ;
#19758=FACE_OUTER_BOUND('',#25541,.T.) ;
#19759=FACE_OUTER_BOUND('',#25542,.T.) ;
#19760=FACE_OUTER_BOUND('',#25543,.T.) ;
#19761=FACE_OUTER_BOUND('',#25544,.T.) ;
#19762=FACE_OUTER_BOUND('',#25545,.T.) ;
#19763=FACE_OUTER_BOUND('',#25546,.T.) ;
#19764=FACE_OUTER_BOUND('',#25547,.T.) ;
#19765=FACE_OUTER_BOUND('',#25548,.T.) ;
#19766=FACE_OUTER_BOUND('',#25549,.T.) ;
#19767=FACE_OUTER_BOUND('',#25550,.T.) ;
#19768=FACE_OUTER_BOUND('',#25551,.T.) ;
#19769=FACE_OUTER_BOUND('',#25552,.T.) ;
#19770=FACE_OUTER_BOUND('',#25553,.T.) ;
#19771=FACE_OUTER_BOUND('',#25554,.T.) ;
#19772=FACE_OUTER_BOUND('',#25555,.T.) ;
#19773=FACE_OUTER_BOUND('',#25556,.T.) ;
#19774=FACE_OUTER_BOUND('',#25557,.T.) ;
#19775=FACE_OUTER_BOUND('',#25558,.T.) ;
#19776=FACE_OUTER_BOUND('',#25559,.T.) ;
#19777=FACE_OUTER_BOUND('',#25560,.T.) ;
#19778=FACE_OUTER_BOUND('',#25561,.T.) ;
#19779=FACE_OUTER_BOUND('',#25562,.T.) ;
#19780=FACE_OUTER_BOUND('',#25563,.T.) ;
#19781=FACE_OUTER_BOUND('',#25564,.T.) ;
#19782=FACE_OUTER_BOUND('',#25565,.T.) ;
#19783=FACE_OUTER_BOUND('',#25566,.T.) ;
#19784=FACE_OUTER_BOUND('',#25567,.T.) ;
#19785=FACE_OUTER_BOUND('',#25568,.T.) ;
#19786=FACE_OUTER_BOUND('',#25569,.T.) ;
#19787=FACE_OUTER_BOUND('',#25570,.T.) ;
#19788=FACE_OUTER_BOUND('',#25571,.T.) ;
#19789=FACE_OUTER_BOUND('',#25572,.T.) ;
#19790=FACE_OUTER_BOUND('',#25573,.T.) ;
#19791=FACE_OUTER_BOUND('',#25574,.T.) ;
#19792=FACE_OUTER_BOUND('',#25575,.T.) ;
#19793=FACE_OUTER_BOUND('',#25576,.T.) ;
#19794=FACE_OUTER_BOUND('',#25577,.T.) ;
#19795=FACE_OUTER_BOUND('',#25578,.T.) ;
#19796=FACE_OUTER_BOUND('',#25579,.T.) ;
#19797=FACE_OUTER_BOUND('',#25580,.T.) ;
#19798=FACE_OUTER_BOUND('',#25581,.T.) ;
#19799=FACE_OUTER_BOUND('',#25582,.T.) ;
#19800=FACE_OUTER_BOUND('',#25583,.T.) ;
#19801=FACE_OUTER_BOUND('',#25584,.T.) ;
#19802=FACE_OUTER_BOUND('',#25585,.T.) ;
#19803=FACE_OUTER_BOUND('',#25586,.T.) ;
#19804=FACE_OUTER_BOUND('',#25587,.T.) ;
#19805=FACE_OUTER_BOUND('',#25588,.T.) ;
#19806=FACE_OUTER_BOUND('',#25589,.T.) ;
#19807=FACE_OUTER_BOUND('',#25590,.T.) ;
#19808=FACE_OUTER_BOUND('',#25591,.T.) ;
#19809=FACE_OUTER_BOUND('',#25592,.T.) ;
#19810=FACE_OUTER_BOUND('',#25593,.T.) ;
#19811=FACE_OUTER_BOUND('',#25594,.T.) ;
#19812=FACE_OUTER_BOUND('',#25595,.T.) ;
#19813=FACE_OUTER_BOUND('',#25596,.T.) ;
#19814=FACE_OUTER_BOUND('',#25597,.T.) ;
#19815=FACE_OUTER_BOUND('',#25598,.T.) ;
#19816=FACE_OUTER_BOUND('',#25599,.T.) ;
#19817=FACE_OUTER_BOUND('',#25600,.T.) ;
#19818=FACE_OUTER_BOUND('',#25601,.T.) ;
#19819=FACE_OUTER_BOUND('',#25602,.T.) ;
#19820=FACE_OUTER_BOUND('',#25603,.T.) ;
#19821=FACE_OUTER_BOUND('',#25604,.T.) ;
#19822=FACE_OUTER_BOUND('',#25605,.T.) ;
#19823=FACE_OUTER_BOUND('',#25606,.T.) ;
#19824=FACE_OUTER_BOUND('',#25607,.T.) ;
#19825=FACE_OUTER_BOUND('',#25608,.T.) ;
#19826=FACE_OUTER_BOUND('',#25609,.T.) ;
#19827=FACE_OUTER_BOUND('',#25610,.T.) ;
#19828=FACE_OUTER_BOUND('',#25611,.T.) ;
#19829=FACE_OUTER_BOUND('',#25612,.T.) ;
#19830=FACE_OUTER_BOUND('',#25613,.T.) ;
#19831=FACE_OUTER_BOUND('',#25614,.T.) ;
#19832=FACE_OUTER_BOUND('',#25615,.T.) ;
#19833=FACE_OUTER_BOUND('',#25616,.T.) ;
#19834=FACE_OUTER_BOUND('',#25617,.T.) ;
#19835=FACE_OUTER_BOUND('',#25618,.T.) ;
#19836=FACE_OUTER_BOUND('',#25619,.T.) ;
#19837=FACE_OUTER_BOUND('',#25620,.T.) ;
#19838=FACE_OUTER_BOUND('',#25621,.T.) ;
#19839=FACE_OUTER_BOUND('',#25622,.T.) ;
#19840=FACE_OUTER_BOUND('',#25623,.T.) ;
#19841=FACE_OUTER_BOUND('',#25624,.T.) ;
#19842=FACE_OUTER_BOUND('',#25625,.T.) ;
#19843=FACE_OUTER_BOUND('',#25626,.T.) ;
#19844=FACE_OUTER_BOUND('',#25627,.T.) ;
#19845=FACE_OUTER_BOUND('',#25628,.T.) ;
#19846=FACE_OUTER_BOUND('',#25629,.T.) ;
#19847=FACE_OUTER_BOUND('',#25630,.T.) ;
#19848=FACE_OUTER_BOUND('',#25631,.T.) ;
#19849=FACE_OUTER_BOUND('',#25632,.T.) ;
#19850=FACE_OUTER_BOUND('',#25633,.T.) ;
#19851=FACE_OUTER_BOUND('',#25634,.T.) ;
#19852=FACE_OUTER_BOUND('',#25635,.T.) ;
#19853=FACE_OUTER_BOUND('',#25636,.T.) ;
#19854=FACE_OUTER_BOUND('',#25637,.T.) ;
#19855=FACE_OUTER_BOUND('',#25638,.T.) ;
#19856=FACE_OUTER_BOUND('',#25639,.T.) ;
#19857=FACE_OUTER_BOUND('',#25640,.T.) ;
#19858=FACE_OUTER_BOUND('',#25641,.T.) ;
#19859=FACE_OUTER_BOUND('',#25642,.T.) ;
#19860=FACE_OUTER_BOUND('',#25643,.T.) ;
#19861=FACE_OUTER_BOUND('',#25644,.T.) ;
#19862=FACE_OUTER_BOUND('',#25645,.T.) ;
#19863=FACE_OUTER_BOUND('',#25646,.T.) ;
#19864=FACE_OUTER_BOUND('',#25647,.T.) ;
#19865=FACE_OUTER_BOUND('',#25648,.T.) ;
#19866=FACE_OUTER_BOUND('',#25649,.T.) ;
#19867=FACE_OUTER_BOUND('',#25650,.T.) ;
#19868=FACE_OUTER_BOUND('',#25651,.T.) ;
#19869=FACE_OUTER_BOUND('',#25652,.T.) ;
#19870=FACE_OUTER_BOUND('',#25653,.T.) ;
#19871=FACE_OUTER_BOUND('',#25654,.T.) ;
#19872=FACE_OUTER_BOUND('',#25655,.T.) ;
#19873=FACE_OUTER_BOUND('',#25656,.T.) ;
#19874=FACE_OUTER_BOUND('',#25657,.T.) ;
#19875=FACE_OUTER_BOUND('',#25658,.T.) ;
#19876=FACE_OUTER_BOUND('',#25659,.T.) ;
#19877=FACE_OUTER_BOUND('',#25660,.T.) ;
#19878=FACE_OUTER_BOUND('',#25661,.T.) ;
#19879=FACE_OUTER_BOUND('',#25662,.T.) ;
#19880=FACE_OUTER_BOUND('',#25663,.T.) ;
#19881=FACE_OUTER_BOUND('',#25664,.T.) ;
#19882=FACE_OUTER_BOUND('',#25665,.T.) ;
#19883=FACE_OUTER_BOUND('',#25666,.T.) ;
#19884=FACE_OUTER_BOUND('',#25667,.T.) ;
#19885=FACE_OUTER_BOUND('',#25668,.T.) ;
#19886=FACE_OUTER_BOUND('',#25669,.T.) ;
#19887=FACE_OUTER_BOUND('',#25670,.T.) ;
#19888=FACE_OUTER_BOUND('',#25671,.T.) ;
#19889=FACE_OUTER_BOUND('',#25672,.T.) ;
#19890=FACE_OUTER_BOUND('',#25673,.T.) ;
#19891=FACE_OUTER_BOUND('',#25674,.T.) ;
#19892=FACE_OUTER_BOUND('',#25675,.T.) ;
#19893=FACE_OUTER_BOUND('',#25676,.T.) ;
#19894=FACE_OUTER_BOUND('',#25677,.T.) ;
#19895=FACE_OUTER_BOUND('',#25678,.T.) ;
#19896=FACE_OUTER_BOUND('',#25679,.T.) ;
#19897=FACE_OUTER_BOUND('',#25680,.T.) ;
#19898=FACE_OUTER_BOUND('',#25681,.T.) ;
#19899=FACE_OUTER_BOUND('',#25682,.T.) ;
#19900=FACE_OUTER_BOUND('',#25683,.T.) ;
#19901=FACE_OUTER_BOUND('',#25684,.T.) ;
#19902=FACE_OUTER_BOUND('',#25685,.T.) ;
#19903=FACE_OUTER_BOUND('',#25686,.T.) ;
#19904=FACE_OUTER_BOUND('',#25687,.T.) ;
#19905=FACE_OUTER_BOUND('',#25688,.T.) ;
#19906=FACE_OUTER_BOUND('',#25689,.T.) ;
#19907=FACE_OUTER_BOUND('',#25690,.T.) ;
#19908=FACE_OUTER_BOUND('',#25691,.T.) ;
#19909=FACE_OUTER_BOUND('',#25692,.T.) ;
#19910=FACE_OUTER_BOUND('',#25693,.T.) ;
#19911=FACE_OUTER_BOUND('',#25694,.T.) ;
#19912=FACE_OUTER_BOUND('',#25695,.T.) ;
#19913=FACE_OUTER_BOUND('',#25696,.T.) ;
#19914=FACE_OUTER_BOUND('',#25697,.T.) ;
#19915=FACE_OUTER_BOUND('',#25698,.T.) ;
#19916=FACE_OUTER_BOUND('',#25699,.T.) ;
#19917=FACE_OUTER_BOUND('',#25700,.T.) ;
#19918=FACE_OUTER_BOUND('',#25701,.T.) ;
#19919=FACE_OUTER_BOUND('',#25702,.T.) ;
#19920=FACE_OUTER_BOUND('',#25703,.T.) ;
#19921=FACE_OUTER_BOUND('',#25704,.T.) ;
#19922=FACE_OUTER_BOUND('',#25705,.T.) ;
#19923=FACE_OUTER_BOUND('',#25706,.T.) ;
#19924=FACE_OUTER_BOUND('',#25707,.T.) ;
#19925=FACE_OUTER_BOUND('',#25708,.T.) ;
#19926=FACE_OUTER_BOUND('',#25709,.T.) ;
#19927=FACE_OUTER_BOUND('',#25710,.T.) ;
#19928=FACE_OUTER_BOUND('',#25711,.T.) ;
#19929=FACE_OUTER_BOUND('',#25712,.T.) ;
#19930=FACE_OUTER_BOUND('',#25713,.T.) ;
#19931=FACE_OUTER_BOUND('',#25714,.T.) ;
#19932=FACE_OUTER_BOUND('',#25715,.T.) ;
#19933=FACE_OUTER_BOUND('',#25716,.T.) ;
#19934=FACE_OUTER_BOUND('',#25717,.T.) ;
#19935=FACE_OUTER_BOUND('',#25718,.T.) ;
#19936=FACE_OUTER_BOUND('',#25719,.T.) ;
#19937=FACE_OUTER_BOUND('',#25720,.T.) ;
#19938=FACE_OUTER_BOUND('',#25721,.T.) ;
#19939=FACE_OUTER_BOUND('',#25722,.T.) ;
#19940=FACE_OUTER_BOUND('',#25723,.T.) ;
#19941=FACE_OUTER_BOUND('',#25724,.T.) ;
#19942=FACE_OUTER_BOUND('',#25725,.T.) ;
#19943=FACE_OUTER_BOUND('',#25726,.T.) ;
#19944=FACE_OUTER_BOUND('',#25727,.T.) ;
#19945=FACE_OUTER_BOUND('',#25728,.T.) ;
#19946=FACE_OUTER_BOUND('',#25729,.T.) ;
#19947=FACE_OUTER_BOUND('',#25730,.T.) ;
#19948=FACE_OUTER_BOUND('',#25731,.T.) ;
#19949=FACE_OUTER_BOUND('',#25732,.T.) ;
#19950=FACE_OUTER_BOUND('',#25733,.T.) ;
#19951=FACE_OUTER_BOUND('',#25734,.T.) ;
#19952=FACE_OUTER_BOUND('',#25735,.T.) ;
#19953=FACE_OUTER_BOUND('',#25736,.T.) ;
#19954=FACE_OUTER_BOUND('',#25737,.T.) ;
#19955=FACE_OUTER_BOUND('',#25738,.T.) ;
#19956=FACE_OUTER_BOUND('',#25739,.T.) ;
#19957=FACE_OUTER_BOUND('',#25740,.T.) ;
#19958=FACE_OUTER_BOUND('',#25741,.T.) ;
#19959=FACE_OUTER_BOUND('',#25742,.T.) ;
#19960=FACE_OUTER_BOUND('',#25743,.T.) ;
#19961=FACE_OUTER_BOUND('',#25744,.T.) ;
#19962=FACE_OUTER_BOUND('',#25745,.T.) ;
#19963=FACE_OUTER_BOUND('',#25746,.T.) ;
#19964=FACE_OUTER_BOUND('',#25747,.T.) ;
#19965=FACE_OUTER_BOUND('',#25748,.T.) ;
#19966=FACE_OUTER_BOUND('',#25749,.T.) ;
#19967=FACE_OUTER_BOUND('',#25750,.T.) ;
#19968=FACE_OUTER_BOUND('',#25751,.T.) ;
#19969=FACE_OUTER_BOUND('',#25752,.T.) ;
#19970=FACE_OUTER_BOUND('',#25753,.T.) ;
#19971=FACE_OUTER_BOUND('',#25754,.T.) ;
#19972=FACE_OUTER_BOUND('',#25755,.T.) ;
#19973=FACE_OUTER_BOUND('',#25756,.T.) ;
#19974=FACE_OUTER_BOUND('',#25757,.T.) ;
#19975=FACE_OUTER_BOUND('',#25758,.T.) ;
#19976=FACE_OUTER_BOUND('',#25759,.T.) ;
#19977=FACE_OUTER_BOUND('',#25760,.T.) ;
#19978=FACE_OUTER_BOUND('',#25761,.T.) ;
#19979=FACE_OUTER_BOUND('',#25762,.T.) ;
#19980=FACE_OUTER_BOUND('',#25763,.T.) ;
#19981=FACE_OUTER_BOUND('',#25764,.T.) ;
#19982=FACE_OUTER_BOUND('',#25765,.T.) ;
#19983=FACE_OUTER_BOUND('',#25766,.T.) ;
#19984=FACE_OUTER_BOUND('',#25767,.T.) ;
#19985=FACE_OUTER_BOUND('',#25768,.T.) ;
#19986=FACE_OUTER_BOUND('',#25769,.T.) ;
#19987=FACE_OUTER_BOUND('',#25770,.T.) ;
#19988=FACE_OUTER_BOUND('',#25771,.T.) ;
#19989=FACE_OUTER_BOUND('',#25772,.T.) ;
#19990=FACE_OUTER_BOUND('',#25773,.T.) ;
#19991=FACE_OUTER_BOUND('',#25774,.T.) ;
#19992=FACE_OUTER_BOUND('',#25775,.T.) ;
#19993=FACE_OUTER_BOUND('',#25776,.T.) ;
#19994=FACE_OUTER_BOUND('',#25777,.T.) ;
#19995=FACE_OUTER_BOUND('',#25778,.T.) ;
#19996=FACE_OUTER_BOUND('',#25779,.T.) ;
#19997=FACE_OUTER_BOUND('',#25780,.T.) ;
#19998=FACE_OUTER_BOUND('',#25781,.T.) ;
#19999=FACE_OUTER_BOUND('',#25782,.T.) ;
#20000=FACE_OUTER_BOUND('',#25783,.T.) ;
#20001=FACE_OUTER_BOUND('',#25784,.T.) ;
#20002=FACE_OUTER_BOUND('',#25785,.T.) ;
#20003=FACE_OUTER_BOUND('',#25786,.T.) ;
#20004=FACE_OUTER_BOUND('',#25787,.T.) ;
#20005=FACE_OUTER_BOUND('',#25788,.T.) ;
#20006=FACE_OUTER_BOUND('',#25789,.T.) ;
#20007=FACE_OUTER_BOUND('',#25790,.T.) ;
#20008=FACE_OUTER_BOUND('',#25791,.T.) ;
#20009=FACE_OUTER_BOUND('',#25792,.T.) ;
#20010=FACE_OUTER_BOUND('',#25793,.T.) ;
#20011=FACE_OUTER_BOUND('',#25794,.T.) ;
#20012=FACE_OUTER_BOUND('',#25795,.T.) ;
#20013=FACE_OUTER_BOUND('',#25796,.T.) ;
#20014=FACE_OUTER_BOUND('',#25797,.T.) ;
#20015=FACE_OUTER_BOUND('',#25798,.T.) ;
#20016=FACE_OUTER_BOUND('',#25799,.T.) ;
#20017=FACE_OUTER_BOUND('',#25800,.T.) ;
#20018=FACE_OUTER_BOUND('',#25801,.T.) ;
#20019=FACE_OUTER_BOUND('',#25802,.T.) ;
#20020=FACE_OUTER_BOUND('',#25803,.T.) ;
#20021=FACE_OUTER_BOUND('',#25804,.T.) ;
#20022=FACE_OUTER_BOUND('',#25805,.T.) ;
#20023=FACE_OUTER_BOUND('',#25806,.T.) ;
#20024=FACE_OUTER_BOUND('',#25807,.T.) ;
#20025=FACE_OUTER_BOUND('',#25808,.T.) ;
#20026=FACE_OUTER_BOUND('',#25809,.T.) ;
#20027=FACE_OUTER_BOUND('',#25810,.T.) ;
#20028=FACE_OUTER_BOUND('',#25811,.T.) ;
#20029=FACE_OUTER_BOUND('',#25812,.T.) ;
#20030=FACE_OUTER_BOUND('',#25813,.T.) ;
#20031=FACE_OUTER_BOUND('',#25814,.T.) ;
#20032=FACE_OUTER_BOUND('',#25815,.T.) ;
#20033=FACE_OUTER_BOUND('',#25816,.T.) ;
#20034=FACE_OUTER_BOUND('',#25817,.T.) ;
#20035=FACE_OUTER_BOUND('',#25818,.T.) ;
#20036=FACE_OUTER_BOUND('',#25819,.T.) ;
#20037=FACE_OUTER_BOUND('',#25820,.T.) ;
#20038=FACE_OUTER_BOUND('',#25821,.T.) ;
#20039=FACE_OUTER_BOUND('',#25822,.T.) ;
#20040=FACE_OUTER_BOUND('',#25823,.T.) ;
#20041=FACE_OUTER_BOUND('',#25824,.T.) ;
#20042=FACE_OUTER_BOUND('',#25825,.T.) ;
#20043=FACE_OUTER_BOUND('',#25826,.T.) ;
#20044=FACE_OUTER_BOUND('',#25827,.T.) ;
#20045=FACE_OUTER_BOUND('',#25828,.T.) ;
#20046=FACE_OUTER_BOUND('',#25829,.T.) ;
#20047=FACE_OUTER_BOUND('',#25830,.T.) ;
#20048=FACE_OUTER_BOUND('',#25831,.T.) ;
#20049=FACE_OUTER_BOUND('',#25832,.T.) ;
#20050=FACE_OUTER_BOUND('',#25833,.T.) ;
#20051=FACE_OUTER_BOUND('',#25834,.T.) ;
#20052=FACE_OUTER_BOUND('',#25835,.T.) ;
#20053=FACE_OUTER_BOUND('',#25836,.T.) ;
#20054=FACE_OUTER_BOUND('',#25837,.T.) ;
#20055=FACE_OUTER_BOUND('',#25838,.T.) ;
#20056=FACE_OUTER_BOUND('',#25839,.T.) ;
#20057=FACE_OUTER_BOUND('',#25840,.T.) ;
#20058=FACE_OUTER_BOUND('',#25841,.T.) ;
#20059=FACE_OUTER_BOUND('',#25842,.T.) ;
#20060=FACE_OUTER_BOUND('',#25843,.T.) ;
#20061=FACE_OUTER_BOUND('',#25844,.T.) ;
#20062=FACE_OUTER_BOUND('',#25845,.T.) ;
#20063=FACE_OUTER_BOUND('',#25846,.T.) ;
#20064=FACE_OUTER_BOUND('',#25847,.T.) ;
#20065=FACE_OUTER_BOUND('',#25848,.T.) ;
#20066=FACE_OUTER_BOUND('',#25849,.T.) ;
#20067=FACE_OUTER_BOUND('',#25850,.T.) ;
#20068=FACE_OUTER_BOUND('',#25851,.T.) ;
#20069=FACE_OUTER_BOUND('',#25852,.T.) ;
#20070=FACE_OUTER_BOUND('',#25853,.T.) ;
#20071=FACE_OUTER_BOUND('',#25854,.T.) ;
#20072=FACE_OUTER_BOUND('',#25855,.T.) ;
#20073=FACE_OUTER_BOUND('',#25856,.T.) ;
#20074=FACE_OUTER_BOUND('',#25857,.T.) ;
#20075=FACE_OUTER_BOUND('',#25858,.T.) ;
#20076=FACE_OUTER_BOUND('',#25859,.T.) ;
#20077=FACE_OUTER_BOUND('',#25860,.T.) ;
#20078=FACE_OUTER_BOUND('',#25861,.T.) ;
#20079=FACE_OUTER_BOUND('',#25862,.T.) ;
#20080=FACE_OUTER_BOUND('',#25863,.T.) ;
#20081=FACE_OUTER_BOUND('',#25864,.T.) ;
#20082=FACE_OUTER_BOUND('',#25865,.T.) ;
#20083=FACE_OUTER_BOUND('',#25866,.T.) ;
#20084=FACE_OUTER_BOUND('',#25867,.T.) ;
#20085=FACE_OUTER_BOUND('',#25868,.T.) ;
#20086=FACE_OUTER_BOUND('',#25869,.T.) ;
#20087=FACE_OUTER_BOUND('',#25870,.T.) ;
#20088=FACE_OUTER_BOUND('',#25871,.T.) ;
#20089=FACE_OUTER_BOUND('',#25872,.T.) ;
#20090=FACE_OUTER_BOUND('',#25873,.T.) ;
#20091=FACE_OUTER_BOUND('',#25874,.T.) ;
#20092=FACE_OUTER_BOUND('',#25875,.T.) ;
#20093=FACE_OUTER_BOUND('',#25876,.T.) ;
#20094=FACE_OUTER_BOUND('',#25877,.T.) ;
#20095=FACE_OUTER_BOUND('',#25878,.T.) ;
#20096=FACE_OUTER_BOUND('',#25879,.T.) ;
#20097=FACE_OUTER_BOUND('',#25880,.T.) ;
#20098=FACE_OUTER_BOUND('',#25881,.T.) ;
#20099=FACE_OUTER_BOUND('',#25882,.T.) ;
#20100=FACE_OUTER_BOUND('',#25883,.T.) ;
#20101=FACE_OUTER_BOUND('',#25884,.T.) ;
#20102=FACE_OUTER_BOUND('',#25885,.T.) ;
#20103=FACE_OUTER_BOUND('',#25886,.T.) ;
#20104=FACE_OUTER_BOUND('',#25887,.T.) ;
#20105=FACE_OUTER_BOUND('',#25888,.T.) ;
#20106=FACE_OUTER_BOUND('',#25889,.T.) ;
#20107=FACE_OUTER_BOUND('',#25890,.T.) ;
#20108=FACE_OUTER_BOUND('',#25891,.T.) ;
#20109=FACE_OUTER_BOUND('',#25892,.T.) ;
#20110=FACE_OUTER_BOUND('',#25893,.T.) ;
#20111=FACE_OUTER_BOUND('',#25894,.T.) ;
#20112=FACE_OUTER_BOUND('',#25895,.T.) ;
#20113=FACE_OUTER_BOUND('',#25896,.T.) ;
#20114=FACE_OUTER_BOUND('',#25897,.T.) ;
#20115=FACE_OUTER_BOUND('',#25898,.T.) ;
#20116=FACE_OUTER_BOUND('',#25899,.T.) ;
#20117=FACE_OUTER_BOUND('',#25900,.T.) ;
#20118=FACE_OUTER_BOUND('',#25901,.T.) ;
#20119=FACE_OUTER_BOUND('',#25902,.T.) ;
#20120=FACE_OUTER_BOUND('',#25903,.T.) ;
#20121=FACE_OUTER_BOUND('',#25904,.T.) ;
#20122=FACE_OUTER_BOUND('',#25905,.T.) ;
#20123=FACE_OUTER_BOUND('',#25906,.T.) ;
#20124=FACE_OUTER_BOUND('',#25907,.T.) ;
#20125=FACE_OUTER_BOUND('',#25908,.T.) ;
#20126=FACE_OUTER_BOUND('',#25909,.T.) ;
#20127=FACE_OUTER_BOUND('',#25910,.T.) ;
#20128=FACE_OUTER_BOUND('',#25911,.T.) ;
#20129=FACE_OUTER_BOUND('',#25912,.T.) ;
#20130=FACE_OUTER_BOUND('',#25913,.T.) ;
#20131=FACE_OUTER_BOUND('',#25914,.T.) ;
#20132=FACE_OUTER_BOUND('',#25915,.T.) ;
#20133=FACE_OUTER_BOUND('',#25916,.T.) ;
#20134=FACE_OUTER_BOUND('',#25917,.T.) ;
#20135=FACE_OUTER_BOUND('',#25918,.T.) ;
#20136=FACE_OUTER_BOUND('',#25919,.T.) ;
#20137=FACE_OUTER_BOUND('',#25920,.T.) ;
#20138=FACE_OUTER_BOUND('',#25921,.T.) ;
#20139=FACE_OUTER_BOUND('',#25922,.T.) ;
#20140=FACE_OUTER_BOUND('',#25923,.T.) ;
#20141=FACE_OUTER_BOUND('',#25924,.T.) ;
#20142=FACE_OUTER_BOUND('',#25925,.T.) ;
#20143=FACE_OUTER_BOUND('',#25926,.T.) ;
#20144=FACE_OUTER_BOUND('',#25927,.T.) ;
#20145=FACE_OUTER_BOUND('',#25928,.T.) ;
#20146=FACE_OUTER_BOUND('',#25929,.T.) ;
#20147=FACE_OUTER_BOUND('',#25930,.T.) ;
#20148=FACE_OUTER_BOUND('',#25931,.T.) ;
#20149=FACE_OUTER_BOUND('',#25932,.T.) ;
#20150=FACE_OUTER_BOUND('',#25933,.T.) ;
#20151=FACE_OUTER_BOUND('',#25934,.T.) ;
#20152=FACE_OUTER_BOUND('',#25935,.T.) ;
#20153=FACE_OUTER_BOUND('',#25936,.T.) ;
#20154=FACE_OUTER_BOUND('',#25937,.T.) ;
#20155=FACE_OUTER_BOUND('',#25938,.T.) ;
#20156=FACE_OUTER_BOUND('',#25939,.T.) ;
#20157=FACE_OUTER_BOUND('',#25940,.T.) ;
#20158=FACE_OUTER_BOUND('',#25941,.T.) ;
#20159=FACE_OUTER_BOUND('',#25942,.T.) ;
#20160=FACE_OUTER_BOUND('',#25943,.T.) ;
#20161=FACE_OUTER_BOUND('',#25944,.T.) ;
#20162=FACE_OUTER_BOUND('',#25945,.T.) ;
#20163=FACE_OUTER_BOUND('',#25946,.T.) ;
#20164=FACE_OUTER_BOUND('',#25947,.T.) ;
#20165=FACE_OUTER_BOUND('',#25948,.T.) ;
#20166=FACE_OUTER_BOUND('',#25949,.T.) ;
#20167=FACE_OUTER_BOUND('',#25950,.T.) ;
#20168=FACE_OUTER_BOUND('',#25951,.T.) ;
#20169=FACE_OUTER_BOUND('',#25952,.T.) ;
#20170=FACE_OUTER_BOUND('',#25953,.T.) ;
#20171=FACE_OUTER_BOUND('',#25954,.T.) ;
#20172=FACE_OUTER_BOUND('',#25955,.T.) ;
#20173=FACE_OUTER_BOUND('',#25956,.T.) ;
#20174=FACE_OUTER_BOUND('',#25957,.T.) ;
#20175=FACE_OUTER_BOUND('',#25958,.T.) ;
#20176=FACE_OUTER_BOUND('',#25959,.T.) ;
#20177=FACE_OUTER_BOUND('',#25960,.T.) ;
#20178=FACE_OUTER_BOUND('',#25961,.T.) ;
#20179=FACE_OUTER_BOUND('',#25962,.T.) ;
#20180=FACE_OUTER_BOUND('',#25963,.T.) ;
#20181=FACE_OUTER_BOUND('',#25964,.T.) ;
#20182=FACE_OUTER_BOUND('',#25965,.T.) ;
#20183=FACE_OUTER_BOUND('',#25966,.T.) ;
#20184=FACE_OUTER_BOUND('',#25967,.T.) ;
#20185=FACE_OUTER_BOUND('',#25968,.T.) ;
#20186=FACE_OUTER_BOUND('',#25969,.T.) ;
#20187=FACE_OUTER_BOUND('',#25970,.T.) ;
#20188=FACE_OUTER_BOUND('',#25971,.T.) ;
#20189=FACE_OUTER_BOUND('',#25972,.T.) ;
#20190=FACE_OUTER_BOUND('',#25973,.T.) ;
#20191=FACE_OUTER_BOUND('',#25974,.T.) ;
#20192=FACE_OUTER_BOUND('',#25975,.T.) ;
#20193=FACE_OUTER_BOUND('',#25976,.T.) ;
#20194=FACE_OUTER_BOUND('',#25977,.T.) ;
#20195=FACE_OUTER_BOUND('',#25978,.T.) ;
#20196=FACE_OUTER_BOUND('',#25979,.T.) ;
#20197=FACE_OUTER_BOUND('',#25980,.T.) ;
#20198=FACE_OUTER_BOUND('',#25981,.T.) ;
#20199=FACE_OUTER_BOUND('',#25982,.T.) ;
#20200=FACE_OUTER_BOUND('',#25983,.T.) ;
#20201=FACE_OUTER_BOUND('',#25984,.T.) ;
#20202=FACE_OUTER_BOUND('',#25985,.T.) ;
#20203=FACE_OUTER_BOUND('',#25986,.T.) ;
#20204=FACE_OUTER_BOUND('',#25987,.T.) ;
#20205=FACE_OUTER_BOUND('',#25988,.T.) ;
#20206=FACE_OUTER_BOUND('',#25989,.T.) ;
#20207=FACE_OUTER_BOUND('',#25990,.T.) ;
#20208=FACE_OUTER_BOUND('',#25991,.T.) ;
#20209=FACE_OUTER_BOUND('',#25992,.T.) ;
#20210=FACE_OUTER_BOUND('',#25993,.T.) ;
#20211=FACE_OUTER_BOUND('',#25994,.T.) ;
#20212=FACE_OUTER_BOUND('',#25995,.T.) ;
#20213=FACE_OUTER_BOUND('',#25996,.T.) ;
#20214=FACE_OUTER_BOUND('',#25997,.T.) ;
#20215=FACE_OUTER_BOUND('',#25998,.T.) ;
#20216=FACE_OUTER_BOUND('',#25999,.T.) ;
#20217=FACE_OUTER_BOUND('',#26000,.T.) ;
#20218=FACE_OUTER_BOUND('',#26001,.T.) ;
#20219=FACE_OUTER_BOUND('',#26002,.T.) ;
#20220=FACE_OUTER_BOUND('',#26003,.T.) ;
#20221=FACE_OUTER_BOUND('',#26004,.T.) ;
#20222=FACE_OUTER_BOUND('',#26005,.T.) ;
#20223=FACE_OUTER_BOUND('',#26006,.T.) ;
#20224=FACE_OUTER_BOUND('',#26007,.T.) ;
#20225=FACE_OUTER_BOUND('',#26008,.T.) ;
#20226=FACE_OUTER_BOUND('',#26009,.T.) ;
#20227=FACE_OUTER_BOUND('',#26010,.T.) ;
#20228=FACE_OUTER_BOUND('',#26011,.T.) ;
#20229=FACE_OUTER_BOUND('',#26012,.T.) ;
#20230=FACE_OUTER_BOUND('',#26013,.T.) ;
#20231=FACE_OUTER_BOUND('',#26014,.T.) ;
#20232=FACE_OUTER_BOUND('',#26015,.T.) ;
#20233=FACE_OUTER_BOUND('',#26016,.T.) ;
#20234=FACE_OUTER_BOUND('',#26017,.T.) ;
#20235=FACE_OUTER_BOUND('',#26018,.T.) ;
#20236=FACE_OUTER_BOUND('',#26019,.T.) ;
#20237=FACE_OUTER_BOUND('',#26020,.T.) ;
#20238=FACE_OUTER_BOUND('',#26021,.T.) ;
#20239=FACE_OUTER_BOUND('',#26022,.T.) ;
#20240=FACE_OUTER_BOUND('',#26023,.T.) ;
#20241=FACE_OUTER_BOUND('',#26024,.T.) ;
#20242=FACE_OUTER_BOUND('',#26025,.T.) ;
#20243=FACE_OUTER_BOUND('',#26026,.T.) ;
#20244=FACE_OUTER_BOUND('',#26027,.T.) ;
#20245=FACE_OUTER_BOUND('',#26028,.T.) ;
#20246=FACE_OUTER_BOUND('',#26029,.T.) ;
#20247=FACE_OUTER_BOUND('',#26030,.T.) ;
#20248=FACE_OUTER_BOUND('',#26031,.T.) ;
#20249=FACE_OUTER_BOUND('',#26032,.T.) ;
#20250=FACE_OUTER_BOUND('',#26033,.T.) ;
#20251=FACE_OUTER_BOUND('',#26034,.T.) ;
#20252=FACE_OUTER_BOUND('',#26035,.T.) ;
#20253=FACE_OUTER_BOUND('',#26036,.T.) ;
#20254=FACE_OUTER_BOUND('',#26037,.T.) ;
#20255=FACE_OUTER_BOUND('',#26038,.T.) ;
#20256=FACE_OUTER_BOUND('',#26039,.T.) ;
#20257=FACE_OUTER_BOUND('',#26040,.T.) ;
#20258=FACE_OUTER_BOUND('',#26041,.T.) ;
#20259=FACE_OUTER_BOUND('',#26042,.T.) ;
#20260=FACE_OUTER_BOUND('',#26043,.T.) ;
#20261=FACE_OUTER_BOUND('',#26044,.T.) ;
#20262=FACE_OUTER_BOUND('',#26045,.T.) ;
#20263=FACE_OUTER_BOUND('',#26046,.T.) ;
#20264=FACE_OUTER_BOUND('',#26047,.T.) ;
#20265=FACE_OUTER_BOUND('',#26048,.T.) ;
#20266=FACE_OUTER_BOUND('',#26049,.T.) ;
#20267=FACE_OUTER_BOUND('',#26050,.T.) ;
#20268=FACE_OUTER_BOUND('',#26051,.T.) ;
#20269=FACE_OUTER_BOUND('',#26052,.T.) ;
#20270=FACE_OUTER_BOUND('',#26053,.T.) ;
#20271=FACE_OUTER_BOUND('',#26054,.T.) ;
#20272=FACE_OUTER_BOUND('',#26055,.T.) ;
#20273=FACE_OUTER_BOUND('',#26056,.T.) ;
#20274=FACE_OUTER_BOUND('',#26057,.T.) ;
#20275=FACE_OUTER_BOUND('',#26058,.T.) ;
#20276=FACE_OUTER_BOUND('',#26059,.T.) ;
#20277=FACE_OUTER_BOUND('',#26060,.T.) ;
#20278=FACE_OUTER_BOUND('',#26061,.T.) ;
#20279=FACE_OUTER_BOUND('',#26062,.T.) ;
#20280=FACE_OUTER_BOUND('',#26063,.T.) ;
#20281=FACE_OUTER_BOUND('',#26064,.T.) ;
#20282=FACE_OUTER_BOUND('',#26065,.T.) ;
#20283=FACE_OUTER_BOUND('',#26066,.T.) ;
#20284=FACE_OUTER_BOUND('',#26067,.T.) ;
#20285=FACE_OUTER_BOUND('',#26068,.T.) ;
#20286=FACE_OUTER_BOUND('',#26069,.T.) ;
#20287=FACE_OUTER_BOUND('',#26070,.T.) ;
#20288=FACE_OUTER_BOUND('',#26071,.T.) ;
#20289=FACE_OUTER_BOUND('',#26072,.T.) ;
#20290=FACE_OUTER_BOUND('',#26073,.T.) ;
#20291=FACE_OUTER_BOUND('',#26074,.T.) ;
#20292=FACE_OUTER_BOUND('',#26075,.T.) ;
#20293=FACE_OUTER_BOUND('',#26076,.T.) ;
#20294=FACE_OUTER_BOUND('',#26077,.T.) ;
#20295=FACE_OUTER_BOUND('',#26078,.T.) ;
#20296=FACE_OUTER_BOUND('',#26079,.T.) ;
#20297=FACE_OUTER_BOUND('',#26080,.T.) ;
#20298=FACE_OUTER_BOUND('',#26081,.T.) ;
#20299=FACE_OUTER_BOUND('',#26082,.T.) ;
#20300=FACE_OUTER_BOUND('',#26083,.T.) ;
#20301=FACE_OUTER_BOUND('',#26084,.T.) ;
#20302=FACE_OUTER_BOUND('',#26085,.T.) ;
#20303=FACE_OUTER_BOUND('',#26086,.T.) ;
#20304=FACE_OUTER_BOUND('',#26087,.T.) ;
#20305=FACE_OUTER_BOUND('',#26088,.T.) ;
#20306=FACE_OUTER_BOUND('',#26089,.T.) ;
#20307=FACE_OUTER_BOUND('',#26090,.T.) ;
#20308=FACE_OUTER_BOUND('',#26091,.T.) ;
#20309=FACE_OUTER_BOUND('',#26092,.T.) ;
#20310=FACE_OUTER_BOUND('',#26093,.T.) ;
#20311=FACE_OUTER_BOUND('',#26094,.T.) ;
#20312=FACE_OUTER_BOUND('',#26095,.T.) ;
#20313=FACE_OUTER_BOUND('',#26096,.T.) ;
#20314=FACE_OUTER_BOUND('',#26097,.T.) ;
#20315=FACE_OUTER_BOUND('',#26098,.T.) ;
#20316=FACE_OUTER_BOUND('',#26099,.T.) ;
#20317=FACE_OUTER_BOUND('',#26100,.T.) ;
#20318=FACE_OUTER_BOUND('',#26101,.T.) ;
#20319=FACE_OUTER_BOUND('',#26102,.T.) ;
#20320=FACE_OUTER_BOUND('',#26103,.T.) ;
#20321=FACE_OUTER_BOUND('',#26104,.T.) ;
#20322=FACE_OUTER_BOUND('',#26105,.T.) ;
#20323=FACE_OUTER_BOUND('',#26106,.T.) ;
#20324=FACE_OUTER_BOUND('',#26107,.T.) ;
#20325=FACE_OUTER_BOUND('',#26108,.T.) ;
#20326=FACE_OUTER_BOUND('',#26109,.T.) ;
#20327=FACE_OUTER_BOUND('',#26110,.T.) ;
#20328=FACE_OUTER_BOUND('',#26111,.T.) ;
#20329=FACE_OUTER_BOUND('',#26112,.T.) ;
#20330=FACE_OUTER_BOUND('',#26113,.T.) ;
#20331=FACE_OUTER_BOUND('',#26114,.T.) ;
#20332=FACE_OUTER_BOUND('',#26115,.T.) ;
#20333=FACE_OUTER_BOUND('',#26116,.T.) ;
#20334=FACE_OUTER_BOUND('',#26117,.T.) ;
#20335=FACE_OUTER_BOUND('',#26118,.T.) ;
#20336=FACE_OUTER_BOUND('',#26119,.T.) ;
#20337=FACE_OUTER_BOUND('',#26120,.T.) ;
#20338=FACE_OUTER_BOUND('',#26121,.T.) ;
#20339=FACE_OUTER_BOUND('',#26122,.T.) ;
#20340=FACE_OUTER_BOUND('',#26123,.T.) ;
#20341=FACE_OUTER_BOUND('',#26124,.T.) ;
#20342=FACE_OUTER_BOUND('',#26125,.T.) ;
#20343=FACE_OUTER_BOUND('',#26126,.T.) ;
#20344=FACE_OUTER_BOUND('',#26127,.T.) ;
#20345=FACE_OUTER_BOUND('',#26128,.T.) ;
#20346=FACE_OUTER_BOUND('',#26129,.T.) ;
#20347=FACE_OUTER_BOUND('',#26130,.T.) ;
#20348=FACE_OUTER_BOUND('',#26131,.T.) ;
#20349=FACE_OUTER_BOUND('',#26132,.T.) ;
#20350=FACE_OUTER_BOUND('',#26133,.T.) ;
#20351=FACE_OUTER_BOUND('',#26134,.T.) ;
#20352=FACE_OUTER_BOUND('',#26135,.T.) ;
#20353=FACE_OUTER_BOUND('',#26136,.T.) ;
#20354=FACE_OUTER_BOUND('',#26137,.T.) ;
#20355=FACE_OUTER_BOUND('',#26138,.T.) ;
#20356=FACE_OUTER_BOUND('',#26139,.T.) ;
#20357=FACE_OUTER_BOUND('',#26140,.T.) ;
#20358=FACE_OUTER_BOUND('',#26141,.T.) ;
#20359=FACE_OUTER_BOUND('',#26142,.T.) ;
#20360=FACE_OUTER_BOUND('',#26143,.T.) ;
#20361=FACE_OUTER_BOUND('',#26144,.T.) ;
#20362=FACE_OUTER_BOUND('',#26145,.T.) ;
#20363=FACE_OUTER_BOUND('',#26146,.T.) ;
#20364=FACE_OUTER_BOUND('',#26147,.T.) ;
#20365=FACE_OUTER_BOUND('',#26148,.T.) ;
#20366=FACE_OUTER_BOUND('',#26149,.T.) ;
#20367=FACE_OUTER_BOUND('',#26150,.T.) ;
#20368=FACE_OUTER_BOUND('',#26151,.T.) ;
#20369=FACE_OUTER_BOUND('',#26152,.T.) ;
#20370=FACE_OUTER_BOUND('',#26153,.T.) ;
#20371=FACE_OUTER_BOUND('',#26154,.T.) ;
#20372=FACE_OUTER_BOUND('',#26155,.T.) ;
#20373=FACE_OUTER_BOUND('',#26156,.T.) ;
#20374=FACE_OUTER_BOUND('',#26157,.T.) ;
#20375=FACE_OUTER_BOUND('',#26158,.T.) ;
#20376=FACE_OUTER_BOUND('',#26159,.T.) ;
#20377=FACE_OUTER_BOUND('',#26160,.T.) ;
#20378=FACE_OUTER_BOUND('',#26161,.T.) ;
#20379=FACE_OUTER_BOUND('',#26162,.T.) ;
#20380=FACE_OUTER_BOUND('',#26163,.T.) ;
#20381=FACE_OUTER_BOUND('',#26164,.T.) ;
#20382=FACE_OUTER_BOUND('',#26165,.T.) ;
#20383=FACE_OUTER_BOUND('',#26166,.T.) ;
#20384=FACE_OUTER_BOUND('',#26167,.T.) ;
#20385=FACE_OUTER_BOUND('',#26168,.T.) ;
#20386=FACE_OUTER_BOUND('',#26169,.T.) ;
#20387=FACE_OUTER_BOUND('',#26170,.T.) ;
#20388=FACE_OUTER_BOUND('',#26171,.T.) ;
#20389=FACE_OUTER_BOUND('',#26172,.T.) ;
#20390=FACE_OUTER_BOUND('',#26173,.T.) ;
#20391=FACE_OUTER_BOUND('',#26174,.T.) ;
#20392=FACE_OUTER_BOUND('',#26175,.T.) ;
#20393=FACE_OUTER_BOUND('',#26176,.T.) ;
#20394=FACE_OUTER_BOUND('',#26177,.T.) ;
#20395=FACE_OUTER_BOUND('',#26178,.T.) ;
#20396=FACE_OUTER_BOUND('',#26179,.T.) ;
#20397=FACE_OUTER_BOUND('',#26180,.T.) ;
#23921=EDGE_LOOP('',(#59139,#59140,#59141,#59142,#59143)) ;
#23922=EDGE_LOOP('',(#59144,#59145,#59146,#59147)) ;
#23923=EDGE_LOOP('',(#59148,#59149,#59150)) ;
#23924=EDGE_LOOP('',(#59151,#59152,#59153,#59154,#59155,#59156,#59157)) ;
#23925=EDGE_LOOP('',(#59158,#59159,#59160,#59161,#59162)) ;
#23926=EDGE_LOOP('',(#59163,#59164,#59165,#59166)) ;
#23927=EDGE_LOOP('',(#59167,#59168,#59169)) ;
#23928=EDGE_LOOP('',(#59170,#59171,#59172,#59173,#59174,#59175,#59176)) ;
#23929=EDGE_LOOP('',(#59177,#59178,#59179,#59180,#59181)) ;
#23930=EDGE_LOOP('',(#59182,#59183,#59184,#59185)) ;
#23931=EDGE_LOOP('',(#59186,#59187,#59188)) ;
#23932=EDGE_LOOP('',(#59189,#59190,#59191,#59192,#59193,#59194,#59195)) ;
#23933=EDGE_LOOP('',(#59196,#59197,#59198,#59199,#59200)) ;
#23934=EDGE_LOOP('',(#59201,#59202,#59203,#59204)) ;
#23935=EDGE_LOOP('',(#59205,#59206,#59207)) ;
#23936=EDGE_LOOP('',(#59208,#59209,#59210,#59211,#59212,#59213,#59214)) ;
#23937=EDGE_LOOP('',(#59215,#59216,#59217,#59218,#59219)) ;
#23938=EDGE_LOOP('',(#59220,#59221,#59222,#59223)) ;
#23939=EDGE_LOOP('',(#59224,#59225,#59226)) ;
#23940=EDGE_LOOP('',(#59227,#59228,#59229,#59230,#59231,#59232,#59233)) ;
#23941=EDGE_LOOP('',(#59234,#59235,#59236,#59237,#59238)) ;
#23942=EDGE_LOOP('',(#59239,#59240,#59241,#59242)) ;
#23943=EDGE_LOOP('',(#59243,#59244,#59245)) ;
#23944=EDGE_LOOP('',(#59246,#59247,#59248,#59249,#59250,#59251,#59252)) ;
#23945=EDGE_LOOP('',(#59253,#59254,#59255,#59256,#59257)) ;
#23946=EDGE_LOOP('',(#59258,#59259,#59260,#59261)) ;
#23947=EDGE_LOOP('',(#59262,#59263,#59264)) ;
#23948=EDGE_LOOP('',(#59265,#59266,#59267,#59268,#59269,#59270,#59271)) ;
#23949=EDGE_LOOP('',(#59272,#59273,#59274,#59275,#59276)) ;
#23950=EDGE_LOOP('',(#59277,#59278,#59279,#59280)) ;
#23951=EDGE_LOOP('',(#59281,#59282,#59283)) ;
#23952=EDGE_LOOP('',(#59284,#59285,#59286,#59287,#59288,#59289,#59290)) ;
#23953=EDGE_LOOP('',(#59291,#59292,#59293,#59294,#59295)) ;
#23954=EDGE_LOOP('',(#59296,#59297,#59298,#59299)) ;
#23955=EDGE_LOOP('',(#59300,#59301,#59302,#59303)) ;
#23956=EDGE_LOOP('',(#59304,#59305,#59306,#59307)) ;
#23957=EDGE_LOOP('',(#59308,#59309,#59310,#59311)) ;
#23958=EDGE_LOOP('',(#59312,#59313,#59314,#59315)) ;
#23959=EDGE_LOOP('',(#59316,#59317,#59318,#59319)) ;
#23960=EDGE_LOOP('',(#59320,#59321,#59322,#59323)) ;
#23961=EDGE_LOOP('',(#59324,#59325,#59326,#59327)) ;
#23962=EDGE_LOOP('',(#59328,#59329,#59330,#59331)) ;
#23963=EDGE_LOOP('',(#59332,#59333,#59334,#59335)) ;
#23964=EDGE_LOOP('',(#59336,#59337,#59338)) ;
#23965=EDGE_LOOP('',(#59339,#59340,#59341,#59342,#59343,#59344,#59345)) ;
#23966=EDGE_LOOP('',(#59346,#59347,#59348,#59349,#59350)) ;
#23967=EDGE_LOOP('',(#59351,#59352,#59353,#59354,#59355)) ;
#23968=EDGE_LOOP('',(#59356,#59357,#59358,#59359,#59360)) ;
#23969=EDGE_LOOP('',(#59361,#59362,#59363,#59364,#59365)) ;
#23970=EDGE_LOOP('',(#59366,#59367,#59368,#59369,#59370)) ;
#23971=EDGE_LOOP('',(#59371,#59372,#59373,#59374,#59375)) ;
#23972=EDGE_LOOP('',(#59376,#59377,#59378,#59379,#59380)) ;
#23973=EDGE_LOOP('',(#59381,#59382,#59383,#59384,#59385)) ;
#23974=EDGE_LOOP('',(#59386,#59387,#59388,#59389,#59390)) ;
#23975=EDGE_LOOP('',(#59391,#59392,#59393,#59394)) ;
#23976=EDGE_LOOP('',(#59395,#59396,#59397,#59398)) ;
#23977=EDGE_LOOP('',(#59399,#59400,#59401,#59402)) ;
#23978=EDGE_LOOP('',(#59403,#59404,#59405,#59406)) ;
#23979=EDGE_LOOP('',(#59407,#59408,#59409,#59410)) ;
#23980=EDGE_LOOP('',(#59411,#59412,#59413,#59414)) ;
#23981=EDGE_LOOP('',(#59415,#59416,#59417,#59418)) ;
#23982=EDGE_LOOP('',(#59419,#59420,#59421,#59422)) ;
#23983=EDGE_LOOP('',(#59423,#59424,#59425,#59426)) ;
#23984=EDGE_LOOP('',(#59427,#59428,#59429,#59430,#59431)) ;
#23985=EDGE_LOOP('',(#59432,#59433,#59434,#59435)) ;
#23986=EDGE_LOOP('',(#59436,#59437,#59438,#59439)) ;
#23987=EDGE_LOOP('',(#59440,#59441,#59442)) ;
#23988=EDGE_LOOP('',(#59443,#59444,#59445,#59446,#59447,#59448,#59449)) ;
#23989=EDGE_LOOP('',(#59450,#59451,#59452,#59453,#59454)) ;
#23990=EDGE_LOOP('',(#59455,#59456,#59457,#59458)) ;
#23991=EDGE_LOOP('',(#59459,#59460,#59461,#59462,#59463,#59464,#59465,#59466,
#59467,#59468,#59469,#59470)) ;
#23992=EDGE_LOOP('',(#59471,#59472,#59473,#59474,#59475,#59476,#59477,#59478,
#59479,#59480,#59481,#59482)) ;
#23993=EDGE_LOOP('',(#59483,#59484,#59485,#59486,#59487,#59488,#59489,#59490,
#59491,#59492,#59493,#59494)) ;
#23994=EDGE_LOOP('',(#59495,#59496,#59497,#59498,#59499,#59500,#59501,#59502,
#59503,#59504,#59505,#59506)) ;
#23995=EDGE_LOOP('',(#59507,#59508,#59509,#59510,#59511,#59512,#59513,#59514,
#59515,#59516,#59517,#59518)) ;
#23996=EDGE_LOOP('',(#59519,#59520,#59521,#59522,#59523,#59524,#59525,#59526,
#59527,#59528,#59529,#59530)) ;
#23997=EDGE_LOOP('',(#59531,#59532,#59533,#59534,#59535,#59536,#59537,#59538,
#59539,#59540,#59541,#59542)) ;
#23998=EDGE_LOOP('',(#59543,#59544,#59545,#59546,#59547,#59548,#59549,#59550,
#59551,#59552,#59553,#59554)) ;
#23999=EDGE_LOOP('',(#59555,#59556,#59557,#59558,#59559,#59560,#59561,#59562,
#59563,#59564,#59565,#59566)) ;
#24000=EDGE_LOOP('',(#59567,#59568,#59569,#59570,#59571)) ;
#24001=EDGE_LOOP('',(#59572,#59573,#59574,#59575,#59576)) ;
#24002=EDGE_LOOP('',(#59577,#59578,#59579,#59580,#59581)) ;
#24003=EDGE_LOOP('',(#59582,#59583,#59584,#59585,#59586)) ;
#24004=EDGE_LOOP('',(#59587,#59588,#59589,#59590,#59591)) ;
#24005=EDGE_LOOP('',(#59592,#59593,#59594,#59595,#59596)) ;
#24006=EDGE_LOOP('',(#59597,#59598,#59599,#59600,#59601)) ;
#24007=EDGE_LOOP('',(#59602,#59603,#59604,#59605,#59606)) ;
#24008=EDGE_LOOP('',(#59607,#59608,#59609,#59610,#59611)) ;
#24009=EDGE_LOOP('',(#59612,#59613,#59614,#59615,#59616)) ;
#24010=EDGE_LOOP('',(#59617,#59618,#59619,#59620,#59621)) ;
#24011=EDGE_LOOP('',(#59622,#59623,#59624,#59625,#59626)) ;
#24012=EDGE_LOOP('',(#59627,#59628,#59629,#59630,#59631)) ;
#24013=EDGE_LOOP('',(#59632,#59633,#59634,#59635,#59636)) ;
#24014=EDGE_LOOP('',(#59637,#59638,#59639,#59640,#59641)) ;
#24015=EDGE_LOOP('',(#59642,#59643,#59644,#59645,#59646)) ;
#24016=EDGE_LOOP('',(#59647,#59648,#59649,#59650,#59651)) ;
#24017=EDGE_LOOP('',(#59652,#59653,#59654,#59655,#59656)) ;
#24018=EDGE_LOOP('',(#59657,#59658,#59659,#59660)) ;
#24019=EDGE_LOOP('',(#59661,#59662,#59663,#59664)) ;
#24020=EDGE_LOOP('',(#59665,#59666,#59667,#59668)) ;
#24021=EDGE_LOOP('',(#59669,#59670,#59671,#59672)) ;
#24022=EDGE_LOOP('',(#59673,#59674,#59675,#59676)) ;
#24023=EDGE_LOOP('',(#59677,#59678,#59679,#59680)) ;
#24024=EDGE_LOOP('',(#59681,#59682,#59683,#59684)) ;
#24025=EDGE_LOOP('',(#59685,#59686,#59687,#59688)) ;
#24026=EDGE_LOOP('',(#59689,#59690,#59691,#59692)) ;
#24027=EDGE_LOOP('',(#59693,#59694,#59695,#59696,#59697,#59698,#59699,#59700,
#59701,#59702,#59703,#59704)) ;
#24028=EDGE_LOOP('',(#59705,#59706,#59707,#59708,#59709)) ;
#24029=EDGE_LOOP('',(#59710,#59711,#59712,#59713,#59714)) ;
#24030=EDGE_LOOP('',(#59715,#59716,#59717,#59718)) ;
#24031=EDGE_LOOP('',(#59719,#59720,#59721,#59722)) ;
#24032=EDGE_LOOP('',(#59723,#59724,#59725,#59726,#59727,#59728,#59729,#59730,
#59731,#59732,#59733,#59734,#59735,#59736,#59737,#59738,#59739,#59740,#59741,
#59742,#59743,#59744,#59745,#59746,#59747,#59748,#59749,#59750,#59751,#59752,
#59753,#59754,#59755,#59756,#59757,#59758,#59759,#59760,#59761,#59762,#59763,
#59764,#59765,#59766,#59767,#59768,#59769,#59770,#59771,#59772,#59773,#59774,
#59775,#59776,#59777,#59778,#59779,#59780,#59781,#59782,#59783,#59784,#59785,
#59786)) ;
#24033=EDGE_LOOP('',(#59787,#59788,#59789,#59790)) ;
#24034=EDGE_LOOP('',(#59791,#59792,#59793,#59794,#59795,#59796,#59797,#59798,
#59799,#59800,#59801,#59802,#59803,#59804,#59805,#59806,#59807,#59808,#59809,
#59810,#59811,#59812,#59813,#59814,#59815,#59816,#59817,#59818,#59819,#59820,
#59821,#59822,#59823,#59824,#59825,#59826,#59827,#59828,#59829,#59830,#59831,
#59832,#59833,#59834,#59835,#59836,#59837,#59838,#59839,#59840,#59841,#59842,
#59843,#59844,#59845,#59846,#59847,#59848,#59849,#59850,#59851,#59852,#59853,
#59854)) ;
#24035=EDGE_LOOP('',(#59855,#59856,#59857,#59858)) ;
#24036=EDGE_LOOP('',(#59859,#59860,#59861,#59862)) ;
#24037=EDGE_LOOP('',(#59863,#59864,#59865,#59866)) ;
#24038=EDGE_LOOP('',(#59867,#59868,#59869,#59870)) ;
#24039=EDGE_LOOP('',(#59871,#59872,#59873,#59874)) ;
#24040=EDGE_LOOP('',(#59875,#59876,#59877,#59878)) ;
#24041=EDGE_LOOP('',(#59879,#59880,#59881,#59882)) ;
#24042=EDGE_LOOP('',(#59883,#59884,#59885,#59886)) ;
#24043=EDGE_LOOP('',(#59887,#59888,#59889,#59890)) ;
#24044=EDGE_LOOP('',(#59891,#59892,#59893,#59894)) ;
#24045=EDGE_LOOP('',(#59895,#59896,#59897,#59898)) ;
#24046=EDGE_LOOP('',(#59899,#59900,#59901,#59902)) ;
#24047=EDGE_LOOP('',(#59903,#59904,#59905,#59906,#59907,#59908,#59909,#59910,
#59911,#59912,#59913,#59914,#59915,#59916,#59917,#59918,#59919,#59920,#59921,
#59922,#59923,#59924,#59925,#59926)) ;
#24048=EDGE_LOOP('',(#59927,#59928,#59929,#59930,#59931,#59932,#59933,#59934,
#59935,#59936,#59937,#59938,#59939,#59940,#59941,#59942,#59943,#59944,#59945,
#59946,#59947,#59948,#59949,#59950)) ;
#24049=EDGE_LOOP('',(#59951,#59952,#59953,#59954,#59955,#59956,#59957,#59958,
#59959,#59960,#59961,#59962,#59963,#59964,#59965,#59966,#59967,#59968,#59969,
#59970,#59971,#59972,#59973,#59974)) ;
#24050=EDGE_LOOP('',(#59975,#59976,#59977,#59978,#59979,#59980,#59981,#59982,
#59983,#59984,#59985,#59986,#59987,#59988,#59989,#59990,#59991,#59992,#59993,
#59994,#59995,#59996,#59997,#59998)) ;
#24051=EDGE_LOOP('',(#59999,#60000,#60001,#60002,#60003,#60004,#60005,#60006,
#60007,#60008,#60009,#60010,#60011,#60012,#60013,#60014,#60015,#60016,#60017,
#60018,#60019,#60020,#60021,#60022)) ;
#24052=EDGE_LOOP('',(#60023,#60024,#60025,#60026,#60027,#60028,#60029,#60030,
#60031,#60032,#60033,#60034,#60035,#60036,#60037,#60038,#60039,#60040,#60041,
#60042,#60043,#60044,#60045,#60046)) ;
#24053=EDGE_LOOP('',(#60047,#60048,#60049,#60050,#60051,#60052,#60053,#60054,
#60055,#60056,#60057,#60058,#60059,#60060,#60061,#60062,#60063,#60064,#60065,
#60066,#60067,#60068,#60069,#60070)) ;
#24054=EDGE_LOOP('',(#60071,#60072,#60073,#60074,#60075,#60076,#60077,#60078,
#60079,#60080,#60081,#60082,#60083,#60084,#60085,#60086,#60087,#60088,#60089,
#60090,#60091,#60092,#60093,#60094)) ;
#24055=EDGE_LOOP('',(#60095,#60096,#60097,#60098,#60099,#60100,#60101,#60102,
#60103,#60104,#60105,#60106,#60107,#60108,#60109,#60110,#60111,#60112,#60113,
#60114,#60115,#60116,#60117,#60118)) ;
#24056=EDGE_LOOP('',(#60119,#60120,#60121,#60122,#60123,#60124,#60125,#60126,
#60127,#60128,#60129,#60130,#60131,#60132,#60133,#60134,#60135,#60136,#60137,
#60138,#60139,#60140,#60141,#60142)) ;
#24057=EDGE_LOOP('',(#60143,#60144,#60145,#60146,#60147,#60148,#60149,#60150,
#60151,#60152)) ;
#24058=EDGE_LOOP('',(#60153,#60154,#60155,#60156,#60157,#60158,#60159,#60160,
#60161,#60162)) ;
#24059=EDGE_LOOP('',(#60163,#60164,#60165,#60166,#60167,#60168,#60169,#60170,
#60171,#60172)) ;
#24060=EDGE_LOOP('',(#60173,#60174,#60175,#60176)) ;
#24061=EDGE_LOOP('',(#60177,#60178,#60179,#60180)) ;
#24062=EDGE_LOOP('',(#60181,#60182,#60183,#60184)) ;
#24063=EDGE_LOOP('',(#60185,#60186,#60187,#60188)) ;
#24064=EDGE_LOOP('',(#60189,#60190,#60191,#60192)) ;
#24065=EDGE_LOOP('',(#60193,#60194,#60195,#60196)) ;
#24066=EDGE_LOOP('',(#60197,#60198,#60199,#60200)) ;
#24067=EDGE_LOOP('',(#60201,#60202,#60203,#60204)) ;
#24068=EDGE_LOOP('',(#60205,#60206,#60207,#60208)) ;
#24069=EDGE_LOOP('',(#60209,#60210,#60211,#60212)) ;
#24070=EDGE_LOOP('',(#60213,#60214,#60215,#60216)) ;
#24071=EDGE_LOOP('',(#60217,#60218,#60219,#60220)) ;
#24072=EDGE_LOOP('',(#60221,#60222,#60223,#60224)) ;
#24073=EDGE_LOOP('',(#60225,#60226,#60227,#60228)) ;
#24074=EDGE_LOOP('',(#60229,#60230,#60231,#60232)) ;
#24075=EDGE_LOOP('',(#60233,#60234,#60235,#60236)) ;
#24076=EDGE_LOOP('',(#60237,#60238,#60239,#60240)) ;
#24077=EDGE_LOOP('',(#60241,#60242,#60243,#60244)) ;
#24078=EDGE_LOOP('',(#60245,#60246,#60247,#60248)) ;
#24079=EDGE_LOOP('',(#60249,#60250,#60251,#60252)) ;
#24080=EDGE_LOOP('',(#60253,#60254,#60255,#60256)) ;
#24081=EDGE_LOOP('',(#60257,#60258,#60259,#60260)) ;
#24082=EDGE_LOOP('',(#60261,#60262,#60263,#60264)) ;
#24083=EDGE_LOOP('',(#60265,#60266,#60267,#60268)) ;
#24084=EDGE_LOOP('',(#60269,#60270,#60271,#60272)) ;
#24085=EDGE_LOOP('',(#60273,#60274,#60275,#60276)) ;
#24086=EDGE_LOOP('',(#60277,#60278,#60279,#60280)) ;
#24087=EDGE_LOOP('',(#60281,#60282,#60283,#60284)) ;
#24088=EDGE_LOOP('',(#60285,#60286,#60287,#60288)) ;
#24089=EDGE_LOOP('',(#60289,#60290,#60291,#60292)) ;
#24090=EDGE_LOOP('',(#60293,#60294,#60295,#60296)) ;
#24091=EDGE_LOOP('',(#60297,#60298,#60299,#60300)) ;
#24092=EDGE_LOOP('',(#60301,#60302,#60303,#60304,#60305,#60306,#60307,#60308,
#60309,#60310,#60311,#60312,#60313,#60314,#60315,#60316,#60317,#60318)) ;
#24093=EDGE_LOOP('',(#60319)) ;
#24094=EDGE_LOOP('',(#60320)) ;
#24095=EDGE_LOOP('',(#60321,#60322,#60323,#60324,#60325,#60326,#60327,#60328)) ;
#24096=EDGE_LOOP('',(#60329,#60330,#60331,#60332)) ;
#24097=EDGE_LOOP('',(#60333,#60334,#60335,#60336)) ;
#24098=EDGE_LOOP('',(#60337,#60338,#60339)) ;
#24099=EDGE_LOOP('',(#60340,#60341,#60342)) ;
#24100=EDGE_LOOP('',(#60343,#60344,#60345,#60346)) ;
#24101=EDGE_LOOP('',(#60347,#60348,#60349,#60350,#60351,#60352)) ;
#24102=EDGE_LOOP('',(#60353,#60354,#60355,#60356,#60357,#60358,#60359)) ;
#24103=EDGE_LOOP('',(#60360,#60361,#60362,#60363)) ;
#24104=EDGE_LOOP('',(#60364,#60365,#60366,#60367)) ;
#24105=EDGE_LOOP('',(#60368,#60369,#60370,#60371)) ;
#24106=EDGE_LOOP('',(#60372,#60373,#60374,#60375)) ;
#24107=EDGE_LOOP('',(#60376,#60377,#60378)) ;
#24108=EDGE_LOOP('',(#60379,#60380,#60381,#60382)) ;
#24109=EDGE_LOOP('',(#60383,#60384,#60385,#60386)) ;
#24110=EDGE_LOOP('',(#60387,#60388,#60389,#60390)) ;
#24111=EDGE_LOOP('',(#60391,#60392,#60393,#60394)) ;
#24112=EDGE_LOOP('',(#60395,#60396,#60397,#60398)) ;
#24113=EDGE_LOOP('',(#60399,#60400,#60401,#60402)) ;
#24114=EDGE_LOOP('',(#60403,#60404,#60405,#60406)) ;
#24115=EDGE_LOOP('',(#60407,#60408,#60409,#60410)) ;
#24116=EDGE_LOOP('',(#60411,#60412,#60413,#60414)) ;
#24117=EDGE_LOOP('',(#60415,#60416,#60417)) ;
#24118=EDGE_LOOP('',(#60418,#60419,#60420)) ;
#24119=EDGE_LOOP('',(#60421,#60422,#60423,#60424,#60425)) ;
#24120=EDGE_LOOP('',(#60426,#60427,#60428)) ;
#24121=EDGE_LOOP('',(#60429,#60430,#60431)) ;
#24122=EDGE_LOOP('',(#60432,#60433,#60434,#60435)) ;
#24123=EDGE_LOOP('',(#60436,#60437,#60438,#60439)) ;
#24124=EDGE_LOOP('',(#60440,#60441,#60442,#60443)) ;
#24125=EDGE_LOOP('',(#60444,#60445,#60446,#60447)) ;
#24126=EDGE_LOOP('',(#60448,#60449,#60450,#60451)) ;
#24127=EDGE_LOOP('',(#60452,#60453,#60454,#60455)) ;
#24128=EDGE_LOOP('',(#60456,#60457,#60458,#60459)) ;
#24129=EDGE_LOOP('',(#60460,#60461,#60462)) ;
#24130=EDGE_LOOP('',(#60463,#60464,#60465,#60466)) ;
#24131=EDGE_LOOP('',(#60467,#60468,#60469,#60470)) ;
#24132=EDGE_LOOP('',(#60471,#60472,#60473)) ;
#24133=EDGE_LOOP('',(#60474,#60475,#60476,#60477)) ;
#24134=EDGE_LOOP('',(#60478,#60479,#60480,#60481)) ;
#24135=EDGE_LOOP('',(#60482,#60483,#60484,#60485)) ;
#24136=EDGE_LOOP('',(#60486,#60487,#60488,#60489)) ;
#24137=EDGE_LOOP('',(#60490,#60491,#60492,#60493)) ;
#24138=EDGE_LOOP('',(#60494,#60495,#60496,#60497)) ;
#24139=EDGE_LOOP('',(#60498,#60499,#60500,#60501,#60502)) ;
#24140=EDGE_LOOP('',(#60503,#60504,#60505,#60506)) ;
#24141=EDGE_LOOP('',(#60507,#60508,#60509)) ;
#24142=EDGE_LOOP('',(#60510,#60511,#60512)) ;
#24143=EDGE_LOOP('',(#60513,#60514,#60515,#60516)) ;
#24144=EDGE_LOOP('',(#60517,#60518,#60519,#60520)) ;
#24145=EDGE_LOOP('',(#60521,#60522,#60523,#60524)) ;
#24146=EDGE_LOOP('',(#60525,#60526,#60527)) ;
#24147=EDGE_LOOP('',(#60528,#60529,#60530,#60531)) ;
#24148=EDGE_LOOP('',(#60532,#60533,#60534,#60535)) ;
#24149=EDGE_LOOP('',(#60536,#60537,#60538)) ;
#24150=EDGE_LOOP('',(#60539,#60540,#60541,#60542)) ;
#24151=EDGE_LOOP('',(#60543,#60544,#60545,#60546)) ;
#24152=EDGE_LOOP('',(#60547,#60548,#60549,#60550)) ;
#24153=EDGE_LOOP('',(#60551,#60552,#60553)) ;
#24154=EDGE_LOOP('',(#60554,#60555,#60556)) ;
#24155=EDGE_LOOP('',(#60557,#60558,#60559,#60560)) ;
#24156=EDGE_LOOP('',(#60561,#60562,#60563,#60564)) ;
#24157=EDGE_LOOP('',(#60565,#60566,#60567)) ;
#24158=EDGE_LOOP('',(#60568,#60569,#60570)) ;
#24159=EDGE_LOOP('',(#60571,#60572,#60573,#60574)) ;
#24160=EDGE_LOOP('',(#60575,#60576,#60577,#60578)) ;
#24161=EDGE_LOOP('',(#60579,#60580,#60581,#60582)) ;
#24162=EDGE_LOOP('',(#60583,#60584,#60585)) ;
#24163=EDGE_LOOP('',(#60586,#60587,#60588,#60589)) ;
#24164=EDGE_LOOP('',(#60590,#60591,#60592,#60593)) ;
#24165=EDGE_LOOP('',(#60594,#60595,#60596)) ;
#24166=EDGE_LOOP('',(#60597,#60598,#60599,#60600)) ;
#24167=EDGE_LOOP('',(#60601,#60602,#60603,#60604)) ;
#24168=EDGE_LOOP('',(#60605,#60606,#60607,#60608)) ;
#24169=EDGE_LOOP('',(#60609,#60610,#60611)) ;
#24170=EDGE_LOOP('',(#60612,#60613,#60614)) ;
#24171=EDGE_LOOP('',(#60615,#60616,#60617,#60618)) ;
#24172=EDGE_LOOP('',(#60619,#60620,#60621,#60622)) ;
#24173=EDGE_LOOP('',(#60623,#60624,#60625)) ;
#24174=EDGE_LOOP('',(#60626,#60627,#60628,#60629)) ;
#24175=EDGE_LOOP('',(#60630,#60631,#60632,#60633)) ;
#24176=EDGE_LOOP('',(#60634,#60635,#60636)) ;
#24177=EDGE_LOOP('',(#60637,#60638,#60639,#60640)) ;
#24178=EDGE_LOOP('',(#60641,#60642,#60643,#60644)) ;
#24179=EDGE_LOOP('',(#60645,#60646,#60647,#60648)) ;
#24180=EDGE_LOOP('',(#60649,#60650,#60651)) ;
#24181=EDGE_LOOP('',(#60652,#60653,#60654,#60655)) ;
#24182=EDGE_LOOP('',(#60656,#60657,#60658,#60659)) ;
#24183=EDGE_LOOP('',(#60660,#60661,#60662)) ;
#24184=EDGE_LOOP('',(#60663,#60664,#60665)) ;
#24185=EDGE_LOOP('',(#60666,#60667,#60668,#60669)) ;
#24186=EDGE_LOOP('',(#60670,#60671,#60672,#60673)) ;
#24187=EDGE_LOOP('',(#60674,#60675,#60676)) ;
#24188=EDGE_LOOP('',(#60677,#60678,#60679)) ;
#24189=EDGE_LOOP('',(#60680,#60681,#60682,#60683)) ;
#24190=EDGE_LOOP('',(#60684,#60685,#60686,#60687)) ;
#24191=EDGE_LOOP('',(#60688,#60689,#60690)) ;
#24192=EDGE_LOOP('',(#60691,#60692,#60693,#60694)) ;
#24193=EDGE_LOOP('',(#60695,#60696,#60697,#60698)) ;
#24194=EDGE_LOOP('',(#60699,#60700,#60701)) ;
#24195=EDGE_LOOP('',(#60702,#60703,#60704)) ;
#24196=EDGE_LOOP('',(#60705,#60706,#60707,#60708)) ;
#24197=EDGE_LOOP('',(#60709,#60710,#60711,#60712)) ;
#24198=EDGE_LOOP('',(#60713,#60714,#60715,#60716)) ;
#24199=EDGE_LOOP('',(#60717,#60718,#60719,#60720)) ;
#24200=EDGE_LOOP('',(#60721,#60722,#60723,#60724)) ;
#24201=EDGE_LOOP('',(#60725,#60726,#60727,#60728)) ;
#24202=EDGE_LOOP('',(#60729,#60730,#60731)) ;
#24203=EDGE_LOOP('',(#60732,#60733,#60734)) ;
#24204=EDGE_LOOP('',(#60735,#60736,#60737,#60738)) ;
#24205=EDGE_LOOP('',(#60739,#60740,#60741,#60742)) ;
#24206=EDGE_LOOP('',(#60743,#60744,#60745,#60746)) ;
#24207=EDGE_LOOP('',(#60747,#60748,#60749,#60750)) ;
#24208=EDGE_LOOP('',(#60751,#60752,#60753,#60754)) ;
#24209=EDGE_LOOP('',(#60755,#60756,#60757,#60758)) ;
#24210=EDGE_LOOP('',(#60759,#60760,#60761,#60762)) ;
#24211=EDGE_LOOP('',(#60763,#60764,#60765,#60766)) ;
#24212=EDGE_LOOP('',(#60767,#60768,#60769,#60770)) ;
#24213=EDGE_LOOP('',(#60771,#60772,#60773,#60774)) ;
#24214=EDGE_LOOP('',(#60775,#60776,#60777,#60778)) ;
#24215=EDGE_LOOP('',(#60779,#60780,#60781,#60782)) ;
#24216=EDGE_LOOP('',(#60783,#60784,#60785,#60786)) ;
#24217=EDGE_LOOP('',(#60787,#60788,#60789,#60790)) ;
#24218=EDGE_LOOP('',(#60791,#60792,#60793,#60794)) ;
#24219=EDGE_LOOP('',(#60795,#60796,#60797,#60798)) ;
#24220=EDGE_LOOP('',(#60799,#60800,#60801,#60802)) ;
#24221=EDGE_LOOP('',(#60803,#60804,#60805)) ;
#24222=EDGE_LOOP('',(#60806,#60807,#60808,#60809)) ;
#24223=EDGE_LOOP('',(#60810,#60811,#60812,#60813)) ;
#24224=EDGE_LOOP('',(#60814,#60815,#60816,#60817)) ;
#24225=EDGE_LOOP('',(#60818,#60819,#60820)) ;
#24226=EDGE_LOOP('',(#60821,#60822,#60823,#60824)) ;
#24227=EDGE_LOOP('',(#60825,#60826,#60827,#60828)) ;
#24228=EDGE_LOOP('',(#60829,#60830,#60831,#60832)) ;
#24229=EDGE_LOOP('',(#60833,#60834,#60835,#60836)) ;
#24230=EDGE_LOOP('',(#60837,#60838,#60839,#60840)) ;
#24231=EDGE_LOOP('',(#60841,#60842,#60843,#60844)) ;
#24232=EDGE_LOOP('',(#60845,#60846,#60847,#60848)) ;
#24233=EDGE_LOOP('',(#60849,#60850,#60851,#60852,#60853,#60854)) ;
#24234=EDGE_LOOP('',(#60855,#60856,#60857,#60858,#60859,#60860)) ;
#24235=EDGE_LOOP('',(#60861,#60862,#60863,#60864,#60865)) ;
#24236=EDGE_LOOP('',(#60866,#60867,#60868,#60869)) ;
#24237=EDGE_LOOP('',(#60870,#60871,#60872,#60873)) ;
#24238=EDGE_LOOP('',(#60874,#60875,#60876,#60877)) ;
#24239=EDGE_LOOP('',(#60878,#60879,#60880,#60881)) ;
#24240=EDGE_LOOP('',(#60882,#60883,#60884,#60885)) ;
#24241=EDGE_LOOP('',(#60886,#60887,#60888,#60889)) ;
#24242=EDGE_LOOP('',(#60890,#60891,#60892,#60893)) ;
#24243=EDGE_LOOP('',(#60894,#60895,#60896,#60897)) ;
#24244=EDGE_LOOP('',(#60898,#60899,#60900,#60901)) ;
#24245=EDGE_LOOP('',(#60902,#60903,#60904,#60905)) ;
#24246=EDGE_LOOP('',(#60906,#60907,#60908,#60909)) ;
#24247=EDGE_LOOP('',(#60910,#60911,#60912,#60913)) ;
#24248=EDGE_LOOP('',(#60914,#60915,#60916,#60917)) ;
#24249=EDGE_LOOP('',(#60918,#60919,#60920,#60921)) ;
#24250=EDGE_LOOP('',(#60922,#60923,#60924)) ;
#24251=EDGE_LOOP('',(#60925,#60926,#60927,#60928)) ;
#24252=EDGE_LOOP('',(#60929,#60930,#60931,#60932)) ;
#24253=EDGE_LOOP('',(#60933,#60934,#60935,#60936)) ;
#24254=EDGE_LOOP('',(#60937,#60938,#60939)) ;
#24255=EDGE_LOOP('',(#60940,#60941,#60942)) ;
#24256=EDGE_LOOP('',(#60943,#60944,#60945,#60946)) ;
#24257=EDGE_LOOP('',(#60947,#60948,#60949,#60950)) ;
#24258=EDGE_LOOP('',(#60951,#60952,#60953,#60954)) ;
#24259=EDGE_LOOP('',(#60955,#60956,#60957)) ;
#24260=EDGE_LOOP('',(#60958,#60959,#60960,#60961)) ;
#24261=EDGE_LOOP('',(#60962,#60963,#60964,#60965)) ;
#24262=EDGE_LOOP('',(#60966,#60967,#60968,#60969)) ;
#24263=EDGE_LOOP('',(#60970,#60971,#60972,#60973)) ;
#24264=EDGE_LOOP('',(#60974,#60975,#60976)) ;
#24265=EDGE_LOOP('',(#60977,#60978,#60979,#60980)) ;
#24266=EDGE_LOOP('',(#60981,#60982,#60983,#60984)) ;
#24267=EDGE_LOOP('',(#60985,#60986,#60987,#60988)) ;
#24268=EDGE_LOOP('',(#60989,#60990,#60991)) ;
#24269=EDGE_LOOP('',(#60992,#60993,#60994)) ;
#24270=EDGE_LOOP('',(#60995,#60996,#60997,#60998)) ;
#24271=EDGE_LOOP('',(#60999,#61000,#61001,#61002)) ;
#24272=EDGE_LOOP('',(#61003,#61004,#61005,#61006)) ;
#24273=EDGE_LOOP('',(#61007,#61008,#61009)) ;
#24274=EDGE_LOOP('',(#61010,#61011,#61012,#61013)) ;
#24275=EDGE_LOOP('',(#61014,#61015,#61016,#61017)) ;
#24276=EDGE_LOOP('',(#61018,#61019,#61020,#61021)) ;
#24277=EDGE_LOOP('',(#61022,#61023,#61024,#61025)) ;
#24278=EDGE_LOOP('',(#61026,#61027,#61028,#61029)) ;
#24279=EDGE_LOOP('',(#61030,#61031,#61032,#61033)) ;
#24280=EDGE_LOOP('',(#61034,#61035,#61036,#61037)) ;
#24281=EDGE_LOOP('',(#61038,#61039,#61040,#61041)) ;
#24282=EDGE_LOOP('',(#61042,#61043,#61044,#61045,#61046)) ;
#24283=EDGE_LOOP('',(#61047,#61048,#61049,#61050)) ;
#24284=EDGE_LOOP('',(#61051,#61052,#61053,#61054)) ;
#24285=EDGE_LOOP('',(#61055,#61056,#61057,#61058)) ;
#24286=EDGE_LOOP('',(#61059,#61060,#61061,#61062)) ;
#24287=EDGE_LOOP('',(#61063,#61064,#61065,#61066)) ;
#24288=EDGE_LOOP('',(#61067,#61068,#61069,#61070)) ;
#24289=EDGE_LOOP('',(#61071,#61072,#61073,#61074)) ;
#24290=EDGE_LOOP('',(#61075,#61076,#61077,#61078)) ;
#24291=EDGE_LOOP('',(#61079,#61080,#61081,#61082)) ;
#24292=EDGE_LOOP('',(#61083,#61084,#61085,#61086)) ;
#24293=EDGE_LOOP('',(#61087,#61088,#61089,#61090)) ;
#24294=EDGE_LOOP('',(#61091,#61092,#61093,#61094)) ;
#24295=EDGE_LOOP('',(#61095,#61096,#61097,#61098)) ;
#24296=EDGE_LOOP('',(#61099,#61100,#61101,#61102)) ;
#24297=EDGE_LOOP('',(#61103,#61104,#61105,#61106)) ;
#24298=EDGE_LOOP('',(#61107,#61108,#61109,#61110)) ;
#24299=EDGE_LOOP('',(#61111,#61112,#61113,#61114)) ;
#24300=EDGE_LOOP('',(#61115,#61116,#61117,#61118,#61119,#61120,#61121,#61122,
#61123,#61124)) ;
#24301=EDGE_LOOP('',(#61125,#61126,#61127,#61128,#61129,#61130,#61131,#61132,
#61133,#61134)) ;
#24302=EDGE_LOOP('',(#61135,#61136,#61137,#61138,#61139,#61140,#61141,#61142,
#61143,#61144)) ;
#24303=EDGE_LOOP('',(#61145,#61146,#61147,#61148,#61149,#61150,#61151,#61152,
#61153,#61154)) ;
#24304=EDGE_LOOP('',(#61155,#61156,#61157,#61158,#61159,#61160,#61161,#61162,
#61163,#61164)) ;
#24305=EDGE_LOOP('',(#61165,#61166,#61167,#61168,#61169,#61170,#61171,#61172,
#61173,#61174)) ;
#24306=EDGE_LOOP('',(#61175,#61176,#61177,#61178,#61179,#61180,#61181,#61182,
#61183,#61184)) ;
#24307=EDGE_LOOP('',(#61185,#61186,#61187,#61188,#61189,#61190,#61191,#61192,
#61193,#61194)) ;
#24308=EDGE_LOOP('',(#61195,#61196,#61197,#61198,#61199,#61200,#61201,#61202,
#61203,#61204)) ;
#24309=EDGE_LOOP('',(#61205,#61206,#61207,#61208)) ;
#24310=EDGE_LOOP('',(#61209,#61210,#61211,#61212)) ;
#24311=EDGE_LOOP('',(#61213,#61214,#61215,#61216)) ;
#24312=EDGE_LOOP('',(#61217,#61218,#61219,#61220)) ;
#24313=EDGE_LOOP('',(#61221,#61222,#61223,#61224)) ;
#24314=EDGE_LOOP('',(#61225,#61226,#61227,#61228)) ;
#24315=EDGE_LOOP('',(#61229,#61230,#61231,#61232)) ;
#24316=EDGE_LOOP('',(#61233,#61234,#61235,#61236)) ;
#24317=EDGE_LOOP('',(#61237,#61238,#61239,#61240)) ;
#24318=EDGE_LOOP('',(#61241,#61242,#61243,#61244)) ;
#24319=EDGE_LOOP('',(#61245,#61246,#61247,#61248)) ;
#24320=EDGE_LOOP('',(#61249,#61250,#61251,#61252)) ;
#24321=EDGE_LOOP('',(#61253,#61254,#61255,#61256)) ;
#24322=EDGE_LOOP('',(#61257,#61258,#61259,#61260)) ;
#24323=EDGE_LOOP('',(#61261,#61262,#61263,#61264)) ;
#24324=EDGE_LOOP('',(#61265,#61266,#61267,#61268)) ;
#24325=EDGE_LOOP('',(#61269,#61270,#61271,#61272)) ;
#24326=EDGE_LOOP('',(#61273,#61274,#61275,#61276)) ;
#24327=EDGE_LOOP('',(#61277,#61278,#61279,#61280)) ;
#24328=EDGE_LOOP('',(#61281,#61282,#61283,#61284)) ;
#24329=EDGE_LOOP('',(#61285,#61286,#61287,#61288)) ;
#24330=EDGE_LOOP('',(#61289,#61290,#61291,#61292)) ;
#24331=EDGE_LOOP('',(#61293,#61294,#61295,#61296)) ;
#24332=EDGE_LOOP('',(#61297,#61298,#61299,#61300)) ;
#24333=EDGE_LOOP('',(#61301,#61302,#61303,#61304)) ;
#24334=EDGE_LOOP('',(#61305,#61306,#61307,#61308)) ;
#24335=EDGE_LOOP('',(#61309,#61310,#61311,#61312)) ;
#24336=EDGE_LOOP('',(#61313,#61314,#61315,#61316)) ;
#24337=EDGE_LOOP('',(#61317,#61318,#61319,#61320)) ;
#24338=EDGE_LOOP('',(#61321,#61322,#61323,#61324)) ;
#24339=EDGE_LOOP('',(#61325,#61326,#61327,#61328)) ;
#24340=EDGE_LOOP('',(#61329,#61330,#61331,#61332)) ;
#24341=EDGE_LOOP('',(#61333,#61334,#61335,#61336)) ;
#24342=EDGE_LOOP('',(#61337,#61338,#61339,#61340)) ;
#24343=EDGE_LOOP('',(#61341,#61342,#61343,#61344)) ;
#24344=EDGE_LOOP('',(#61345,#61346,#61347,#61348)) ;
#24345=EDGE_LOOP('',(#61349,#61350,#61351,#61352)) ;
#24346=EDGE_LOOP('',(#61353,#61354,#61355,#61356)) ;
#24347=EDGE_LOOP('',(#61357,#61358,#61359,#61360)) ;
#24348=EDGE_LOOP('',(#61361,#61362,#61363,#61364)) ;
#24349=EDGE_LOOP('',(#61365,#61366,#61367,#61368)) ;
#24350=EDGE_LOOP('',(#61369,#61370,#61371,#61372)) ;
#24351=EDGE_LOOP('',(#61373,#61374,#61375,#61376)) ;
#24352=EDGE_LOOP('',(#61377,#61378,#61379,#61380)) ;
#24353=EDGE_LOOP('',(#61381,#61382,#61383,#61384)) ;
#24354=EDGE_LOOP('',(#61385,#61386,#61387,#61388)) ;
#24355=EDGE_LOOP('',(#61389,#61390,#61391,#61392)) ;
#24356=EDGE_LOOP('',(#61393,#61394,#61395,#61396)) ;
#24357=EDGE_LOOP('',(#61397,#61398,#61399,#61400)) ;
#24358=EDGE_LOOP('',(#61401,#61402,#61403,#61404)) ;
#24359=EDGE_LOOP('',(#61405,#61406,#61407,#61408)) ;
#24360=EDGE_LOOP('',(#61409,#61410,#61411,#61412)) ;
#24361=EDGE_LOOP('',(#61413,#61414,#61415,#61416)) ;
#24362=EDGE_LOOP('',(#61417,#61418,#61419,#61420)) ;
#24363=EDGE_LOOP('',(#61421,#61422,#61423,#61424)) ;
#24364=EDGE_LOOP('',(#61425,#61426,#61427,#61428)) ;
#24365=EDGE_LOOP('',(#61429,#61430,#61431,#61432)) ;
#24366=EDGE_LOOP('',(#61433,#61434,#61435,#61436)) ;
#24367=EDGE_LOOP('',(#61437,#61438,#61439,#61440)) ;
#24368=EDGE_LOOP('',(#61441,#61442,#61443,#61444)) ;
#24369=EDGE_LOOP('',(#61445,#61446,#61447,#61448)) ;
#24370=EDGE_LOOP('',(#61449,#61450,#61451,#61452)) ;
#24371=EDGE_LOOP('',(#61453,#61454,#61455,#61456)) ;
#24372=EDGE_LOOP('',(#61457,#61458,#61459,#61460)) ;
#24373=EDGE_LOOP('',(#61461,#61462,#61463,#61464)) ;
#24374=EDGE_LOOP('',(#61465,#61466,#61467,#61468)) ;
#24375=EDGE_LOOP('',(#61469,#61470,#61471,#61472)) ;
#24376=EDGE_LOOP('',(#61473,#61474,#61475,#61476)) ;
#24377=EDGE_LOOP('',(#61477,#61478,#61479,#61480)) ;
#24378=EDGE_LOOP('',(#61481,#61482,#61483,#61484)) ;
#24379=EDGE_LOOP('',(#61485,#61486,#61487,#61488)) ;
#24380=EDGE_LOOP('',(#61489,#61490,#61491,#61492)) ;
#24381=EDGE_LOOP('',(#61493,#61494,#61495,#61496,#61497,#61498,#61499,#61500,
#61501,#61502,#61503,#61504,#61505,#61506,#61507,#61508,#61509,#61510)) ;
#24382=EDGE_LOOP('',(#61511)) ;
#24383=EDGE_LOOP('',(#61512,#61513,#61514,#61515)) ;
#24384=EDGE_LOOP('',(#61516,#61517,#61518,#61519)) ;
#24385=EDGE_LOOP('',(#61520,#61521,#61522,#61523)) ;
#24386=EDGE_LOOP('',(#61524,#61525,#61526,#61527)) ;
#24387=EDGE_LOOP('',(#61528,#61529,#61530,#61531)) ;
#24388=EDGE_LOOP('',(#61532,#61533,#61534,#61535)) ;
#24389=EDGE_LOOP('',(#61536,#61537,#61538,#61539)) ;
#24390=EDGE_LOOP('',(#61540,#61541,#61542,#61543)) ;
#24391=EDGE_LOOP('',(#61544,#61545,#61546,#61547)) ;
#24392=EDGE_LOOP('',(#61548,#61549,#61550,#61551)) ;
#24393=EDGE_LOOP('',(#61552,#61553,#61554,#61555)) ;
#24394=EDGE_LOOP('',(#61556,#61557,#61558,#61559)) ;
#24395=EDGE_LOOP('',(#61560,#61561,#61562,#61563)) ;
#24396=EDGE_LOOP('',(#61564,#61565,#61566,#61567)) ;
#24397=EDGE_LOOP('',(#61568,#61569,#61570,#61571)) ;
#24398=EDGE_LOOP('',(#61572,#61573,#61574,#61575)) ;
#24399=EDGE_LOOP('',(#61576,#61577,#61578,#61579)) ;
#24400=EDGE_LOOP('',(#61580,#61581,#61582,#61583)) ;
#24401=EDGE_LOOP('',(#61584,#61585,#61586,#61587)) ;
#24402=EDGE_LOOP('',(#61588,#61589,#61590,#61591)) ;
#24403=EDGE_LOOP('',(#61592,#61593,#61594,#61595)) ;
#24404=EDGE_LOOP('',(#61596,#61597,#61598,#61599)) ;
#24405=EDGE_LOOP('',(#61600,#61601,#61602,#61603)) ;
#24406=EDGE_LOOP('',(#61604,#61605,#61606,#61607)) ;
#24407=EDGE_LOOP('',(#61608,#61609,#61610,#61611)) ;
#24408=EDGE_LOOP('',(#61612,#61613,#61614,#61615)) ;
#24409=EDGE_LOOP('',(#61616,#61617,#61618,#61619)) ;
#24410=EDGE_LOOP('',(#61620,#61621,#61622,#61623,#61624,#61625,#61626,#61627,
#61628,#61629,#61630,#61631,#61632,#61633,#61634,#61635,#61636,#61637)) ;
#24411=EDGE_LOOP('',(#61638)) ;
#24412=EDGE_LOOP('',(#61639,#61640,#61641,#61642)) ;
#24413=EDGE_LOOP('',(#61643,#61644,#61645,#61646)) ;
#24414=EDGE_LOOP('',(#61647,#61648,#61649,#61650)) ;
#24415=EDGE_LOOP('',(#61651,#61652,#61653,#61654)) ;
#24416=EDGE_LOOP('',(#61655,#61656,#61657,#61658)) ;
#24417=EDGE_LOOP('',(#61659,#61660,#61661,#61662)) ;
#24418=EDGE_LOOP('',(#61663,#61664,#61665,#61666)) ;
#24419=EDGE_LOOP('',(#61667,#61668,#61669,#61670)) ;
#24420=EDGE_LOOP('',(#61671,#61672,#61673,#61674)) ;
#24421=EDGE_LOOP('',(#61675,#61676,#61677,#61678)) ;
#24422=EDGE_LOOP('',(#61679,#61680,#61681,#61682)) ;
#24423=EDGE_LOOP('',(#61683,#61684,#61685,#61686)) ;
#24424=EDGE_LOOP('',(#61687,#61688,#61689,#61690)) ;
#24425=EDGE_LOOP('',(#61691,#61692,#61693,#61694)) ;
#24426=EDGE_LOOP('',(#61695,#61696,#61697,#61698)) ;
#24427=EDGE_LOOP('',(#61699,#61700,#61701,#61702)) ;
#24428=EDGE_LOOP('',(#61703,#61704,#61705,#61706)) ;
#24429=EDGE_LOOP('',(#61707,#61708,#61709,#61710)) ;
#24430=EDGE_LOOP('',(#61711,#61712,#61713,#61714)) ;
#24431=EDGE_LOOP('',(#61715,#61716,#61717,#61718)) ;
#24432=EDGE_LOOP('',(#61719,#61720,#61721,#61722)) ;
#24433=EDGE_LOOP('',(#61723,#61724,#61725,#61726)) ;
#24434=EDGE_LOOP('',(#61727,#61728,#61729,#61730)) ;
#24435=EDGE_LOOP('',(#61731,#61732,#61733,#61734)) ;
#24436=EDGE_LOOP('',(#61735,#61736,#61737,#61738)) ;
#24437=EDGE_LOOP('',(#61739,#61740,#61741,#61742)) ;
#24438=EDGE_LOOP('',(#61743,#61744,#61745,#61746)) ;
#24439=EDGE_LOOP('',(#61747,#61748,#61749,#61750,#61751,#61752,#61753,#61754,
#61755,#61756,#61757,#61758,#61759,#61760,#61761,#61762,#61763,#61764)) ;
#24440=EDGE_LOOP('',(#61765)) ;
#24441=EDGE_LOOP('',(#61766,#61767,#61768,#61769)) ;
#24442=EDGE_LOOP('',(#61770,#61771,#61772,#61773)) ;
#24443=EDGE_LOOP('',(#61774,#61775,#61776,#61777)) ;
#24444=EDGE_LOOP('',(#61778,#61779,#61780,#61781)) ;
#24445=EDGE_LOOP('',(#61782,#61783,#61784,#61785)) ;
#24446=EDGE_LOOP('',(#61786,#61787,#61788,#61789)) ;
#24447=EDGE_LOOP('',(#61790,#61791,#61792,#61793)) ;
#24448=EDGE_LOOP('',(#61794,#61795,#61796,#61797)) ;
#24449=EDGE_LOOP('',(#61798,#61799,#61800,#61801)) ;
#24450=EDGE_LOOP('',(#61802,#61803,#61804,#61805)) ;
#24451=EDGE_LOOP('',(#61806,#61807,#61808,#61809)) ;
#24452=EDGE_LOOP('',(#61810,#61811,#61812,#61813)) ;
#24453=EDGE_LOOP('',(#61814,#61815,#61816,#61817)) ;
#24454=EDGE_LOOP('',(#61818,#61819,#61820,#61821)) ;
#24455=EDGE_LOOP('',(#61822,#61823,#61824,#61825)) ;
#24456=EDGE_LOOP('',(#61826,#61827,#61828,#61829)) ;
#24457=EDGE_LOOP('',(#61830,#61831,#61832,#61833)) ;
#24458=EDGE_LOOP('',(#61834,#61835,#61836,#61837)) ;
#24459=EDGE_LOOP('',(#61838,#61839,#61840,#61841)) ;
#24460=EDGE_LOOP('',(#61842,#61843,#61844,#61845)) ;
#24461=EDGE_LOOP('',(#61846,#61847,#61848,#61849)) ;
#24462=EDGE_LOOP('',(#61850,#61851,#61852,#61853)) ;
#24463=EDGE_LOOP('',(#61854,#61855,#61856,#61857)) ;
#24464=EDGE_LOOP('',(#61858,#61859,#61860,#61861)) ;
#24465=EDGE_LOOP('',(#61862,#61863,#61864,#61865)) ;
#24466=EDGE_LOOP('',(#61866,#61867,#61868,#61869)) ;
#24467=EDGE_LOOP('',(#61870,#61871,#61872,#61873)) ;
#24468=EDGE_LOOP('',(#61874,#61875,#61876,#61877,#61878,#61879,#61880,#61881,
#61882,#61883,#61884,#61885,#61886,#61887,#61888,#61889,#61890,#61891)) ;
#24469=EDGE_LOOP('',(#61892)) ;
#24470=EDGE_LOOP('',(#61893,#61894,#61895,#61896)) ;
#24471=EDGE_LOOP('',(#61897,#61898,#61899,#61900)) ;
#24472=EDGE_LOOP('',(#61901,#61902,#61903,#61904)) ;
#24473=EDGE_LOOP('',(#61905,#61906,#61907,#61908)) ;
#24474=EDGE_LOOP('',(#61909,#61910,#61911,#61912)) ;
#24475=EDGE_LOOP('',(#61913,#61914,#61915,#61916)) ;
#24476=EDGE_LOOP('',(#61917,#61918,#61919,#61920)) ;
#24477=EDGE_LOOP('',(#61921,#61922,#61923,#61924)) ;
#24478=EDGE_LOOP('',(#61925,#61926,#61927,#61928)) ;
#24479=EDGE_LOOP('',(#61929,#61930,#61931,#61932)) ;
#24480=EDGE_LOOP('',(#61933,#61934,#61935,#61936)) ;
#24481=EDGE_LOOP('',(#61937,#61938,#61939,#61940)) ;
#24482=EDGE_LOOP('',(#61941,#61942,#61943,#61944)) ;
#24483=EDGE_LOOP('',(#61945,#61946,#61947,#61948)) ;
#24484=EDGE_LOOP('',(#61949,#61950,#61951,#61952)) ;
#24485=EDGE_LOOP('',(#61953,#61954,#61955,#61956)) ;
#24486=EDGE_LOOP('',(#61957,#61958,#61959,#61960)) ;
#24487=EDGE_LOOP('',(#61961,#61962,#61963,#61964)) ;
#24488=EDGE_LOOP('',(#61965,#61966,#61967,#61968)) ;
#24489=EDGE_LOOP('',(#61969,#61970,#61971,#61972)) ;
#24490=EDGE_LOOP('',(#61973,#61974,#61975,#61976)) ;
#24491=EDGE_LOOP('',(#61977,#61978,#61979,#61980)) ;
#24492=EDGE_LOOP('',(#61981,#61982,#61983,#61984)) ;
#24493=EDGE_LOOP('',(#61985,#61986,#61987,#61988)) ;
#24494=EDGE_LOOP('',(#61989,#61990,#61991,#61992)) ;
#24495=EDGE_LOOP('',(#61993,#61994,#61995,#61996)) ;
#24496=EDGE_LOOP('',(#61997,#61998,#61999,#62000)) ;
#24497=EDGE_LOOP('',(#62001,#62002,#62003,#62004,#62005,#62006,#62007,#62008,
#62009,#62010,#62011,#62012,#62013,#62014,#62015,#62016,#62017,#62018)) ;
#24498=EDGE_LOOP('',(#62019)) ;
#24499=EDGE_LOOP('',(#62020,#62021,#62022,#62023)) ;
#24500=EDGE_LOOP('',(#62024,#62025,#62026,#62027)) ;
#24501=EDGE_LOOP('',(#62028,#62029,#62030,#62031)) ;
#24502=EDGE_LOOP('',(#62032,#62033,#62034,#62035)) ;
#24503=EDGE_LOOP('',(#62036,#62037,#62038,#62039)) ;
#24504=EDGE_LOOP('',(#62040,#62041,#62042,#62043)) ;
#24505=EDGE_LOOP('',(#62044,#62045,#62046,#62047)) ;
#24506=EDGE_LOOP('',(#62048,#62049,#62050,#62051)) ;
#24507=EDGE_LOOP('',(#62052,#62053,#62054,#62055)) ;
#24508=EDGE_LOOP('',(#62056,#62057,#62058,#62059)) ;
#24509=EDGE_LOOP('',(#62060,#62061,#62062,#62063)) ;
#24510=EDGE_LOOP('',(#62064,#62065,#62066,#62067)) ;
#24511=EDGE_LOOP('',(#62068,#62069,#62070,#62071)) ;
#24512=EDGE_LOOP('',(#62072,#62073,#62074,#62075)) ;
#24513=EDGE_LOOP('',(#62076,#62077,#62078,#62079)) ;
#24514=EDGE_LOOP('',(#62080,#62081,#62082,#62083)) ;
#24515=EDGE_LOOP('',(#62084,#62085,#62086,#62087)) ;
#24516=EDGE_LOOP('',(#62088,#62089,#62090,#62091)) ;
#24517=EDGE_LOOP('',(#62092,#62093,#62094,#62095)) ;
#24518=EDGE_LOOP('',(#62096,#62097,#62098,#62099)) ;
#24519=EDGE_LOOP('',(#62100,#62101,#62102,#62103)) ;
#24520=EDGE_LOOP('',(#62104,#62105,#62106,#62107)) ;
#24521=EDGE_LOOP('',(#62108,#62109,#62110,#62111)) ;
#24522=EDGE_LOOP('',(#62112,#62113,#62114,#62115)) ;
#24523=EDGE_LOOP('',(#62116,#62117,#62118,#62119)) ;
#24524=EDGE_LOOP('',(#62120,#62121,#62122,#62123)) ;
#24525=EDGE_LOOP('',(#62124,#62125,#62126,#62127)) ;
#24526=EDGE_LOOP('',(#62128,#62129,#62130,#62131,#62132,#62133,#62134,#62135,
#62136,#62137,#62138,#62139,#62140,#62141,#62142,#62143,#62144,#62145)) ;
#24527=EDGE_LOOP('',(#62146)) ;
#24528=EDGE_LOOP('',(#62147,#62148,#62149,#62150)) ;
#24529=EDGE_LOOP('',(#62151,#62152,#62153,#62154)) ;
#24530=EDGE_LOOP('',(#62155,#62156,#62157,#62158)) ;
#24531=EDGE_LOOP('',(#62159,#62160,#62161,#62162)) ;
#24532=EDGE_LOOP('',(#62163,#62164,#62165,#62166)) ;
#24533=EDGE_LOOP('',(#62167,#62168,#62169,#62170)) ;
#24534=EDGE_LOOP('',(#62171,#62172,#62173,#62174)) ;
#24535=EDGE_LOOP('',(#62175,#62176,#62177,#62178)) ;
#24536=EDGE_LOOP('',(#62179,#62180,#62181,#62182)) ;
#24537=EDGE_LOOP('',(#62183,#62184,#62185,#62186)) ;
#24538=EDGE_LOOP('',(#62187,#62188,#62189,#62190)) ;
#24539=EDGE_LOOP('',(#62191,#62192,#62193,#62194)) ;
#24540=EDGE_LOOP('',(#62195,#62196,#62197,#62198)) ;
#24541=EDGE_LOOP('',(#62199,#62200,#62201,#62202)) ;
#24542=EDGE_LOOP('',(#62203,#62204,#62205,#62206)) ;
#24543=EDGE_LOOP('',(#62207,#62208,#62209,#62210)) ;
#24544=EDGE_LOOP('',(#62211,#62212,#62213,#62214)) ;
#24545=EDGE_LOOP('',(#62215,#62216,#62217,#62218)) ;
#24546=EDGE_LOOP('',(#62219,#62220,#62221,#62222)) ;
#24547=EDGE_LOOP('',(#62223,#62224,#62225,#62226)) ;
#24548=EDGE_LOOP('',(#62227,#62228,#62229,#62230)) ;
#24549=EDGE_LOOP('',(#62231,#62232,#62233,#62234)) ;
#24550=EDGE_LOOP('',(#62235,#62236,#62237,#62238)) ;
#24551=EDGE_LOOP('',(#62239,#62240,#62241,#62242)) ;
#24552=EDGE_LOOP('',(#62243,#62244,#62245,#62246)) ;
#24553=EDGE_LOOP('',(#62247,#62248,#62249,#62250)) ;
#24554=EDGE_LOOP('',(#62251,#62252,#62253,#62254)) ;
#24555=EDGE_LOOP('',(#62255,#62256,#62257,#62258,#62259,#62260,#62261,#62262,
#62263,#62264,#62265,#62266,#62267,#62268,#62269,#62270,#62271,#62272)) ;
#24556=EDGE_LOOP('',(#62273)) ;
#24557=EDGE_LOOP('',(#62274,#62275,#62276,#62277)) ;
#24558=EDGE_LOOP('',(#62278,#62279,#62280,#62281)) ;
#24559=EDGE_LOOP('',(#62282,#62283,#62284,#62285)) ;
#24560=EDGE_LOOP('',(#62286,#62287,#62288,#62289)) ;
#24561=EDGE_LOOP('',(#62290,#62291,#62292,#62293)) ;
#24562=EDGE_LOOP('',(#62294,#62295,#62296,#62297)) ;
#24563=EDGE_LOOP('',(#62298,#62299,#62300,#62301)) ;
#24564=EDGE_LOOP('',(#62302,#62303,#62304,#62305)) ;
#24565=EDGE_LOOP('',(#62306,#62307,#62308,#62309)) ;
#24566=EDGE_LOOP('',(#62310,#62311,#62312,#62313)) ;
#24567=EDGE_LOOP('',(#62314,#62315,#62316,#62317)) ;
#24568=EDGE_LOOP('',(#62318,#62319,#62320,#62321)) ;
#24569=EDGE_LOOP('',(#62322,#62323,#62324,#62325)) ;
#24570=EDGE_LOOP('',(#62326,#62327,#62328,#62329)) ;
#24571=EDGE_LOOP('',(#62330,#62331,#62332,#62333)) ;
#24572=EDGE_LOOP('',(#62334,#62335,#62336,#62337)) ;
#24573=EDGE_LOOP('',(#62338,#62339,#62340,#62341)) ;
#24574=EDGE_LOOP('',(#62342,#62343,#62344,#62345)) ;
#24575=EDGE_LOOP('',(#62346,#62347,#62348,#62349)) ;
#24576=EDGE_LOOP('',(#62350,#62351,#62352,#62353)) ;
#24577=EDGE_LOOP('',(#62354,#62355,#62356,#62357)) ;
#24578=EDGE_LOOP('',(#62358,#62359,#62360,#62361)) ;
#24579=EDGE_LOOP('',(#62362,#62363,#62364,#62365)) ;
#24580=EDGE_LOOP('',(#62366,#62367,#62368,#62369)) ;
#24581=EDGE_LOOP('',(#62370,#62371,#62372,#62373)) ;
#24582=EDGE_LOOP('',(#62374,#62375,#62376,#62377)) ;
#24583=EDGE_LOOP('',(#62378,#62379,#62380,#62381)) ;
#24584=EDGE_LOOP('',(#62382,#62383,#62384,#62385,#62386,#62387,#62388,#62389,
#62390,#62391,#62392,#62393,#62394,#62395,#62396,#62397,#62398,#62399)) ;
#24585=EDGE_LOOP('',(#62400)) ;
#24586=EDGE_LOOP('',(#62401,#62402,#62403,#62404)) ;
#24587=EDGE_LOOP('',(#62405,#62406,#62407,#62408)) ;
#24588=EDGE_LOOP('',(#62409,#62410,#62411,#62412)) ;
#24589=EDGE_LOOP('',(#62413,#62414,#62415,#62416)) ;
#24590=EDGE_LOOP('',(#62417,#62418,#62419,#62420)) ;
#24591=EDGE_LOOP('',(#62421,#62422,#62423,#62424)) ;
#24592=EDGE_LOOP('',(#62425,#62426,#62427,#62428)) ;
#24593=EDGE_LOOP('',(#62429,#62430,#62431,#62432)) ;
#24594=EDGE_LOOP('',(#62433,#62434,#62435,#62436)) ;
#24595=EDGE_LOOP('',(#62437,#62438,#62439,#62440)) ;
#24596=EDGE_LOOP('',(#62441,#62442,#62443,#62444)) ;
#24597=EDGE_LOOP('',(#62445,#62446,#62447,#62448)) ;
#24598=EDGE_LOOP('',(#62449,#62450,#62451,#62452)) ;
#24599=EDGE_LOOP('',(#62453,#62454,#62455,#62456)) ;
#24600=EDGE_LOOP('',(#62457,#62458,#62459,#62460)) ;
#24601=EDGE_LOOP('',(#62461,#62462,#62463,#62464)) ;
#24602=EDGE_LOOP('',(#62465,#62466,#62467,#62468)) ;
#24603=EDGE_LOOP('',(#62469,#62470,#62471,#62472)) ;
#24604=EDGE_LOOP('',(#62473,#62474,#62475,#62476)) ;
#24605=EDGE_LOOP('',(#62477,#62478,#62479,#62480)) ;
#24606=EDGE_LOOP('',(#62481,#62482,#62483,#62484)) ;
#24607=EDGE_LOOP('',(#62485,#62486,#62487,#62488)) ;
#24608=EDGE_LOOP('',(#62489,#62490,#62491,#62492)) ;
#24609=EDGE_LOOP('',(#62493,#62494,#62495,#62496)) ;
#24610=EDGE_LOOP('',(#62497,#62498,#62499,#62500)) ;
#24611=EDGE_LOOP('',(#62501,#62502,#62503,#62504)) ;
#24612=EDGE_LOOP('',(#62505,#62506,#62507,#62508)) ;
#24613=EDGE_LOOP('',(#62509,#62510,#62511,#62512,#62513,#62514,#62515,#62516,
#62517,#62518,#62519,#62520,#62521,#62522,#62523,#62524,#62525,#62526)) ;
#24614=EDGE_LOOP('',(#62527)) ;
#24615=EDGE_LOOP('',(#62528)) ;
#24616=EDGE_LOOP('',(#62529,#62530,#62531,#62532,#62533,#62534,#62535,#62536)) ;
#24617=EDGE_LOOP('',(#62537)) ;
#24618=EDGE_LOOP('',(#62538,#62539,#62540,#62541,#62542,#62543,#62544,#62545)) ;
#24619=EDGE_LOOP('',(#62546)) ;
#24620=EDGE_LOOP('',(#62547,#62548,#62549,#62550,#62551,#62552,#62553,#62554)) ;
#24621=EDGE_LOOP('',(#62555)) ;
#24622=EDGE_LOOP('',(#62556,#62557,#62558,#62559,#62560,#62561,#62562,#62563)) ;
#24623=EDGE_LOOP('',(#62564)) ;
#24624=EDGE_LOOP('',(#62565,#62566,#62567,#62568,#62569,#62570,#62571,#62572)) ;
#24625=EDGE_LOOP('',(#62573)) ;
#24626=EDGE_LOOP('',(#62574,#62575,#62576,#62577,#62578,#62579,#62580,#62581)) ;
#24627=EDGE_LOOP('',(#62582)) ;
#24628=EDGE_LOOP('',(#62583,#62584,#62585,#62586,#62587,#62588,#62589,#62590)) ;
#24629=EDGE_LOOP('',(#62591)) ;
#24630=EDGE_LOOP('',(#62592,#62593,#62594,#62595,#62596,#62597,#62598,#62599)) ;
#24631=EDGE_LOOP('',(#62600)) ;
#24632=EDGE_LOOP('',(#62601,#62602,#62603,#62604,#62605,#62606,#62607,#62608)) ;
#24633=EDGE_LOOP('',(#62609,#62610,#62611,#62612)) ;
#24634=EDGE_LOOP('',(#62613,#62614,#62615,#62616)) ;
#24635=EDGE_LOOP('',(#62617,#62618,#62619)) ;
#24636=EDGE_LOOP('',(#62620,#62621,#62622)) ;
#24637=EDGE_LOOP('',(#62623,#62624,#62625,#62626)) ;
#24638=EDGE_LOOP('',(#62627,#62628,#62629,#62630,#62631,#62632)) ;
#24639=EDGE_LOOP('',(#62633,#62634,#62635,#62636,#62637,#62638,#62639)) ;
#24640=EDGE_LOOP('',(#62640,#62641,#62642,#62643)) ;
#24641=EDGE_LOOP('',(#62644,#62645,#62646,#62647)) ;
#24642=EDGE_LOOP('',(#62648,#62649,#62650,#62651)) ;
#24643=EDGE_LOOP('',(#62652,#62653,#62654,#62655)) ;
#24644=EDGE_LOOP('',(#62656,#62657,#62658)) ;
#24645=EDGE_LOOP('',(#62659,#62660,#62661,#62662)) ;
#24646=EDGE_LOOP('',(#62663,#62664,#62665,#62666)) ;
#24647=EDGE_LOOP('',(#62667,#62668,#62669,#62670)) ;
#24648=EDGE_LOOP('',(#62671,#62672,#62673,#62674)) ;
#24649=EDGE_LOOP('',(#62675,#62676,#62677,#62678)) ;
#24650=EDGE_LOOP('',(#62679,#62680,#62681,#62682)) ;
#24651=EDGE_LOOP('',(#62683,#62684,#62685,#62686)) ;
#24652=EDGE_LOOP('',(#62687,#62688,#62689,#62690)) ;
#24653=EDGE_LOOP('',(#62691,#62692,#62693,#62694)) ;
#24654=EDGE_LOOP('',(#62695,#62696,#62697)) ;
#24655=EDGE_LOOP('',(#62698,#62699,#62700)) ;
#24656=EDGE_LOOP('',(#62701,#62702,#62703,#62704,#62705)) ;
#24657=EDGE_LOOP('',(#62706,#62707,#62708)) ;
#24658=EDGE_LOOP('',(#62709,#62710,#62711)) ;
#24659=EDGE_LOOP('',(#62712,#62713,#62714,#62715)) ;
#24660=EDGE_LOOP('',(#62716,#62717,#62718,#62719)) ;
#24661=EDGE_LOOP('',(#62720,#62721,#62722,#62723)) ;
#24662=EDGE_LOOP('',(#62724,#62725,#62726,#62727)) ;
#24663=EDGE_LOOP('',(#62728,#62729,#62730,#62731)) ;
#24664=EDGE_LOOP('',(#62732,#62733,#62734,#62735)) ;
#24665=EDGE_LOOP('',(#62736,#62737,#62738,#62739)) ;
#24666=EDGE_LOOP('',(#62740,#62741,#62742)) ;
#24667=EDGE_LOOP('',(#62743,#62744,#62745,#62746)) ;
#24668=EDGE_LOOP('',(#62747,#62748,#62749,#62750)) ;
#24669=EDGE_LOOP('',(#62751,#62752,#62753)) ;
#24670=EDGE_LOOP('',(#62754,#62755,#62756,#62757)) ;
#24671=EDGE_LOOP('',(#62758,#62759,#62760,#62761)) ;
#24672=EDGE_LOOP('',(#62762,#62763,#62764,#62765)) ;
#24673=EDGE_LOOP('',(#62766,#62767,#62768,#62769)) ;
#24674=EDGE_LOOP('',(#62770,#62771,#62772,#62773)) ;
#24675=EDGE_LOOP('',(#62774,#62775,#62776,#62777)) ;
#24676=EDGE_LOOP('',(#62778,#62779,#62780,#62781,#62782)) ;
#24677=EDGE_LOOP('',(#62783,#62784,#62785,#62786)) ;
#24678=EDGE_LOOP('',(#62787,#62788,#62789)) ;
#24679=EDGE_LOOP('',(#62790,#62791,#62792,#62793)) ;
#24680=EDGE_LOOP('',(#62794,#62795,#62796,#62797)) ;
#24681=EDGE_LOOP('',(#62798,#62799,#62800)) ;
#24682=EDGE_LOOP('',(#62801,#62802,#62803,#62804)) ;
#24683=EDGE_LOOP('',(#62805,#62806,#62807,#62808)) ;
#24684=EDGE_LOOP('',(#62809,#62810,#62811,#62812)) ;
#24685=EDGE_LOOP('',(#62813,#62814,#62815)) ;
#24686=EDGE_LOOP('',(#62816,#62817,#62818,#62819)) ;
#24687=EDGE_LOOP('',(#62820,#62821,#62822,#62823)) ;
#24688=EDGE_LOOP('',(#62824,#62825,#62826)) ;
#24689=EDGE_LOOP('',(#62827,#62828,#62829)) ;
#24690=EDGE_LOOP('',(#62830,#62831,#62832,#62833)) ;
#24691=EDGE_LOOP('',(#62834,#62835,#62836,#62837)) ;
#24692=EDGE_LOOP('',(#62838,#62839,#62840)) ;
#24693=EDGE_LOOP('',(#62841,#62842,#62843)) ;
#24694=EDGE_LOOP('',(#62844,#62845,#62846,#62847)) ;
#24695=EDGE_LOOP('',(#62848,#62849,#62850,#62851)) ;
#24696=EDGE_LOOP('',(#62852,#62853,#62854)) ;
#24697=EDGE_LOOP('',(#62855,#62856,#62857,#62858)) ;
#24698=EDGE_LOOP('',(#62859,#62860,#62861,#62862)) ;
#24699=EDGE_LOOP('',(#62863,#62864,#62865)) ;
#24700=EDGE_LOOP('',(#62866,#62867,#62868)) ;
#24701=EDGE_LOOP('',(#62869,#62870,#62871,#62872)) ;
#24702=EDGE_LOOP('',(#62873,#62874,#62875,#62876)) ;
#24703=EDGE_LOOP('',(#62877,#62878,#62879,#62880)) ;
#24704=EDGE_LOOP('',(#62881,#62882,#62883,#62884)) ;
#24705=EDGE_LOOP('',(#62885,#62886,#62887,#62888)) ;
#24706=EDGE_LOOP('',(#62889,#62890,#62891,#62892)) ;
#24707=EDGE_LOOP('',(#62893,#62894,#62895)) ;
#24708=EDGE_LOOP('',(#62896,#62897,#62898)) ;
#24709=EDGE_LOOP('',(#62899,#62900,#62901,#62902)) ;
#24710=EDGE_LOOP('',(#62903,#62904,#62905,#62906)) ;
#24711=EDGE_LOOP('',(#62907,#62908,#62909,#62910)) ;
#24712=EDGE_LOOP('',(#62911,#62912,#62913,#62914)) ;
#24713=EDGE_LOOP('',(#62915,#62916,#62917,#62918)) ;
#24714=EDGE_LOOP('',(#62919,#62920,#62921,#62922)) ;
#24715=EDGE_LOOP('',(#62923,#62924,#62925,#62926)) ;
#24716=EDGE_LOOP('',(#62927,#62928,#62929,#62930)) ;
#24717=EDGE_LOOP('',(#62931,#62932,#62933,#62934)) ;
#24718=EDGE_LOOP('',(#62935,#62936,#62937,#62938)) ;
#24719=EDGE_LOOP('',(#62939,#62940,#62941,#62942)) ;
#24720=EDGE_LOOP('',(#62943,#62944,#62945,#62946)) ;
#24721=EDGE_LOOP('',(#62947,#62948,#62949,#62950)) ;
#24722=EDGE_LOOP('',(#62951,#62952,#62953,#62954)) ;
#24723=EDGE_LOOP('',(#62955,#62956,#62957,#62958)) ;
#24724=EDGE_LOOP('',(#62959,#62960,#62961,#62962)) ;
#24725=EDGE_LOOP('',(#62963,#62964,#62965,#62966)) ;
#24726=EDGE_LOOP('',(#62967,#62968,#62969)) ;
#24727=EDGE_LOOP('',(#62970,#62971,#62972,#62973)) ;
#24728=EDGE_LOOP('',(#62974,#62975,#62976,#62977)) ;
#24729=EDGE_LOOP('',(#62978,#62979,#62980,#62981)) ;
#24730=EDGE_LOOP('',(#62982,#62983,#62984)) ;
#24731=EDGE_LOOP('',(#62985,#62986,#62987,#62988)) ;
#24732=EDGE_LOOP('',(#62989,#62990,#62991,#62992)) ;
#24733=EDGE_LOOP('',(#62993,#62994,#62995,#62996)) ;
#24734=EDGE_LOOP('',(#62997,#62998,#62999)) ;
#24735=EDGE_LOOP('',(#63000,#63001,#63002)) ;
#24736=EDGE_LOOP('',(#63003,#63004,#63005,#63006)) ;
#24737=EDGE_LOOP('',(#63007,#63008,#63009,#63010)) ;
#24738=EDGE_LOOP('',(#63011,#63012,#63013,#63014)) ;
#24739=EDGE_LOOP('',(#63015,#63016,#63017,#63018)) ;
#24740=EDGE_LOOP('',(#63019,#63020,#63021,#63022)) ;
#24741=EDGE_LOOP('',(#63023,#63024,#63025,#63026)) ;
#24742=EDGE_LOOP('',(#63027,#63028,#63029,#63030)) ;
#24743=EDGE_LOOP('',(#63031,#63032,#63033,#63034)) ;
#24744=EDGE_LOOP('',(#63035,#63036,#63037,#63038)) ;
#24745=EDGE_LOOP('',(#63039,#63040,#63041,#63042)) ;
#24746=EDGE_LOOP('',(#63043,#63044,#63045,#63046)) ;
#24747=EDGE_LOOP('',(#63047,#63048,#63049,#63050)) ;
#24748=EDGE_LOOP('',(#63051,#63052,#63053,#63054)) ;
#24749=EDGE_LOOP('',(#63055,#63056,#63057,#63058)) ;
#24750=EDGE_LOOP('',(#63059,#63060,#63061,#63062)) ;
#24751=EDGE_LOOP('',(#63063,#63064,#63065,#63066)) ;
#24752=EDGE_LOOP('',(#63067,#63068,#63069,#63070)) ;
#24753=EDGE_LOOP('',(#63071,#63072,#63073)) ;
#24754=EDGE_LOOP('',(#63074,#63075,#63076,#63077)) ;
#24755=EDGE_LOOP('',(#63078,#63079,#63080,#63081)) ;
#24756=EDGE_LOOP('',(#63082,#63083,#63084,#63085)) ;
#24757=EDGE_LOOP('',(#63086,#63087,#63088)) ;
#24758=EDGE_LOOP('',(#63089,#63090,#63091,#63092)) ;
#24759=EDGE_LOOP('',(#63093,#63094,#63095,#63096)) ;
#24760=EDGE_LOOP('',(#63097,#63098,#63099,#63100)) ;
#24761=EDGE_LOOP('',(#63101,#63102,#63103)) ;
#24762=EDGE_LOOP('',(#63104,#63105,#63106)) ;
#24763=EDGE_LOOP('',(#63107,#63108,#63109,#63110)) ;
#24764=EDGE_LOOP('',(#63111,#63112,#63113,#63114)) ;
#24765=EDGE_LOOP('',(#63115,#63116,#63117,#63118)) ;
#24766=EDGE_LOOP('',(#63119,#63120,#63121,#63122)) ;
#24767=EDGE_LOOP('',(#63123,#63124,#63125,#63126)) ;
#24768=EDGE_LOOP('',(#63127,#63128,#63129,#63130)) ;
#24769=EDGE_LOOP('',(#63131,#63132,#63133,#63134)) ;
#24770=EDGE_LOOP('',(#63135,#63136,#63137,#63138)) ;
#24771=EDGE_LOOP('',(#63139,#63140,#63141,#63142)) ;
#24772=EDGE_LOOP('',(#63143,#63144,#63145,#63146)) ;
#24773=EDGE_LOOP('',(#63147,#63148,#63149,#63150)) ;
#24774=EDGE_LOOP('',(#63151,#63152,#63153,#63154)) ;
#24775=EDGE_LOOP('',(#63155,#63156,#63157,#63158)) ;
#24776=EDGE_LOOP('',(#63159,#63160,#63161,#63162)) ;
#24777=EDGE_LOOP('',(#63163,#63164,#63165,#63166)) ;
#24778=EDGE_LOOP('',(#63167,#63168,#63169,#63170)) ;
#24779=EDGE_LOOP('',(#63171,#63172,#63173,#63174)) ;
#24780=EDGE_LOOP('',(#63175,#63176,#63177)) ;
#24781=EDGE_LOOP('',(#63178,#63179,#63180,#63181)) ;
#24782=EDGE_LOOP('',(#63182,#63183,#63184,#63185)) ;
#24783=EDGE_LOOP('',(#63186,#63187,#63188,#63189)) ;
#24784=EDGE_LOOP('',(#63190,#63191,#63192)) ;
#24785=EDGE_LOOP('',(#63193,#63194,#63195,#63196)) ;
#24786=EDGE_LOOP('',(#63197,#63198,#63199,#63200)) ;
#24787=EDGE_LOOP('',(#63201,#63202,#63203,#63204)) ;
#24788=EDGE_LOOP('',(#63205,#63206,#63207)) ;
#24789=EDGE_LOOP('',(#63208,#63209,#63210)) ;
#24790=EDGE_LOOP('',(#63211,#63212,#63213,#63214)) ;
#24791=EDGE_LOOP('',(#63215,#63216,#63217,#63218)) ;
#24792=EDGE_LOOP('',(#63219,#63220,#63221,#63222)) ;
#24793=EDGE_LOOP('',(#63223,#63224,#63225,#63226)) ;
#24794=EDGE_LOOP('',(#63227,#63228,#63229,#63230)) ;
#24795=EDGE_LOOP('',(#63231,#63232,#63233,#63234)) ;
#24796=EDGE_LOOP('',(#63235,#63236,#63237,#63238)) ;
#24797=EDGE_LOOP('',(#63239,#63240,#63241,#63242)) ;
#24798=EDGE_LOOP('',(#63243,#63244,#63245,#63246)) ;
#24799=EDGE_LOOP('',(#63247,#63248,#63249,#63250)) ;
#24800=EDGE_LOOP('',(#63251,#63252,#63253,#63254)) ;
#24801=EDGE_LOOP('',(#63255,#63256,#63257,#63258)) ;
#24802=EDGE_LOOP('',(#63259,#63260,#63261,#63262)) ;
#24803=EDGE_LOOP('',(#63263,#63264,#63265,#63266)) ;
#24804=EDGE_LOOP('',(#63267,#63268,#63269,#63270)) ;
#24805=EDGE_LOOP('',(#63271,#63272,#63273,#63274)) ;
#24806=EDGE_LOOP('',(#63275,#63276,#63277,#63278)) ;
#24807=EDGE_LOOP('',(#63279,#63280,#63281)) ;
#24808=EDGE_LOOP('',(#63282,#63283,#63284,#63285)) ;
#24809=EDGE_LOOP('',(#63286,#63287,#63288,#63289)) ;
#24810=EDGE_LOOP('',(#63290,#63291,#63292,#63293)) ;
#24811=EDGE_LOOP('',(#63294,#63295,#63296)) ;
#24812=EDGE_LOOP('',(#63297,#63298,#63299,#63300)) ;
#24813=EDGE_LOOP('',(#63301,#63302,#63303,#63304)) ;
#24814=EDGE_LOOP('',(#63305,#63306,#63307,#63308)) ;
#24815=EDGE_LOOP('',(#63309,#63310,#63311)) ;
#24816=EDGE_LOOP('',(#63312,#63313,#63314)) ;
#24817=EDGE_LOOP('',(#63315,#63316,#63317,#63318)) ;
#24818=EDGE_LOOP('',(#63319,#63320,#63321,#63322)) ;
#24819=EDGE_LOOP('',(#63323,#63324,#63325,#63326)) ;
#24820=EDGE_LOOP('',(#63327,#63328,#63329,#63330)) ;
#24821=EDGE_LOOP('',(#63331,#63332,#63333,#63334)) ;
#24822=EDGE_LOOP('',(#63335,#63336,#63337,#63338)) ;
#24823=EDGE_LOOP('',(#63339,#63340,#63341,#63342)) ;
#24824=EDGE_LOOP('',(#63343,#63344,#63345,#63346)) ;
#24825=EDGE_LOOP('',(#63347,#63348,#63349,#63350)) ;
#24826=EDGE_LOOP('',(#63351,#63352,#63353,#63354)) ;
#24827=EDGE_LOOP('',(#63355,#63356,#63357,#63358)) ;
#24828=EDGE_LOOP('',(#63359,#63360,#63361,#63362)) ;
#24829=EDGE_LOOP('',(#63363,#63364,#63365,#63366)) ;
#24830=EDGE_LOOP('',(#63367,#63368,#63369,#63370)) ;
#24831=EDGE_LOOP('',(#63371,#63372,#63373,#63374)) ;
#24832=EDGE_LOOP('',(#63375,#63376,#63377,#63378)) ;
#24833=EDGE_LOOP('',(#63379,#63380,#63381,#63382)) ;
#24834=EDGE_LOOP('',(#63383,#63384,#63385)) ;
#24835=EDGE_LOOP('',(#63386,#63387,#63388,#63389)) ;
#24836=EDGE_LOOP('',(#63390,#63391,#63392,#63393)) ;
#24837=EDGE_LOOP('',(#63394,#63395,#63396,#63397)) ;
#24838=EDGE_LOOP('',(#63398,#63399,#63400)) ;
#24839=EDGE_LOOP('',(#63401,#63402,#63403,#63404)) ;
#24840=EDGE_LOOP('',(#63405,#63406,#63407,#63408)) ;
#24841=EDGE_LOOP('',(#63409,#63410,#63411,#63412)) ;
#24842=EDGE_LOOP('',(#63413,#63414,#63415)) ;
#24843=EDGE_LOOP('',(#63416,#63417,#63418)) ;
#24844=EDGE_LOOP('',(#63419,#63420,#63421,#63422)) ;
#24845=EDGE_LOOP('',(#63423,#63424,#63425,#63426)) ;
#24846=EDGE_LOOP('',(#63427,#63428,#63429,#63430)) ;
#24847=EDGE_LOOP('',(#63431,#63432,#63433,#63434)) ;
#24848=EDGE_LOOP('',(#63435,#63436,#63437,#63438)) ;
#24849=EDGE_LOOP('',(#63439,#63440,#63441,#63442)) ;
#24850=EDGE_LOOP('',(#63443,#63444,#63445,#63446)) ;
#24851=EDGE_LOOP('',(#63447,#63448,#63449,#63450)) ;
#24852=EDGE_LOOP('',(#63451,#63452,#63453,#63454)) ;
#24853=EDGE_LOOP('',(#63455,#63456,#63457,#63458)) ;
#24854=EDGE_LOOP('',(#63459,#63460,#63461,#63462)) ;
#24855=EDGE_LOOP('',(#63463,#63464,#63465,#63466)) ;
#24856=EDGE_LOOP('',(#63467,#63468,#63469,#63470)) ;
#24857=EDGE_LOOP('',(#63471,#63472,#63473,#63474)) ;
#24858=EDGE_LOOP('',(#63475,#63476,#63477,#63478)) ;
#24859=EDGE_LOOP('',(#63479,#63480,#63481,#63482)) ;
#24860=EDGE_LOOP('',(#63483,#63484,#63485,#63486)) ;
#24861=EDGE_LOOP('',(#63487,#63488,#63489)) ;
#24862=EDGE_LOOP('',(#63490,#63491,#63492,#63493)) ;
#24863=EDGE_LOOP('',(#63494,#63495,#63496,#63497)) ;
#24864=EDGE_LOOP('',(#63498,#63499,#63500,#63501)) ;
#24865=EDGE_LOOP('',(#63502,#63503,#63504)) ;
#24866=EDGE_LOOP('',(#63505,#63506,#63507,#63508)) ;
#24867=EDGE_LOOP('',(#63509,#63510,#63511,#63512)) ;
#24868=EDGE_LOOP('',(#63513,#63514,#63515,#63516)) ;
#24869=EDGE_LOOP('',(#63517,#63518,#63519)) ;
#24870=EDGE_LOOP('',(#63520,#63521,#63522)) ;
#24871=EDGE_LOOP('',(#63523,#63524,#63525,#63526)) ;
#24872=EDGE_LOOP('',(#63527,#63528,#63529,#63530)) ;
#24873=EDGE_LOOP('',(#63531,#63532,#63533,#63534)) ;
#24874=EDGE_LOOP('',(#63535,#63536,#63537,#63538)) ;
#24875=EDGE_LOOP('',(#63539,#63540,#63541,#63542)) ;
#24876=EDGE_LOOP('',(#63543,#63544,#63545,#63546)) ;
#24877=EDGE_LOOP('',(#63547,#63548,#63549,#63550)) ;
#24878=EDGE_LOOP('',(#63551,#63552,#63553,#63554)) ;
#24879=EDGE_LOOP('',(#63555,#63556,#63557,#63558)) ;
#24880=EDGE_LOOP('',(#63559,#63560,#63561,#63562)) ;
#24881=EDGE_LOOP('',(#63563,#63564,#63565,#63566)) ;
#24882=EDGE_LOOP('',(#63567,#63568,#63569,#63570)) ;
#24883=EDGE_LOOP('',(#63571,#63572,#63573,#63574)) ;
#24884=EDGE_LOOP('',(#63575,#63576,#63577,#63578)) ;
#24885=EDGE_LOOP('',(#63579,#63580,#63581,#63582)) ;
#24886=EDGE_LOOP('',(#63583,#63584,#63585,#63586)) ;
#24887=EDGE_LOOP('',(#63587,#63588,#63589,#63590)) ;
#24888=EDGE_LOOP('',(#63591,#63592,#63593)) ;
#24889=EDGE_LOOP('',(#63594,#63595,#63596,#63597)) ;
#24890=EDGE_LOOP('',(#63598,#63599,#63600,#63601)) ;
#24891=EDGE_LOOP('',(#63602,#63603,#63604,#63605)) ;
#24892=EDGE_LOOP('',(#63606,#63607,#63608)) ;
#24893=EDGE_LOOP('',(#63609,#63610,#63611,#63612)) ;
#24894=EDGE_LOOP('',(#63613,#63614,#63615,#63616)) ;
#24895=EDGE_LOOP('',(#63617,#63618,#63619,#63620)) ;
#24896=EDGE_LOOP('',(#63621,#63622,#63623)) ;
#24897=EDGE_LOOP('',(#63624,#63625,#63626)) ;
#24898=EDGE_LOOP('',(#63627,#63628,#63629,#63630)) ;
#24899=EDGE_LOOP('',(#63631,#63632,#63633,#63634)) ;
#24900=EDGE_LOOP('',(#63635,#63636,#63637,#63638)) ;
#24901=EDGE_LOOP('',(#63639,#63640,#63641,#63642)) ;
#24902=EDGE_LOOP('',(#63643,#63644,#63645,#63646)) ;
#24903=EDGE_LOOP('',(#63647,#63648,#63649,#63650)) ;
#24904=EDGE_LOOP('',(#63651,#63652,#63653,#63654)) ;
#24905=EDGE_LOOP('',(#63655,#63656,#63657,#63658)) ;
#24906=EDGE_LOOP('',(#63659,#63660,#63661,#63662)) ;
#24907=EDGE_LOOP('',(#63663,#63664,#63665,#63666)) ;
#24908=EDGE_LOOP('',(#63667,#63668,#63669,#63670)) ;
#24909=EDGE_LOOP('',(#63671,#63672,#63673,#63674)) ;
#24910=EDGE_LOOP('',(#63675,#63676,#63677,#63678)) ;
#24911=EDGE_LOOP('',(#63679,#63680,#63681,#63682)) ;
#24912=EDGE_LOOP('',(#63683,#63684,#63685,#63686)) ;
#24913=EDGE_LOOP('',(#63687,#63688,#63689,#63690)) ;
#24914=EDGE_LOOP('',(#63691,#63692,#63693,#63694)) ;
#24915=EDGE_LOOP('',(#63695,#63696,#63697)) ;
#24916=EDGE_LOOP('',(#63698,#63699,#63700,#63701)) ;
#24917=EDGE_LOOP('',(#63702,#63703,#63704,#63705)) ;
#24918=EDGE_LOOP('',(#63706,#63707,#63708,#63709)) ;
#24919=EDGE_LOOP('',(#63710,#63711,#63712)) ;
#24920=EDGE_LOOP('',(#63713,#63714,#63715,#63716)) ;
#24921=EDGE_LOOP('',(#63717,#63718,#63719,#63720)) ;
#24922=EDGE_LOOP('',(#63721,#63722,#63723,#63724)) ;
#24923=EDGE_LOOP('',(#63725,#63726,#63727)) ;
#24924=EDGE_LOOP('',(#63728,#63729,#63730)) ;
#24925=EDGE_LOOP('',(#63731,#63732,#63733,#63734)) ;
#24926=EDGE_LOOP('',(#63735,#63736,#63737,#63738)) ;
#24927=EDGE_LOOP('',(#63739,#63740,#63741,#63742)) ;
#24928=EDGE_LOOP('',(#63743,#63744,#63745,#63746)) ;
#24929=EDGE_LOOP('',(#63747,#63748,#63749,#63750)) ;
#24930=EDGE_LOOP('',(#63751,#63752,#63753,#63754)) ;
#24931=EDGE_LOOP('',(#63755,#63756,#63757,#63758)) ;
#24932=EDGE_LOOP('',(#63759,#63760,#63761,#63762)) ;
#24933=EDGE_LOOP('',(#63763,#63764,#63765,#63766)) ;
#24934=EDGE_LOOP('',(#63767,#63768,#63769,#63770)) ;
#24935=EDGE_LOOP('',(#63771,#63772,#63773,#63774)) ;
#24936=EDGE_LOOP('',(#63775,#63776,#63777,#63778)) ;
#24937=EDGE_LOOP('',(#63779,#63780,#63781,#63782)) ;
#24938=EDGE_LOOP('',(#63783,#63784,#63785,#63786)) ;
#24939=EDGE_LOOP('',(#63787,#63788,#63789,#63790)) ;
#24940=EDGE_LOOP('',(#63791,#63792,#63793,#63794)) ;
#24941=EDGE_LOOP('',(#63795,#63796,#63797,#63798)) ;
#24942=EDGE_LOOP('',(#63799,#63800,#63801)) ;
#24943=EDGE_LOOP('',(#63802,#63803,#63804,#63805)) ;
#24944=EDGE_LOOP('',(#63806,#63807,#63808,#63809)) ;
#24945=EDGE_LOOP('',(#63810,#63811,#63812,#63813)) ;
#24946=EDGE_LOOP('',(#63814,#63815,#63816)) ;
#24947=EDGE_LOOP('',(#63817,#63818,#63819,#63820)) ;
#24948=EDGE_LOOP('',(#63821,#63822,#63823,#63824)) ;
#24949=EDGE_LOOP('',(#63825,#63826,#63827,#63828)) ;
#24950=EDGE_LOOP('',(#63829,#63830,#63831,#63832)) ;
#24951=EDGE_LOOP('',(#63833,#63834,#63835)) ;
#24952=EDGE_LOOP('',(#63836,#63837,#63838)) ;
#24953=EDGE_LOOP('',(#63839,#63840,#63841,#63842)) ;
#24954=EDGE_LOOP('',(#63843,#63844,#63845,#63846,#63847,#63848)) ;
#24955=EDGE_LOOP('',(#63849,#63850,#63851,#63852,#63853,#63854,#63855)) ;
#24956=EDGE_LOOP('',(#63856,#63857,#63858,#63859)) ;
#24957=EDGE_LOOP('',(#63860,#63861,#63862,#63863)) ;
#24958=EDGE_LOOP('',(#63864,#63865,#63866,#63867)) ;
#24959=EDGE_LOOP('',(#63868,#63869,#63870,#63871)) ;
#24960=EDGE_LOOP('',(#63872,#63873,#63874)) ;
#24961=EDGE_LOOP('',(#63875,#63876,#63877,#63878)) ;
#24962=EDGE_LOOP('',(#63879,#63880,#63881,#63882)) ;
#24963=EDGE_LOOP('',(#63883,#63884,#63885,#63886)) ;
#24964=EDGE_LOOP('',(#63887,#63888,#63889,#63890)) ;
#24965=EDGE_LOOP('',(#63891,#63892,#63893,#63894)) ;
#24966=EDGE_LOOP('',(#63895,#63896,#63897,#63898)) ;
#24967=EDGE_LOOP('',(#63899,#63900,#63901,#63902)) ;
#24968=EDGE_LOOP('',(#63903,#63904,#63905,#63906)) ;
#24969=EDGE_LOOP('',(#63907,#63908,#63909,#63910)) ;
#24970=EDGE_LOOP('',(#63911,#63912,#63913)) ;
#24971=EDGE_LOOP('',(#63914,#63915,#63916)) ;
#24972=EDGE_LOOP('',(#63917,#63918,#63919,#63920,#63921)) ;
#24973=EDGE_LOOP('',(#63922,#63923,#63924)) ;
#24974=EDGE_LOOP('',(#63925,#63926,#63927)) ;
#24975=EDGE_LOOP('',(#63928,#63929,#63930,#63931)) ;
#24976=EDGE_LOOP('',(#63932,#63933,#63934,#63935)) ;
#24977=EDGE_LOOP('',(#63936,#63937,#63938,#63939)) ;
#24978=EDGE_LOOP('',(#63940,#63941,#63942,#63943)) ;
#24979=EDGE_LOOP('',(#63944,#63945,#63946,#63947)) ;
#24980=EDGE_LOOP('',(#63948,#63949,#63950,#63951)) ;
#24981=EDGE_LOOP('',(#63952,#63953,#63954,#63955)) ;
#24982=EDGE_LOOP('',(#63956,#63957,#63958)) ;
#24983=EDGE_LOOP('',(#63959,#63960,#63961,#63962)) ;
#24984=EDGE_LOOP('',(#63963,#63964,#63965,#63966)) ;
#24985=EDGE_LOOP('',(#63967,#63968,#63969)) ;
#24986=EDGE_LOOP('',(#63970,#63971,#63972,#63973)) ;
#24987=EDGE_LOOP('',(#63974,#63975,#63976,#63977)) ;
#24988=EDGE_LOOP('',(#63978,#63979,#63980,#63981)) ;
#24989=EDGE_LOOP('',(#63982,#63983,#63984,#63985)) ;
#24990=EDGE_LOOP('',(#63986,#63987,#63988,#63989)) ;
#24991=EDGE_LOOP('',(#63990,#63991,#63992,#63993)) ;
#24992=EDGE_LOOP('',(#63994,#63995,#63996,#63997,#63998)) ;
#24993=EDGE_LOOP('',(#63999,#64000,#64001,#64002)) ;
#24994=EDGE_LOOP('',(#64003,#64004,#64005)) ;
#24995=EDGE_LOOP('',(#64006,#64007,#64008,#64009)) ;
#24996=EDGE_LOOP('',(#64010,#64011,#64012,#64013)) ;
#24997=EDGE_LOOP('',(#64014,#64015,#64016)) ;
#24998=EDGE_LOOP('',(#64017,#64018,#64019,#64020)) ;
#24999=EDGE_LOOP('',(#64021,#64022,#64023,#64024)) ;
#25000=EDGE_LOOP('',(#64025,#64026,#64027,#64028)) ;
#25001=EDGE_LOOP('',(#64029,#64030,#64031)) ;
#25002=EDGE_LOOP('',(#64032,#64033,#64034,#64035)) ;
#25003=EDGE_LOOP('',(#64036,#64037,#64038,#64039)) ;
#25004=EDGE_LOOP('',(#64040,#64041,#64042)) ;
#25005=EDGE_LOOP('',(#64043,#64044,#64045)) ;
#25006=EDGE_LOOP('',(#64046,#64047,#64048,#64049)) ;
#25007=EDGE_LOOP('',(#64050,#64051,#64052,#64053)) ;
#25008=EDGE_LOOP('',(#64054,#64055,#64056)) ;
#25009=EDGE_LOOP('',(#64057,#64058,#64059)) ;
#25010=EDGE_LOOP('',(#64060,#64061,#64062,#64063)) ;
#25011=EDGE_LOOP('',(#64064,#64065,#64066,#64067)) ;
#25012=EDGE_LOOP('',(#64068,#64069,#64070)) ;
#25013=EDGE_LOOP('',(#64071,#64072,#64073,#64074)) ;
#25014=EDGE_LOOP('',(#64075,#64076,#64077,#64078)) ;
#25015=EDGE_LOOP('',(#64079,#64080,#64081)) ;
#25016=EDGE_LOOP('',(#64082,#64083,#64084)) ;
#25017=EDGE_LOOP('',(#64085,#64086,#64087,#64088)) ;
#25018=EDGE_LOOP('',(#64089,#64090,#64091,#64092)) ;
#25019=EDGE_LOOP('',(#64093,#64094,#64095,#64096)) ;
#25020=EDGE_LOOP('',(#64097,#64098,#64099,#64100)) ;
#25021=EDGE_LOOP('',(#64101,#64102,#64103,#64104)) ;
#25022=EDGE_LOOP('',(#64105,#64106,#64107,#64108)) ;
#25023=EDGE_LOOP('',(#64109,#64110,#64111,#64112)) ;
#25024=EDGE_LOOP('',(#64113,#64114,#64115)) ;
#25025=EDGE_LOOP('',(#64116,#64117,#64118)) ;
#25026=EDGE_LOOP('',(#64119,#64120,#64121,#64122)) ;
#25027=EDGE_LOOP('',(#64123,#64124,#64125,#64126,#64127,#64128)) ;
#25028=EDGE_LOOP('',(#64129,#64130,#64131,#64132,#64133,#64134,#64135)) ;
#25029=EDGE_LOOP('',(#64136,#64137,#64138,#64139)) ;
#25030=EDGE_LOOP('',(#64140,#64141,#64142,#64143)) ;
#25031=EDGE_LOOP('',(#64144,#64145,#64146,#64147)) ;
#25032=EDGE_LOOP('',(#64148,#64149,#64150,#64151)) ;
#25033=EDGE_LOOP('',(#64152,#64153,#64154)) ;
#25034=EDGE_LOOP('',(#64155,#64156,#64157,#64158)) ;
#25035=EDGE_LOOP('',(#64159,#64160,#64161,#64162)) ;
#25036=EDGE_LOOP('',(#64163,#64164,#64165,#64166)) ;
#25037=EDGE_LOOP('',(#64167,#64168,#64169,#64170)) ;
#25038=EDGE_LOOP('',(#64171,#64172,#64173,#64174)) ;
#25039=EDGE_LOOP('',(#64175,#64176,#64177,#64178)) ;
#25040=EDGE_LOOP('',(#64179,#64180,#64181,#64182)) ;
#25041=EDGE_LOOP('',(#64183,#64184,#64185,#64186)) ;
#25042=EDGE_LOOP('',(#64187,#64188,#64189,#64190)) ;
#25043=EDGE_LOOP('',(#64191,#64192,#64193)) ;
#25044=EDGE_LOOP('',(#64194,#64195,#64196)) ;
#25045=EDGE_LOOP('',(#64197,#64198,#64199,#64200,#64201)) ;
#25046=EDGE_LOOP('',(#64202,#64203,#64204)) ;
#25047=EDGE_LOOP('',(#64205,#64206,#64207)) ;
#25048=EDGE_LOOP('',(#64208,#64209,#64210,#64211)) ;
#25049=EDGE_LOOP('',(#64212,#64213,#64214,#64215)) ;
#25050=EDGE_LOOP('',(#64216,#64217,#64218,#64219)) ;
#25051=EDGE_LOOP('',(#64220,#64221,#64222,#64223)) ;
#25052=EDGE_LOOP('',(#64224,#64225,#64226,#64227)) ;
#25053=EDGE_LOOP('',(#64228,#64229,#64230,#64231)) ;
#25054=EDGE_LOOP('',(#64232,#64233,#64234,#64235)) ;
#25055=EDGE_LOOP('',(#64236,#64237,#64238)) ;
#25056=EDGE_LOOP('',(#64239,#64240,#64241,#64242)) ;
#25057=EDGE_LOOP('',(#64243,#64244,#64245,#64246)) ;
#25058=EDGE_LOOP('',(#64247,#64248,#64249)) ;
#25059=EDGE_LOOP('',(#64250,#64251,#64252,#64253)) ;
#25060=EDGE_LOOP('',(#64254,#64255,#64256,#64257)) ;
#25061=EDGE_LOOP('',(#64258,#64259,#64260,#64261)) ;
#25062=EDGE_LOOP('',(#64262,#64263,#64264,#64265)) ;
#25063=EDGE_LOOP('',(#64266,#64267,#64268,#64269)) ;
#25064=EDGE_LOOP('',(#64270,#64271,#64272,#64273)) ;
#25065=EDGE_LOOP('',(#64274,#64275,#64276,#64277,#64278)) ;
#25066=EDGE_LOOP('',(#64279,#64280,#64281,#64282)) ;
#25067=EDGE_LOOP('',(#64283,#64284,#64285)) ;
#25068=EDGE_LOOP('',(#64286,#64287,#64288,#64289)) ;
#25069=EDGE_LOOP('',(#64290,#64291,#64292,#64293)) ;
#25070=EDGE_LOOP('',(#64294,#64295,#64296)) ;
#25071=EDGE_LOOP('',(#64297,#64298,#64299,#64300)) ;
#25072=EDGE_LOOP('',(#64301,#64302,#64303,#64304)) ;
#25073=EDGE_LOOP('',(#64305,#64306,#64307,#64308)) ;
#25074=EDGE_LOOP('',(#64309,#64310,#64311)) ;
#25075=EDGE_LOOP('',(#64312,#64313,#64314,#64315)) ;
#25076=EDGE_LOOP('',(#64316,#64317,#64318,#64319)) ;
#25077=EDGE_LOOP('',(#64320,#64321,#64322)) ;
#25078=EDGE_LOOP('',(#64323,#64324,#64325)) ;
#25079=EDGE_LOOP('',(#64326,#64327,#64328,#64329)) ;
#25080=EDGE_LOOP('',(#64330,#64331,#64332,#64333)) ;
#25081=EDGE_LOOP('',(#64334,#64335,#64336)) ;
#25082=EDGE_LOOP('',(#64337,#64338,#64339)) ;
#25083=EDGE_LOOP('',(#64340,#64341,#64342,#64343)) ;
#25084=EDGE_LOOP('',(#64344,#64345,#64346,#64347)) ;
#25085=EDGE_LOOP('',(#64348,#64349,#64350)) ;
#25086=EDGE_LOOP('',(#64351,#64352,#64353,#64354)) ;
#25087=EDGE_LOOP('',(#64355,#64356,#64357,#64358)) ;
#25088=EDGE_LOOP('',(#64359,#64360,#64361)) ;
#25089=EDGE_LOOP('',(#64362,#64363,#64364)) ;
#25090=EDGE_LOOP('',(#64365,#64366,#64367,#64368)) ;
#25091=EDGE_LOOP('',(#64369,#64370,#64371,#64372)) ;
#25092=EDGE_LOOP('',(#64373,#64374,#64375,#64376)) ;
#25093=EDGE_LOOP('',(#64377,#64378,#64379,#64380)) ;
#25094=EDGE_LOOP('',(#64381,#64382,#64383,#64384)) ;
#25095=EDGE_LOOP('',(#64385,#64386,#64387,#64388)) ;
#25096=EDGE_LOOP('',(#64389,#64390,#64391,#64392)) ;
#25097=EDGE_LOOP('',(#64393,#64394,#64395)) ;
#25098=EDGE_LOOP('',(#64396,#64397,#64398)) ;
#25099=EDGE_LOOP('',(#64399,#64400,#64401,#64402)) ;
#25100=EDGE_LOOP('',(#64403,#64404,#64405,#64406,#64407,#64408)) ;
#25101=EDGE_LOOP('',(#64409,#64410,#64411,#64412,#64413,#64414,#64415)) ;
#25102=EDGE_LOOP('',(#64416,#64417,#64418,#64419)) ;
#25103=EDGE_LOOP('',(#64420,#64421,#64422,#64423)) ;
#25104=EDGE_LOOP('',(#64424,#64425,#64426,#64427)) ;
#25105=EDGE_LOOP('',(#64428,#64429,#64430,#64431)) ;
#25106=EDGE_LOOP('',(#64432,#64433,#64434)) ;
#25107=EDGE_LOOP('',(#64435,#64436,#64437,#64438)) ;
#25108=EDGE_LOOP('',(#64439,#64440,#64441,#64442)) ;
#25109=EDGE_LOOP('',(#64443,#64444,#64445,#64446)) ;
#25110=EDGE_LOOP('',(#64447,#64448,#64449,#64450)) ;
#25111=EDGE_LOOP('',(#64451,#64452,#64453,#64454)) ;
#25112=EDGE_LOOP('',(#64455,#64456,#64457,#64458)) ;
#25113=EDGE_LOOP('',(#64459,#64460,#64461,#64462)) ;
#25114=EDGE_LOOP('',(#64463,#64464,#64465,#64466)) ;
#25115=EDGE_LOOP('',(#64467,#64468,#64469,#64470)) ;
#25116=EDGE_LOOP('',(#64471,#64472,#64473)) ;
#25117=EDGE_LOOP('',(#64474,#64475,#64476)) ;
#25118=EDGE_LOOP('',(#64477,#64478,#64479,#64480,#64481)) ;
#25119=EDGE_LOOP('',(#64482,#64483,#64484)) ;
#25120=EDGE_LOOP('',(#64485,#64486,#64487)) ;
#25121=EDGE_LOOP('',(#64488,#64489,#64490,#64491)) ;
#25122=EDGE_LOOP('',(#64492,#64493,#64494,#64495)) ;
#25123=EDGE_LOOP('',(#64496,#64497,#64498,#64499)) ;
#25124=EDGE_LOOP('',(#64500,#64501,#64502,#64503)) ;
#25125=EDGE_LOOP('',(#64504,#64505,#64506,#64507)) ;
#25126=EDGE_LOOP('',(#64508,#64509,#64510,#64511)) ;
#25127=EDGE_LOOP('',(#64512,#64513,#64514,#64515)) ;
#25128=EDGE_LOOP('',(#64516,#64517,#64518)) ;
#25129=EDGE_LOOP('',(#64519,#64520,#64521,#64522)) ;
#25130=EDGE_LOOP('',(#64523,#64524,#64525,#64526)) ;
#25131=EDGE_LOOP('',(#64527,#64528,#64529)) ;
#25132=EDGE_LOOP('',(#64530,#64531,#64532,#64533)) ;
#25133=EDGE_LOOP('',(#64534,#64535,#64536,#64537)) ;
#25134=EDGE_LOOP('',(#64538,#64539,#64540,#64541)) ;
#25135=EDGE_LOOP('',(#64542,#64543,#64544,#64545)) ;
#25136=EDGE_LOOP('',(#64546,#64547,#64548,#64549)) ;
#25137=EDGE_LOOP('',(#64550,#64551,#64552,#64553)) ;
#25138=EDGE_LOOP('',(#64554,#64555,#64556,#64557,#64558)) ;
#25139=EDGE_LOOP('',(#64559,#64560,#64561,#64562)) ;
#25140=EDGE_LOOP('',(#64563,#64564,#64565)) ;
#25141=EDGE_LOOP('',(#64566,#64567,#64568,#64569)) ;
#25142=EDGE_LOOP('',(#64570,#64571,#64572,#64573)) ;
#25143=EDGE_LOOP('',(#64574,#64575,#64576)) ;
#25144=EDGE_LOOP('',(#64577,#64578,#64579,#64580)) ;
#25145=EDGE_LOOP('',(#64581,#64582,#64583,#64584)) ;
#25146=EDGE_LOOP('',(#64585,#64586,#64587,#64588)) ;
#25147=EDGE_LOOP('',(#64589,#64590,#64591)) ;
#25148=EDGE_LOOP('',(#64592,#64593,#64594,#64595)) ;
#25149=EDGE_LOOP('',(#64596,#64597,#64598,#64599)) ;
#25150=EDGE_LOOP('',(#64600,#64601,#64602)) ;
#25151=EDGE_LOOP('',(#64603,#64604,#64605)) ;
#25152=EDGE_LOOP('',(#64606,#64607,#64608,#64609)) ;
#25153=EDGE_LOOP('',(#64610,#64611,#64612,#64613)) ;
#25154=EDGE_LOOP('',(#64614,#64615,#64616)) ;
#25155=EDGE_LOOP('',(#64617,#64618,#64619)) ;
#25156=EDGE_LOOP('',(#64620,#64621,#64622,#64623)) ;
#25157=EDGE_LOOP('',(#64624,#64625,#64626,#64627)) ;
#25158=EDGE_LOOP('',(#64628,#64629,#64630)) ;
#25159=EDGE_LOOP('',(#64631,#64632,#64633,#64634)) ;
#25160=EDGE_LOOP('',(#64635,#64636,#64637,#64638)) ;
#25161=EDGE_LOOP('',(#64639,#64640,#64641)) ;
#25162=EDGE_LOOP('',(#64642,#64643,#64644)) ;
#25163=EDGE_LOOP('',(#64645,#64646,#64647,#64648)) ;
#25164=EDGE_LOOP('',(#64649,#64650,#64651,#64652)) ;
#25165=EDGE_LOOP('',(#64653,#64654,#64655,#64656)) ;
#25166=EDGE_LOOP('',(#64657,#64658,#64659,#64660)) ;
#25167=EDGE_LOOP('',(#64661,#64662,#64663,#64664)) ;
#25168=EDGE_LOOP('',(#64665,#64666,#64667,#64668)) ;
#25169=EDGE_LOOP('',(#64669,#64670,#64671,#64672)) ;
#25170=EDGE_LOOP('',(#64673,#64674,#64675)) ;
#25171=EDGE_LOOP('',(#64676,#64677,#64678)) ;
#25172=EDGE_LOOP('',(#64679,#64680,#64681,#64682)) ;
#25173=EDGE_LOOP('',(#64683,#64684,#64685,#64686,#64687,#64688)) ;
#25174=EDGE_LOOP('',(#64689,#64690,#64691,#64692,#64693,#64694,#64695)) ;
#25175=EDGE_LOOP('',(#64696,#64697,#64698,#64699)) ;
#25176=EDGE_LOOP('',(#64700,#64701,#64702,#64703)) ;
#25177=EDGE_LOOP('',(#64704,#64705,#64706,#64707)) ;
#25178=EDGE_LOOP('',(#64708,#64709,#64710,#64711)) ;
#25179=EDGE_LOOP('',(#64712,#64713,#64714)) ;
#25180=EDGE_LOOP('',(#64715,#64716,#64717,#64718)) ;
#25181=EDGE_LOOP('',(#64719,#64720,#64721,#64722)) ;
#25182=EDGE_LOOP('',(#64723,#64724,#64725,#64726)) ;
#25183=EDGE_LOOP('',(#64727,#64728,#64729,#64730)) ;
#25184=EDGE_LOOP('',(#64731,#64732,#64733,#64734)) ;
#25185=EDGE_LOOP('',(#64735,#64736,#64737,#64738)) ;
#25186=EDGE_LOOP('',(#64739,#64740,#64741,#64742)) ;
#25187=EDGE_LOOP('',(#64743,#64744,#64745,#64746)) ;
#25188=EDGE_LOOP('',(#64747,#64748,#64749,#64750)) ;
#25189=EDGE_LOOP('',(#64751,#64752,#64753)) ;
#25190=EDGE_LOOP('',(#64754,#64755,#64756)) ;
#25191=EDGE_LOOP('',(#64757,#64758,#64759,#64760,#64761)) ;
#25192=EDGE_LOOP('',(#64762,#64763,#64764)) ;
#25193=EDGE_LOOP('',(#64765,#64766,#64767)) ;
#25194=EDGE_LOOP('',(#64768,#64769,#64770,#64771)) ;
#25195=EDGE_LOOP('',(#64772,#64773,#64774,#64775)) ;
#25196=EDGE_LOOP('',(#64776,#64777,#64778,#64779)) ;
#25197=EDGE_LOOP('',(#64780,#64781,#64782,#64783)) ;
#25198=EDGE_LOOP('',(#64784,#64785,#64786,#64787)) ;
#25199=EDGE_LOOP('',(#64788,#64789,#64790,#64791)) ;
#25200=EDGE_LOOP('',(#64792,#64793,#64794,#64795)) ;
#25201=EDGE_LOOP('',(#64796,#64797,#64798)) ;
#25202=EDGE_LOOP('',(#64799,#64800,#64801,#64802)) ;
#25203=EDGE_LOOP('',(#64803,#64804,#64805,#64806)) ;
#25204=EDGE_LOOP('',(#64807,#64808,#64809)) ;
#25205=EDGE_LOOP('',(#64810,#64811,#64812,#64813)) ;
#25206=EDGE_LOOP('',(#64814,#64815,#64816,#64817)) ;
#25207=EDGE_LOOP('',(#64818,#64819,#64820,#64821)) ;
#25208=EDGE_LOOP('',(#64822,#64823,#64824,#64825)) ;
#25209=EDGE_LOOP('',(#64826,#64827,#64828,#64829)) ;
#25210=EDGE_LOOP('',(#64830,#64831,#64832,#64833)) ;
#25211=EDGE_LOOP('',(#64834,#64835,#64836,#64837,#64838)) ;
#25212=EDGE_LOOP('',(#64839,#64840,#64841,#64842)) ;
#25213=EDGE_LOOP('',(#64843,#64844,#64845)) ;
#25214=EDGE_LOOP('',(#64846,#64847,#64848,#64849)) ;
#25215=EDGE_LOOP('',(#64850,#64851,#64852,#64853)) ;
#25216=EDGE_LOOP('',(#64854,#64855,#64856)) ;
#25217=EDGE_LOOP('',(#64857,#64858,#64859,#64860)) ;
#25218=EDGE_LOOP('',(#64861,#64862,#64863,#64864)) ;
#25219=EDGE_LOOP('',(#64865,#64866,#64867,#64868)) ;
#25220=EDGE_LOOP('',(#64869,#64870,#64871)) ;
#25221=EDGE_LOOP('',(#64872,#64873,#64874,#64875)) ;
#25222=EDGE_LOOP('',(#64876,#64877,#64878,#64879)) ;
#25223=EDGE_LOOP('',(#64880,#64881,#64882)) ;
#25224=EDGE_LOOP('',(#64883,#64884,#64885)) ;
#25225=EDGE_LOOP('',(#64886,#64887,#64888,#64889)) ;
#25226=EDGE_LOOP('',(#64890,#64891,#64892,#64893)) ;
#25227=EDGE_LOOP('',(#64894,#64895,#64896)) ;
#25228=EDGE_LOOP('',(#64897,#64898,#64899)) ;
#25229=EDGE_LOOP('',(#64900,#64901,#64902,#64903)) ;
#25230=EDGE_LOOP('',(#64904,#64905,#64906,#64907)) ;
#25231=EDGE_LOOP('',(#64908,#64909,#64910)) ;
#25232=EDGE_LOOP('',(#64911,#64912,#64913,#64914)) ;
#25233=EDGE_LOOP('',(#64915,#64916,#64917,#64918)) ;
#25234=EDGE_LOOP('',(#64919,#64920,#64921)) ;
#25235=EDGE_LOOP('',(#64922,#64923,#64924)) ;
#25236=EDGE_LOOP('',(#64925,#64926,#64927,#64928)) ;
#25237=EDGE_LOOP('',(#64929,#64930,#64931,#64932)) ;
#25238=EDGE_LOOP('',(#64933,#64934,#64935,#64936)) ;
#25239=EDGE_LOOP('',(#64937,#64938,#64939,#64940)) ;
#25240=EDGE_LOOP('',(#64941,#64942,#64943,#64944)) ;
#25241=EDGE_LOOP('',(#64945,#64946,#64947,#64948)) ;
#25242=EDGE_LOOP('',(#64949,#64950,#64951,#64952)) ;
#25243=EDGE_LOOP('',(#64953,#64954,#64955)) ;
#25244=EDGE_LOOP('',(#64956,#64957,#64958)) ;
#25245=EDGE_LOOP('',(#64959,#64960,#64961,#64962)) ;
#25246=EDGE_LOOP('',(#64963,#64964,#64965,#64966,#64967,#64968)) ;
#25247=EDGE_LOOP('',(#64969,#64970,#64971,#64972,#64973,#64974,#64975)) ;
#25248=EDGE_LOOP('',(#64976,#64977,#64978,#64979)) ;
#25249=EDGE_LOOP('',(#64980,#64981,#64982,#64983)) ;
#25250=EDGE_LOOP('',(#64984,#64985,#64986,#64987)) ;
#25251=EDGE_LOOP('',(#64988,#64989,#64990,#64991)) ;
#25252=EDGE_LOOP('',(#64992,#64993,#64994)) ;
#25253=EDGE_LOOP('',(#64995,#64996,#64997,#64998)) ;
#25254=EDGE_LOOP('',(#64999,#65000,#65001,#65002)) ;
#25255=EDGE_LOOP('',(#65003,#65004,#65005,#65006)) ;
#25256=EDGE_LOOP('',(#65007,#65008,#65009,#65010)) ;
#25257=EDGE_LOOP('',(#65011,#65012,#65013,#65014)) ;
#25258=EDGE_LOOP('',(#65015,#65016,#65017,#65018)) ;
#25259=EDGE_LOOP('',(#65019,#65020,#65021,#65022)) ;
#25260=EDGE_LOOP('',(#65023,#65024,#65025,#65026)) ;
#25261=EDGE_LOOP('',(#65027,#65028,#65029,#65030)) ;
#25262=EDGE_LOOP('',(#65031,#65032,#65033)) ;
#25263=EDGE_LOOP('',(#65034,#65035,#65036)) ;
#25264=EDGE_LOOP('',(#65037,#65038,#65039,#65040,#65041)) ;
#25265=EDGE_LOOP('',(#65042,#65043,#65044)) ;
#25266=EDGE_LOOP('',(#65045,#65046,#65047)) ;
#25267=EDGE_LOOP('',(#65048,#65049,#65050,#65051)) ;
#25268=EDGE_LOOP('',(#65052,#65053,#65054,#65055)) ;
#25269=EDGE_LOOP('',(#65056,#65057,#65058,#65059)) ;
#25270=EDGE_LOOP('',(#65060,#65061,#65062,#65063)) ;
#25271=EDGE_LOOP('',(#65064,#65065,#65066,#65067)) ;
#25272=EDGE_LOOP('',(#65068,#65069,#65070,#65071)) ;
#25273=EDGE_LOOP('',(#65072,#65073,#65074,#65075)) ;
#25274=EDGE_LOOP('',(#65076,#65077,#65078)) ;
#25275=EDGE_LOOP('',(#65079,#65080,#65081,#65082)) ;
#25276=EDGE_LOOP('',(#65083,#65084,#65085,#65086)) ;
#25277=EDGE_LOOP('',(#65087,#65088,#65089)) ;
#25278=EDGE_LOOP('',(#65090,#65091,#65092,#65093)) ;
#25279=EDGE_LOOP('',(#65094,#65095,#65096,#65097)) ;
#25280=EDGE_LOOP('',(#65098,#65099,#65100,#65101)) ;
#25281=EDGE_LOOP('',(#65102,#65103,#65104,#65105)) ;
#25282=EDGE_LOOP('',(#65106,#65107,#65108,#65109)) ;
#25283=EDGE_LOOP('',(#65110,#65111,#65112,#65113)) ;
#25284=EDGE_LOOP('',(#65114,#65115,#65116,#65117,#65118)) ;
#25285=EDGE_LOOP('',(#65119,#65120,#65121,#65122)) ;
#25286=EDGE_LOOP('',(#65123,#65124,#65125)) ;
#25287=EDGE_LOOP('',(#65126,#65127,#65128,#65129)) ;
#25288=EDGE_LOOP('',(#65130,#65131,#65132,#65133)) ;
#25289=EDGE_LOOP('',(#65134,#65135,#65136)) ;
#25290=EDGE_LOOP('',(#65137,#65138,#65139,#65140)) ;
#25291=EDGE_LOOP('',(#65141,#65142,#65143,#65144)) ;
#25292=EDGE_LOOP('',(#65145,#65146,#65147,#65148)) ;
#25293=EDGE_LOOP('',(#65149,#65150,#65151)) ;
#25294=EDGE_LOOP('',(#65152,#65153,#65154,#65155)) ;
#25295=EDGE_LOOP('',(#65156,#65157,#65158,#65159)) ;
#25296=EDGE_LOOP('',(#65160,#65161,#65162)) ;
#25297=EDGE_LOOP('',(#65163,#65164,#65165)) ;
#25298=EDGE_LOOP('',(#65166,#65167,#65168,#65169)) ;
#25299=EDGE_LOOP('',(#65170,#65171,#65172,#65173)) ;
#25300=EDGE_LOOP('',(#65174,#65175,#65176)) ;
#25301=EDGE_LOOP('',(#65177,#65178,#65179)) ;
#25302=EDGE_LOOP('',(#65180,#65181,#65182,#65183)) ;
#25303=EDGE_LOOP('',(#65184,#65185,#65186,#65187)) ;
#25304=EDGE_LOOP('',(#65188,#65189,#65190)) ;
#25305=EDGE_LOOP('',(#65191,#65192,#65193,#65194)) ;
#25306=EDGE_LOOP('',(#65195,#65196,#65197,#65198)) ;
#25307=EDGE_LOOP('',(#65199,#65200,#65201)) ;
#25308=EDGE_LOOP('',(#65202,#65203,#65204)) ;
#25309=EDGE_LOOP('',(#65205,#65206,#65207,#65208)) ;
#25310=EDGE_LOOP('',(#65209,#65210,#65211,#65212)) ;
#25311=EDGE_LOOP('',(#65213,#65214,#65215,#65216)) ;
#25312=EDGE_LOOP('',(#65217,#65218,#65219,#65220)) ;
#25313=EDGE_LOOP('',(#65221,#65222,#65223,#65224)) ;
#25314=EDGE_LOOP('',(#65225,#65226,#65227,#65228)) ;
#25315=EDGE_LOOP('',(#65229,#65230,#65231,#65232)) ;
#25316=EDGE_LOOP('',(#65233,#65234,#65235)) ;
#25317=EDGE_LOOP('',(#65236,#65237,#65238)) ;
#25318=EDGE_LOOP('',(#65239,#65240,#65241,#65242)) ;
#25319=EDGE_LOOP('',(#65243,#65244,#65245,#65246,#65247,#65248)) ;
#25320=EDGE_LOOP('',(#65249,#65250,#65251,#65252,#65253,#65254,#65255)) ;
#25321=EDGE_LOOP('',(#65256,#65257,#65258,#65259)) ;
#25322=EDGE_LOOP('',(#65260,#65261,#65262,#65263)) ;
#25323=EDGE_LOOP('',(#65264,#65265,#65266,#65267)) ;
#25324=EDGE_LOOP('',(#65268,#65269,#65270,#65271)) ;
#25325=EDGE_LOOP('',(#65272,#65273,#65274)) ;
#25326=EDGE_LOOP('',(#65275,#65276,#65277,#65278)) ;
#25327=EDGE_LOOP('',(#65279,#65280,#65281,#65282)) ;
#25328=EDGE_LOOP('',(#65283,#65284,#65285,#65286)) ;
#25329=EDGE_LOOP('',(#65287,#65288,#65289,#65290)) ;
#25330=EDGE_LOOP('',(#65291,#65292,#65293,#65294)) ;
#25331=EDGE_LOOP('',(#65295,#65296,#65297,#65298)) ;
#25332=EDGE_LOOP('',(#65299,#65300,#65301,#65302)) ;
#25333=EDGE_LOOP('',(#65303,#65304,#65305,#65306)) ;
#25334=EDGE_LOOP('',(#65307,#65308,#65309,#65310)) ;
#25335=EDGE_LOOP('',(#65311,#65312,#65313)) ;
#25336=EDGE_LOOP('',(#65314,#65315,#65316)) ;
#25337=EDGE_LOOP('',(#65317,#65318,#65319,#65320,#65321)) ;
#25338=EDGE_LOOP('',(#65322,#65323,#65324)) ;
#25339=EDGE_LOOP('',(#65325,#65326,#65327)) ;
#25340=EDGE_LOOP('',(#65328,#65329,#65330,#65331)) ;
#25341=EDGE_LOOP('',(#65332,#65333,#65334,#65335)) ;
#25342=EDGE_LOOP('',(#65336,#65337,#65338,#65339)) ;
#25343=EDGE_LOOP('',(#65340,#65341,#65342,#65343)) ;
#25344=EDGE_LOOP('',(#65344,#65345,#65346,#65347)) ;
#25345=EDGE_LOOP('',(#65348,#65349,#65350,#65351)) ;
#25346=EDGE_LOOP('',(#65352,#65353,#65354,#65355)) ;
#25347=EDGE_LOOP('',(#65356,#65357,#65358)) ;
#25348=EDGE_LOOP('',(#65359,#65360,#65361,#65362)) ;
#25349=EDGE_LOOP('',(#65363,#65364,#65365,#65366)) ;
#25350=EDGE_LOOP('',(#65367,#65368,#65369)) ;
#25351=EDGE_LOOP('',(#65370,#65371,#65372,#65373)) ;
#25352=EDGE_LOOP('',(#65374,#65375,#65376,#65377)) ;
#25353=EDGE_LOOP('',(#65378,#65379,#65380,#65381)) ;
#25354=EDGE_LOOP('',(#65382,#65383,#65384,#65385)) ;
#25355=EDGE_LOOP('',(#65386,#65387,#65388,#65389)) ;
#25356=EDGE_LOOP('',(#65390,#65391,#65392,#65393)) ;
#25357=EDGE_LOOP('',(#65394,#65395,#65396,#65397,#65398)) ;
#25358=EDGE_LOOP('',(#65399,#65400,#65401,#65402)) ;
#25359=EDGE_LOOP('',(#65403,#65404,#65405)) ;
#25360=EDGE_LOOP('',(#65406,#65407,#65408,#65409)) ;
#25361=EDGE_LOOP('',(#65410,#65411,#65412,#65413)) ;
#25362=EDGE_LOOP('',(#65414,#65415,#65416)) ;
#25363=EDGE_LOOP('',(#65417,#65418,#65419,#65420)) ;
#25364=EDGE_LOOP('',(#65421,#65422,#65423,#65424)) ;
#25365=EDGE_LOOP('',(#65425,#65426,#65427,#65428)) ;
#25366=EDGE_LOOP('',(#65429,#65430,#65431)) ;
#25367=EDGE_LOOP('',(#65432,#65433,#65434,#65435)) ;
#25368=EDGE_LOOP('',(#65436,#65437,#65438,#65439)) ;
#25369=EDGE_LOOP('',(#65440,#65441,#65442)) ;
#25370=EDGE_LOOP('',(#65443,#65444,#65445)) ;
#25371=EDGE_LOOP('',(#65446,#65447,#65448,#65449)) ;
#25372=EDGE_LOOP('',(#65450,#65451,#65452,#65453)) ;
#25373=EDGE_LOOP('',(#65454,#65455,#65456)) ;
#25374=EDGE_LOOP('',(#65457,#65458,#65459)) ;
#25375=EDGE_LOOP('',(#65460,#65461,#65462,#65463)) ;
#25376=EDGE_LOOP('',(#65464,#65465,#65466,#65467)) ;
#25377=EDGE_LOOP('',(#65468,#65469,#65470)) ;
#25378=EDGE_LOOP('',(#65471,#65472,#65473,#65474)) ;
#25379=EDGE_LOOP('',(#65475,#65476,#65477,#65478)) ;
#25380=EDGE_LOOP('',(#65479,#65480,#65481)) ;
#25381=EDGE_LOOP('',(#65482,#65483,#65484)) ;
#25382=EDGE_LOOP('',(#65485,#65486,#65487,#65488)) ;
#25383=EDGE_LOOP('',(#65489,#65490,#65491,#65492)) ;
#25384=EDGE_LOOP('',(#65493,#65494,#65495,#65496)) ;
#25385=EDGE_LOOP('',(#65497,#65498,#65499,#65500)) ;
#25386=EDGE_LOOP('',(#65501,#65502,#65503,#65504)) ;
#25387=EDGE_LOOP('',(#65505,#65506,#65507,#65508)) ;
#25388=EDGE_LOOP('',(#65509,#65510,#65511,#65512)) ;
#25389=EDGE_LOOP('',(#65513,#65514,#65515)) ;
#25390=EDGE_LOOP('',(#65516,#65517,#65518)) ;
#25391=EDGE_LOOP('',(#65519,#65520,#65521,#65522)) ;
#25392=EDGE_LOOP('',(#65523,#65524,#65525,#65526,#65527,#65528)) ;
#25393=EDGE_LOOP('',(#65529,#65530,#65531,#65532,#65533,#65534,#65535)) ;
#25394=EDGE_LOOP('',(#65536,#65537,#65538,#65539)) ;
#25395=EDGE_LOOP('',(#65540,#65541,#65542,#65543)) ;
#25396=EDGE_LOOP('',(#65544,#65545,#65546,#65547)) ;
#25397=EDGE_LOOP('',(#65548,#65549,#65550,#65551)) ;
#25398=EDGE_LOOP('',(#65552,#65553,#65554)) ;
#25399=EDGE_LOOP('',(#65555,#65556,#65557,#65558)) ;
#25400=EDGE_LOOP('',(#65559,#65560,#65561,#65562)) ;
#25401=EDGE_LOOP('',(#65563,#65564,#65565,#65566)) ;
#25402=EDGE_LOOP('',(#65567,#65568,#65569,#65570)) ;
#25403=EDGE_LOOP('',(#65571,#65572,#65573,#65574)) ;
#25404=EDGE_LOOP('',(#65575,#65576,#65577,#65578)) ;
#25405=EDGE_LOOP('',(#65579,#65580,#65581,#65582)) ;
#25406=EDGE_LOOP('',(#65583,#65584,#65585,#65586)) ;
#25407=EDGE_LOOP('',(#65587,#65588,#65589,#65590)) ;
#25408=EDGE_LOOP('',(#65591,#65592,#65593)) ;
#25409=EDGE_LOOP('',(#65594,#65595,#65596)) ;
#25410=EDGE_LOOP('',(#65597,#65598,#65599,#65600,#65601)) ;
#25411=EDGE_LOOP('',(#65602,#65603,#65604)) ;
#25412=EDGE_LOOP('',(#65605,#65606,#65607)) ;
#25413=EDGE_LOOP('',(#65608,#65609,#65610,#65611)) ;
#25414=EDGE_LOOP('',(#65612,#65613,#65614,#65615)) ;
#25415=EDGE_LOOP('',(#65616,#65617,#65618,#65619)) ;
#25416=EDGE_LOOP('',(#65620,#65621,#65622,#65623)) ;
#25417=EDGE_LOOP('',(#65624,#65625,#65626,#65627)) ;
#25418=EDGE_LOOP('',(#65628,#65629,#65630,#65631)) ;
#25419=EDGE_LOOP('',(#65632,#65633,#65634,#65635)) ;
#25420=EDGE_LOOP('',(#65636,#65637,#65638)) ;
#25421=EDGE_LOOP('',(#65639,#65640,#65641,#65642)) ;
#25422=EDGE_LOOP('',(#65643,#65644,#65645,#65646)) ;
#25423=EDGE_LOOP('',(#65647,#65648,#65649)) ;
#25424=EDGE_LOOP('',(#65650,#65651,#65652,#65653)) ;
#25425=EDGE_LOOP('',(#65654,#65655,#65656,#65657)) ;
#25426=EDGE_LOOP('',(#65658,#65659,#65660,#65661)) ;
#25427=EDGE_LOOP('',(#65662,#65663,#65664,#65665)) ;
#25428=EDGE_LOOP('',(#65666,#65667,#65668,#65669)) ;
#25429=EDGE_LOOP('',(#65670,#65671,#65672,#65673)) ;
#25430=EDGE_LOOP('',(#65674,#65675,#65676,#65677,#65678)) ;
#25431=EDGE_LOOP('',(#65679,#65680,#65681,#65682)) ;
#25432=EDGE_LOOP('',(#65683,#65684,#65685)) ;
#25433=EDGE_LOOP('',(#65686,#65687,#65688,#65689)) ;
#25434=EDGE_LOOP('',(#65690,#65691,#65692,#65693)) ;
#25435=EDGE_LOOP('',(#65694,#65695,#65696)) ;
#25436=EDGE_LOOP('',(#65697,#65698,#65699,#65700)) ;
#25437=EDGE_LOOP('',(#65701,#65702,#65703,#65704)) ;
#25438=EDGE_LOOP('',(#65705,#65706,#65707,#65708)) ;
#25439=EDGE_LOOP('',(#65709,#65710,#65711)) ;
#25440=EDGE_LOOP('',(#65712,#65713,#65714,#65715)) ;
#25441=EDGE_LOOP('',(#65716,#65717,#65718,#65719)) ;
#25442=EDGE_LOOP('',(#65720,#65721,#65722)) ;
#25443=EDGE_LOOP('',(#65723,#65724,#65725)) ;
#25444=EDGE_LOOP('',(#65726,#65727,#65728,#65729)) ;
#25445=EDGE_LOOP('',(#65730,#65731,#65732,#65733)) ;
#25446=EDGE_LOOP('',(#65734,#65735,#65736)) ;
#25447=EDGE_LOOP('',(#65737,#65738,#65739)) ;
#25448=EDGE_LOOP('',(#65740,#65741,#65742,#65743)) ;
#25449=EDGE_LOOP('',(#65744,#65745,#65746,#65747)) ;
#25450=EDGE_LOOP('',(#65748,#65749,#65750)) ;
#25451=EDGE_LOOP('',(#65751,#65752,#65753,#65754)) ;
#25452=EDGE_LOOP('',(#65755,#65756,#65757,#65758)) ;
#25453=EDGE_LOOP('',(#65759,#65760,#65761)) ;
#25454=EDGE_LOOP('',(#65762,#65763,#65764)) ;
#25455=EDGE_LOOP('',(#65765,#65766,#65767,#65768)) ;
#25456=EDGE_LOOP('',(#65769,#65770,#65771,#65772)) ;
#25457=EDGE_LOOP('',(#65773,#65774,#65775,#65776)) ;
#25458=EDGE_LOOP('',(#65777,#65778,#65779,#65780)) ;
#25459=EDGE_LOOP('',(#65781,#65782,#65783,#65784)) ;
#25460=EDGE_LOOP('',(#65785,#65786,#65787,#65788)) ;
#25461=EDGE_LOOP('',(#65789,#65790,#65791,#65792)) ;
#25462=EDGE_LOOP('',(#65793,#65794,#65795)) ;
#25463=EDGE_LOOP('',(#65796,#65797,#65798)) ;
#25464=EDGE_LOOP('',(#65799,#65800,#65801,#65802)) ;
#25465=EDGE_LOOP('',(#65803,#65804,#65805,#65806,#65807,#65808)) ;
#25466=EDGE_LOOP('',(#65809,#65810,#65811,#65812,#65813,#65814,#65815)) ;
#25467=EDGE_LOOP('',(#65816,#65817,#65818,#65819)) ;
#25468=EDGE_LOOP('',(#65820,#65821,#65822,#65823)) ;
#25469=EDGE_LOOP('',(#65824,#65825,#65826,#65827)) ;
#25470=EDGE_LOOP('',(#65828,#65829,#65830,#65831)) ;
#25471=EDGE_LOOP('',(#65832,#65833,#65834)) ;
#25472=EDGE_LOOP('',(#65835,#65836,#65837,#65838)) ;
#25473=EDGE_LOOP('',(#65839,#65840,#65841,#65842)) ;
#25474=EDGE_LOOP('',(#65843,#65844,#65845,#65846)) ;
#25475=EDGE_LOOP('',(#65847,#65848,#65849,#65850)) ;
#25476=EDGE_LOOP('',(#65851,#65852,#65853,#65854)) ;
#25477=EDGE_LOOP('',(#65855,#65856,#65857,#65858)) ;
#25478=EDGE_LOOP('',(#65859,#65860,#65861,#65862)) ;
#25479=EDGE_LOOP('',(#65863,#65864,#65865,#65866)) ;
#25480=EDGE_LOOP('',(#65867,#65868,#65869,#65870)) ;
#25481=EDGE_LOOP('',(#65871,#65872,#65873)) ;
#25482=EDGE_LOOP('',(#65874,#65875,#65876)) ;
#25483=EDGE_LOOP('',(#65877,#65878,#65879,#65880,#65881)) ;
#25484=EDGE_LOOP('',(#65882,#65883,#65884)) ;
#25485=EDGE_LOOP('',(#65885,#65886,#65887)) ;
#25486=EDGE_LOOP('',(#65888,#65889,#65890,#65891)) ;
#25487=EDGE_LOOP('',(#65892,#65893,#65894,#65895)) ;
#25488=EDGE_LOOP('',(#65896,#65897,#65898,#65899)) ;
#25489=EDGE_LOOP('',(#65900,#65901,#65902,#65903)) ;
#25490=EDGE_LOOP('',(#65904,#65905,#65906,#65907)) ;
#25491=EDGE_LOOP('',(#65908,#65909,#65910,#65911)) ;
#25492=EDGE_LOOP('',(#65912,#65913,#65914,#65915)) ;
#25493=EDGE_LOOP('',(#65916,#65917,#65918)) ;
#25494=EDGE_LOOP('',(#65919,#65920,#65921,#65922)) ;
#25495=EDGE_LOOP('',(#65923,#65924,#65925,#65926)) ;
#25496=EDGE_LOOP('',(#65927,#65928,#65929)) ;
#25497=EDGE_LOOP('',(#65930,#65931,#65932,#65933)) ;
#25498=EDGE_LOOP('',(#65934,#65935,#65936,#65937)) ;
#25499=EDGE_LOOP('',(#65938,#65939,#65940,#65941)) ;
#25500=EDGE_LOOP('',(#65942,#65943,#65944,#65945)) ;
#25501=EDGE_LOOP('',(#65946,#65947,#65948,#65949)) ;
#25502=EDGE_LOOP('',(#65950,#65951,#65952,#65953)) ;
#25503=EDGE_LOOP('',(#65954,#65955,#65956,#65957,#65958)) ;
#25504=EDGE_LOOP('',(#65959,#65960,#65961,#65962)) ;
#25505=EDGE_LOOP('',(#65963,#65964,#65965)) ;
#25506=EDGE_LOOP('',(#65966,#65967,#65968,#65969)) ;
#25507=EDGE_LOOP('',(#65970,#65971,#65972,#65973)) ;
#25508=EDGE_LOOP('',(#65974,#65975,#65976)) ;
#25509=EDGE_LOOP('',(#65977,#65978,#65979,#65980)) ;
#25510=EDGE_LOOP('',(#65981,#65982,#65983,#65984)) ;
#25511=EDGE_LOOP('',(#65985,#65986,#65987,#65988)) ;
#25512=EDGE_LOOP('',(#65989,#65990,#65991)) ;
#25513=EDGE_LOOP('',(#65992,#65993,#65994,#65995)) ;
#25514=EDGE_LOOP('',(#65996,#65997,#65998,#65999)) ;
#25515=EDGE_LOOP('',(#66000,#66001,#66002)) ;
#25516=EDGE_LOOP('',(#66003,#66004,#66005)) ;
#25517=EDGE_LOOP('',(#66006,#66007,#66008,#66009)) ;
#25518=EDGE_LOOP('',(#66010,#66011,#66012,#66013)) ;
#25519=EDGE_LOOP('',(#66014,#66015,#66016)) ;
#25520=EDGE_LOOP('',(#66017,#66018,#66019)) ;
#25521=EDGE_LOOP('',(#66020,#66021,#66022,#66023)) ;
#25522=EDGE_LOOP('',(#66024,#66025,#66026,#66027)) ;
#25523=EDGE_LOOP('',(#66028,#66029,#66030)) ;
#25524=EDGE_LOOP('',(#66031,#66032,#66033,#66034)) ;
#25525=EDGE_LOOP('',(#66035,#66036,#66037,#66038)) ;
#25526=EDGE_LOOP('',(#66039,#66040,#66041)) ;
#25527=EDGE_LOOP('',(#66042,#66043,#66044)) ;
#25528=EDGE_LOOP('',(#66045,#66046,#66047,#66048)) ;
#25529=EDGE_LOOP('',(#66049,#66050,#66051,#66052)) ;
#25530=EDGE_LOOP('',(#66053,#66054,#66055,#66056)) ;
#25531=EDGE_LOOP('',(#66057,#66058,#66059,#66060)) ;
#25532=EDGE_LOOP('',(#66061,#66062,#66063,#66064)) ;
#25533=EDGE_LOOP('',(#66065,#66066,#66067,#66068)) ;
#25534=EDGE_LOOP('',(#66069,#66070,#66071,#66072)) ;
#25535=EDGE_LOOP('',(#66073,#66074,#66075,#66076)) ;
#25536=EDGE_LOOP('',(#66077,#66078,#66079,#66080)) ;
#25537=EDGE_LOOP('',(#66081,#66082,#66083,#66084)) ;
#25538=EDGE_LOOP('',(#66085,#66086,#66087,#66088,#66089,#66090)) ;
#25539=EDGE_LOOP('',(#66091,#66092,#66093,#66094,#66095,#66096)) ;
#25540=EDGE_LOOP('',(#66097,#66098,#66099,#66100,#66101)) ;
#25541=EDGE_LOOP('',(#66102,#66103,#66104,#66105)) ;
#25542=EDGE_LOOP('',(#66106,#66107,#66108,#66109)) ;
#25543=EDGE_LOOP('',(#66110,#66111,#66112,#66113)) ;
#25544=EDGE_LOOP('',(#66114,#66115,#66116,#66117)) ;
#25545=EDGE_LOOP('',(#66118,#66119,#66120,#66121)) ;
#25546=EDGE_LOOP('',(#66122,#66123,#66124,#66125)) ;
#25547=EDGE_LOOP('',(#66126,#66127,#66128,#66129)) ;
#25548=EDGE_LOOP('',(#66130,#66131,#66132,#66133)) ;
#25549=EDGE_LOOP('',(#66134,#66135,#66136,#66137)) ;
#25550=EDGE_LOOP('',(#66138,#66139,#66140,#66141)) ;
#25551=EDGE_LOOP('',(#66142,#66143,#66144,#66145)) ;
#25552=EDGE_LOOP('',(#66146,#66147,#66148,#66149)) ;
#25553=EDGE_LOOP('',(#66150,#66151,#66152,#66153)) ;
#25554=EDGE_LOOP('',(#66154,#66155,#66156,#66157,#66158,#66159)) ;
#25555=EDGE_LOOP('',(#66160,#66161,#66162,#66163,#66164,#66165)) ;
#25556=EDGE_LOOP('',(#66166,#66167,#66168,#66169,#66170)) ;
#25557=EDGE_LOOP('',(#66171,#66172,#66173,#66174)) ;
#25558=EDGE_LOOP('',(#66175,#66176,#66177,#66178)) ;
#25559=EDGE_LOOP('',(#66179,#66180,#66181,#66182)) ;
#25560=EDGE_LOOP('',(#66183,#66184,#66185,#66186)) ;
#25561=EDGE_LOOP('',(#66187,#66188,#66189,#66190)) ;
#25562=EDGE_LOOP('',(#66191,#66192,#66193,#66194)) ;
#25563=EDGE_LOOP('',(#66195,#66196,#66197,#66198)) ;
#25564=EDGE_LOOP('',(#66199,#66200,#66201,#66202)) ;
#25565=EDGE_LOOP('',(#66203,#66204,#66205,#66206)) ;
#25566=EDGE_LOOP('',(#66207,#66208,#66209,#66210)) ;
#25567=EDGE_LOOP('',(#66211,#66212,#66213,#66214)) ;
#25568=EDGE_LOOP('',(#66215,#66216,#66217,#66218)) ;
#25569=EDGE_LOOP('',(#66219,#66220,#66221,#66222)) ;
#25570=EDGE_LOOP('',(#66223,#66224,#66225,#66226,#66227,#66228)) ;
#25571=EDGE_LOOP('',(#66229,#66230,#66231,#66232,#66233,#66234)) ;
#25572=EDGE_LOOP('',(#66235,#66236,#66237,#66238,#66239)) ;
#25573=EDGE_LOOP('',(#66240,#66241,#66242,#66243)) ;
#25574=EDGE_LOOP('',(#66244,#66245,#66246,#66247)) ;
#25575=EDGE_LOOP('',(#66248,#66249,#66250,#66251)) ;
#25576=EDGE_LOOP('',(#66252,#66253,#66254,#66255)) ;
#25577=EDGE_LOOP('',(#66256,#66257,#66258,#66259)) ;
#25578=EDGE_LOOP('',(#66260,#66261,#66262,#66263)) ;
#25579=EDGE_LOOP('',(#66264,#66265,#66266,#66267)) ;
#25580=EDGE_LOOP('',(#66268,#66269,#66270,#66271)) ;
#25581=EDGE_LOOP('',(#66272,#66273,#66274,#66275)) ;
#25582=EDGE_LOOP('',(#66276,#66277,#66278,#66279)) ;
#25583=EDGE_LOOP('',(#66280,#66281,#66282,#66283)) ;
#25584=EDGE_LOOP('',(#66284,#66285,#66286,#66287)) ;
#25585=EDGE_LOOP('',(#66288,#66289,#66290,#66291)) ;
#25586=EDGE_LOOP('',(#66292,#66293,#66294,#66295,#66296,#66297)) ;
#25587=EDGE_LOOP('',(#66298,#66299,#66300,#66301,#66302,#66303)) ;
#25588=EDGE_LOOP('',(#66304,#66305,#66306,#66307,#66308)) ;
#25589=EDGE_LOOP('',(#66309,#66310,#66311,#66312)) ;
#25590=EDGE_LOOP('',(#66313,#66314,#66315,#66316)) ;
#25591=EDGE_LOOP('',(#66317,#66318,#66319,#66320)) ;
#25592=EDGE_LOOP('',(#66321,#66322,#66323,#66324)) ;
#25593=EDGE_LOOP('',(#66325,#66326,#66327,#66328)) ;
#25594=EDGE_LOOP('',(#66329,#66330,#66331,#66332)) ;
#25595=EDGE_LOOP('',(#66333,#66334,#66335,#66336)) ;
#25596=EDGE_LOOP('',(#66337,#66338,#66339,#66340)) ;
#25597=EDGE_LOOP('',(#66341,#66342,#66343,#66344)) ;
#25598=EDGE_LOOP('',(#66345,#66346,#66347,#66348)) ;
#25599=EDGE_LOOP('',(#66349,#66350,#66351,#66352)) ;
#25600=EDGE_LOOP('',(#66353,#66354,#66355,#66356)) ;
#25601=EDGE_LOOP('',(#66357,#66358,#66359,#66360)) ;
#25602=EDGE_LOOP('',(#66361,#66362,#66363,#66364,#66365,#66366)) ;
#25603=EDGE_LOOP('',(#66367,#66368,#66369,#66370,#66371,#66372)) ;
#25604=EDGE_LOOP('',(#66373,#66374,#66375,#66376,#66377)) ;
#25605=EDGE_LOOP('',(#66378,#66379,#66380,#66381)) ;
#25606=EDGE_LOOP('',(#66382,#66383,#66384,#66385)) ;
#25607=EDGE_LOOP('',(#66386,#66387,#66388,#66389)) ;
#25608=EDGE_LOOP('',(#66390,#66391,#66392,#66393)) ;
#25609=EDGE_LOOP('',(#66394,#66395,#66396,#66397)) ;
#25610=EDGE_LOOP('',(#66398,#66399,#66400,#66401)) ;
#25611=EDGE_LOOP('',(#66402,#66403,#66404,#66405)) ;
#25612=EDGE_LOOP('',(#66406,#66407,#66408,#66409)) ;
#25613=EDGE_LOOP('',(#66410,#66411,#66412,#66413)) ;
#25614=EDGE_LOOP('',(#66414,#66415,#66416,#66417)) ;
#25615=EDGE_LOOP('',(#66418,#66419,#66420,#66421)) ;
#25616=EDGE_LOOP('',(#66422,#66423,#66424,#66425)) ;
#25617=EDGE_LOOP('',(#66426,#66427,#66428,#66429)) ;
#25618=EDGE_LOOP('',(#66430,#66431,#66432,#66433,#66434,#66435)) ;
#25619=EDGE_LOOP('',(#66436,#66437,#66438,#66439,#66440,#66441)) ;
#25620=EDGE_LOOP('',(#66442,#66443,#66444,#66445,#66446)) ;
#25621=EDGE_LOOP('',(#66447,#66448,#66449,#66450)) ;
#25622=EDGE_LOOP('',(#66451,#66452,#66453,#66454)) ;
#25623=EDGE_LOOP('',(#66455,#66456,#66457,#66458)) ;
#25624=EDGE_LOOP('',(#66459,#66460,#66461,#66462)) ;
#25625=EDGE_LOOP('',(#66463,#66464,#66465,#66466)) ;
#25626=EDGE_LOOP('',(#66467,#66468,#66469,#66470)) ;
#25627=EDGE_LOOP('',(#66471,#66472,#66473,#66474)) ;
#25628=EDGE_LOOP('',(#66475,#66476,#66477,#66478)) ;
#25629=EDGE_LOOP('',(#66479,#66480,#66481,#66482)) ;
#25630=EDGE_LOOP('',(#66483,#66484,#66485,#66486)) ;
#25631=EDGE_LOOP('',(#66487,#66488,#66489,#66490)) ;
#25632=EDGE_LOOP('',(#66491,#66492,#66493,#66494)) ;
#25633=EDGE_LOOP('',(#66495,#66496,#66497,#66498)) ;
#25634=EDGE_LOOP('',(#66499,#66500,#66501,#66502,#66503,#66504)) ;
#25635=EDGE_LOOP('',(#66505,#66506,#66507,#66508,#66509,#66510)) ;
#25636=EDGE_LOOP('',(#66511,#66512,#66513,#66514,#66515)) ;
#25637=EDGE_LOOP('',(#66516,#66517,#66518,#66519)) ;
#25638=EDGE_LOOP('',(#66520,#66521,#66522,#66523)) ;
#25639=EDGE_LOOP('',(#66524,#66525,#66526,#66527)) ;
#25640=EDGE_LOOP('',(#66528,#66529,#66530,#66531)) ;
#25641=EDGE_LOOP('',(#66532,#66533,#66534,#66535)) ;
#25642=EDGE_LOOP('',(#66536,#66537,#66538,#66539)) ;
#25643=EDGE_LOOP('',(#66540,#66541,#66542,#66543)) ;
#25644=EDGE_LOOP('',(#66544,#66545,#66546,#66547)) ;
#25645=EDGE_LOOP('',(#66548,#66549,#66550,#66551)) ;
#25646=EDGE_LOOP('',(#66552,#66553,#66554,#66555)) ;
#25647=EDGE_LOOP('',(#66556,#66557,#66558,#66559)) ;
#25648=EDGE_LOOP('',(#66560,#66561,#66562,#66563)) ;
#25649=EDGE_LOOP('',(#66564,#66565,#66566,#66567)) ;
#25650=EDGE_LOOP('',(#66568,#66569,#66570,#66571,#66572,#66573)) ;
#25651=EDGE_LOOP('',(#66574,#66575,#66576,#66577,#66578,#66579)) ;
#25652=EDGE_LOOP('',(#66580,#66581,#66582,#66583,#66584)) ;
#25653=EDGE_LOOP('',(#66585,#66586,#66587,#66588)) ;
#25654=EDGE_LOOP('',(#66589,#66590,#66591,#66592)) ;
#25655=EDGE_LOOP('',(#66593,#66594,#66595,#66596)) ;
#25656=EDGE_LOOP('',(#66597,#66598,#66599,#66600)) ;
#25657=EDGE_LOOP('',(#66601,#66602,#66603,#66604)) ;
#25658=EDGE_LOOP('',(#66605,#66606,#66607,#66608)) ;
#25659=EDGE_LOOP('',(#66609,#66610,#66611,#66612)) ;
#25660=EDGE_LOOP('',(#66613,#66614,#66615,#66616)) ;
#25661=EDGE_LOOP('',(#66617,#66618,#66619,#66620)) ;
#25662=EDGE_LOOP('',(#66621,#66622,#66623,#66624)) ;
#25663=EDGE_LOOP('',(#66625,#66626,#66627,#66628)) ;
#25664=EDGE_LOOP('',(#66629,#66630,#66631,#66632)) ;
#25665=EDGE_LOOP('',(#66633,#66634,#66635,#66636)) ;
#25666=EDGE_LOOP('',(#66637,#66638,#66639,#66640,#66641,#66642)) ;
#25667=EDGE_LOOP('',(#66643,#66644,#66645,#66646,#66647,#66648)) ;
#25668=EDGE_LOOP('',(#66649,#66650,#66651,#66652,#66653)) ;
#25669=EDGE_LOOP('',(#66654,#66655,#66656,#66657)) ;
#25670=EDGE_LOOP('',(#66658,#66659,#66660,#66661)) ;
#25671=EDGE_LOOP('',(#66662,#66663,#66664,#66665)) ;
#25672=EDGE_LOOP('',(#66666,#66667,#66668,#66669)) ;
#25673=EDGE_LOOP('',(#66670,#66671,#66672,#66673)) ;
#25674=EDGE_LOOP('',(#66674,#66675,#66676,#66677)) ;
#25675=EDGE_LOOP('',(#66678,#66679,#66680,#66681)) ;
#25676=EDGE_LOOP('',(#66682,#66683,#66684,#66685)) ;
#25677=EDGE_LOOP('',(#66686,#66687,#66688,#66689)) ;
#25678=EDGE_LOOP('',(#66690,#66691,#66692,#66693)) ;
#25679=EDGE_LOOP('',(#66694,#66695,#66696,#66697)) ;
#25680=EDGE_LOOP('',(#66698,#66699,#66700,#66701)) ;
#25681=EDGE_LOOP('',(#66702,#66703,#66704,#66705)) ;
#25682=EDGE_LOOP('',(#66706,#66707,#66708,#66709)) ;
#25683=EDGE_LOOP('',(#66710,#66711,#66712,#66713)) ;
#25684=EDGE_LOOP('',(#66714,#66715,#66716,#66717)) ;
#25685=EDGE_LOOP('',(#66718,#66719,#66720,#66721)) ;
#25686=EDGE_LOOP('',(#66722,#66723,#66724,#66725)) ;
#25687=EDGE_LOOP('',(#66726,#66727,#66728,#66729)) ;
#25688=EDGE_LOOP('',(#66730,#66731,#66732,#66733)) ;
#25689=EDGE_LOOP('',(#66734,#66735,#66736,#66737)) ;
#25690=EDGE_LOOP('',(#66738,#66739,#66740,#66741)) ;
#25691=EDGE_LOOP('',(#66742,#66743,#66744,#66745)) ;
#25692=EDGE_LOOP('',(#66746,#66747,#66748,#66749)) ;
#25693=EDGE_LOOP('',(#66750,#66751,#66752,#66753)) ;
#25694=EDGE_LOOP('',(#66754,#66755,#66756,#66757)) ;
#25695=EDGE_LOOP('',(#66758,#66759,#66760,#66761)) ;
#25696=EDGE_LOOP('',(#66762,#66763,#66764,#66765)) ;
#25697=EDGE_LOOP('',(#66766,#66767,#66768,#66769)) ;
#25698=EDGE_LOOP('',(#66770,#66771,#66772,#66773)) ;
#25699=EDGE_LOOP('',(#66774,#66775,#66776,#66777)) ;
#25700=EDGE_LOOP('',(#66778,#66779,#66780,#66781)) ;
#25701=EDGE_LOOP('',(#66782,#66783,#66784,#66785)) ;
#25702=EDGE_LOOP('',(#66786,#66787,#66788,#66789)) ;
#25703=EDGE_LOOP('',(#66790,#66791,#66792,#66793)) ;
#25704=EDGE_LOOP('',(#66794,#66795,#66796,#66797)) ;
#25705=EDGE_LOOP('',(#66798,#66799,#66800,#66801)) ;
#25706=EDGE_LOOP('',(#66802,#66803,#66804,#66805)) ;
#25707=EDGE_LOOP('',(#66806,#66807,#66808,#66809)) ;
#25708=EDGE_LOOP('',(#66810,#66811,#66812,#66813)) ;
#25709=EDGE_LOOP('',(#66814,#66815,#66816,#66817)) ;
#25710=EDGE_LOOP('',(#66818,#66819,#66820,#66821)) ;
#25711=EDGE_LOOP('',(#66822,#66823,#66824,#66825)) ;
#25712=EDGE_LOOP('',(#66826,#66827,#66828,#66829)) ;
#25713=EDGE_LOOP('',(#66830,#66831,#66832,#66833)) ;
#25714=EDGE_LOOP('',(#66834,#66835,#66836,#66837)) ;
#25715=EDGE_LOOP('',(#66838,#66839,#66840)) ;
#25716=EDGE_LOOP('',(#66841,#66842,#66843,#66844)) ;
#25717=EDGE_LOOP('',(#66845,#66846,#66847,#66848)) ;
#25718=EDGE_LOOP('',(#66849,#66850,#66851,#66852)) ;
#25719=EDGE_LOOP('',(#66853,#66854,#66855)) ;
#25720=EDGE_LOOP('',(#66856,#66857,#66858)) ;
#25721=EDGE_LOOP('',(#66859,#66860,#66861,#66862)) ;
#25722=EDGE_LOOP('',(#66863,#66864,#66865,#66866)) ;
#25723=EDGE_LOOP('',(#66867,#66868,#66869,#66870)) ;
#25724=EDGE_LOOP('',(#66871,#66872,#66873)) ;
#25725=EDGE_LOOP('',(#66874,#66875,#66876,#66877)) ;
#25726=EDGE_LOOP('',(#66878,#66879,#66880,#66881)) ;
#25727=EDGE_LOOP('',(#66882,#66883,#66884,#66885)) ;
#25728=EDGE_LOOP('',(#66886,#66887,#66888,#66889)) ;
#25729=EDGE_LOOP('',(#66890,#66891,#66892)) ;
#25730=EDGE_LOOP('',(#66893,#66894,#66895,#66896)) ;
#25731=EDGE_LOOP('',(#66897,#66898,#66899,#66900)) ;
#25732=EDGE_LOOP('',(#66901,#66902,#66903,#66904)) ;
#25733=EDGE_LOOP('',(#66905,#66906,#66907)) ;
#25734=EDGE_LOOP('',(#66908,#66909,#66910)) ;
#25735=EDGE_LOOP('',(#66911,#66912,#66913,#66914)) ;
#25736=EDGE_LOOP('',(#66915,#66916,#66917,#66918)) ;
#25737=EDGE_LOOP('',(#66919,#66920,#66921,#66922)) ;
#25738=EDGE_LOOP('',(#66923,#66924,#66925)) ;
#25739=EDGE_LOOP('',(#66926,#66927,#66928,#66929)) ;
#25740=EDGE_LOOP('',(#66930,#66931,#66932,#66933)) ;
#25741=EDGE_LOOP('',(#66934,#66935,#66936,#66937)) ;
#25742=EDGE_LOOP('',(#66938,#66939,#66940,#66941)) ;
#25743=EDGE_LOOP('',(#66942,#66943,#66944)) ;
#25744=EDGE_LOOP('',(#66945,#66946,#66947,#66948)) ;
#25745=EDGE_LOOP('',(#66949,#66950,#66951,#66952)) ;
#25746=EDGE_LOOP('',(#66953,#66954,#66955,#66956)) ;
#25747=EDGE_LOOP('',(#66957,#66958,#66959)) ;
#25748=EDGE_LOOP('',(#66960,#66961,#66962)) ;
#25749=EDGE_LOOP('',(#66963,#66964,#66965,#66966)) ;
#25750=EDGE_LOOP('',(#66967,#66968,#66969,#66970)) ;
#25751=EDGE_LOOP('',(#66971,#66972,#66973,#66974)) ;
#25752=EDGE_LOOP('',(#66975,#66976,#66977)) ;
#25753=EDGE_LOOP('',(#66978,#66979,#66980,#66981)) ;
#25754=EDGE_LOOP('',(#66982,#66983,#66984,#66985)) ;
#25755=EDGE_LOOP('',(#66986,#66987,#66988,#66989)) ;
#25756=EDGE_LOOP('',(#66990,#66991,#66992,#66993)) ;
#25757=EDGE_LOOP('',(#66994,#66995,#66996)) ;
#25758=EDGE_LOOP('',(#66997,#66998,#66999,#67000)) ;
#25759=EDGE_LOOP('',(#67001,#67002,#67003,#67004)) ;
#25760=EDGE_LOOP('',(#67005,#67006,#67007,#67008)) ;
#25761=EDGE_LOOP('',(#67009,#67010,#67011)) ;
#25762=EDGE_LOOP('',(#67012,#67013,#67014)) ;
#25763=EDGE_LOOP('',(#67015,#67016,#67017,#67018)) ;
#25764=EDGE_LOOP('',(#67019,#67020,#67021,#67022)) ;
#25765=EDGE_LOOP('',(#67023,#67024,#67025,#67026)) ;
#25766=EDGE_LOOP('',(#67027,#67028,#67029)) ;
#25767=EDGE_LOOP('',(#67030,#67031,#67032,#67033)) ;
#25768=EDGE_LOOP('',(#67034,#67035,#67036,#67037)) ;
#25769=EDGE_LOOP('',(#67038,#67039,#67040,#67041)) ;
#25770=EDGE_LOOP('',(#67042,#67043,#67044,#67045)) ;
#25771=EDGE_LOOP('',(#67046,#67047,#67048)) ;
#25772=EDGE_LOOP('',(#67049,#67050,#67051,#67052)) ;
#25773=EDGE_LOOP('',(#67053,#67054,#67055,#67056)) ;
#25774=EDGE_LOOP('',(#67057,#67058,#67059,#67060)) ;
#25775=EDGE_LOOP('',(#67061,#67062,#67063)) ;
#25776=EDGE_LOOP('',(#67064,#67065,#67066)) ;
#25777=EDGE_LOOP('',(#67067,#67068,#67069,#67070)) ;
#25778=EDGE_LOOP('',(#67071,#67072,#67073,#67074)) ;
#25779=EDGE_LOOP('',(#67075,#67076,#67077,#67078)) ;
#25780=EDGE_LOOP('',(#67079,#67080,#67081)) ;
#25781=EDGE_LOOP('',(#67082,#67083,#67084,#67085)) ;
#25782=EDGE_LOOP('',(#67086,#67087,#67088,#67089)) ;
#25783=EDGE_LOOP('',(#67090,#67091,#67092,#67093)) ;
#25784=EDGE_LOOP('',(#67094,#67095,#67096,#67097)) ;
#25785=EDGE_LOOP('',(#67098,#67099,#67100)) ;
#25786=EDGE_LOOP('',(#67101,#67102,#67103,#67104)) ;
#25787=EDGE_LOOP('',(#67105,#67106,#67107,#67108)) ;
#25788=EDGE_LOOP('',(#67109,#67110,#67111,#67112)) ;
#25789=EDGE_LOOP('',(#67113,#67114,#67115)) ;
#25790=EDGE_LOOP('',(#67116,#67117,#67118)) ;
#25791=EDGE_LOOP('',(#67119,#67120,#67121,#67122)) ;
#25792=EDGE_LOOP('',(#67123,#67124,#67125,#67126)) ;
#25793=EDGE_LOOP('',(#67127,#67128,#67129,#67130)) ;
#25794=EDGE_LOOP('',(#67131,#67132,#67133)) ;
#25795=EDGE_LOOP('',(#67134,#67135,#67136,#67137)) ;
#25796=EDGE_LOOP('',(#67138,#67139,#67140,#67141)) ;
#25797=EDGE_LOOP('',(#67142,#67143,#67144,#67145)) ;
#25798=EDGE_LOOP('',(#67146,#67147,#67148,#67149)) ;
#25799=EDGE_LOOP('',(#67150,#67151,#67152)) ;
#25800=EDGE_LOOP('',(#67153,#67154,#67155,#67156)) ;
#25801=EDGE_LOOP('',(#67157,#67158,#67159,#67160)) ;
#25802=EDGE_LOOP('',(#67161,#67162,#67163,#67164)) ;
#25803=EDGE_LOOP('',(#67165,#67166,#67167)) ;
#25804=EDGE_LOOP('',(#67168,#67169,#67170)) ;
#25805=EDGE_LOOP('',(#67171,#67172,#67173,#67174)) ;
#25806=EDGE_LOOP('',(#67175,#67176,#67177,#67178)) ;
#25807=EDGE_LOOP('',(#67179,#67180,#67181,#67182)) ;
#25808=EDGE_LOOP('',(#67183,#67184,#67185)) ;
#25809=EDGE_LOOP('',(#67186,#67187,#67188,#67189)) ;
#25810=EDGE_LOOP('',(#67190,#67191,#67192,#67193)) ;
#25811=EDGE_LOOP('',(#67194,#67195,#67196,#67197)) ;
#25812=EDGE_LOOP('',(#67198,#67199,#67200,#67201)) ;
#25813=EDGE_LOOP('',(#67202,#67203,#67204)) ;
#25814=EDGE_LOOP('',(#67205,#67206,#67207,#67208)) ;
#25815=EDGE_LOOP('',(#67209,#67210,#67211,#67212)) ;
#25816=EDGE_LOOP('',(#67213,#67214,#67215,#67216)) ;
#25817=EDGE_LOOP('',(#67217,#67218,#67219)) ;
#25818=EDGE_LOOP('',(#67220,#67221,#67222)) ;
#25819=EDGE_LOOP('',(#67223,#67224,#67225,#67226)) ;
#25820=EDGE_LOOP('',(#67227,#67228,#67229,#67230)) ;
#25821=EDGE_LOOP('',(#67231,#67232,#67233,#67234)) ;
#25822=EDGE_LOOP('',(#67235,#67236,#67237)) ;
#25823=EDGE_LOOP('',(#67238,#67239,#67240,#67241)) ;
#25824=EDGE_LOOP('',(#67242,#67243,#67244,#67245)) ;
#25825=EDGE_LOOP('',(#67246,#67247,#67248,#67249)) ;
#25826=EDGE_LOOP('',(#67250,#67251,#67252,#67253)) ;
#25827=EDGE_LOOP('',(#67254,#67255,#67256)) ;
#25828=EDGE_LOOP('',(#67257,#67258,#67259,#67260)) ;
#25829=EDGE_LOOP('',(#67261,#67262,#67263,#67264)) ;
#25830=EDGE_LOOP('',(#67265,#67266,#67267,#67268)) ;
#25831=EDGE_LOOP('',(#67269,#67270,#67271)) ;
#25832=EDGE_LOOP('',(#67272,#67273,#67274)) ;
#25833=EDGE_LOOP('',(#67275,#67276,#67277,#67278)) ;
#25834=EDGE_LOOP('',(#67279,#67280,#67281,#67282)) ;
#25835=EDGE_LOOP('',(#67283,#67284,#67285,#67286)) ;
#25836=EDGE_LOOP('',(#67287,#67288,#67289)) ;
#25837=EDGE_LOOP('',(#67290,#67291,#67292,#67293)) ;
#25838=EDGE_LOOP('',(#67294,#67295,#67296,#67297)) ;
#25839=EDGE_LOOP('',(#67298,#67299,#67300,#67301)) ;
#25840=EDGE_LOOP('',(#67302,#67303,#67304,#67305)) ;
#25841=EDGE_LOOP('',(#67306,#67307,#67308)) ;
#25842=EDGE_LOOP('',(#67309,#67310,#67311,#67312)) ;
#25843=EDGE_LOOP('',(#67313,#67314,#67315,#67316)) ;
#25844=EDGE_LOOP('',(#67317,#67318,#67319,#67320)) ;
#25845=EDGE_LOOP('',(#67321,#67322,#67323)) ;
#25846=EDGE_LOOP('',(#67324,#67325,#67326)) ;
#25847=EDGE_LOOP('',(#67327,#67328,#67329,#67330)) ;
#25848=EDGE_LOOP('',(#67331,#67332,#67333,#67334)) ;
#25849=EDGE_LOOP('',(#67335,#67336,#67337,#67338)) ;
#25850=EDGE_LOOP('',(#67339,#67340,#67341)) ;
#25851=EDGE_LOOP('',(#67342,#67343,#67344,#67345)) ;
#25852=EDGE_LOOP('',(#67346,#67347,#67348,#67349)) ;
#25853=EDGE_LOOP('',(#67350,#67351,#67352,#67353)) ;
#25854=EDGE_LOOP('',(#67354,#67355,#67356,#67357)) ;
#25855=EDGE_LOOP('',(#67358,#67359,#67360)) ;
#25856=EDGE_LOOP('',(#67361,#67362,#67363,#67364)) ;
#25857=EDGE_LOOP('',(#67365,#67366,#67367,#67368)) ;
#25858=EDGE_LOOP('',(#67369,#67370,#67371,#67372)) ;
#25859=EDGE_LOOP('',(#67373,#67374,#67375)) ;
#25860=EDGE_LOOP('',(#67376,#67377,#67378)) ;
#25861=EDGE_LOOP('',(#67379,#67380,#67381,#67382)) ;
#25862=EDGE_LOOP('',(#67383,#67384,#67385,#67386)) ;
#25863=EDGE_LOOP('',(#67387,#67388,#67389,#67390)) ;
#25864=EDGE_LOOP('',(#67391,#67392,#67393)) ;
#25865=EDGE_LOOP('',(#67394,#67395,#67396,#67397)) ;
#25866=EDGE_LOOP('',(#67398,#67399,#67400,#67401)) ;
#25867=EDGE_LOOP('',(#67402,#67403,#67404,#67405)) ;
#25868=EDGE_LOOP('',(#67406,#67407,#67408,#67409)) ;
#25869=EDGE_LOOP('',(#67410,#67411,#67412)) ;
#25870=EDGE_LOOP('',(#67413,#67414,#67415,#67416)) ;
#25871=EDGE_LOOP('',(#67417,#67418,#67419,#67420)) ;
#25872=EDGE_LOOP('',(#67421,#67422,#67423,#67424)) ;
#25873=EDGE_LOOP('',(#67425,#67426,#67427)) ;
#25874=EDGE_LOOP('',(#67428,#67429,#67430)) ;
#25875=EDGE_LOOP('',(#67431,#67432,#67433,#67434)) ;
#25876=EDGE_LOOP('',(#67435,#67436,#67437,#67438)) ;
#25877=EDGE_LOOP('',(#67439,#67440,#67441,#67442)) ;
#25878=EDGE_LOOP('',(#67443,#67444,#67445)) ;
#25879=EDGE_LOOP('',(#67446,#67447,#67448,#67449)) ;
#25880=EDGE_LOOP('',(#67450,#67451,#67452,#67453)) ;
#25881=EDGE_LOOP('',(#67454,#67455,#67456,#67457)) ;
#25882=EDGE_LOOP('',(#67458,#67459,#67460,#67461)) ;
#25883=EDGE_LOOP('',(#67462,#67463,#67464)) ;
#25884=EDGE_LOOP('',(#67465,#67466,#67467,#67468)) ;
#25885=EDGE_LOOP('',(#67469,#67470,#67471,#67472)) ;
#25886=EDGE_LOOP('',(#67473,#67474,#67475,#67476)) ;
#25887=EDGE_LOOP('',(#67477,#67478,#67479)) ;
#25888=EDGE_LOOP('',(#67480,#67481,#67482)) ;
#25889=EDGE_LOOP('',(#67483,#67484,#67485,#67486)) ;
#25890=EDGE_LOOP('',(#67487,#67488,#67489,#67490)) ;
#25891=EDGE_LOOP('',(#67491,#67492,#67493,#67494)) ;
#25892=EDGE_LOOP('',(#67495,#67496,#67497)) ;
#25893=EDGE_LOOP('',(#67498,#67499,#67500,#67501)) ;
#25894=EDGE_LOOP('',(#67502,#67503,#67504,#67505)) ;
#25895=EDGE_LOOP('',(#67506,#67507,#67508,#67509)) ;
#25896=EDGE_LOOP('',(#67510,#67511,#67512,#67513)) ;
#25897=EDGE_LOOP('',(#67514,#67515,#67516)) ;
#25898=EDGE_LOOP('',(#67517,#67518,#67519,#67520)) ;
#25899=EDGE_LOOP('',(#67521,#67522,#67523,#67524)) ;
#25900=EDGE_LOOP('',(#67525,#67526,#67527,#67528)) ;
#25901=EDGE_LOOP('',(#67529,#67530,#67531)) ;
#25902=EDGE_LOOP('',(#67532,#67533,#67534)) ;
#25903=EDGE_LOOP('',(#67535,#67536,#67537,#67538)) ;
#25904=EDGE_LOOP('',(#67539,#67540,#67541,#67542)) ;
#25905=EDGE_LOOP('',(#67543,#67544,#67545,#67546)) ;
#25906=EDGE_LOOP('',(#67547,#67548,#67549)) ;
#25907=EDGE_LOOP('',(#67550,#67551,#67552,#67553)) ;
#25908=EDGE_LOOP('',(#67554,#67555,#67556,#67557)) ;
#25909=EDGE_LOOP('',(#67558,#67559,#67560,#67561)) ;
#25910=EDGE_LOOP('',(#67562,#67563,#67564,#67565)) ;
#25911=EDGE_LOOP('',(#67566,#67567,#67568)) ;
#25912=EDGE_LOOP('',(#67569,#67570,#67571,#67572)) ;
#25913=EDGE_LOOP('',(#67573,#67574,#67575,#67576)) ;
#25914=EDGE_LOOP('',(#67577,#67578,#67579,#67580)) ;
#25915=EDGE_LOOP('',(#67581,#67582,#67583)) ;
#25916=EDGE_LOOP('',(#67584,#67585,#67586)) ;
#25917=EDGE_LOOP('',(#67587,#67588,#67589,#67590)) ;
#25918=EDGE_LOOP('',(#67591,#67592,#67593,#67594)) ;
#25919=EDGE_LOOP('',(#67595,#67596,#67597,#67598)) ;
#25920=EDGE_LOOP('',(#67599,#67600,#67601)) ;
#25921=EDGE_LOOP('',(#67602,#67603,#67604,#67605)) ;
#25922=EDGE_LOOP('',(#67606,#67607,#67608,#67609)) ;
#25923=EDGE_LOOP('',(#67610,#67611,#67612,#67613)) ;
#25924=EDGE_LOOP('',(#67614,#67615,#67616,#67617)) ;
#25925=EDGE_LOOP('',(#67618,#67619,#67620)) ;
#25926=EDGE_LOOP('',(#67621,#67622,#67623,#67624)) ;
#25927=EDGE_LOOP('',(#67625,#67626,#67627,#67628)) ;
#25928=EDGE_LOOP('',(#67629,#67630,#67631,#67632)) ;
#25929=EDGE_LOOP('',(#67633,#67634,#67635)) ;
#25930=EDGE_LOOP('',(#67636,#67637,#67638)) ;
#25931=EDGE_LOOP('',(#67639,#67640,#67641,#67642)) ;
#25932=EDGE_LOOP('',(#67643,#67644,#67645,#67646)) ;
#25933=EDGE_LOOP('',(#67647,#67648,#67649,#67650)) ;
#25934=EDGE_LOOP('',(#67651,#67652,#67653)) ;
#25935=EDGE_LOOP('',(#67654,#67655,#67656,#67657)) ;
#25936=EDGE_LOOP('',(#67658,#67659,#67660,#67661)) ;
#25937=EDGE_LOOP('',(#67662,#67663,#67664,#67665)) ;
#25938=EDGE_LOOP('',(#67666,#67667,#67668,#67669)) ;
#25939=EDGE_LOOP('',(#67670,#67671,#67672)) ;
#25940=EDGE_LOOP('',(#67673,#67674,#67675,#67676)) ;
#25941=EDGE_LOOP('',(#67677,#67678,#67679,#67680)) ;
#25942=EDGE_LOOP('',(#67681,#67682,#67683,#67684)) ;
#25943=EDGE_LOOP('',(#67685,#67686,#67687)) ;
#25944=EDGE_LOOP('',(#67688,#67689,#67690)) ;
#25945=EDGE_LOOP('',(#67691,#67692,#67693,#67694)) ;
#25946=EDGE_LOOP('',(#67695,#67696,#67697,#67698)) ;
#25947=EDGE_LOOP('',(#67699,#67700,#67701,#67702)) ;
#25948=EDGE_LOOP('',(#67703,#67704,#67705)) ;
#25949=EDGE_LOOP('',(#67706,#67707,#67708,#67709)) ;
#25950=EDGE_LOOP('',(#67710,#67711,#67712,#67713)) ;
#25951=EDGE_LOOP('',(#67714,#67715,#67716,#67717)) ;
#25952=EDGE_LOOP('',(#67718,#67719,#67720,#67721)) ;
#25953=EDGE_LOOP('',(#67722,#67723,#67724)) ;
#25954=EDGE_LOOP('',(#67725,#67726,#67727,#67728)) ;
#25955=EDGE_LOOP('',(#67729,#67730,#67731,#67732)) ;
#25956=EDGE_LOOP('',(#67733,#67734,#67735,#67736)) ;
#25957=EDGE_LOOP('',(#67737,#67738,#67739)) ;
#25958=EDGE_LOOP('',(#67740,#67741,#67742)) ;
#25959=EDGE_LOOP('',(#67743,#67744,#67745,#67746)) ;
#25960=EDGE_LOOP('',(#67747,#67748,#67749,#67750)) ;
#25961=EDGE_LOOP('',(#67751,#67752,#67753,#67754)) ;
#25962=EDGE_LOOP('',(#67755,#67756,#67757)) ;
#25963=EDGE_LOOP('',(#67758,#67759,#67760,#67761)) ;
#25964=EDGE_LOOP('',(#67762,#67763,#67764,#67765)) ;
#25965=EDGE_LOOP('',(#67766,#67767,#67768,#67769)) ;
#25966=EDGE_LOOP('',(#67770,#67771,#67772,#67773)) ;
#25967=EDGE_LOOP('',(#67774,#67775,#67776,#67777)) ;
#25968=EDGE_LOOP('',(#67778,#67779,#67780,#67781)) ;
#25969=EDGE_LOOP('',(#67782,#67783,#67784,#67785)) ;
#25970=EDGE_LOOP('',(#67786,#67787,#67788,#67789)) ;
#25971=EDGE_LOOP('',(#67790,#67791,#67792,#67793,#67794)) ;
#25972=EDGE_LOOP('',(#67795,#67796,#67797,#67798)) ;
#25973=EDGE_LOOP('',(#67799,#67800,#67801,#67802)) ;
#25974=EDGE_LOOP('',(#67803,#67804,#67805,#67806)) ;
#25975=EDGE_LOOP('',(#67807,#67808,#67809,#67810)) ;
#25976=EDGE_LOOP('',(#67811,#67812,#67813,#67814)) ;
#25977=EDGE_LOOP('',(#67815,#67816,#67817,#67818)) ;
#25978=EDGE_LOOP('',(#67819,#67820,#67821,#67822)) ;
#25979=EDGE_LOOP('',(#67823,#67824,#67825,#67826)) ;
#25980=EDGE_LOOP('',(#67827,#67828,#67829,#67830)) ;
#25981=EDGE_LOOP('',(#67831,#67832,#67833,#67834)) ;
#25982=EDGE_LOOP('',(#67835,#67836,#67837,#67838)) ;
#25983=EDGE_LOOP('',(#67839,#67840,#67841,#67842)) ;
#25984=EDGE_LOOP('',(#67843,#67844,#67845,#67846)) ;
#25985=EDGE_LOOP('',(#67847,#67848,#67849,#67850)) ;
#25986=EDGE_LOOP('',(#67851,#67852,#67853,#67854)) ;
#25987=EDGE_LOOP('',(#67855,#67856,#67857,#67858)) ;
#25988=EDGE_LOOP('',(#67859,#67860,#67861,#67862)) ;
#25989=EDGE_LOOP('',(#67863,#67864,#67865,#67866)) ;
#25990=EDGE_LOOP('',(#67867,#67868,#67869,#67870)) ;
#25991=EDGE_LOOP('',(#67871,#67872,#67873,#67874)) ;
#25992=EDGE_LOOP('',(#67875,#67876,#67877,#67878)) ;
#25993=EDGE_LOOP('',(#67879,#67880,#67881,#67882)) ;
#25994=EDGE_LOOP('',(#67883,#67884,#67885,#67886)) ;
#25995=EDGE_LOOP('',(#67887,#67888,#67889,#67890,#67891)) ;
#25996=EDGE_LOOP('',(#67892,#67893,#67894,#67895)) ;
#25997=EDGE_LOOP('',(#67896,#67897,#67898,#67899)) ;
#25998=EDGE_LOOP('',(#67900,#67901,#67902,#67903)) ;
#25999=EDGE_LOOP('',(#67904,#67905,#67906,#67907)) ;
#26000=EDGE_LOOP('',(#67908,#67909,#67910,#67911)) ;
#26001=EDGE_LOOP('',(#67912,#67913,#67914,#67915)) ;
#26002=EDGE_LOOP('',(#67916,#67917,#67918,#67919)) ;
#26003=EDGE_LOOP('',(#67920,#67921,#67922,#67923)) ;
#26004=EDGE_LOOP('',(#67924,#67925,#67926,#67927)) ;
#26005=EDGE_LOOP('',(#67928,#67929,#67930,#67931)) ;
#26006=EDGE_LOOP('',(#67932,#67933,#67934,#67935)) ;
#26007=EDGE_LOOP('',(#67936,#67937,#67938,#67939)) ;
#26008=EDGE_LOOP('',(#67940,#67941,#67942,#67943)) ;
#26009=EDGE_LOOP('',(#67944,#67945,#67946,#67947)) ;
#26010=EDGE_LOOP('',(#67948,#67949,#67950,#67951)) ;
#26011=EDGE_LOOP('',(#67952,#67953,#67954,#67955)) ;
#26012=EDGE_LOOP('',(#67956,#67957,#67958,#67959)) ;
#26013=EDGE_LOOP('',(#67960,#67961,#67962,#67963)) ;
#26014=EDGE_LOOP('',(#67964,#67965,#67966,#67967)) ;
#26015=EDGE_LOOP('',(#67968,#67969,#67970,#67971)) ;
#26016=EDGE_LOOP('',(#67972,#67973,#67974,#67975)) ;
#26017=EDGE_LOOP('',(#67976,#67977,#67978,#67979)) ;
#26018=EDGE_LOOP('',(#67980,#67981,#67982,#67983)) ;
#26019=EDGE_LOOP('',(#67984,#67985,#67986,#67987,#67988)) ;
#26020=EDGE_LOOP('',(#67989,#67990,#67991,#67992)) ;
#26021=EDGE_LOOP('',(#67993,#67994,#67995,#67996)) ;
#26022=EDGE_LOOP('',(#67997,#67998,#67999,#68000)) ;
#26023=EDGE_LOOP('',(#68001,#68002,#68003,#68004)) ;
#26024=EDGE_LOOP('',(#68005,#68006,#68007,#68008)) ;
#26025=EDGE_LOOP('',(#68009,#68010,#68011,#68012)) ;
#26026=EDGE_LOOP('',(#68013,#68014,#68015,#68016)) ;
#26027=EDGE_LOOP('',(#68017,#68018,#68019,#68020)) ;
#26028=EDGE_LOOP('',(#68021,#68022,#68023,#68024)) ;
#26029=EDGE_LOOP('',(#68025,#68026,#68027,#68028)) ;
#26030=EDGE_LOOP('',(#68029,#68030,#68031,#68032)) ;
#26031=EDGE_LOOP('',(#68033,#68034,#68035,#68036)) ;
#26032=EDGE_LOOP('',(#68037,#68038,#68039,#68040)) ;
#26033=EDGE_LOOP('',(#68041,#68042,#68043,#68044)) ;
#26034=EDGE_LOOP('',(#68045,#68046,#68047,#68048)) ;
#26035=EDGE_LOOP('',(#68049,#68050,#68051,#68052)) ;
#26036=EDGE_LOOP('',(#68053,#68054,#68055,#68056)) ;
#26037=EDGE_LOOP('',(#68057,#68058,#68059,#68060)) ;
#26038=EDGE_LOOP('',(#68061,#68062,#68063,#68064)) ;
#26039=EDGE_LOOP('',(#68065,#68066,#68067,#68068)) ;
#26040=EDGE_LOOP('',(#68069,#68070,#68071,#68072)) ;
#26041=EDGE_LOOP('',(#68073,#68074,#68075,#68076)) ;
#26042=EDGE_LOOP('',(#68077,#68078,#68079,#68080)) ;
#26043=EDGE_LOOP('',(#68081,#68082,#68083,#68084,#68085)) ;
#26044=EDGE_LOOP('',(#68086,#68087,#68088,#68089)) ;
#26045=EDGE_LOOP('',(#68090,#68091,#68092,#68093)) ;
#26046=EDGE_LOOP('',(#68094,#68095,#68096,#68097)) ;
#26047=EDGE_LOOP('',(#68098,#68099,#68100,#68101)) ;
#26048=EDGE_LOOP('',(#68102,#68103,#68104,#68105)) ;
#26049=EDGE_LOOP('',(#68106,#68107,#68108,#68109)) ;
#26050=EDGE_LOOP('',(#68110,#68111,#68112,#68113)) ;
#26051=EDGE_LOOP('',(#68114,#68115,#68116,#68117)) ;
#26052=EDGE_LOOP('',(#68118,#68119,#68120,#68121)) ;
#26053=EDGE_LOOP('',(#68122,#68123,#68124,#68125)) ;
#26054=EDGE_LOOP('',(#68126,#68127,#68128,#68129)) ;
#26055=EDGE_LOOP('',(#68130,#68131,#68132,#68133)) ;
#26056=EDGE_LOOP('',(#68134,#68135,#68136,#68137)) ;
#26057=EDGE_LOOP('',(#68138,#68139,#68140,#68141)) ;
#26058=EDGE_LOOP('',(#68142,#68143,#68144,#68145)) ;
#26059=EDGE_LOOP('',(#68146,#68147,#68148,#68149)) ;
#26060=EDGE_LOOP('',(#68150,#68151,#68152,#68153)) ;
#26061=EDGE_LOOP('',(#68154,#68155,#68156,#68157)) ;
#26062=EDGE_LOOP('',(#68158,#68159,#68160,#68161)) ;
#26063=EDGE_LOOP('',(#68162,#68163,#68164,#68165)) ;
#26064=EDGE_LOOP('',(#68166,#68167,#68168,#68169)) ;
#26065=EDGE_LOOP('',(#68170,#68171,#68172,#68173)) ;
#26066=EDGE_LOOP('',(#68174,#68175,#68176,#68177)) ;
#26067=EDGE_LOOP('',(#68178,#68179,#68180,#68181,#68182)) ;
#26068=EDGE_LOOP('',(#68183,#68184,#68185,#68186)) ;
#26069=EDGE_LOOP('',(#68187,#68188,#68189,#68190)) ;
#26070=EDGE_LOOP('',(#68191,#68192,#68193,#68194)) ;
#26071=EDGE_LOOP('',(#68195,#68196,#68197,#68198)) ;
#26072=EDGE_LOOP('',(#68199,#68200,#68201,#68202)) ;
#26073=EDGE_LOOP('',(#68203,#68204,#68205,#68206)) ;
#26074=EDGE_LOOP('',(#68207,#68208,#68209,#68210)) ;
#26075=EDGE_LOOP('',(#68211,#68212,#68213,#68214)) ;
#26076=EDGE_LOOP('',(#68215,#68216,#68217,#68218)) ;
#26077=EDGE_LOOP('',(#68219,#68220,#68221,#68222)) ;
#26078=EDGE_LOOP('',(#68223,#68224,#68225,#68226)) ;
#26079=EDGE_LOOP('',(#68227,#68228,#68229,#68230)) ;
#26080=EDGE_LOOP('',(#68231,#68232,#68233,#68234)) ;
#26081=EDGE_LOOP('',(#68235,#68236,#68237,#68238)) ;
#26082=EDGE_LOOP('',(#68239,#68240,#68241,#68242)) ;
#26083=EDGE_LOOP('',(#68243,#68244,#68245,#68246)) ;
#26084=EDGE_LOOP('',(#68247,#68248,#68249,#68250)) ;
#26085=EDGE_LOOP('',(#68251,#68252,#68253,#68254)) ;
#26086=EDGE_LOOP('',(#68255,#68256,#68257,#68258)) ;
#26087=EDGE_LOOP('',(#68259,#68260,#68261,#68262)) ;
#26088=EDGE_LOOP('',(#68263,#68264,#68265,#68266)) ;
#26089=EDGE_LOOP('',(#68267,#68268,#68269,#68270)) ;
#26090=EDGE_LOOP('',(#68271,#68272,#68273,#68274)) ;
#26091=EDGE_LOOP('',(#68275,#68276,#68277,#68278,#68279)) ;
#26092=EDGE_LOOP('',(#68280,#68281,#68282,#68283)) ;
#26093=EDGE_LOOP('',(#68284,#68285,#68286,#68287)) ;
#26094=EDGE_LOOP('',(#68288,#68289,#68290,#68291)) ;
#26095=EDGE_LOOP('',(#68292,#68293,#68294,#68295)) ;
#26096=EDGE_LOOP('',(#68296,#68297,#68298,#68299)) ;
#26097=EDGE_LOOP('',(#68300,#68301,#68302,#68303)) ;
#26098=EDGE_LOOP('',(#68304,#68305,#68306,#68307)) ;
#26099=EDGE_LOOP('',(#68308,#68309,#68310,#68311)) ;
#26100=EDGE_LOOP('',(#68312,#68313,#68314,#68315)) ;
#26101=EDGE_LOOP('',(#68316,#68317,#68318,#68319)) ;
#26102=EDGE_LOOP('',(#68320,#68321,#68322,#68323)) ;
#26103=EDGE_LOOP('',(#68324,#68325,#68326,#68327)) ;
#26104=EDGE_LOOP('',(#68328,#68329,#68330,#68331)) ;
#26105=EDGE_LOOP('',(#68332,#68333,#68334,#68335)) ;
#26106=EDGE_LOOP('',(#68336,#68337,#68338,#68339)) ;
#26107=EDGE_LOOP('',(#68340,#68341,#68342,#68343)) ;
#26108=EDGE_LOOP('',(#68344,#68345,#68346,#68347)) ;
#26109=EDGE_LOOP('',(#68348,#68349,#68350,#68351)) ;
#26110=EDGE_LOOP('',(#68352,#68353,#68354,#68355)) ;
#26111=EDGE_LOOP('',(#68356,#68357,#68358,#68359)) ;
#26112=EDGE_LOOP('',(#68360,#68361,#68362,#68363)) ;
#26113=EDGE_LOOP('',(#68364,#68365,#68366,#68367)) ;
#26114=EDGE_LOOP('',(#68368,#68369,#68370,#68371)) ;
#26115=EDGE_LOOP('',(#68372,#68373,#68374,#68375,#68376)) ;
#26116=EDGE_LOOP('',(#68377,#68378,#68379,#68380)) ;
#26117=EDGE_LOOP('',(#68381,#68382,#68383,#68384)) ;
#26118=EDGE_LOOP('',(#68385,#68386,#68387,#68388)) ;
#26119=EDGE_LOOP('',(#68389,#68390,#68391,#68392)) ;
#26120=EDGE_LOOP('',(#68393,#68394,#68395,#68396)) ;
#26121=EDGE_LOOP('',(#68397,#68398,#68399,#68400)) ;
#26122=EDGE_LOOP('',(#68401,#68402,#68403,#68404)) ;
#26123=EDGE_LOOP('',(#68405,#68406,#68407,#68408)) ;
#26124=EDGE_LOOP('',(#68409,#68410,#68411,#68412)) ;
#26125=EDGE_LOOP('',(#68413,#68414,#68415,#68416)) ;
#26126=EDGE_LOOP('',(#68417,#68418,#68419,#68420)) ;
#26127=EDGE_LOOP('',(#68421,#68422,#68423,#68424)) ;
#26128=EDGE_LOOP('',(#68425,#68426,#68427,#68428)) ;
#26129=EDGE_LOOP('',(#68429,#68430,#68431,#68432)) ;
#26130=EDGE_LOOP('',(#68433,#68434,#68435,#68436)) ;
#26131=EDGE_LOOP('',(#68437,#68438,#68439,#68440)) ;
#26132=EDGE_LOOP('',(#68441,#68442,#68443,#68444)) ;
#26133=EDGE_LOOP('',(#68445,#68446,#68447,#68448)) ;
#26134=EDGE_LOOP('',(#68449,#68450,#68451,#68452)) ;
#26135=EDGE_LOOP('',(#68453,#68454,#68455,#68456)) ;
#26136=EDGE_LOOP('',(#68457,#68458,#68459,#68460)) ;
#26137=EDGE_LOOP('',(#68461,#68462,#68463,#68464)) ;
#26138=EDGE_LOOP('',(#68465,#68466,#68467,#68468)) ;
#26139=EDGE_LOOP('',(#68469,#68470,#68471,#68472,#68473)) ;
#26140=EDGE_LOOP('',(#68474,#68475,#68476,#68477)) ;
#26141=EDGE_LOOP('',(#68478,#68479,#68480,#68481)) ;
#26142=EDGE_LOOP('',(#68482,#68483,#68484,#68485)) ;
#26143=EDGE_LOOP('',(#68486,#68487,#68488,#68489)) ;
#26144=EDGE_LOOP('',(#68490,#68491,#68492,#68493)) ;
#26145=EDGE_LOOP('',(#68494,#68495,#68496,#68497)) ;
#26146=EDGE_LOOP('',(#68498,#68499,#68500,#68501)) ;
#26147=EDGE_LOOP('',(#68502,#68503,#68504,#68505)) ;
#26148=EDGE_LOOP('',(#68506,#68507,#68508,#68509)) ;
#26149=EDGE_LOOP('',(#68510,#68511,#68512,#68513)) ;
#26150=EDGE_LOOP('',(#68514,#68515,#68516,#68517)) ;
#26151=EDGE_LOOP('',(#68518,#68519,#68520,#68521)) ;
#26152=EDGE_LOOP('',(#68522,#68523,#68524,#68525)) ;
#26153=EDGE_LOOP('',(#68526,#68527,#68528,#68529)) ;
#26154=EDGE_LOOP('',(#68530,#68531,#68532,#68533)) ;
#26155=EDGE_LOOP('',(#68534,#68535,#68536,#68537)) ;
#26156=EDGE_LOOP('',(#68538,#68539,#68540,#68541)) ;
#26157=EDGE_LOOP('',(#68542,#68543,#68544,#68545)) ;
#26158=EDGE_LOOP('',(#68546,#68547,#68548,#68549)) ;
#26159=EDGE_LOOP('',(#68550,#68551,#68552,#68553)) ;
#26160=EDGE_LOOP('',(#68554,#68555,#68556,#68557)) ;
#26161=EDGE_LOOP('',(#68558,#68559,#68560,#68561)) ;
#26162=EDGE_LOOP('',(#68562,#68563,#68564,#68565)) ;
#26163=EDGE_LOOP('',(#68566,#68567,#68568,#68569,#68570)) ;
#26164=EDGE_LOOP('',(#68571,#68572,#68573,#68574)) ;
#26165=EDGE_LOOP('',(#68575,#68576,#68577,#68578)) ;
#26166=EDGE_LOOP('',(#68579,#68580,#68581,#68582)) ;
#26167=EDGE_LOOP('',(#68583,#68584,#68585,#68586)) ;
#26168=EDGE_LOOP('',(#68587,#68588,#68589,#68590)) ;
#26169=EDGE_LOOP('',(#68591,#68592,#68593,#68594)) ;
#26170=EDGE_LOOP('',(#68595,#68596,#68597,#68598)) ;
#26171=EDGE_LOOP('',(#68599,#68600,#68601,#68602)) ;
#26172=EDGE_LOOP('',(#68603,#68604,#68605,#68606)) ;
#26173=EDGE_LOOP('',(#68607,#68608,#68609,#68610)) ;
#26174=EDGE_LOOP('',(#68611,#68612,#68613,#68614)) ;
#26175=EDGE_LOOP('',(#68615,#68616,#68617,#68618)) ;
#26176=EDGE_LOOP('',(#68619,#68620,#68621,#68622)) ;
#26177=EDGE_LOOP('',(#68623,#68624,#68625,#68626)) ;
#26178=EDGE_LOOP('',(#68627,#68628,#68629,#68630)) ;
#26179=EDGE_LOOP('',(#68631,#68632,#68633,#68634)) ;
#26180=EDGE_LOOP('',(#68635,#68636,#68637,#68638)) ;
#29733=CIRCLE('',#93350,0.899999999999998) ;
#29734=CIRCLE('',#93351,0.1) ;
#29735=CIRCLE('',#93352,1.) ;
#29736=CIRCLE('',#93353,1.) ;
#29737=CIRCLE('',#93355,1.1) ;
#29738=CIRCLE('',#93356,0.1) ;
#29739=CIRCLE('',#93357,1.) ;
#29740=CIRCLE('',#93359,0.100000000000003) ;
#29741=CIRCLE('',#93360,0.0999999999999999) ;
#29742=CIRCLE('',#93361,0.1) ;
#29743=CIRCLE('',#93364,0.1) ;
#29744=CIRCLE('',#93365,0.100000000000003) ;
#29745=CIRCLE('',#93367,0.899999999999998) ;
#29746=CIRCLE('',#93368,0.1) ;
#29747=CIRCLE('',#93369,1.) ;
#29748=CIRCLE('',#93370,1.) ;
#29749=CIRCLE('',#93372,1.1) ;
#29750=CIRCLE('',#93373,0.1) ;
#29751=CIRCLE('',#93374,1.) ;
#29752=CIRCLE('',#93376,0.0999999999999994) ;
#29753=CIRCLE('',#93377,0.1) ;
#29754=CIRCLE('',#93378,0.1) ;
#29755=CIRCLE('',#93381,0.1) ;
#29756=CIRCLE('',#93382,0.0999999999999994) ;
#29757=CIRCLE('',#93384,0.899999999999998) ;
#29758=CIRCLE('',#93385,0.1) ;
#29759=CIRCLE('',#93386,1.) ;
#29760=CIRCLE('',#93387,1.) ;
#29761=CIRCLE('',#93389,1.1) ;
#29762=CIRCLE('',#93390,0.1) ;
#29763=CIRCLE('',#93391,1.) ;
#29764=CIRCLE('',#93393,0.0999999999999994) ;
#29765=CIRCLE('',#93394,0.1) ;
#29766=CIRCLE('',#93395,0.1) ;
#29767=CIRCLE('',#93398,0.1) ;
#29768=CIRCLE('',#93399,0.0999999999999994) ;
#29769=CIRCLE('',#93401,0.899999999999998) ;
#29770=CIRCLE('',#93402,0.1) ;
#29771=CIRCLE('',#93403,1.) ;
#29772=CIRCLE('',#93404,1.) ;
#29773=CIRCLE('',#93406,1.1) ;
#29774=CIRCLE('',#93407,0.1) ;
#29775=CIRCLE('',#93408,1.) ;
#29776=CIRCLE('',#93410,0.0999999999999994) ;
#29777=CIRCLE('',#93411,0.1) ;
#29778=CIRCLE('',#93412,0.1) ;
#29779=CIRCLE('',#93415,0.1) ;
#29780=CIRCLE('',#93416,0.0999999999999994) ;
#29781=CIRCLE('',#93418,0.900000000000001) ;
#29782=CIRCLE('',#93419,0.1) ;
#29783=CIRCLE('',#93420,1.) ;
#29784=CIRCLE('',#93421,1.) ;
#29785=CIRCLE('',#93423,1.1) ;
#29786=CIRCLE('',#93424,0.1) ;
#29787=CIRCLE('',#93425,1.) ;
#29788=CIRCLE('',#93427,0.0999999999999994) ;
#29789=CIRCLE('',#93428,0.1) ;
#29790=CIRCLE('',#93429,0.1) ;
#29791=CIRCLE('',#93432,0.1) ;
#29792=CIRCLE('',#93433,0.0999999999999994) ;
#29793=CIRCLE('',#93435,0.900000000000001) ;
#29794=CIRCLE('',#93436,0.1) ;
#29795=CIRCLE('',#93437,1.) ;
#29796=CIRCLE('',#93438,1.) ;
#29797=CIRCLE('',#93440,1.1) ;
#29798=CIRCLE('',#93441,0.1) ;
#29799=CIRCLE('',#93442,0.999999999999999) ;
#29800=CIRCLE('',#93444,0.100000000000001) ;
#29801=CIRCLE('',#93445,0.1) ;
#29802=CIRCLE('',#93446,0.1) ;
#29803=CIRCLE('',#93449,0.1) ;
#29804=CIRCLE('',#93450,0.0999999999999994) ;
#29805=CIRCLE('',#93452,0.9) ;
#29806=CIRCLE('',#93453,0.1) ;
#29807=CIRCLE('',#93454,0.999999999999999) ;
#29808=CIRCLE('',#93455,0.999999999999999) ;
#29809=CIRCLE('',#93457,1.1) ;
#29810=CIRCLE('',#93458,0.1) ;
#29811=CIRCLE('',#93459,0.999999999999999) ;
#29812=CIRCLE('',#93461,0.100000000000001) ;
#29813=CIRCLE('',#93462,0.1) ;
#29814=CIRCLE('',#93463,0.1) ;
#29815=CIRCLE('',#93466,0.1) ;
#29816=CIRCLE('',#93467,0.0999999999999994) ;
#29817=CIRCLE('',#93469,0.9) ;
#29818=CIRCLE('',#93470,0.1) ;
#29819=CIRCLE('',#93471,0.999999999999999) ;
#29820=CIRCLE('',#93472,0.999999999999999) ;
#29821=CIRCLE('',#93474,1.1) ;
#29822=CIRCLE('',#93475,0.1) ;
#29823=CIRCLE('',#93476,1.) ;
#29824=CIRCLE('',#93478,0.1) ;
#29825=CIRCLE('',#93479,0.1) ;
#29826=CIRCLE('',#93480,0.1) ;
#29827=CIRCLE('',#93483,0.1) ;
#29828=CIRCLE('',#93484,0.0999999999999994) ;
#29829=CIRCLE('',#93486,0.9) ;
#29830=CIRCLE('',#93487,0.1) ;
#29831=CIRCLE('',#93488,1.) ;
#29832=CIRCLE('',#93489,1.) ;
#29833=CIRCLE('',#93491,0.200000000000001) ;
#29834=CIRCLE('',#93492,0.0999999999999994) ;
#29835=CIRCLE('',#93493,0.1) ;
#29836=CIRCLE('',#93494,0.1) ;
#29837=CIRCLE('',#93496,0.200000000000001) ;
#29838=CIRCLE('',#93497,0.0999999999999994) ;
#29839=CIRCLE('',#93498,0.100000000000001) ;
#29840=CIRCLE('',#93499,0.1) ;
#29841=CIRCLE('',#93501,0.200000000000001) ;
#29842=CIRCLE('',#93502,0.0999999999999994) ;
#29843=CIRCLE('',#93503,0.100000000000001) ;
#29844=CIRCLE('',#93504,0.1) ;
#29845=CIRCLE('',#93506,0.199999999999999) ;
#29846=CIRCLE('',#93507,0.0999999999999994) ;
#29847=CIRCLE('',#93508,0.0999999999999994) ;
#29848=CIRCLE('',#93509,0.0999999999999995) ;
#29849=CIRCLE('',#93511,0.199999999999999) ;
#29850=CIRCLE('',#93512,0.0999999999999994) ;
#29851=CIRCLE('',#93513,0.0999999999999994) ;
#29852=CIRCLE('',#93514,0.0999999999999995) ;
#29853=CIRCLE('',#93516,0.199999999999999) ;
#29854=CIRCLE('',#93517,0.0999999999999994) ;
#29855=CIRCLE('',#93518,0.0999999999999994) ;
#29856=CIRCLE('',#93519,0.0999999999999995) ;
#29857=CIRCLE('',#93521,0.199999999999999) ;
#29858=CIRCLE('',#93522,0.0999999999999994) ;
#29859=CIRCLE('',#93523,0.0999999999999994) ;
#29860=CIRCLE('',#93524,0.0999999999999995) ;
#29861=CIRCLE('',#93526,0.199999999999999) ;
#29862=CIRCLE('',#93527,0.0999999999999994) ;
#29863=CIRCLE('',#93528,0.100000000000003) ;
#29864=CIRCLE('',#93529,0.0999999999999995) ;
#29865=CIRCLE('',#93531,0.199999999999999) ;
#29866=CIRCLE('',#93532,0.0999999999999994) ;
#29867=CIRCLE('',#93533,0.100000000000003) ;
#29868=CIRCLE('',#93534,0.0999999999999995) ;
#29869=CIRCLE('',#93536,1.1) ;
#29870=CIRCLE('',#93537,0.1) ;
#29871=CIRCLE('',#93538,1.) ;
#29872=CIRCLE('',#93540,0.100000000000001) ;
#29873=CIRCLE('',#93541,0.0999999999999998) ;
#29874=CIRCLE('',#93542,0.1) ;
#29875=CIRCLE('',#93545,0.1) ;
#29876=CIRCLE('',#93546,0.1) ;
#29877=CIRCLE('',#93557,0.1) ;
#29878=CIRCLE('',#93559,0.100000000000001) ;
#29879=CIRCLE('',#93561,0.100000000000001) ;
#29880=CIRCLE('',#93563,0.0999999999999994) ;
#29881=CIRCLE('',#93565,0.0999999999999994) ;
#29882=CIRCLE('',#93567,0.0999999999999994) ;
#29883=CIRCLE('',#93569,0.0999999999999994) ;
#29884=CIRCLE('',#93571,0.100000000000003) ;
#29885=CIRCLE('',#93573,0.100000000000003) ;
#29886=CIRCLE('',#93575,0.9) ;
#29887=CIRCLE('',#93576,0.1) ;
#29888=CIRCLE('',#93577,1.) ;
#29889=CIRCLE('',#93578,1.) ;
#29890=CIRCLE('',#93580,0.200000000000001) ;
#29891=CIRCLE('',#93581,0.0999999999999994) ;
#29892=CIRCLE('',#93582,0.1) ;
#29893=CIRCLE('',#93583,0.1) ;
#29894=CIRCLE('',#93585,1.1) ;
#29895=CIRCLE('',#93586,0.1) ;
#29896=CIRCLE('',#93587,1.) ;
#29897=CIRCLE('',#93589,0.1) ;
#29898=CIRCLE('',#93590,0.1) ;
#29899=CIRCLE('',#93591,0.1) ;
#29900=CIRCLE('',#93594,0.1) ;
#29901=CIRCLE('',#93595,0.1) ;
#29902=CIRCLE('',#93598,0.1) ;
#29903=CIRCLE('',#93600,0.1) ;
#29904=CIRCLE('',#93601,0.1) ;
#29905=CIRCLE('',#93602,0.2) ;
#29906=CIRCLE('',#93603,0.2) ;
#29907=CIRCLE('',#93605,0.1) ;
#29908=CIRCLE('',#93606,0.1) ;
#29909=CIRCLE('',#93607,0.2) ;
#29910=CIRCLE('',#93608,0.2) ;
#29911=CIRCLE('',#93610,0.1) ;
#29912=CIRCLE('',#93611,0.1) ;
#29913=CIRCLE('',#93612,0.2) ;
#29914=CIRCLE('',#93613,0.2) ;
#29915=CIRCLE('',#93615,0.1) ;
#29916=CIRCLE('',#93616,0.1) ;
#29917=CIRCLE('',#93617,0.2) ;
#29918=CIRCLE('',#93618,0.2) ;
#29919=CIRCLE('',#93620,0.1) ;
#29920=CIRCLE('',#93621,0.1) ;
#29921=CIRCLE('',#93622,0.2) ;
#29922=CIRCLE('',#93623,0.2) ;
#29923=CIRCLE('',#93625,0.1) ;
#29924=CIRCLE('',#93626,0.1) ;
#29925=CIRCLE('',#93627,0.2) ;
#29926=CIRCLE('',#93628,0.2) ;
#29927=CIRCLE('',#93630,0.1) ;
#29928=CIRCLE('',#93631,0.1) ;
#29929=CIRCLE('',#93632,0.2) ;
#29930=CIRCLE('',#93633,0.2) ;
#29931=CIRCLE('',#93635,0.1) ;
#29932=CIRCLE('',#93636,0.1) ;
#29933=CIRCLE('',#93637,0.2) ;
#29934=CIRCLE('',#93638,0.2) ;
#29935=CIRCLE('',#93640,0.1) ;
#29936=CIRCLE('',#93641,0.1) ;
#29937=CIRCLE('',#93642,0.2) ;
#29938=CIRCLE('',#93643,0.2) ;
#29939=CIRCLE('',#93645,0.2) ;
#29940=CIRCLE('',#93647,0.2) ;
#29941=CIRCLE('',#93649,0.2) ;
#29942=CIRCLE('',#93651,0.2) ;
#29943=CIRCLE('',#93653,0.2) ;
#29944=CIRCLE('',#93655,0.2) ;
#29945=CIRCLE('',#93657,0.2) ;
#29946=CIRCLE('',#93659,0.2) ;
#29947=CIRCLE('',#93661,0.2) ;
#29948=CIRCLE('',#93663,0.2) ;
#29949=CIRCLE('',#93665,0.2) ;
#29950=CIRCLE('',#93667,0.2) ;
#29951=CIRCLE('',#93669,0.2) ;
#29952=CIRCLE('',#93671,0.2) ;
#29953=CIRCLE('',#93673,0.2) ;
#29954=CIRCLE('',#93675,0.2) ;
#29955=CIRCLE('',#93677,0.2) ;
#29956=CIRCLE('',#93679,0.2) ;
#29957=CIRCLE('',#93681,0.1) ;
#29958=CIRCLE('',#93682,0.1) ;
#29959=CIRCLE('',#93684,0.1) ;
#29960=CIRCLE('',#93685,0.1) ;
#29961=CIRCLE('',#93687,0.1) ;
#29962=CIRCLE('',#93688,0.1) ;
#29963=CIRCLE('',#93690,0.1) ;
#29964=CIRCLE('',#93691,0.1) ;
#29965=CIRCLE('',#93693,0.1) ;
#29966=CIRCLE('',#93694,0.1) ;
#29967=CIRCLE('',#93696,0.1) ;
#29968=CIRCLE('',#93697,0.1) ;
#29969=CIRCLE('',#93699,0.1) ;
#29970=CIRCLE('',#93700,0.1) ;
#29971=CIRCLE('',#93702,0.1) ;
#29972=CIRCLE('',#93703,0.1) ;
#29973=CIRCLE('',#93705,0.1) ;
#29974=CIRCLE('',#93706,0.1) ;
#29975=CIRCLE('',#93708,0.1) ;
#29976=CIRCLE('',#93709,0.1) ;
#29977=CIRCLE('',#93710,0.2) ;
#29978=CIRCLE('',#93711,0.2) ;
#29979=CIRCLE('',#93713,0.2) ;
#29980=CIRCLE('',#93715,0.2) ;
#29981=CIRCLE('',#93717,0.1) ;
#29982=CIRCLE('',#93718,0.1) ;
#29983=CIRCLE('',#93720,0.0999999999999994) ;
#29984=CIRCLE('',#93721,0.0999999999999994) ;
#29985=CIRCLE('',#93723,0.199999999999999) ;
#29986=CIRCLE('',#93724,0.2) ;
#29987=CIRCLE('',#93725,0.2) ;
#29988=CIRCLE('',#93726,0.2) ;
#29989=CIRCLE('',#93727,0.2) ;
#29990=CIRCLE('',#93728,0.2) ;
#29991=CIRCLE('',#93729,0.200000000000001) ;
#29992=CIRCLE('',#93730,0.200000000000001) ;
#29993=CIRCLE('',#93731,0.200000000000001) ;
#29994=CIRCLE('',#93732,0.200000000000001) ;
#29995=CIRCLE('',#93733,0.199999999999999) ;
#29996=CIRCLE('',#93734,0.199999999999999) ;
#29997=CIRCLE('',#93735,0.199999999999999) ;
#29998=CIRCLE('',#93736,0.199999999999999) ;
#29999=CIRCLE('',#93737,0.199999999999999) ;
#30000=CIRCLE('',#93738,0.199999999999999) ;
#30001=CIRCLE('',#93739,0.199999999999999) ;
#30002=CIRCLE('',#93740,0.199999999999999) ;
#30003=CIRCLE('',#93741,0.199999999999999) ;
#30004=CIRCLE('',#93742,0.199999999999999) ;
#30005=CIRCLE('',#93744,0.1) ;
#30006=CIRCLE('',#93745,0.1) ;
#30007=CIRCLE('',#93747,0.2) ;
#30008=CIRCLE('',#93748,0.2) ;
#30009=CIRCLE('',#93749,0.2) ;
#30010=CIRCLE('',#93750,0.2) ;
#30011=CIRCLE('',#93751,0.2) ;
#30012=CIRCLE('',#93752,0.2) ;
#30013=CIRCLE('',#93753,0.2) ;
#30014=CIRCLE('',#93754,0.2) ;
#30015=CIRCLE('',#93755,0.2) ;
#30016=CIRCLE('',#93756,0.2) ;
#30017=CIRCLE('',#93757,0.2) ;
#30018=CIRCLE('',#93758,0.2) ;
#30019=CIRCLE('',#93759,0.2) ;
#30020=CIRCLE('',#93760,0.2) ;
#30021=CIRCLE('',#93761,0.2) ;
#30022=CIRCLE('',#93762,0.2) ;
#30023=CIRCLE('',#93763,0.2) ;
#30024=CIRCLE('',#93764,0.2) ;
#30025=CIRCLE('',#93765,0.2) ;
#30026=CIRCLE('',#93766,0.2) ;
#30027=CIRCLE('',#93768,0.1) ;
#30028=CIRCLE('',#93769,0.1) ;
#30029=CIRCLE('',#93772,0.1) ;
#30030=CIRCLE('',#93773,0.1) ;
#30031=CIRCLE('',#93776,0.1) ;
#30032=CIRCLE('',#93777,0.1) ;
#30033=CIRCLE('',#93780,0.100000000000001) ;
#30034=CIRCLE('',#93781,0.100000000000001) ;
#30035=CIRCLE('',#93784,0.1) ;
#30036=CIRCLE('',#93785,0.1) ;
#30037=CIRCLE('',#93788,0.0999999999999994) ;
#30038=CIRCLE('',#93789,0.0999999999999994) ;
#30039=CIRCLE('',#93791,0.199999999999999) ;
#30040=CIRCLE('',#93792,0.199999999999999) ;
#30041=CIRCLE('',#93793,0.199999999999999) ;
#30042=CIRCLE('',#93794,0.199999999999999) ;
#30043=CIRCLE('',#93795,0.199999999999999) ;
#30044=CIRCLE('',#93796,0.199999999999999) ;
#30045=CIRCLE('',#93797,0.199999999999999) ;
#30046=CIRCLE('',#93798,1.55625) ;
#30047=CIRCLE('',#93799,0.199999999999999) ;
#30048=CIRCLE('',#93800,0.199999999999999) ;
#30049=CIRCLE('',#93801,0.199999999999999) ;
#30050=CIRCLE('',#93802,0.199999999999999) ;
#30051=CIRCLE('',#93803,0.199999999999999) ;
#30052=CIRCLE('',#93804,0.199999999999999) ;
#30053=CIRCLE('',#93805,0.199999999999999) ;
#30054=CIRCLE('',#93806,0.199999999999999) ;
#30055=CIRCLE('',#93807,0.199999999999999) ;
#30056=CIRCLE('',#93808,1.55625) ;
#30057=CIRCLE('',#93809,0.199999999999999) ;
#30058=CIRCLE('',#93810,0.199999999999999) ;
#30059=CIRCLE('',#93811,0.199999999999999) ;
#30060=CIRCLE('',#93812,0.199999999999999) ;
#30061=CIRCLE('',#93813,0.199999999999999) ;
#30062=CIRCLE('',#93814,0.199999999999999) ;
#30063=CIRCLE('',#93815,0.199999999999999) ;
#30064=CIRCLE('',#93816,0.199999999999999) ;
#30065=CIRCLE('',#93817,0.199999999999999) ;
#30066=CIRCLE('',#93818,1.55625) ;
#30067=CIRCLE('',#93819,0.199999999999999) ;
#30068=CIRCLE('',#93820,0.199999999999999) ;
#30069=CIRCLE('',#93821,0.199999999999999) ;
#30070=CIRCLE('',#93822,0.199999999999999) ;
#30071=CIRCLE('',#93823,0.199999999999999) ;
#30072=CIRCLE('',#93824,0.199999999999999) ;
#30073=CIRCLE('',#93825,0.199999999999999) ;
#30074=CIRCLE('',#93826,0.199999999999999) ;
#30075=CIRCLE('',#93827,0.199999999999999) ;
#30076=CIRCLE('',#93828,1.55625) ;
#30077=CIRCLE('',#93829,0.199999999999999) ;
#30078=CIRCLE('',#93830,0.199999999999999) ;
#30079=CIRCLE('',#93831,0.199999999999999) ;
#30080=CIRCLE('',#93832,0.199999999999999) ;
#30081=CIRCLE('',#93833,0.199999999999999) ;
#30082=CIRCLE('',#93834,0.199999999999999) ;
#30083=CIRCLE('',#93835,0.199999999999999) ;
#30084=CIRCLE('',#93836,0.199999999999999) ;
#30085=CIRCLE('',#93837,0.199999999999999) ;
#30086=CIRCLE('',#93838,1.55625) ;
#30087=CIRCLE('',#93839,0.199999999999999) ;
#30088=CIRCLE('',#93840,0.199999999999999) ;
#30089=CIRCLE('',#93841,0.200000000000001) ;
#30090=CIRCLE('',#93842,0.199999999999999) ;
#30091=CIRCLE('',#93843,0.200000000000001) ;
#30092=CIRCLE('',#93844,0.199999999999999) ;
#30093=CIRCLE('',#93845,0.199999999999999) ;
#30094=CIRCLE('',#93846,0.199999999999999) ;
#30095=CIRCLE('',#93847,0.199999999999999) ;
#30096=CIRCLE('',#93848,1.55625) ;
#30097=CIRCLE('',#93849,0.200000000000001) ;
#30098=CIRCLE('',#93850,0.200000000000001) ;
#30099=CIRCLE('',#93851,0.200000000000001) ;
#30100=CIRCLE('',#93852,0.199999999999999) ;
#30101=CIRCLE('',#93853,0.200000000000001) ;
#30102=CIRCLE('',#93854,0.200000000000001) ;
#30103=CIRCLE('',#93855,0.200000000000001) ;
#30104=CIRCLE('',#93856,0.200000000000001) ;
#30105=CIRCLE('',#93857,0.200000000000001) ;
#30106=CIRCLE('',#93858,1.55625) ;
#30107=CIRCLE('',#93859,0.200000000000001) ;
#30108=CIRCLE('',#93860,0.200000000000001) ;
#30109=CIRCLE('',#93861,0.2) ;
#30110=CIRCLE('',#93862,0.2) ;
#30111=CIRCLE('',#93863,0.200000000000001) ;
#30112=CIRCLE('',#93864,0.200000000000001) ;
#30113=CIRCLE('',#93865,0.200000000000001) ;
#30114=CIRCLE('',#93866,0.200000000000001) ;
#30115=CIRCLE('',#93867,0.200000000000001) ;
#30116=CIRCLE('',#93868,1.55625) ;
#30117=CIRCLE('',#93869,0.2) ;
#30118=CIRCLE('',#93870,0.2) ;
#30119=CIRCLE('',#93871,0.2) ;
#30120=CIRCLE('',#93872,0.199999999999999) ;
#30121=CIRCLE('',#93873,0.200000000000001) ;
#30122=CIRCLE('',#93874,0.200000000000001) ;
#30123=CIRCLE('',#93875,0.2) ;
#30124=CIRCLE('',#93876,0.2) ;
#30125=CIRCLE('',#93877,0.2) ;
#30126=CIRCLE('',#93878,1.55625) ;
#30127=CIRCLE('',#93879,0.2) ;
#30128=CIRCLE('',#93880,0.2) ;
#30129=CIRCLE('',#93881,0.2) ;
#30130=CIRCLE('',#93882,0.199999999999999) ;
#30131=CIRCLE('',#93883,0.200000000000001) ;
#30132=CIRCLE('',#93884,0.2) ;
#30133=CIRCLE('',#93885,0.2) ;
#30134=CIRCLE('',#93886,0.2) ;
#30135=CIRCLE('',#93887,0.2) ;
#30136=CIRCLE('',#93888,1.55625) ;
#30137=CIRCLE('',#93889,0.2) ;
#30138=CIRCLE('',#93890,0.2) ;
#30139=CIRCLE('',#93892,0.200000000000001) ;
#30140=CIRCLE('',#93893,0.200000000000001) ;
#30141=CIRCLE('',#93895,0.200000000000001) ;
#30142=CIRCLE('',#93896,0.200000000000001) ;
#30143=CIRCLE('',#93898,0.2) ;
#30144=CIRCLE('',#93899,0.2) ;
#30145=CIRCLE('',#93906,0.1) ;
#30146=CIRCLE('',#93907,0.1) ;
#30147=CIRCLE('',#93910,0.1) ;
#30148=CIRCLE('',#93911,0.1) ;
#30149=CIRCLE('',#93914,0.0999999999999994) ;
#30150=CIRCLE('',#93915,0.0999999999999994) ;
#30151=CIRCLE('',#93918,0.1) ;
#30152=CIRCLE('',#93922,0.1) ;
#30153=CIRCLE('',#93923,0.1) ;
#30154=CIRCLE('',#93926,0.1) ;
#30155=CIRCLE('',#93927,0.1) ;
#30156=CIRCLE('',#93930,0.1) ;
#30157=CIRCLE('',#93931,0.1) ;
#30158=CIRCLE('',#93934,0.1) ;
#30159=CIRCLE('',#93935,0.1) ;
#30160=CIRCLE('',#93938,0.1) ;
#30161=CIRCLE('',#93939,0.1) ;
#30162=CIRCLE('',#93942,0.1) ;
#30163=CIRCLE('',#93943,0.1) ;
#30164=CIRCLE('',#93945,1.65625) ;
#30165=CIRCLE('',#93946,1.65625) ;
#30166=CIRCLE('',#93948,0.1) ;
#30167=CIRCLE('',#93949,0.1) ;
#30168=CIRCLE('',#93952,0.1) ;
#30169=CIRCLE('',#93953,0.1) ;
#30170=CIRCLE('',#93956,0.1) ;
#30171=CIRCLE('',#93957,0.1) ;
#30172=CIRCLE('',#93960,0.2) ;
#30173=CIRCLE('',#93961,0.2) ;
#30174=CIRCLE('',#93962,1.75625) ;
#30175=CIRCLE('',#93963,0.2) ;
#30176=CIRCLE('',#93964,0.2) ;
#30177=CIRCLE('',#93966,0.1) ;
#30178=CIRCLE('',#93967,0.1) ;
#30179=CIRCLE('',#93968,0.1) ;
#30180=CIRCLE('',#93969,0.1) ;
#30181=CIRCLE('',#93971,0.1) ;
#30182=CIRCLE('',#93972,0.1) ;
#30183=CIRCLE('',#93974,0.1) ;
#30184=CIRCLE('',#93975,0.1) ;
#30185=CIRCLE('',#93977,0.1) ;
#30186=CIRCLE('',#93978,0.1) ;
#30187=CIRCLE('',#93980,0.1) ;
#30188=CIRCLE('',#93981,0.0999999999999998) ;
#30189=CIRCLE('',#93983,0.1) ;
#30190=CIRCLE('',#93985,0.1) ;
#30191=CIRCLE('',#93987,0.1) ;
#30192=CIRCLE('',#93989,0.1) ;
#30193=CIRCLE('',#93991,0.0999999999999998) ;
#30194=CIRCLE('',#93993,0.1) ;
#30195=CIRCLE('',#93995,0.1) ;
#30196=CIRCLE('',#93996,0.1) ;
#30197=CIRCLE('',#93999,0.1) ;
#30198=CIRCLE('',#94001,0.1) ;
#30199=CIRCLE('',#94002,0.1) ;
#30200=CIRCLE('',#94004,0.1) ;
#30201=CIRCLE('',#94006,0.1) ;
#30202=CIRCLE('',#94008,0.1) ;
#30203=CIRCLE('',#94010,0.1) ;
#30204=CIRCLE('',#94012,0.1) ;
#30205=CIRCLE('',#94014,0.1) ;
#30206=CIRCLE('',#94015,0.1) ;
#30207=CIRCLE('',#94017,0.1) ;
#30208=CIRCLE('',#94019,0.1) ;
#30209=CIRCLE('',#94021,0.0999999999999998) ;
#30210=CIRCLE('',#94022,0.1) ;
#30211=CIRCLE('',#94024,0.1) ;
#30212=CIRCLE('',#94026,0.1) ;
#30213=CIRCLE('',#94027,0.1) ;
#30214=CIRCLE('',#94029,0.1) ;
#30215=CIRCLE('',#94031,0.1) ;
#30216=CIRCLE('',#94033,0.1) ;
#30217=CIRCLE('',#94035,0.1) ;
#30218=CIRCLE('',#94037,0.1) ;
#30219=CIRCLE('',#94039,0.1) ;
#30220=CIRCLE('',#94041,0.1) ;
#30221=CIRCLE('',#94043,0.1) ;
#30222=CIRCLE('',#94044,0.1) ;
#30223=CIRCLE('',#94046,0.1) ;
#30224=CIRCLE('',#94048,0.1) ;
#30225=CIRCLE('',#94050,0.1) ;
#30226=CIRCLE('',#94052,0.1) ;
#30227=CIRCLE('',#94053,0.1) ;
#30228=CIRCLE('',#94055,0.1) ;
#30229=CIRCLE('',#94057,0.1) ;
#30230=CIRCLE('',#94059,0.1) ;
#30231=CIRCLE('',#94061,0.1) ;
#30232=CIRCLE('',#94064,0.1) ;
#30233=CIRCLE('',#94066,0.1) ;
#30234=CIRCLE('',#94068,0.1) ;
#30235=CIRCLE('',#94071,0.100000000000003) ;
#30236=CIRCLE('',#94072,0.100000000000003) ;
#30237=CIRCLE('',#94074,0.100000000000003) ;
#30238=CIRCLE('',#94076,0.100000000000003) ;
#30239=CIRCLE('',#94078,0.1) ;
#30240=CIRCLE('',#94080,0.100000000000003) ;
#30241=CIRCLE('',#94082,0.100000000000003) ;
#30242=CIRCLE('',#94084,0.1) ;
#30243=CIRCLE('',#94086,0.1) ;
#30244=CIRCLE('',#94088,0.1) ;
#30245=CIRCLE('',#94090,0.100000000000003) ;
#30246=CIRCLE('',#94092,0.100000000000003) ;
#30247=CIRCLE('',#94094,0.0999999999999998) ;
#30248=CIRCLE('',#94096,0.100000000000003) ;
#30249=CIRCLE('',#94098,0.100000000000003) ;
#30250=CIRCLE('',#94100,0.0999999999999994) ;
#30251=CIRCLE('',#94103,0.0999999999999998) ;
#30252=CIRCLE('',#94104,0.0999999999999998) ;
#30253=CIRCLE('',#94106,0.0999999999999998) ;
#30254=CIRCLE('',#94108,0.0999999999999998) ;
#30255=CIRCLE('',#94110,0.0999999999999998) ;
#30256=CIRCLE('',#94112,0.0999999999999998) ;
#30257=CIRCLE('',#94114,0.1) ;
#30258=CIRCLE('',#94116,0.1) ;
#30259=CIRCLE('',#94118,0.1) ;
#30260=CIRCLE('',#94120,0.1) ;
#30261=CIRCLE('',#94122,0.1) ;
#30262=CIRCLE('',#94124,0.0999999999999998) ;
#30263=CIRCLE('',#94126,0.0999999999999998) ;
#30264=CIRCLE('',#94128,0.0999999999999998) ;
#30265=CIRCLE('',#94130,0.0999999999999998) ;
#30266=CIRCLE('',#94132,0.0999999999999998) ;
#30267=CIRCLE('',#94135,0.1) ;
#30268=CIRCLE('',#94136,0.1) ;
#30269=CIRCLE('',#94138,0.1) ;
#30270=CIRCLE('',#94140,0.1) ;
#30271=CIRCLE('',#94142,0.1) ;
#30272=CIRCLE('',#94144,0.1) ;
#30273=CIRCLE('',#94146,0.1) ;
#30274=CIRCLE('',#94148,0.0999999999999998) ;
#30275=CIRCLE('',#94150,0.0999999999999998) ;
#30276=CIRCLE('',#94152,0.1) ;
#30277=CIRCLE('',#94154,0.1) ;
#30278=CIRCLE('',#94156,0.1) ;
#30279=CIRCLE('',#94158,0.1) ;
#30280=CIRCLE('',#94160,0.1) ;
#30281=CIRCLE('',#94162,0.1) ;
#30282=CIRCLE('',#94164,0.1) ;
#30283=CIRCLE('',#94167,0.1) ;
#30284=CIRCLE('',#94169,0.1) ;
#30285=CIRCLE('',#94171,0.1) ;
#30286=CIRCLE('',#94173,0.1) ;
#30287=CIRCLE('',#94175,0.0999999999999998) ;
#30288=CIRCLE('',#94177,0.1) ;
#30289=CIRCLE('',#94179,0.1) ;
#30290=CIRCLE('',#94181,0.1) ;
#30291=CIRCLE('',#94183,0.1) ;
#30292=CIRCLE('',#94185,0.1) ;
#30293=CIRCLE('',#94188,0.1) ;
#30294=CIRCLE('',#94189,0.1) ;
#30295=CIRCLE('',#94191,0.0999999999999998) ;
#30296=CIRCLE('',#94193,0.1) ;
#30297=CIRCLE('',#94195,0.1) ;
#30298=CIRCLE('',#94197,0.0999999999999998) ;
#30299=CIRCLE('',#94199,0.1) ;
#30300=CIRCLE('',#94201,0.1) ;
#30301=CIRCLE('',#94204,0.1) ;
#30302=CIRCLE('',#94206,0.0999999999999994) ;
#30303=CIRCLE('',#94208,0.0999999999999994) ;
#30304=CIRCLE('',#94210,0.0999999999999994) ;
#30305=CIRCLE('',#94212,0.1) ;
#30306=CIRCLE('',#94214,0.1) ;
#30307=CIRCLE('',#94216,0.1) ;
#30308=CIRCLE('',#94218,0.1) ;
#30309=CIRCLE('',#94220,0.0999999999999998) ;
#30310=CIRCLE('',#94222,0.0999999999999994) ;
#30311=CIRCLE('',#94224,0.0999999999999998) ;
#30312=CIRCLE('',#94226,0.0999999999999998) ;
#30313=CIRCLE('',#94228,0.1) ;
#30314=CIRCLE('',#94230,0.1) ;
#30315=CIRCLE('',#94232,0.1) ;
#30316=CIRCLE('',#94234,0.1) ;
#30317=CIRCLE('',#94236,0.0999999999999994) ;
#30318=CIRCLE('',#94238,0.1) ;
#30319=CIRCLE('',#94246,0.3) ;
#30320=CIRCLE('',#94247,0.9) ;
#30321=CIRCLE('',#94249,0.9) ;
#30322=CIRCLE('',#94250,0.3) ;
#30323=CIRCLE('',#94252,1.) ;
#30324=CIRCLE('',#94253,1.) ;
#30325=CIRCLE('',#94255,0.2) ;
#30326=CIRCLE('',#94256,0.2) ;
#30327=CIRCLE('',#94269,0.1) ;
#30328=CIRCLE('',#94270,0.1) ;
#30329=CIRCLE('',#94272,0.1) ;
#30330=CIRCLE('',#94273,0.1) ;
#30331=CIRCLE('',#94275,0.1) ;
#30332=CIRCLE('',#94276,0.1) ;
#30333=CIRCLE('',#94278,0.1) ;
#30334=CIRCLE('',#94279,0.1) ;
#30335=CIRCLE('',#94281,0.1) ;
#30336=CIRCLE('',#94283,0.1) ;
#30337=CIRCLE('',#94285,0.1) ;
#30338=CIRCLE('',#94287,0.1) ;
#30339=CIRCLE('',#94288,0.1) ;
#30340=CIRCLE('',#94290,0.1) ;
#30341=CIRCLE('',#94292,0.1) ;
#30342=CIRCLE('',#94294,0.1) ;
#30343=CIRCLE('',#94296,0.1) ;
#30344=CIRCLE('',#94298,0.1) ;
#30345=CIRCLE('',#94299,0.1) ;
#30346=CIRCLE('',#94301,0.1) ;
#30347=CIRCLE('',#94303,0.1) ;
#30348=CIRCLE('',#94304,0.1) ;
#30349=CIRCLE('',#94306,0.1) ;
#30350=CIRCLE('',#94307,0.1) ;
#30351=CIRCLE('',#94309,0.1) ;
#30352=CIRCLE('',#94310,0.1) ;
#30353=CIRCLE('',#94312,0.1) ;
#30354=CIRCLE('',#94313,0.1) ;
#30355=CIRCLE('',#94315,0.1) ;
#30356=CIRCLE('',#94317,0.1) ;
#30357=CIRCLE('',#94319,0.1) ;
#30358=CIRCLE('',#94321,0.1) ;
#30359=CIRCLE('',#94322,0.1) ;
#30360=CIRCLE('',#94324,0.1) ;
#30361=CIRCLE('',#94326,0.1) ;
#30362=CIRCLE('',#94328,0.1) ;
#30363=CIRCLE('',#94330,0.1) ;
#30364=CIRCLE('',#94332,0.1) ;
#30365=CIRCLE('',#94333,0.1) ;
#30366=CIRCLE('',#94335,0.1) ;
#30367=CIRCLE('',#94337,0.1) ;
#30368=CIRCLE('',#94339,0.1) ;
#30369=CIRCLE('',#94341,0.1) ;
#30370=CIRCLE('',#94343,0.1) ;
#30371=CIRCLE('',#94345,0.1) ;
#30372=CIRCLE('',#94347,0.1) ;
#30373=CIRCLE('',#94350,0.1) ;
#30374=CIRCLE('',#94352,0.1) ;
#30375=CIRCLE('',#94354,0.1) ;
#30376=CIRCLE('',#94356,0.1) ;
#30377=CIRCLE('',#94358,0.1) ;
#30378=CIRCLE('',#94360,0.1) ;
#30379=CIRCLE('',#94363,0.1) ;
#30380=CIRCLE('',#94365,0.1) ;
#30381=CIRCLE('',#94367,0.1) ;
#30382=CIRCLE('',#94369,0.1) ;
#30383=CIRCLE('',#94372,0.1) ;
#30384=CIRCLE('',#94374,0.1) ;
#30385=CIRCLE('',#94376,0.1) ;
#30386=CIRCLE('',#94378,0.1) ;
#30387=CIRCLE('',#94381,0.2) ;
#30388=CIRCLE('',#94382,0.2) ;
#30389=CIRCLE('',#94384,0.2) ;
#30390=CIRCLE('',#94385,0.2) ;
#30391=CIRCLE('',#94387,0.2) ;
#30392=CIRCLE('',#94388,0.2) ;
#30393=CIRCLE('',#94390,0.2) ;
#30394=CIRCLE('',#94391,0.2) ;
#30395=CIRCLE('',#94393,0.2) ;
#30396=CIRCLE('',#94394,0.2) ;
#30397=CIRCLE('',#94396,0.2) ;
#30398=CIRCLE('',#94397,0.2) ;
#30399=CIRCLE('',#94399,0.2) ;
#30400=CIRCLE('',#94400,0.2) ;
#30401=CIRCLE('',#94402,0.2) ;
#30402=CIRCLE('',#94403,0.2) ;
#30403=CIRCLE('',#94405,0.2) ;
#30404=CIRCLE('',#94406,0.2) ;
#30405=CIRCLE('',#94453,0.100000000000003) ;
#30406=CIRCLE('',#94454,0.100000000000003) ;
#30407=CIRCLE('',#94457,0.100000000000003) ;
#30408=CIRCLE('',#94458,0.100000000000003) ;
#30409=CIRCLE('',#94461,0.0999999999999959) ;
#30410=CIRCLE('',#94462,0.0999999999999959) ;
#30411=CIRCLE('',#94465,0.100000000000003) ;
#30412=CIRCLE('',#94469,0.100000000000003) ;
#30413=CIRCLE('',#94470,0.100000000000003) ;
#30414=CIRCLE('',#94473,0.100000000000003) ;
#30415=CIRCLE('',#94474,0.100000000000003) ;
#30416=CIRCLE('',#94477,0.100000000000003) ;
#30417=CIRCLE('',#94478,0.100000000000003) ;
#30418=CIRCLE('',#94481,0.100000000000003) ;
#30419=CIRCLE('',#94482,0.100000000000003) ;
#30420=CIRCLE('',#94485,0.100000000000003) ;
#30421=CIRCLE('',#94486,0.100000000000003) ;
#30422=CIRCLE('',#94489,0.100000000000003) ;
#30423=CIRCLE('',#94490,0.100000000000003) ;
#30424=CIRCLE('',#94492,1.65625) ;
#30425=CIRCLE('',#94493,1.65625) ;
#30426=CIRCLE('',#94495,0.100000000000003) ;
#30427=CIRCLE('',#94496,0.100000000000003) ;
#30428=CIRCLE('',#94499,0.100000000000003) ;
#30429=CIRCLE('',#94500,0.100000000000003) ;
#30430=CIRCLE('',#94503,0.100000000000003) ;
#30431=CIRCLE('',#94504,0.100000000000003) ;
#30432=CIRCLE('',#94507,0.199999999999999) ;
#30433=CIRCLE('',#94508,0.199999999999999) ;
#30434=CIRCLE('',#94509,1.75625) ;
#30435=CIRCLE('',#94510,0.199999999999999) ;
#30436=CIRCLE('',#94511,0.199999999999999) ;
#30437=CIRCLE('',#94513,0.0999999999999994) ;
#30438=CIRCLE('',#94514,0.0999999999999994) ;
#30439=CIRCLE('',#94517,0.0999999999999994) ;
#30440=CIRCLE('',#94518,0.0999999999999994) ;
#30441=CIRCLE('',#94521,0.0999999999999994) ;
#30442=CIRCLE('',#94522,0.0999999999999994) ;
#30443=CIRCLE('',#94525,0.0999999999999994) ;
#30444=CIRCLE('',#94529,0.100000000000003) ;
#30445=CIRCLE('',#94530,0.100000000000003) ;
#30446=CIRCLE('',#94533,0.0999999999999994) ;
#30447=CIRCLE('',#94534,0.0999999999999994) ;
#30448=CIRCLE('',#94537,0.0999999999999994) ;
#30449=CIRCLE('',#94538,0.0999999999999994) ;
#30450=CIRCLE('',#94541,0.100000000000003) ;
#30451=CIRCLE('',#94542,0.100000000000003) ;
#30452=CIRCLE('',#94545,0.100000000000003) ;
#30453=CIRCLE('',#94546,0.100000000000003) ;
#30454=CIRCLE('',#94549,0.100000000000003) ;
#30455=CIRCLE('',#94550,0.100000000000003) ;
#30456=CIRCLE('',#94552,1.65625) ;
#30457=CIRCLE('',#94553,1.65625) ;
#30458=CIRCLE('',#94555,0.0999999999999994) ;
#30459=CIRCLE('',#94556,0.0999999999999994) ;
#30460=CIRCLE('',#94559,0.0999999999999994) ;
#30461=CIRCLE('',#94560,0.0999999999999994) ;
#30462=CIRCLE('',#94563,0.0999999999999994) ;
#30463=CIRCLE('',#94564,0.0999999999999994) ;
#30464=CIRCLE('',#94567,0.199999999999999) ;
#30465=CIRCLE('',#94568,0.199999999999999) ;
#30466=CIRCLE('',#94569,1.75625) ;
#30467=CIRCLE('',#94570,0.199999999999999) ;
#30468=CIRCLE('',#94571,0.199999999999999) ;
#30469=CIRCLE('',#94573,0.0999999999999994) ;
#30470=CIRCLE('',#94574,0.0999999999999994) ;
#30471=CIRCLE('',#94577,0.0999999999999994) ;
#30472=CIRCLE('',#94578,0.0999999999999994) ;
#30473=CIRCLE('',#94581,0.0999999999999994) ;
#30474=CIRCLE('',#94582,0.0999999999999994) ;
#30475=CIRCLE('',#94585,0.0999999999999994) ;
#30476=CIRCLE('',#94589,0.0999999999999994) ;
#30477=CIRCLE('',#94590,0.0999999999999994) ;
#30478=CIRCLE('',#94593,0.0999999999999994) ;
#30479=CIRCLE('',#94594,0.0999999999999994) ;
#30480=CIRCLE('',#94597,0.0999999999999994) ;
#30481=CIRCLE('',#94598,0.0999999999999994) ;
#30482=CIRCLE('',#94601,0.0999999999999994) ;
#30483=CIRCLE('',#94602,0.0999999999999994) ;
#30484=CIRCLE('',#94605,0.0999999999999994) ;
#30485=CIRCLE('',#94606,0.0999999999999994) ;
#30486=CIRCLE('',#94609,0.0999999999999994) ;
#30487=CIRCLE('',#94610,0.0999999999999994) ;
#30488=CIRCLE('',#94612,1.65625) ;
#30489=CIRCLE('',#94613,1.65625) ;
#30490=CIRCLE('',#94615,0.0999999999999994) ;
#30491=CIRCLE('',#94616,0.0999999999999994) ;
#30492=CIRCLE('',#94619,0.0999999999999994) ;
#30493=CIRCLE('',#94620,0.0999999999999994) ;
#30494=CIRCLE('',#94623,0.0999999999999994) ;
#30495=CIRCLE('',#94624,0.0999999999999994) ;
#30496=CIRCLE('',#94627,0.199999999999999) ;
#30497=CIRCLE('',#94628,0.199999999999999) ;
#30498=CIRCLE('',#94629,1.75625) ;
#30499=CIRCLE('',#94630,0.199999999999999) ;
#30500=CIRCLE('',#94631,0.199999999999999) ;
#30501=CIRCLE('',#94633,0.0999999999999994) ;
#30502=CIRCLE('',#94634,0.0999999999999994) ;
#30503=CIRCLE('',#94637,0.0999999999999994) ;
#30504=CIRCLE('',#94638,0.0999999999999994) ;
#30505=CIRCLE('',#94641,0.0999999999999994) ;
#30506=CIRCLE('',#94642,0.0999999999999994) ;
#30507=CIRCLE('',#94645,0.0999999999999994) ;
#30508=CIRCLE('',#94649,0.0999999999999994) ;
#30509=CIRCLE('',#94650,0.0999999999999994) ;
#30510=CIRCLE('',#94653,0.0999999999999994) ;
#30511=CIRCLE('',#94654,0.0999999999999994) ;
#30512=CIRCLE('',#94657,0.0999999999999994) ;
#30513=CIRCLE('',#94658,0.0999999999999994) ;
#30514=CIRCLE('',#94661,0.0999999999999994) ;
#30515=CIRCLE('',#94662,0.0999999999999994) ;
#30516=CIRCLE('',#94665,0.0999999999999994) ;
#30517=CIRCLE('',#94666,0.0999999999999994) ;
#30518=CIRCLE('',#94669,0.0999999999999994) ;
#30519=CIRCLE('',#94670,0.0999999999999994) ;
#30520=CIRCLE('',#94672,1.65625) ;
#30521=CIRCLE('',#94673,1.65625) ;
#30522=CIRCLE('',#94675,0.0999999999999994) ;
#30523=CIRCLE('',#94676,0.0999999999999994) ;
#30524=CIRCLE('',#94679,0.0999999999999994) ;
#30525=CIRCLE('',#94680,0.0999999999999994) ;
#30526=CIRCLE('',#94683,0.0999999999999994) ;
#30527=CIRCLE('',#94684,0.0999999999999994) ;
#30528=CIRCLE('',#94687,0.199999999999999) ;
#30529=CIRCLE('',#94688,0.199999999999999) ;
#30530=CIRCLE('',#94689,1.75625) ;
#30531=CIRCLE('',#94690,0.199999999999999) ;
#30532=CIRCLE('',#94691,0.199999999999999) ;
#30533=CIRCLE('',#94693,0.0999999999999994) ;
#30534=CIRCLE('',#94694,0.0999999999999994) ;
#30535=CIRCLE('',#94697,0.0999999999999994) ;
#30536=CIRCLE('',#94698,0.0999999999999994) ;
#30537=CIRCLE('',#94701,0.0999999999999994) ;
#30538=CIRCLE('',#94702,0.0999999999999994) ;
#30539=CIRCLE('',#94705,0.0999999999999994) ;
#30540=CIRCLE('',#94709,0.0999999999999994) ;
#30541=CIRCLE('',#94710,0.0999999999999994) ;
#30542=CIRCLE('',#94713,0.0999999999999994) ;
#30543=CIRCLE('',#94714,0.0999999999999994) ;
#30544=CIRCLE('',#94717,0.0999999999999994) ;
#30545=CIRCLE('',#94718,0.0999999999999994) ;
#30546=CIRCLE('',#94721,0.0999999999999994) ;
#30547=CIRCLE('',#94722,0.0999999999999994) ;
#30548=CIRCLE('',#94725,0.0999999999999994) ;
#30549=CIRCLE('',#94726,0.0999999999999994) ;
#30550=CIRCLE('',#94729,0.0999999999999994) ;
#30551=CIRCLE('',#94730,0.0999999999999994) ;
#30552=CIRCLE('',#94732,1.65625) ;
#30553=CIRCLE('',#94733,1.65625) ;
#30554=CIRCLE('',#94735,0.0999999999999994) ;
#30555=CIRCLE('',#94736,0.0999999999999994) ;
#30556=CIRCLE('',#94739,0.0999999999999994) ;
#30557=CIRCLE('',#94740,0.0999999999999994) ;
#30558=CIRCLE('',#94743,0.0999999999999994) ;
#30559=CIRCLE('',#94744,0.0999999999999994) ;
#30560=CIRCLE('',#94747,0.199999999999999) ;
#30561=CIRCLE('',#94748,0.199999999999999) ;
#30562=CIRCLE('',#94749,1.75625) ;
#30563=CIRCLE('',#94750,0.199999999999999) ;
#30564=CIRCLE('',#94751,0.199999999999999) ;
#30565=CIRCLE('',#94753,0.0999999999999994) ;
#30566=CIRCLE('',#94754,0.0999999999999994) ;
#30567=CIRCLE('',#94757,0.0999999999999994) ;
#30568=CIRCLE('',#94758,0.0999999999999994) ;
#30569=CIRCLE('',#94761,0.0999999999999994) ;
#30570=CIRCLE('',#94762,0.0999999999999994) ;
#30571=CIRCLE('',#94765,0.100000000000001) ;
#30572=CIRCLE('',#94769,0.0999999999999994) ;
#30573=CIRCLE('',#94770,0.0999999999999994) ;
#30574=CIRCLE('',#94773,0.0999999999999994) ;
#30575=CIRCLE('',#94774,0.0999999999999994) ;
#30576=CIRCLE('',#94777,0.0999999999999994) ;
#30577=CIRCLE('',#94778,0.0999999999999994) ;
#30578=CIRCLE('',#94781,0.0999999999999994) ;
#30579=CIRCLE('',#94782,0.0999999999999994) ;
#30580=CIRCLE('',#94785,0.0999999999999994) ;
#30581=CIRCLE('',#94786,0.0999999999999994) ;
#30582=CIRCLE('',#94789,0.0999999999999994) ;
#30583=CIRCLE('',#94790,0.0999999999999994) ;
#30584=CIRCLE('',#94792,1.65625) ;
#30585=CIRCLE('',#94793,1.65625) ;
#30586=CIRCLE('',#94795,0.0999999999999994) ;
#30587=CIRCLE('',#94796,0.0999999999999994) ;
#30588=CIRCLE('',#94799,0.0999999999999994) ;
#30589=CIRCLE('',#94800,0.0999999999999994) ;
#30590=CIRCLE('',#94803,0.0999999999999994) ;
#30591=CIRCLE('',#94804,0.0999999999999994) ;
#30592=CIRCLE('',#94807,0.200000000000001) ;
#30593=CIRCLE('',#94808,0.200000000000001) ;
#30594=CIRCLE('',#94809,1.75625) ;
#30595=CIRCLE('',#94810,0.199999999999999) ;
#30596=CIRCLE('',#94811,0.199999999999999) ;
#30597=CIRCLE('',#94813,0.0999999999999994) ;
#30598=CIRCLE('',#94814,0.0999999999999994) ;
#30599=CIRCLE('',#94817,0.0999999999999994) ;
#30600=CIRCLE('',#94818,0.0999999999999994) ;
#30601=CIRCLE('',#94821,0.0999999999999994) ;
#30602=CIRCLE('',#94822,0.0999999999999994) ;
#30603=CIRCLE('',#94825,0.100000000000001) ;
#30604=CIRCLE('',#94829,0.100000000000001) ;
#30605=CIRCLE('',#94830,0.100000000000001) ;
#30606=CIRCLE('',#94833,0.0999999999999994) ;
#30607=CIRCLE('',#94834,0.0999999999999994) ;
#30608=CIRCLE('',#94837,0.0999999999999994) ;
#30609=CIRCLE('',#94838,0.0999999999999994) ;
#30610=CIRCLE('',#94841,0.0999999999999994) ;
#30611=CIRCLE('',#94842,0.0999999999999994) ;
#30612=CIRCLE('',#94845,0.0999999999999994) ;
#30613=CIRCLE('',#94846,0.0999999999999994) ;
#30614=CIRCLE('',#94849,0.0999999999999994) ;
#30615=CIRCLE('',#94850,0.0999999999999994) ;
#30616=CIRCLE('',#94852,1.65625) ;
#30617=CIRCLE('',#94853,1.65625) ;
#30618=CIRCLE('',#94855,0.0999999999999994) ;
#30619=CIRCLE('',#94856,0.0999999999999994) ;
#30620=CIRCLE('',#94859,0.0999999999999994) ;
#30621=CIRCLE('',#94860,0.0999999999999994) ;
#30622=CIRCLE('',#94863,0.0999999999999994) ;
#30623=CIRCLE('',#94864,0.0999999999999994) ;
#30624=CIRCLE('',#94867,0.200000000000001) ;
#30625=CIRCLE('',#94868,0.200000000000001) ;
#30626=CIRCLE('',#94869,1.75625) ;
#30627=CIRCLE('',#94870,0.200000000000001) ;
#30628=CIRCLE('',#94871,0.200000000000001) ;
#30629=CIRCLE('',#94873,0.1) ;
#30630=CIRCLE('',#94874,0.1) ;
#30631=CIRCLE('',#94877,0.1) ;
#30632=CIRCLE('',#94878,0.1) ;
#30633=CIRCLE('',#94881,0.0999999999999994) ;
#30634=CIRCLE('',#94882,0.0999999999999994) ;
#30635=CIRCLE('',#94885,0.1) ;
#30636=CIRCLE('',#94889,0.100000000000001) ;
#30637=CIRCLE('',#94890,0.100000000000001) ;
#30638=CIRCLE('',#94893,0.0999999999999994) ;
#30639=CIRCLE('',#94894,0.0999999999999994) ;
#30640=CIRCLE('',#94897,0.0999999999999994) ;
#30641=CIRCLE('',#94898,0.0999999999999994) ;
#30642=CIRCLE('',#94901,0.0999999999999994) ;
#30643=CIRCLE('',#94902,0.0999999999999994) ;
#30644=CIRCLE('',#94905,0.0999999999999994) ;
#30645=CIRCLE('',#94906,0.0999999999999994) ;
#30646=CIRCLE('',#94909,0.0999999999999994) ;
#30647=CIRCLE('',#94910,0.0999999999999994) ;
#30648=CIRCLE('',#94912,1.65625) ;
#30649=CIRCLE('',#94913,1.65625) ;
#30650=CIRCLE('',#94915,0.1) ;
#30651=CIRCLE('',#94916,0.1) ;
#30652=CIRCLE('',#94919,0.1) ;
#30653=CIRCLE('',#94920,0.1) ;
#30654=CIRCLE('',#94923,0.1) ;
#30655=CIRCLE('',#94924,0.1) ;
#30656=CIRCLE('',#94927,0.2) ;
#30657=CIRCLE('',#94928,0.2) ;
#30658=CIRCLE('',#94929,1.75625) ;
#30659=CIRCLE('',#94930,0.200000000000001) ;
#30660=CIRCLE('',#94931,0.200000000000001) ;
#30661=CIRCLE('',#94933,0.0999999999999998) ;
#30662=CIRCLE('',#94934,0.0999999999999998) ;
#30663=CIRCLE('',#94937,0.0999999999999998) ;
#30664=CIRCLE('',#94938,0.0999999999999998) ;
#30665=CIRCLE('',#94941,0.0999999999999994) ;
#30666=CIRCLE('',#94942,0.0999999999999994) ;
#30667=CIRCLE('',#94945,0.100000000000001) ;
#30668=CIRCLE('',#94949,0.1) ;
#30669=CIRCLE('',#94950,0.1) ;
#30670=CIRCLE('',#94953,0.1) ;
#30671=CIRCLE('',#94954,0.1) ;
#30672=CIRCLE('',#94957,0.1) ;
#30673=CIRCLE('',#94958,0.1) ;
#30674=CIRCLE('',#94961,0.1) ;
#30675=CIRCLE('',#94962,0.1) ;
#30676=CIRCLE('',#94965,0.1) ;
#30677=CIRCLE('',#94966,0.1) ;
#30678=CIRCLE('',#94969,0.1) ;
#30679=CIRCLE('',#94970,0.1) ;
#30680=CIRCLE('',#94972,1.65625) ;
#30681=CIRCLE('',#94973,1.65625) ;
#30682=CIRCLE('',#94975,0.0999999999999998) ;
#30683=CIRCLE('',#94976,0.0999999999999998) ;
#30684=CIRCLE('',#94979,0.0999999999999998) ;
#30685=CIRCLE('',#94980,0.0999999999999998) ;
#30686=CIRCLE('',#94983,0.1) ;
#30687=CIRCLE('',#94984,0.1) ;
#30688=CIRCLE('',#94987,0.2) ;
#30689=CIRCLE('',#94988,0.2) ;
#30690=CIRCLE('',#94989,1.75625) ;
#30691=CIRCLE('',#94990,0.2) ;
#30692=CIRCLE('',#94991,0.2) ;
#30693=CIRCLE('',#94993,0.0999999999999998) ;
#30694=CIRCLE('',#94994,0.1) ;
#30695=CIRCLE('',#94995,0.1) ;
#30696=CIRCLE('',#94996,0.0999999999999998) ;
#30697=CIRCLE('',#94998,0.1) ;
#30698=CIRCLE('',#94999,0.0999999999999994) ;
#30699=CIRCLE('',#95000,0.0999999999999994) ;
#30700=CIRCLE('',#95001,0.1) ;
#30701=CIRCLE('',#95003,0.0999999999999994) ;
#30702=CIRCLE('',#95004,0.0999999999999994) ;
#30703=CIRCLE('',#95005,0.0999999999999994) ;
#30704=CIRCLE('',#95006,0.0999999999999994) ;
#30705=CIRCLE('',#95008,0.0999999999999994) ;
#30706=CIRCLE('',#95009,0.0999999999999994) ;
#30707=CIRCLE('',#95010,0.0999999999999994) ;
#30708=CIRCLE('',#95011,0.0999999999999994) ;
#30709=CIRCLE('',#95013,0.0999999999999994) ;
#30710=CIRCLE('',#95014,0.0999999999999994) ;
#30711=CIRCLE('',#95015,0.0999999999999994) ;
#30712=CIRCLE('',#95016,0.0999999999999994) ;
#30713=CIRCLE('',#95018,0.0999999999999994) ;
#30714=CIRCLE('',#95019,0.0999999999999994) ;
#30715=CIRCLE('',#95020,0.0999999999999994) ;
#30716=CIRCLE('',#95021,0.0999999999999994) ;
#30717=CIRCLE('',#95023,0.0999999999999994) ;
#30718=CIRCLE('',#95024,0.0999999999999994) ;
#30719=CIRCLE('',#95025,0.0999999999999994) ;
#30720=CIRCLE('',#95026,0.0999999999999994) ;
#30721=CIRCLE('',#95028,0.0999999999999994) ;
#30722=CIRCLE('',#95029,0.0999999999999994) ;
#30723=CIRCLE('',#95030,0.0999999999999994) ;
#30724=CIRCLE('',#95031,0.0999999999999994) ;
#30725=CIRCLE('',#95033,0.100000000000003) ;
#30726=CIRCLE('',#95034,0.100000000000003) ;
#30727=CIRCLE('',#95035,0.100000000000003) ;
#30728=CIRCLE('',#95036,0.100000000000003) ;
#30729=CIRCLE('',#95038,0.0999999999999998) ;
#30730=CIRCLE('',#95039,0.0999999999999998) ;
#30731=CIRCLE('',#95041,0.0999999999999998) ;
#30732=CIRCLE('',#95042,0.1) ;
#30733=CIRCLE('',#95044,0.0999999999999998) ;
#30734=CIRCLE('',#95045,0.1) ;
#30735=CIRCLE('',#95047,0.1) ;
#30736=CIRCLE('',#95048,0.0999999999999998) ;
#30737=CIRCLE('',#95050,0.1) ;
#30738=CIRCLE('',#95052,0.1) ;
#30739=CIRCLE('',#95054,0.0999999999999998) ;
#30740=CIRCLE('',#95056,0.1) ;
#30741=CIRCLE('',#95058,0.0999999999999998) ;
#30742=CIRCLE('',#95060,0.1) ;
#30743=CIRCLE('',#95062,0.1) ;
#30744=CIRCLE('',#95063,0.1) ;
#30745=CIRCLE('',#95066,0.1) ;
#30746=CIRCLE('',#95068,0.0999999999999998) ;
#30747=CIRCLE('',#95069,0.0999999999999998) ;
#30748=CIRCLE('',#95071,0.1) ;
#30749=CIRCLE('',#95073,0.1) ;
#30750=CIRCLE('',#95075,0.0999999999999998) ;
#30751=CIRCLE('',#95077,0.0999999999999998) ;
#30752=CIRCLE('',#95079,0.1) ;
#30753=CIRCLE('',#95081,0.1) ;
#30754=CIRCLE('',#95082,0.1) ;
#30755=CIRCLE('',#95084,0.1) ;
#30756=CIRCLE('',#95086,0.0999999999999998) ;
#30757=CIRCLE('',#95088,0.0999999999999998) ;
#30758=CIRCLE('',#95089,0.1) ;
#30759=CIRCLE('',#95091,0.0999999999999998) ;
#30760=CIRCLE('',#95093,0.1) ;
#30761=CIRCLE('',#95094,0.1) ;
#30762=CIRCLE('',#95096,0.1) ;
#30763=CIRCLE('',#95098,0.1) ;
#30764=CIRCLE('',#95100,0.0999999999999998) ;
#30765=CIRCLE('',#95102,0.0999999999999998) ;
#30766=CIRCLE('',#95104,0.1) ;
#30767=CIRCLE('',#95106,0.1) ;
#30768=CIRCLE('',#95108,0.1) ;
#30769=CIRCLE('',#95110,0.1) ;
#30770=CIRCLE('',#95111,0.1) ;
#30771=CIRCLE('',#95113,0.1) ;
#30772=CIRCLE('',#95115,0.1) ;
#30773=CIRCLE('',#95117,0.1) ;
#30774=CIRCLE('',#95119,0.1) ;
#30775=CIRCLE('',#95120,0.1) ;
#30776=CIRCLE('',#95122,0.1) ;
#30777=CIRCLE('',#95124,0.1) ;
#30778=CIRCLE('',#95126,0.1) ;
#30779=CIRCLE('',#95128,0.1) ;
#30780=CIRCLE('',#95131,0.1) ;
#30781=CIRCLE('',#95133,0.1) ;
#30782=CIRCLE('',#95135,0.1) ;
#30783=CIRCLE('',#95138,0.1) ;
#30784=CIRCLE('',#95139,0.1) ;
#30785=CIRCLE('',#95141,0.1) ;
#30786=CIRCLE('',#95143,0.1) ;
#30787=CIRCLE('',#95145,0.1) ;
#30788=CIRCLE('',#95147,0.1) ;
#30789=CIRCLE('',#95149,0.1) ;
#30790=CIRCLE('',#95151,0.1) ;
#30791=CIRCLE('',#95153,0.1) ;
#30792=CIRCLE('',#95155,0.1) ;
#30793=CIRCLE('',#95157,0.1) ;
#30794=CIRCLE('',#95159,0.1) ;
#30795=CIRCLE('',#95161,0.0999999999999998) ;
#30796=CIRCLE('',#95163,0.1) ;
#30797=CIRCLE('',#95165,0.1) ;
#30798=CIRCLE('',#95167,0.1) ;
#30799=CIRCLE('',#95170,0.1) ;
#30800=CIRCLE('',#95172,0.0999999999999998) ;
#30801=CIRCLE('',#95174,0.0999999999999998) ;
#30802=CIRCLE('',#95176,0.0999999999999998) ;
#30803=CIRCLE('',#95178,0.1) ;
#30804=CIRCLE('',#95180,0.1) ;
#30805=CIRCLE('',#95182,0.1) ;
#30806=CIRCLE('',#95184,0.1) ;
#30807=CIRCLE('',#95186,0.0999999999999998) ;
#30808=CIRCLE('',#95188,0.0999999999999998) ;
#30809=CIRCLE('',#95191,0.100000000000003) ;
#30810=CIRCLE('',#95192,0.100000000000003) ;
#30811=CIRCLE('',#95194,0.1) ;
#30812=CIRCLE('',#95196,0.1) ;
#30813=CIRCLE('',#95198,0.1) ;
#30814=CIRCLE('',#95200,0.0999999999999998) ;
#30815=CIRCLE('',#95202,0.0999999999999998) ;
#30816=CIRCLE('',#95204,0.100000000000003) ;
#30817=CIRCLE('',#95207,0.100000000000003) ;
#30818=CIRCLE('',#95209,0.0999999999999994) ;
#30819=CIRCLE('',#95211,0.0999999999999994) ;
#30820=CIRCLE('',#95213,0.0999999999999994) ;
#30821=CIRCLE('',#95215,0.0999999999999998) ;
#30822=CIRCLE('',#95217,0.1) ;
#30823=CIRCLE('',#95219,0.0999999999999995) ;
#30824=CIRCLE('',#95221,0.1) ;
#30825=CIRCLE('',#95223,0.1) ;
#30826=CIRCLE('',#95225,0.0999999999999994) ;
#30827=CIRCLE('',#95227,0.1) ;
#30828=CIRCLE('',#95229,0.0999999999999998) ;
#30829=CIRCLE('',#95231,0.100000000000003) ;
#30830=CIRCLE('',#95233,0.100000000000003) ;
#30831=CIRCLE('',#95235,0.100000000000003) ;
#30832=CIRCLE('',#95237,0.100000000000003) ;
#30833=CIRCLE('',#95239,0.0999999999999994) ;
#30834=CIRCLE('',#95241,0.1) ;
#30835=CIRCLE('',#95244,0.0999999999999994) ;
#30836=CIRCLE('',#95245,0.0999999999999994) ;
#30837=CIRCLE('',#95247,0.1) ;
#30838=CIRCLE('',#95249,0.1) ;
#30839=CIRCLE('',#95251,0.1) ;
#30840=CIRCLE('',#95253,0.1) ;
#30841=CIRCLE('',#95255,0.0999999999999998) ;
#30842=CIRCLE('',#95257,0.100000000000003) ;
#30843=CIRCLE('',#95260,0.100000000000003) ;
#30844=CIRCLE('',#95262,0.0999999999999994) ;
#30845=CIRCLE('',#95264,0.0999999999999994) ;
#30846=CIRCLE('',#95266,0.0999999999999994) ;
#30847=CIRCLE('',#95268,0.1) ;
#30848=CIRCLE('',#95270,0.1) ;
#30849=CIRCLE('',#95272,0.0999999999999995) ;
#30850=CIRCLE('',#95274,0.1) ;
#30851=CIRCLE('',#95276,0.1) ;
#30852=CIRCLE('',#95278,0.0999999999999994) ;
#30853=CIRCLE('',#95280,0.1) ;
#30854=CIRCLE('',#95282,0.0999999999999994) ;
#30855=CIRCLE('',#95284,0.0999999999999994) ;
#30856=CIRCLE('',#95286,0.0999999999999994) ;
#30857=CIRCLE('',#95288,0.0999999999999994) ;
#30858=CIRCLE('',#95290,0.0999999999999994) ;
#30859=CIRCLE('',#95292,0.0999999999999994) ;
#30860=CIRCLE('',#95294,0.1) ;
#30861=CIRCLE('',#95297,0.0999999999999994) ;
#30862=CIRCLE('',#95298,0.0999999999999994) ;
#30863=CIRCLE('',#95300,0.1) ;
#30864=CIRCLE('',#95302,0.1) ;
#30865=CIRCLE('',#95304,0.1) ;
#30866=CIRCLE('',#95306,0.1) ;
#30867=CIRCLE('',#95308,0.1) ;
#30868=CIRCLE('',#95310,0.0999999999999994) ;
#30869=CIRCLE('',#95313,0.0999999999999994) ;
#30870=CIRCLE('',#95315,0.0999999999999994) ;
#30871=CIRCLE('',#95317,0.0999999999999994) ;
#30872=CIRCLE('',#95319,0.0999999999999994) ;
#30873=CIRCLE('',#95321,0.1) ;
#30874=CIRCLE('',#95323,0.1) ;
#30875=CIRCLE('',#95325,0.0999999999999995) ;
#30876=CIRCLE('',#95327,0.1) ;
#30877=CIRCLE('',#95329,0.1) ;
#30878=CIRCLE('',#95331,0.0999999999999994) ;
#30879=CIRCLE('',#95333,0.1) ;
#30880=CIRCLE('',#95335,0.0999999999999994) ;
#30881=CIRCLE('',#95337,0.0999999999999994) ;
#30882=CIRCLE('',#95339,0.0999999999999994) ;
#30883=CIRCLE('',#95341,0.0999999999999994) ;
#30884=CIRCLE('',#95343,0.0999999999999994) ;
#30885=CIRCLE('',#95345,0.0999999999999994) ;
#30886=CIRCLE('',#95347,0.1) ;
#30887=CIRCLE('',#95350,0.0999999999999994) ;
#30888=CIRCLE('',#95351,0.0999999999999994) ;
#30889=CIRCLE('',#95353,0.1) ;
#30890=CIRCLE('',#95355,0.1) ;
#30891=CIRCLE('',#95357,0.1) ;
#30892=CIRCLE('',#95359,0.1) ;
#30893=CIRCLE('',#95361,0.1) ;
#30894=CIRCLE('',#95363,0.0999999999999994) ;
#30895=CIRCLE('',#95366,0.0999999999999994) ;
#30896=CIRCLE('',#95368,0.0999999999999994) ;
#30897=CIRCLE('',#95370,0.0999999999999994) ;
#30898=CIRCLE('',#95372,0.0999999999999994) ;
#30899=CIRCLE('',#95374,0.1) ;
#30900=CIRCLE('',#95376,0.1) ;
#30901=CIRCLE('',#95378,0.0999999999999995) ;
#30902=CIRCLE('',#95380,0.1) ;
#30903=CIRCLE('',#95382,0.1) ;
#30904=CIRCLE('',#95384,0.0999999999999994) ;
#30905=CIRCLE('',#95386,0.1) ;
#30906=CIRCLE('',#95388,0.0999999999999994) ;
#30907=CIRCLE('',#95390,0.0999999999999994) ;
#30908=CIRCLE('',#95392,0.0999999999999994) ;
#30909=CIRCLE('',#95394,0.0999999999999994) ;
#30910=CIRCLE('',#95396,0.0999999999999994) ;
#30911=CIRCLE('',#95398,0.0999999999999994) ;
#30912=CIRCLE('',#95400,0.1) ;
#30913=CIRCLE('',#95403,0.0999999999999994) ;
#30914=CIRCLE('',#95404,0.0999999999999994) ;
#30915=CIRCLE('',#95406,0.1) ;
#30916=CIRCLE('',#95408,0.1) ;
#30917=CIRCLE('',#95410,0.1) ;
#30918=CIRCLE('',#95412,0.1) ;
#30919=CIRCLE('',#95414,0.1) ;
#30920=CIRCLE('',#95416,0.0999999999999994) ;
#30921=CIRCLE('',#95419,0.0999999999999994) ;
#30922=CIRCLE('',#95421,0.0999999999999994) ;
#30923=CIRCLE('',#95423,0.0999999999999994) ;
#30924=CIRCLE('',#95425,0.0999999999999994) ;
#30925=CIRCLE('',#95427,0.1) ;
#30926=CIRCLE('',#95429,0.1) ;
#30927=CIRCLE('',#95431,0.0999999999999995) ;
#30928=CIRCLE('',#95433,0.1) ;
#30929=CIRCLE('',#95435,0.1) ;
#30930=CIRCLE('',#95437,0.0999999999999994) ;
#30931=CIRCLE('',#95439,0.1) ;
#30932=CIRCLE('',#95441,0.0999999999999994) ;
#30933=CIRCLE('',#95443,0.0999999999999994) ;
#30934=CIRCLE('',#95445,0.0999999999999994) ;
#30935=CIRCLE('',#95447,0.0999999999999994) ;
#30936=CIRCLE('',#95449,0.0999999999999994) ;
#30937=CIRCLE('',#95451,0.0999999999999994) ;
#30938=CIRCLE('',#95453,0.1) ;
#30939=CIRCLE('',#95456,0.0999999999999994) ;
#30940=CIRCLE('',#95457,0.0999999999999994) ;
#30941=CIRCLE('',#95459,0.1) ;
#30942=CIRCLE('',#95461,0.1) ;
#30943=CIRCLE('',#95463,0.1) ;
#30944=CIRCLE('',#95465,0.1) ;
#30945=CIRCLE('',#95467,0.1) ;
#30946=CIRCLE('',#95469,0.0999999999999994) ;
#30947=CIRCLE('',#95472,0.0999999999999994) ;
#30948=CIRCLE('',#95474,0.0999999999999994) ;
#30949=CIRCLE('',#95476,0.0999999999999994) ;
#30950=CIRCLE('',#95478,0.0999999999999994) ;
#30951=CIRCLE('',#95480,0.1) ;
#30952=CIRCLE('',#95482,0.1) ;
#30953=CIRCLE('',#95484,0.1) ;
#30954=CIRCLE('',#95486,0.1) ;
#30955=CIRCLE('',#95488,0.1) ;
#30956=CIRCLE('',#95490,0.0999999999999994) ;
#30957=CIRCLE('',#95492,0.1) ;
#30958=CIRCLE('',#95494,0.0999999999999994) ;
#30959=CIRCLE('',#95496,0.0999999999999994) ;
#30960=CIRCLE('',#95498,0.0999999999999994) ;
#30961=CIRCLE('',#95500,0.0999999999999994) ;
#30962=CIRCLE('',#95502,0.0999999999999994) ;
#30963=CIRCLE('',#95504,0.0999999999999994) ;
#30964=CIRCLE('',#95506,0.1) ;
#30965=CIRCLE('',#95509,0.0999999999999994) ;
#30966=CIRCLE('',#95510,0.0999999999999994) ;
#30967=CIRCLE('',#95512,0.1) ;
#30968=CIRCLE('',#95514,0.1) ;
#30969=CIRCLE('',#95516,0.1) ;
#30970=CIRCLE('',#95518,0.1) ;
#30971=CIRCLE('',#95520,0.1) ;
#30972=CIRCLE('',#95522,0.0999999999999994) ;
#30973=CIRCLE('',#95525,0.0999999999999994) ;
#30974=CIRCLE('',#95527,0.0999999999999994) ;
#30975=CIRCLE('',#95529,0.0999999999999994) ;
#30976=CIRCLE('',#95531,0.0999999999999994) ;
#30977=CIRCLE('',#95533,0.1) ;
#30978=CIRCLE('',#95535,0.1) ;
#30979=CIRCLE('',#95537,0.1) ;
#30980=CIRCLE('',#95539,0.1) ;
#30981=CIRCLE('',#95541,0.1) ;
#30982=CIRCLE('',#95543,0.0999999999999994) ;
#30983=CIRCLE('',#95545,0.1) ;
#30984=CIRCLE('',#95547,0.0999999999999994) ;
#30985=CIRCLE('',#95549,0.0999999999999994) ;
#30986=CIRCLE('',#95551,0.0999999999999994) ;
#30987=CIRCLE('',#95553,0.0999999999999994) ;
#30988=CIRCLE('',#95555,0.0999999999999994) ;
#30989=CIRCLE('',#95557,0.0999999999999994) ;
#30990=CIRCLE('',#95559,0.1) ;
#30991=CIRCLE('',#95562,0.0999999999999994) ;
#30992=CIRCLE('',#95563,0.0999999999999994) ;
#30993=CIRCLE('',#95565,0.1) ;
#30994=CIRCLE('',#95567,0.1) ;
#30995=CIRCLE('',#95569,0.1) ;
#30996=CIRCLE('',#95571,0.1) ;
#30997=CIRCLE('',#95573,0.1) ;
#30998=CIRCLE('',#95575,0.0999999999999994) ;
#30999=CIRCLE('',#95578,0.0999999999999994) ;
#31000=CIRCLE('',#95580,0.0999999999999994) ;
#31001=CIRCLE('',#95582,0.0999999999999994) ;
#31002=CIRCLE('',#95584,0.0999999999999994) ;
#31003=CIRCLE('',#95586,0.1) ;
#31004=CIRCLE('',#95588,0.1) ;
#31005=CIRCLE('',#95590,0.1) ;
#31006=CIRCLE('',#95592,0.1) ;
#31007=CIRCLE('',#95594,0.0999999999999998) ;
#31008=CIRCLE('',#95596,0.0999999999999994) ;
#31009=CIRCLE('',#95598,0.1) ;
#31010=CIRCLE('',#95600,0.0999999999999994) ;
#31011=CIRCLE('',#95602,0.1) ;
#31012=CIRCLE('',#95604,0.1) ;
#31013=CIRCLE('',#95606,0.1) ;
#31014=CIRCLE('',#95608,0.1) ;
#31015=CIRCLE('',#95610,0.0999999999999994) ;
#31016=CIRCLE('',#95612,0.1) ;
#31017=CIRCLE('',#95615,0.1) ;
#31018=CIRCLE('',#95616,0.1) ;
#31019=CIRCLE('',#95618,0.1) ;
#31020=CIRCLE('',#95620,0.1) ;
#31021=CIRCLE('',#95622,0.1) ;
#31022=CIRCLE('',#95624,0.0999999999999998) ;
#31023=CIRCLE('',#95626,0.1) ;
#31024=CIRCLE('',#95628,0.1) ;
#31025=CIRCLE('',#95631,0.1) ;
#31026=CIRCLE('',#95633,0.0999999999999994) ;
#31027=CIRCLE('',#95635,0.0999999999999994) ;
#31028=CIRCLE('',#95637,0.0999999999999994) ;
#31029=CIRCLE('',#95639,0.0999999999999998) ;
#31030=CIRCLE('',#95641,0.1) ;
#31031=CIRCLE('',#95643,0.0999999999999998) ;
#31032=CIRCLE('',#95645,0.1) ;
#31033=CIRCLE('',#95647,0.1) ;
#31034=CIRCLE('',#95649,0.0999999999999994) ;
#31035=CIRCLE('',#95651,0.0999999999999998) ;
#31036=CIRCLE('',#95653,0.0999999999999998) ;
#31037=CIRCLE('',#95655,0.0999999999999998) ;
#31038=CIRCLE('',#95657,0.0999999999999998) ;
#31039=CIRCLE('',#95659,0.0999999999999998) ;
#31040=CIRCLE('',#95661,0.0999999999999998) ;
#31041=CIRCLE('',#95663,0.0999999999999994) ;
#31042=CIRCLE('',#95665,0.1) ;
#31043=CIRCLE('',#95668,0.1) ;
#31044=CIRCLE('',#95669,0.1) ;
#31045=CIRCLE('',#95671,0.1) ;
#31046=CIRCLE('',#95672,0.1) ;
#31047=CIRCLE('',#95674,0.1) ;
#31048=CIRCLE('',#95675,0.1) ;
#31049=CIRCLE('',#95677,0.1) ;
#31050=CIRCLE('',#95678,0.0999999999999998) ;
#31051=CIRCLE('',#95680,0.1) ;
#31052=CIRCLE('',#95682,0.1) ;
#31053=CIRCLE('',#95684,0.1) ;
#31054=CIRCLE('',#95686,0.1) ;
#31055=CIRCLE('',#95688,0.0999999999999998) ;
#31056=CIRCLE('',#95690,0.1) ;
#31057=CIRCLE('',#95692,0.0999999999999994) ;
#31058=CIRCLE('',#95693,0.1) ;
#31059=CIRCLE('',#95696,0.1) ;
#31060=CIRCLE('',#95698,0.1) ;
#31061=CIRCLE('',#95699,0.1) ;
#31062=CIRCLE('',#95701,0.0999999999999994) ;
#31063=CIRCLE('',#95703,0.1) ;
#31064=CIRCLE('',#95705,0.1) ;
#31065=CIRCLE('',#95707,0.1) ;
#31066=CIRCLE('',#95709,0.0999999999999994) ;
#31067=CIRCLE('',#95711,0.1) ;
#31068=CIRCLE('',#95712,0.0999999999999994) ;
#31069=CIRCLE('',#95714,0.1) ;
#31070=CIRCLE('',#95716,0.1) ;
#31071=CIRCLE('',#95718,0.0999999999999998) ;
#31072=CIRCLE('',#95719,0.1) ;
#31073=CIRCLE('',#95721,0.1) ;
#31074=CIRCLE('',#95723,0.1) ;
#31075=CIRCLE('',#95724,0.1) ;
#31076=CIRCLE('',#95726,0.1) ;
#31077=CIRCLE('',#95728,0.1) ;
#31078=CIRCLE('',#95730,0.1) ;
#31079=CIRCLE('',#95732,0.1) ;
#31080=CIRCLE('',#95734,0.1) ;
#31081=CIRCLE('',#95736,0.1) ;
#31082=CIRCLE('',#95738,0.1) ;
#31083=CIRCLE('',#95740,0.0999999999999994) ;
#31084=CIRCLE('',#95741,0.0999999999999994) ;
#31085=CIRCLE('',#95743,0.1) ;
#31086=CIRCLE('',#95745,0.1) ;
#31087=CIRCLE('',#95747,0.1) ;
#31088=CIRCLE('',#95749,0.1) ;
#31089=CIRCLE('',#95750,0.0999999999999994) ;
#31090=CIRCLE('',#95752,0.0999999999999994) ;
#31091=CIRCLE('',#95754,0.0999999999999994) ;
#31092=CIRCLE('',#95756,0.1) ;
#31093=CIRCLE('',#95758,0.0999999999999994) ;
#31094=CIRCLE('',#95761,0.0999999999999994) ;
#31095=CIRCLE('',#95763,0.1) ;
#31096=CIRCLE('',#95765,0.0999999999999994) ;
#31097=CIRCLE('',#95768,0.1) ;
#31098=CIRCLE('',#95769,0.1) ;
#31099=CIRCLE('',#95771,0.0999999999999994) ;
#31100=CIRCLE('',#95773,0.0999999999999994) ;
#31101=CIRCLE('',#95775,0.0999999999999994) ;
#31102=CIRCLE('',#95777,0.0999999999999994) ;
#31103=CIRCLE('',#95779,0.1) ;
#31104=CIRCLE('',#95781,0.0999999999999998) ;
#31105=CIRCLE('',#95783,0.1) ;
#31106=CIRCLE('',#95785,0.1) ;
#31107=CIRCLE('',#95787,0.1) ;
#31108=CIRCLE('',#95789,0.1) ;
#31109=CIRCLE('',#95791,0.1) ;
#31110=CIRCLE('',#95793,0.1) ;
#31111=CIRCLE('',#95795,0.1) ;
#31112=CIRCLE('',#95797,0.1) ;
#31113=CIRCLE('',#95800,0.1) ;
#31114=CIRCLE('',#95802,0.1) ;
#31115=CIRCLE('',#95804,0.1) ;
#31116=CIRCLE('',#95806,0.1) ;
#31117=CIRCLE('',#95808,0.0999999999999998) ;
#31118=CIRCLE('',#95810,0.1) ;
#31119=CIRCLE('',#95812,0.1) ;
#31120=CIRCLE('',#95814,0.1) ;
#31121=CIRCLE('',#95816,0.1) ;
#31122=CIRCLE('',#95818,0.1) ;
#31123=CIRCLE('',#95821,0.0999999999999994) ;
#31124=CIRCLE('',#95822,0.0999999999999994) ;
#31125=CIRCLE('',#95824,0.0999999999999994) ;
#31126=CIRCLE('',#95825,0.1) ;
#31127=CIRCLE('',#95827,0.0999999999999994) ;
#31128=CIRCLE('',#95828,0.1) ;
#31129=CIRCLE('',#95830,0.1) ;
#31130=CIRCLE('',#95831,0.0999999999999998) ;
#31131=CIRCLE('',#95833,0.1) ;
#31132=CIRCLE('',#95835,0.1) ;
#31133=CIRCLE('',#95837,0.0999999999999994) ;
#31134=CIRCLE('',#95839,0.1) ;
#31135=CIRCLE('',#95841,0.0999999999999998) ;
#31136=CIRCLE('',#95843,0.1) ;
#31137=CIRCLE('',#95845,0.0999999999999994) ;
#31138=CIRCLE('',#95846,0.1) ;
#31139=CIRCLE('',#95849,0.1) ;
#31140=CIRCLE('',#95851,0.0999999999999994) ;
#31141=CIRCLE('',#95852,0.0999999999999994) ;
#31142=CIRCLE('',#95854,0.0999999999999994) ;
#31143=CIRCLE('',#95856,0.1) ;
#31144=CIRCLE('',#95858,0.0999999999999994) ;
#31145=CIRCLE('',#95860,0.0999999999999994) ;
#31146=CIRCLE('',#95862,0.0999999999999994) ;
#31147=CIRCLE('',#95864,0.1) ;
#31148=CIRCLE('',#95865,0.0999999999999994) ;
#31149=CIRCLE('',#95867,0.1) ;
#31150=CIRCLE('',#95869,0.0999999999999994) ;
#31151=CIRCLE('',#95871,0.0999999999999998) ;
#31152=CIRCLE('',#95872,0.1) ;
#31153=CIRCLE('',#95874,0.0999999999999994) ;
#31154=CIRCLE('',#95876,0.1) ;
#31155=CIRCLE('',#95877,0.1) ;
#31156=CIRCLE('',#95879,0.1) ;
#31157=CIRCLE('',#95881,0.1) ;
#31158=CIRCLE('',#95883,0.0999999999999994) ;
#31159=CIRCLE('',#95885,0.0999999999999994) ;
#31160=CIRCLE('',#95887,0.1) ;
#31161=CIRCLE('',#95889,0.1) ;
#31162=CIRCLE('',#95891,0.1) ;
#31163=CIRCLE('',#95893,0.0999999999999994) ;
#31164=CIRCLE('',#95894,0.0999999999999994) ;
#31165=CIRCLE('',#95896,0.1) ;
#31166=CIRCLE('',#95898,0.1) ;
#31167=CIRCLE('',#95900,0.1) ;
#31168=CIRCLE('',#95902,0.1) ;
#31169=CIRCLE('',#95903,0.0999999999999994) ;
#31170=CIRCLE('',#95905,0.0999999999999994) ;
#31171=CIRCLE('',#95907,0.0999999999999994) ;
#31172=CIRCLE('',#95909,0.1) ;
#31173=CIRCLE('',#95911,0.0999999999999994) ;
#31174=CIRCLE('',#95914,0.0999999999999994) ;
#31175=CIRCLE('',#95916,0.1) ;
#31176=CIRCLE('',#95918,0.0999999999999994) ;
#31177=CIRCLE('',#95921,0.1) ;
#31178=CIRCLE('',#95922,0.1) ;
#31179=CIRCLE('',#95924,0.0999999999999994) ;
#31180=CIRCLE('',#95926,0.0999999999999994) ;
#31181=CIRCLE('',#95928,0.0999999999999994) ;
#31182=CIRCLE('',#95930,0.0999999999999994) ;
#31183=CIRCLE('',#95932,0.1) ;
#31184=CIRCLE('',#95934,0.0999999999999998) ;
#31185=CIRCLE('',#95936,0.1) ;
#31186=CIRCLE('',#95938,0.1) ;
#31187=CIRCLE('',#95940,0.1) ;
#31188=CIRCLE('',#95942,0.1) ;
#31189=CIRCLE('',#95944,0.1) ;
#31190=CIRCLE('',#95946,0.1) ;
#31191=CIRCLE('',#95948,0.1) ;
#31192=CIRCLE('',#95950,0.1) ;
#31193=CIRCLE('',#95953,0.1) ;
#31194=CIRCLE('',#95955,0.0999999999999994) ;
#31195=CIRCLE('',#95957,0.1) ;
#31196=CIRCLE('',#95959,0.0999999999999994) ;
#31197=CIRCLE('',#95961,0.1) ;
#31198=CIRCLE('',#95963,0.1) ;
#31199=CIRCLE('',#95965,0.1) ;
#31200=CIRCLE('',#95967,0.1) ;
#31201=CIRCLE('',#95969,0.0999999999999994) ;
#31202=CIRCLE('',#95971,0.0999999999999994) ;
#31203=CIRCLE('',#95974,0.0999999999999994) ;
#31204=CIRCLE('',#95975,0.0999999999999994) ;
#31205=CIRCLE('',#95977,0.0999999999999994) ;
#31206=CIRCLE('',#95978,0.1) ;
#31207=CIRCLE('',#95980,0.0999999999999994) ;
#31208=CIRCLE('',#95981,0.1) ;
#31209=CIRCLE('',#95983,0.1) ;
#31210=CIRCLE('',#95984,0.0999999999999998) ;
#31211=CIRCLE('',#95986,0.1) ;
#31212=CIRCLE('',#95988,0.1) ;
#31213=CIRCLE('',#95990,0.0999999999999994) ;
#31214=CIRCLE('',#95992,0.1) ;
#31215=CIRCLE('',#95994,0.0999999999999998) ;
#31216=CIRCLE('',#95996,0.1) ;
#31217=CIRCLE('',#95998,0.0999999999999994) ;
#31218=CIRCLE('',#95999,0.1) ;
#31219=CIRCLE('',#96002,0.1) ;
#31220=CIRCLE('',#96004,0.0999999999999994) ;
#31221=CIRCLE('',#96005,0.0999999999999994) ;
#31222=CIRCLE('',#96007,0.0999999999999994) ;
#31223=CIRCLE('',#96009,0.1) ;
#31224=CIRCLE('',#96011,0.0999999999999994) ;
#31225=CIRCLE('',#96013,0.0999999999999994) ;
#31226=CIRCLE('',#96015,0.0999999999999994) ;
#31227=CIRCLE('',#96017,0.1) ;
#31228=CIRCLE('',#96018,0.0999999999999994) ;
#31229=CIRCLE('',#96020,0.1) ;
#31230=CIRCLE('',#96022,0.0999999999999994) ;
#31231=CIRCLE('',#96024,0.0999999999999998) ;
#31232=CIRCLE('',#96025,0.1) ;
#31233=CIRCLE('',#96027,0.0999999999999994) ;
#31234=CIRCLE('',#96029,0.1) ;
#31235=CIRCLE('',#96030,0.1) ;
#31236=CIRCLE('',#96032,0.1) ;
#31237=CIRCLE('',#96034,0.1) ;
#31238=CIRCLE('',#96036,0.0999999999999994) ;
#31239=CIRCLE('',#96038,0.0999999999999994) ;
#31240=CIRCLE('',#96040,0.1) ;
#31241=CIRCLE('',#96042,0.1) ;
#31242=CIRCLE('',#96044,0.1) ;
#31243=CIRCLE('',#96046,0.0999999999999994) ;
#31244=CIRCLE('',#96047,0.0999999999999994) ;
#31245=CIRCLE('',#96049,0.1) ;
#31246=CIRCLE('',#96051,0.1) ;
#31247=CIRCLE('',#96053,0.1) ;
#31248=CIRCLE('',#96055,0.1) ;
#31249=CIRCLE('',#96056,0.0999999999999994) ;
#31250=CIRCLE('',#96058,0.0999999999999994) ;
#31251=CIRCLE('',#96060,0.0999999999999994) ;
#31252=CIRCLE('',#96062,0.1) ;
#31253=CIRCLE('',#96064,0.0999999999999994) ;
#31254=CIRCLE('',#96067,0.0999999999999994) ;
#31255=CIRCLE('',#96069,0.1) ;
#31256=CIRCLE('',#96071,0.0999999999999994) ;
#31257=CIRCLE('',#96074,0.1) ;
#31258=CIRCLE('',#96075,0.1) ;
#31259=CIRCLE('',#96077,0.0999999999999994) ;
#31260=CIRCLE('',#96079,0.0999999999999994) ;
#31261=CIRCLE('',#96081,0.0999999999999994) ;
#31262=CIRCLE('',#96083,0.0999999999999994) ;
#31263=CIRCLE('',#96085,0.1) ;
#31264=CIRCLE('',#96087,0.1) ;
#31265=CIRCLE('',#96089,0.1) ;
#31266=CIRCLE('',#96091,0.1) ;
#31267=CIRCLE('',#96093,0.1) ;
#31268=CIRCLE('',#96095,0.1) ;
#31269=CIRCLE('',#96097,0.100000000000001) ;
#31270=CIRCLE('',#96099,0.1) ;
#31271=CIRCLE('',#96101,0.1) ;
#31272=CIRCLE('',#96103,0.1) ;
#31273=CIRCLE('',#96106,0.1) ;
#31274=CIRCLE('',#96108,0.0999999999999994) ;
#31275=CIRCLE('',#96110,0.1) ;
#31276=CIRCLE('',#96112,0.0999999999999994) ;
#31277=CIRCLE('',#96114,0.1) ;
#31278=CIRCLE('',#96116,0.1) ;
#31279=CIRCLE('',#96118,0.1) ;
#31280=CIRCLE('',#96120,0.1) ;
#31281=CIRCLE('',#96122,0.0999999999999994) ;
#31282=CIRCLE('',#96124,0.0999999999999994) ;
#31283=CIRCLE('',#96127,0.0999999999999994) ;
#31284=CIRCLE('',#96128,0.0999999999999994) ;
#31285=CIRCLE('',#96130,0.0999999999999994) ;
#31286=CIRCLE('',#96131,0.1) ;
#31287=CIRCLE('',#96133,0.0999999999999994) ;
#31288=CIRCLE('',#96134,0.1) ;
#31289=CIRCLE('',#96136,0.1) ;
#31290=CIRCLE('',#96137,0.0999999999999998) ;
#31291=CIRCLE('',#96139,0.1) ;
#31292=CIRCLE('',#96141,0.1) ;
#31293=CIRCLE('',#96143,0.0999999999999994) ;
#31294=CIRCLE('',#96145,0.1) ;
#31295=CIRCLE('',#96147,0.0999999999999998) ;
#31296=CIRCLE('',#96149,0.1) ;
#31297=CIRCLE('',#96151,0.0999999999999994) ;
#31298=CIRCLE('',#96152,0.1) ;
#31299=CIRCLE('',#96155,0.1) ;
#31300=CIRCLE('',#96157,0.0999999999999994) ;
#31301=CIRCLE('',#96158,0.0999999999999994) ;
#31302=CIRCLE('',#96160,0.0999999999999994) ;
#31303=CIRCLE('',#96162,0.1) ;
#31304=CIRCLE('',#96164,0.0999999999999994) ;
#31305=CIRCLE('',#96166,0.0999999999999994) ;
#31306=CIRCLE('',#96168,0.0999999999999994) ;
#31307=CIRCLE('',#96170,0.1) ;
#31308=CIRCLE('',#96171,0.0999999999999994) ;
#31309=CIRCLE('',#96173,0.1) ;
#31310=CIRCLE('',#96175,0.0999999999999994) ;
#31311=CIRCLE('',#96177,0.0999999999999998) ;
#31312=CIRCLE('',#96178,0.1) ;
#31313=CIRCLE('',#96180,0.0999999999999994) ;
#31314=CIRCLE('',#96182,0.1) ;
#31315=CIRCLE('',#96183,0.1) ;
#31316=CIRCLE('',#96185,0.1) ;
#31317=CIRCLE('',#96187,0.1) ;
#31318=CIRCLE('',#96189,0.0999999999999994) ;
#31319=CIRCLE('',#96191,0.0999999999999994) ;
#31320=CIRCLE('',#96193,0.1) ;
#31321=CIRCLE('',#96195,0.1) ;
#31322=CIRCLE('',#96197,0.1) ;
#31323=CIRCLE('',#96199,0.0999999999999994) ;
#31324=CIRCLE('',#96200,0.0999999999999994) ;
#31325=CIRCLE('',#96202,0.1) ;
#31326=CIRCLE('',#96204,0.1) ;
#31327=CIRCLE('',#96206,0.1) ;
#31328=CIRCLE('',#96208,0.1) ;
#31329=CIRCLE('',#96209,0.0999999999999994) ;
#31330=CIRCLE('',#96211,0.0999999999999994) ;
#31331=CIRCLE('',#96213,0.0999999999999994) ;
#31332=CIRCLE('',#96215,0.1) ;
#31333=CIRCLE('',#96217,0.0999999999999994) ;
#31334=CIRCLE('',#96220,0.0999999999999994) ;
#31335=CIRCLE('',#96222,0.1) ;
#31336=CIRCLE('',#96224,0.0999999999999994) ;
#31337=CIRCLE('',#96227,0.1) ;
#31338=CIRCLE('',#96228,0.1) ;
#31339=CIRCLE('',#96230,0.0999999999999994) ;
#31340=CIRCLE('',#96232,0.0999999999999994) ;
#31341=CIRCLE('',#96234,0.0999999999999994) ;
#31342=CIRCLE('',#96236,0.0999999999999994) ;
#31343=CIRCLE('',#96238,0.1) ;
#31344=CIRCLE('',#96240,0.1) ;
#31345=CIRCLE('',#96242,0.1) ;
#31346=CIRCLE('',#96244,0.1) ;
#31347=CIRCLE('',#96246,0.1) ;
#31348=CIRCLE('',#96248,0.1) ;
#31349=CIRCLE('',#96250,0.0999999999999989) ;
#31350=CIRCLE('',#96252,0.1) ;
#31351=CIRCLE('',#96254,0.1) ;
#31352=CIRCLE('',#96256,0.1) ;
#31353=CIRCLE('',#96259,0.1) ;
#31354=CIRCLE('',#96261,0.0999999999999994) ;
#31355=CIRCLE('',#96263,0.0999999999999995) ;
#31356=CIRCLE('',#96265,0.0999999999999994) ;
#31357=CIRCLE('',#96267,0.1) ;
#31358=CIRCLE('',#96269,0.1) ;
#31359=CIRCLE('',#96271,0.1) ;
#31360=CIRCLE('',#96273,0.1) ;
#31361=CIRCLE('',#96275,0.0999999999999994) ;
#31362=CIRCLE('',#96277,0.0999999999999994) ;
#31363=CIRCLE('',#96280,0.0999999999999994) ;
#31364=CIRCLE('',#96281,0.0999999999999994) ;
#31365=CIRCLE('',#96283,0.0999999999999994) ;
#31366=CIRCLE('',#96284,0.1) ;
#31367=CIRCLE('',#96286,0.0999999999999994) ;
#31368=CIRCLE('',#96287,0.1) ;
#31369=CIRCLE('',#96289,0.1) ;
#31370=CIRCLE('',#96290,0.0999999999999998) ;
#31371=CIRCLE('',#96292,0.1) ;
#31372=CIRCLE('',#96294,0.1) ;
#31373=CIRCLE('',#96296,0.0999999999999994) ;
#31374=CIRCLE('',#96298,0.1) ;
#31375=CIRCLE('',#96300,0.0999999999999998) ;
#31376=CIRCLE('',#96302,0.1) ;
#31377=CIRCLE('',#96304,0.0999999999999994) ;
#31378=CIRCLE('',#96305,0.1) ;
#31379=CIRCLE('',#96308,0.1) ;
#31380=CIRCLE('',#96310,0.0999999999999994) ;
#31381=CIRCLE('',#96311,0.0999999999999994) ;
#31382=CIRCLE('',#96313,0.0999999999999994) ;
#31383=CIRCLE('',#96315,0.1) ;
#31384=CIRCLE('',#96317,0.0999999999999994) ;
#31385=CIRCLE('',#96319,0.0999999999999994) ;
#31386=CIRCLE('',#96321,0.0999999999999994) ;
#31387=CIRCLE('',#96323,0.1) ;
#31388=CIRCLE('',#96324,0.0999999999999994) ;
#31389=CIRCLE('',#96326,0.1) ;
#31390=CIRCLE('',#96328,0.0999999999999994) ;
#31391=CIRCLE('',#96330,0.0999999999999998) ;
#31392=CIRCLE('',#96331,0.1) ;
#31393=CIRCLE('',#96333,0.0999999999999994) ;
#31394=CIRCLE('',#96335,0.1) ;
#31395=CIRCLE('',#96336,0.1) ;
#31396=CIRCLE('',#96338,0.1) ;
#31397=CIRCLE('',#96340,0.1) ;
#31398=CIRCLE('',#96342,0.0999999999999994) ;
#31399=CIRCLE('',#96344,0.0999999999999994) ;
#31400=CIRCLE('',#96346,0.1) ;
#31401=CIRCLE('',#96348,0.1) ;
#31402=CIRCLE('',#96350,0.1) ;
#31403=CIRCLE('',#96352,0.0999999999999994) ;
#31404=CIRCLE('',#96353,0.0999999999999994) ;
#31405=CIRCLE('',#96355,0.1) ;
#31406=CIRCLE('',#96357,0.1) ;
#31407=CIRCLE('',#96359,0.1) ;
#31408=CIRCLE('',#96361,0.1) ;
#31409=CIRCLE('',#96362,0.0999999999999994) ;
#31410=CIRCLE('',#96364,0.0999999999999994) ;
#31411=CIRCLE('',#96366,0.0999999999999994) ;
#31412=CIRCLE('',#96368,0.1) ;
#31413=CIRCLE('',#96370,0.0999999999999994) ;
#31414=CIRCLE('',#96373,0.0999999999999994) ;
#31415=CIRCLE('',#96375,0.1) ;
#31416=CIRCLE('',#96377,0.0999999999999994) ;
#31417=CIRCLE('',#96380,0.1) ;
#31418=CIRCLE('',#96381,0.1) ;
#31419=CIRCLE('',#96383,0.0999999999999994) ;
#31420=CIRCLE('',#96385,0.0999999999999994) ;
#31421=CIRCLE('',#96387,0.0999999999999994) ;
#31422=CIRCLE('',#96389,0.0999999999999994) ;
#31423=CIRCLE('',#96391,0.1) ;
#31424=CIRCLE('',#96393,0.1) ;
#31425=CIRCLE('',#96395,0.1) ;
#31426=CIRCLE('',#96397,0.1) ;
#31427=CIRCLE('',#96399,0.1) ;
#31428=CIRCLE('',#96401,0.1) ;
#31429=CIRCLE('',#96403,0.0999999999999989) ;
#31430=CIRCLE('',#96405,0.1) ;
#31431=CIRCLE('',#96407,0.1) ;
#31432=CIRCLE('',#96409,0.1) ;
#31433=CIRCLE('',#96412,0.1) ;
#31434=CIRCLE('',#96414,0.0999999999999994) ;
#31435=CIRCLE('',#96416,0.0999999999999995) ;
#31436=CIRCLE('',#96418,0.0999999999999994) ;
#31437=CIRCLE('',#96420,0.1) ;
#31438=CIRCLE('',#96422,0.1) ;
#31439=CIRCLE('',#96424,0.1) ;
#31440=CIRCLE('',#96426,0.1) ;
#31441=CIRCLE('',#96428,0.0999999999999994) ;
#31442=CIRCLE('',#96430,0.0999999999999994) ;
#31443=CIRCLE('',#96433,0.0999999999999994) ;
#31444=CIRCLE('',#96434,0.0999999999999994) ;
#31445=CIRCLE('',#96436,0.0999999999999994) ;
#31446=CIRCLE('',#96437,0.1) ;
#31447=CIRCLE('',#96439,0.0999999999999994) ;
#31448=CIRCLE('',#96440,0.1) ;
#31449=CIRCLE('',#96442,0.1) ;
#31450=CIRCLE('',#96443,0.0999999999999998) ;
#31451=CIRCLE('',#96445,0.1) ;
#31452=CIRCLE('',#96447,0.1) ;
#31453=CIRCLE('',#96449,0.0999999999999994) ;
#31454=CIRCLE('',#96451,0.1) ;
#31455=CIRCLE('',#96453,0.0999999999999998) ;
#31456=CIRCLE('',#96455,0.1) ;
#31457=CIRCLE('',#96457,0.0999999999999994) ;
#31458=CIRCLE('',#96458,0.1) ;
#31459=CIRCLE('',#96461,0.1) ;
#31460=CIRCLE('',#96463,0.0999999999999994) ;
#31461=CIRCLE('',#96464,0.0999999999999994) ;
#31462=CIRCLE('',#96466,0.0999999999999994) ;
#31463=CIRCLE('',#96468,0.1) ;
#31464=CIRCLE('',#96470,0.0999999999999994) ;
#31465=CIRCLE('',#96472,0.0999999999999994) ;
#31466=CIRCLE('',#96474,0.0999999999999994) ;
#31467=CIRCLE('',#96476,0.1) ;
#31468=CIRCLE('',#96477,0.0999999999999994) ;
#31469=CIRCLE('',#96479,0.1) ;
#31470=CIRCLE('',#96481,0.0999999999999994) ;
#31471=CIRCLE('',#96483,0.0999999999999998) ;
#31472=CIRCLE('',#96484,0.1) ;
#31473=CIRCLE('',#96486,0.0999999999999994) ;
#31474=CIRCLE('',#96488,0.1) ;
#31475=CIRCLE('',#96489,0.1) ;
#31476=CIRCLE('',#96491,0.1) ;
#31477=CIRCLE('',#96493,0.1) ;
#31478=CIRCLE('',#96495,0.0999999999999994) ;
#31479=CIRCLE('',#96497,0.0999999999999994) ;
#31480=CIRCLE('',#96499,0.1) ;
#31481=CIRCLE('',#96501,0.1) ;
#31482=CIRCLE('',#96503,0.1) ;
#31483=CIRCLE('',#96505,0.0999999999999994) ;
#31484=CIRCLE('',#96506,0.0999999999999994) ;
#31485=CIRCLE('',#96508,0.1) ;
#31486=CIRCLE('',#96510,0.1) ;
#31487=CIRCLE('',#96512,0.1) ;
#31488=CIRCLE('',#96514,0.1) ;
#31489=CIRCLE('',#96515,0.0999999999999994) ;
#31490=CIRCLE('',#96517,0.0999999999999994) ;
#31491=CIRCLE('',#96519,0.0999999999999994) ;
#31492=CIRCLE('',#96521,0.1) ;
#31493=CIRCLE('',#96523,0.0999999999999994) ;
#31494=CIRCLE('',#96526,0.0999999999999994) ;
#31495=CIRCLE('',#96528,0.1) ;
#31496=CIRCLE('',#96530,0.0999999999999994) ;
#31497=CIRCLE('',#96533,0.1) ;
#31498=CIRCLE('',#96534,0.1) ;
#31499=CIRCLE('',#96536,0.0999999999999994) ;
#31500=CIRCLE('',#96538,0.0999999999999994) ;
#31501=CIRCLE('',#96540,0.0999999999999994) ;
#31502=CIRCLE('',#96542,0.0999999999999994) ;
#31503=CIRCLE('',#96544,0.1) ;
#31504=CIRCLE('',#96546,0.1) ;
#31505=CIRCLE('',#96548,0.1) ;
#31506=CIRCLE('',#96550,0.1) ;
#31507=CIRCLE('',#96552,0.1) ;
#31508=CIRCLE('',#96554,0.1) ;
#31509=CIRCLE('',#96556,0.0999999999999989) ;
#31510=CIRCLE('',#96558,0.1) ;
#31511=CIRCLE('',#96560,0.1) ;
#31512=CIRCLE('',#96562,0.1) ;
#31513=CIRCLE('',#96565,0.1) ;
#31514=CIRCLE('',#96567,0.0999999999999994) ;
#31515=CIRCLE('',#96569,0.0999999999999995) ;
#31516=CIRCLE('',#96571,0.0999999999999994) ;
#31517=CIRCLE('',#96573,0.1) ;
#31518=CIRCLE('',#96575,0.1) ;
#31519=CIRCLE('',#96577,0.1) ;
#31520=CIRCLE('',#96579,0.1) ;
#31521=CIRCLE('',#96581,0.0999999999999994) ;
#31522=CIRCLE('',#96583,0.0999999999999994) ;
#31523=CIRCLE('',#96586,0.0999999999999994) ;
#31524=CIRCLE('',#96587,0.0999999999999994) ;
#31525=CIRCLE('',#96589,0.0999999999999994) ;
#31526=CIRCLE('',#96590,0.1) ;
#31527=CIRCLE('',#96592,0.0999999999999994) ;
#31528=CIRCLE('',#96593,0.1) ;
#31529=CIRCLE('',#96595,0.1) ;
#31530=CIRCLE('',#96596,0.0999999999999998) ;
#31531=CIRCLE('',#96598,0.1) ;
#31532=CIRCLE('',#96600,0.1) ;
#31533=CIRCLE('',#96602,0.0999999999999994) ;
#31534=CIRCLE('',#96604,0.1) ;
#31535=CIRCLE('',#96606,0.0999999999999998) ;
#31536=CIRCLE('',#96608,0.1) ;
#31537=CIRCLE('',#96610,0.0999999999999994) ;
#31538=CIRCLE('',#96611,0.1) ;
#31539=CIRCLE('',#96614,0.1) ;
#31540=CIRCLE('',#96616,0.0999999999999994) ;
#31541=CIRCLE('',#96617,0.0999999999999994) ;
#31542=CIRCLE('',#96619,0.0999999999999994) ;
#31543=CIRCLE('',#96621,0.1) ;
#31544=CIRCLE('',#96623,0.0999999999999994) ;
#31545=CIRCLE('',#96625,0.0999999999999994) ;
#31546=CIRCLE('',#96627,0.0999999999999994) ;
#31547=CIRCLE('',#96629,0.1) ;
#31548=CIRCLE('',#96630,0.0999999999999994) ;
#31549=CIRCLE('',#96632,0.1) ;
#31550=CIRCLE('',#96634,0.0999999999999994) ;
#31551=CIRCLE('',#96636,0.0999999999999998) ;
#31552=CIRCLE('',#96637,0.1) ;
#31553=CIRCLE('',#96639,0.0999999999999994) ;
#31554=CIRCLE('',#96641,0.1) ;
#31555=CIRCLE('',#96642,0.1) ;
#31556=CIRCLE('',#96644,0.1) ;
#31557=CIRCLE('',#96646,0.1) ;
#31558=CIRCLE('',#96648,0.0999999999999994) ;
#31559=CIRCLE('',#96650,0.0999999999999994) ;
#31560=CIRCLE('',#96652,0.1) ;
#31561=CIRCLE('',#96654,0.1) ;
#31562=CIRCLE('',#96656,0.1) ;
#31563=CIRCLE('',#96658,0.100000000000003) ;
#31564=CIRCLE('',#96659,0.100000000000003) ;
#31565=CIRCLE('',#96661,0.1) ;
#31566=CIRCLE('',#96663,0.1) ;
#31567=CIRCLE('',#96665,0.1) ;
#31568=CIRCLE('',#96667,0.1) ;
#31569=CIRCLE('',#96668,0.100000000000003) ;
#31570=CIRCLE('',#96670,0.100000000000003) ;
#31571=CIRCLE('',#96672,0.100000000000003) ;
#31572=CIRCLE('',#96674,0.1) ;
#31573=CIRCLE('',#96676,0.100000000000003) ;
#31574=CIRCLE('',#96679,0.100000000000003) ;
#31575=CIRCLE('',#96681,0.1) ;
#31576=CIRCLE('',#96683,0.100000000000003) ;
#31577=CIRCLE('',#96686,0.1) ;
#31578=CIRCLE('',#96687,0.1) ;
#31579=CIRCLE('',#96689,0.0999999999999994) ;
#31580=CIRCLE('',#96691,0.100000000000003) ;
#31581=CIRCLE('',#96693,0.0999999999999994) ;
#31582=CIRCLE('',#96695,0.100000000000003) ;
#31583=CIRCLE('',#96697,0.1) ;
#31584=CIRCLE('',#96699,0.1) ;
#31585=CIRCLE('',#96701,0.1) ;
#31586=CIRCLE('',#96703,0.1) ;
#31587=CIRCLE('',#96705,0.0999999999999999) ;
#31588=CIRCLE('',#96707,0.1) ;
#31589=CIRCLE('',#96709,0.0999999999999992) ;
#31590=CIRCLE('',#96711,0.1) ;
#31591=CIRCLE('',#96713,0.1) ;
#31592=CIRCLE('',#96715,0.1) ;
#31593=CIRCLE('',#96718,0.1) ;
#31594=CIRCLE('',#96720,0.0999999999999994) ;
#31595=CIRCLE('',#96722,0.0999999999999995) ;
#31596=CIRCLE('',#96724,0.0999999999999994) ;
#31597=CIRCLE('',#96726,0.1) ;
#31598=CIRCLE('',#96728,0.1) ;
#31599=CIRCLE('',#96730,0.1) ;
#31600=CIRCLE('',#96732,0.1) ;
#31601=CIRCLE('',#96734,0.0999999999999994) ;
#31602=CIRCLE('',#96736,0.0999999999999994) ;
#31603=CIRCLE('',#96739,0.100000000000003) ;
#31604=CIRCLE('',#96740,0.100000000000003) ;
#31605=CIRCLE('',#96742,0.100000000000003) ;
#31606=CIRCLE('',#96743,0.1) ;
#31607=CIRCLE('',#96745,0.100000000000003) ;
#31608=CIRCLE('',#96746,0.1) ;
#31609=CIRCLE('',#96748,0.1) ;
#31610=CIRCLE('',#96749,0.0999999999999998) ;
#31611=CIRCLE('',#96751,0.1) ;
#31612=CIRCLE('',#96753,0.1) ;
#31613=CIRCLE('',#96755,0.100000000000003) ;
#31614=CIRCLE('',#96757,0.1) ;
#31615=CIRCLE('',#96759,0.0999999999999998) ;
#31616=CIRCLE('',#96761,0.1) ;
#31617=CIRCLE('',#96763,0.100000000000003) ;
#31618=CIRCLE('',#96764,0.1) ;
#31619=CIRCLE('',#96767,0.1) ;
#31620=CIRCLE('',#96769,0.100000000000003) ;
#31621=CIRCLE('',#96770,0.100000000000003) ;
#31622=CIRCLE('',#96772,0.100000000000003) ;
#31623=CIRCLE('',#96774,0.1) ;
#31624=CIRCLE('',#96776,0.100000000000003) ;
#31625=CIRCLE('',#96778,0.100000000000003) ;
#31626=CIRCLE('',#96780,0.100000000000003) ;
#31627=CIRCLE('',#96782,0.1) ;
#31628=CIRCLE('',#96783,0.100000000000003) ;
#31629=CIRCLE('',#96785,0.1) ;
#31630=CIRCLE('',#96787,0.100000000000003) ;
#31631=CIRCLE('',#96789,0.0999999999999998) ;
#31632=CIRCLE('',#96790,0.1) ;
#31633=CIRCLE('',#96792,0.100000000000003) ;
#31634=CIRCLE('',#96794,0.1) ;
#31635=CIRCLE('',#96795,0.1) ;
#31636=CIRCLE('',#96797,0.1) ;
#31637=CIRCLE('',#96799,0.1) ;
#31638=CIRCLE('',#96801,0.100000000000003) ;
#31639=CIRCLE('',#96803,0.100000000000003) ;
#31640=CIRCLE('',#96805,0.1) ;
#31641=CIRCLE('',#96807,0.1) ;
#31642=CIRCLE('',#96809,0.1) ;
#31643=CIRCLE('',#96811,0.100000000000003) ;
#31644=CIRCLE('',#96812,0.100000000000003) ;
#31645=CIRCLE('',#96814,0.1) ;
#31646=CIRCLE('',#96816,0.1) ;
#31647=CIRCLE('',#96818,0.1) ;
#31648=CIRCLE('',#96820,0.1) ;
#31649=CIRCLE('',#96821,0.100000000000003) ;
#31650=CIRCLE('',#96823,0.100000000000003) ;
#31651=CIRCLE('',#96825,0.100000000000003) ;
#31652=CIRCLE('',#96827,0.1) ;
#31653=CIRCLE('',#96829,0.100000000000003) ;
#31654=CIRCLE('',#96832,0.100000000000003) ;
#31655=CIRCLE('',#96834,0.1) ;
#31656=CIRCLE('',#96836,0.100000000000003) ;
#31657=CIRCLE('',#96839,0.1) ;
#31658=CIRCLE('',#96840,0.1) ;
#31659=CIRCLE('',#96842,0.100000000000003) ;
#31660=CIRCLE('',#96844,0.100000000000003) ;
#31661=CIRCLE('',#96846,0.100000000000003) ;
#31662=CIRCLE('',#96848,0.100000000000003) ;
#31663=CIRCLE('',#96850,0.1) ;
#31664=CIRCLE('',#96852,0.1) ;
#31665=CIRCLE('',#96854,0.1) ;
#31666=CIRCLE('',#96856,0.1) ;
#31667=CIRCLE('',#96858,0.0999999999999999) ;
#31668=CIRCLE('',#96860,0.1) ;
#31669=CIRCLE('',#96862,0.0999999999999992) ;
#31670=CIRCLE('',#96864,0.1) ;
#31671=CIRCLE('',#96866,0.1) ;
#31672=CIRCLE('',#96868,0.1) ;
#31673=CIRCLE('',#96871,0.1) ;
#31674=CIRCLE('',#96873,0.100000000000003) ;
#31675=CIRCLE('',#96875,0.0999999999999998) ;
#31676=CIRCLE('',#96877,0.100000000000003) ;
#31677=CIRCLE('',#96879,0.1) ;
#31678=CIRCLE('',#96881,0.1) ;
#31679=CIRCLE('',#96883,0.1) ;
#31680=CIRCLE('',#96885,0.1) ;
#31681=CIRCLE('',#96887,0.100000000000003) ;
#31682=CIRCLE('',#96889,0.100000000000003) ;
#31683=CIRCLE('',#96897,0.3) ;
#31684=CIRCLE('',#96898,0.9) ;
#31685=CIRCLE('',#96900,0.9) ;
#31686=CIRCLE('',#96901,0.3) ;
#31687=CIRCLE('',#96903,1.) ;
#31688=CIRCLE('',#96904,1.) ;
#31689=CIRCLE('',#96906,0.2) ;
#31690=CIRCLE('',#96907,0.2) ;
#31691=CIRCLE('',#96921,0.3) ;
#31692=CIRCLE('',#96922,0.9) ;
#31693=CIRCLE('',#96924,0.9) ;
#31694=CIRCLE('',#96925,0.3) ;
#31695=CIRCLE('',#96927,1.) ;
#31696=CIRCLE('',#96928,1.) ;
#31697=CIRCLE('',#96930,0.2) ;
#31698=CIRCLE('',#96931,0.2) ;
#31699=CIRCLE('',#96945,0.3) ;
#31700=CIRCLE('',#96946,0.9) ;
#31701=CIRCLE('',#96948,0.9) ;
#31702=CIRCLE('',#96949,0.3) ;
#31703=CIRCLE('',#96951,1.) ;
#31704=CIRCLE('',#96952,1.) ;
#31705=CIRCLE('',#96954,0.2) ;
#31706=CIRCLE('',#96955,0.2) ;
#31707=CIRCLE('',#96969,0.3) ;
#31708=CIRCLE('',#96970,0.9) ;
#31709=CIRCLE('',#96972,0.9) ;
#31710=CIRCLE('',#96973,0.3) ;
#31711=CIRCLE('',#96975,1.) ;
#31712=CIRCLE('',#96976,1.) ;
#31713=CIRCLE('',#96978,0.2) ;
#31714=CIRCLE('',#96979,0.2) ;
#31715=CIRCLE('',#96993,0.3) ;
#31716=CIRCLE('',#96994,0.9) ;
#31717=CIRCLE('',#96996,0.9) ;
#31718=CIRCLE('',#96997,0.3) ;
#31719=CIRCLE('',#96999,1.) ;
#31720=CIRCLE('',#97000,1.) ;
#31721=CIRCLE('',#97002,0.2) ;
#31722=CIRCLE('',#97003,0.2) ;
#31723=CIRCLE('',#97017,0.3) ;
#31724=CIRCLE('',#97018,0.9) ;
#31725=CIRCLE('',#97020,0.9) ;
#31726=CIRCLE('',#97021,0.3) ;
#31727=CIRCLE('',#97023,1.) ;
#31728=CIRCLE('',#97024,1.) ;
#31729=CIRCLE('',#97026,0.2) ;
#31730=CIRCLE('',#97027,0.2) ;
#31731=CIRCLE('',#97041,0.3) ;
#31732=CIRCLE('',#97042,0.9) ;
#31733=CIRCLE('',#97044,0.9) ;
#31734=CIRCLE('',#97045,0.3) ;
#31735=CIRCLE('',#97047,1.) ;
#31736=CIRCLE('',#97048,1.) ;
#31737=CIRCLE('',#97050,0.2) ;
#31738=CIRCLE('',#97051,0.2) ;
#31739=CIRCLE('',#97065,0.3) ;
#31740=CIRCLE('',#97066,0.9) ;
#31741=CIRCLE('',#97068,0.9) ;
#31742=CIRCLE('',#97069,0.3) ;
#31743=CIRCLE('',#97071,1.) ;
#31744=CIRCLE('',#97072,1.) ;
#31745=CIRCLE('',#97074,0.2) ;
#31746=CIRCLE('',#97075,0.2) ;
#31747=CIRCLE('',#97089,0.3) ;
#31748=CIRCLE('',#97090,0.9) ;
#31749=CIRCLE('',#97092,0.9) ;
#31750=CIRCLE('',#97093,0.3) ;
#31751=CIRCLE('',#97095,1.) ;
#31752=CIRCLE('',#97096,1.) ;
#31753=CIRCLE('',#97098,0.2) ;
#31754=CIRCLE('',#97099,0.2) ;
#31755=CIRCLE('',#97144,0.1) ;
#31756=CIRCLE('',#97145,0.0999999999999998) ;
#31757=CIRCLE('',#97147,0.1) ;
#31758=CIRCLE('',#97148,0.1) ;
#31759=CIRCLE('',#97150,0.0999999999999998) ;
#31760=CIRCLE('',#97151,0.1) ;
#31761=CIRCLE('',#97153,0.0999999999999999) ;
#31762=CIRCLE('',#97154,0.1) ;
#31763=CIRCLE('',#97156,0.1) ;
#31764=CIRCLE('',#97158,0.0999999999999998) ;
#31765=CIRCLE('',#97160,0.0999999999999998) ;
#31766=CIRCLE('',#97162,0.0999999999999999) ;
#31767=CIRCLE('',#97163,0.1) ;
#31768=CIRCLE('',#97165,0.0999999999999998) ;
#31769=CIRCLE('',#97167,0.1) ;
#31770=CIRCLE('',#97169,0.1) ;
#31771=CIRCLE('',#97171,0.0999999999999999) ;
#31772=CIRCLE('',#97173,0.1) ;
#31773=CIRCLE('',#97174,0.1) ;
#31774=CIRCLE('',#97176,0.1) ;
#31775=CIRCLE('',#97178,0.1) ;
#31776=CIRCLE('',#97179,0.0999999999999998) ;
#31777=CIRCLE('',#97181,0.1) ;
#31778=CIRCLE('',#97182,0.1) ;
#31779=CIRCLE('',#97184,0.0999999999999998) ;
#31780=CIRCLE('',#97185,0.1) ;
#31781=CIRCLE('',#97187,0.1) ;
#31782=CIRCLE('',#97188,0.1) ;
#31783=CIRCLE('',#97190,0.1) ;
#31784=CIRCLE('',#97192,0.1) ;
#31785=CIRCLE('',#97194,0.0999999999999998) ;
#31786=CIRCLE('',#97196,0.1) ;
#31787=CIRCLE('',#97197,0.1) ;
#31788=CIRCLE('',#97199,0.0999999999999998) ;
#31789=CIRCLE('',#97201,0.1) ;
#31790=CIRCLE('',#97203,0.1) ;
#31791=CIRCLE('',#97205,0.1) ;
#31792=CIRCLE('',#97207,0.1) ;
#31793=CIRCLE('',#97208,0.1) ;
#31794=CIRCLE('',#97210,0.1) ;
#31795=CIRCLE('',#97212,0.0999999999999997) ;
#31796=CIRCLE('',#97213,0.0999999999999999) ;
#31797=CIRCLE('',#97215,0.1) ;
#31798=CIRCLE('',#97216,0.1) ;
#31799=CIRCLE('',#97218,0.1) ;
#31800=CIRCLE('',#97219,0.1) ;
#31801=CIRCLE('',#97221,0.1) ;
#31802=CIRCLE('',#97222,0.1) ;
#31803=CIRCLE('',#97224,0.1) ;
#31804=CIRCLE('',#97226,0.1) ;
#31805=CIRCLE('',#97228,0.1) ;
#31806=CIRCLE('',#97230,0.1) ;
#31807=CIRCLE('',#97231,0.1) ;
#31808=CIRCLE('',#97233,0.1) ;
#31809=CIRCLE('',#97235,0.1) ;
#31810=CIRCLE('',#97237,0.1) ;
#31811=CIRCLE('',#97239,0.1) ;
#31812=CIRCLE('',#97241,0.1) ;
#31813=CIRCLE('',#97242,0.1) ;
#31814=CIRCLE('',#97244,0.1) ;
#31815=CIRCLE('',#97246,0.0999999999999999) ;
#31816=CIRCLE('',#97247,0.1) ;
#31817=CIRCLE('',#97249,0.1) ;
#31818=CIRCLE('',#97250,0.1) ;
#31819=CIRCLE('',#97252,0.1) ;
#31820=CIRCLE('',#97253,0.1) ;
#31821=CIRCLE('',#97255,0.1) ;
#31822=CIRCLE('',#97256,0.1) ;
#31823=CIRCLE('',#97258,0.1) ;
#31824=CIRCLE('',#97260,0.1) ;
#31825=CIRCLE('',#97262,0.1) ;
#31826=CIRCLE('',#97264,0.0999999999999999) ;
#31827=CIRCLE('',#97265,0.1) ;
#31828=CIRCLE('',#97267,0.1) ;
#31829=CIRCLE('',#97269,0.1) ;
#31830=CIRCLE('',#97271,0.1) ;
#31831=CIRCLE('',#97273,0.1) ;
#31832=CIRCLE('',#97275,0.1) ;
#31833=CIRCLE('',#97276,0.1) ;
#31834=CIRCLE('',#97278,0.0999999999999997) ;
#31835=CIRCLE('',#97280,0.0999999999999999) ;
#31836=CIRCLE('',#97281,0.1) ;
#31837=CIRCLE('',#97283,0.1) ;
#31838=CIRCLE('',#97284,0.1) ;
#31839=CIRCLE('',#97286,0.0999999999999994) ;
#31840=CIRCLE('',#97287,0.1) ;
#31841=CIRCLE('',#97289,0.1) ;
#31842=CIRCLE('',#97290,0.1) ;
#31843=CIRCLE('',#97292,0.1) ;
#31844=CIRCLE('',#97294,0.0999999999999994) ;
#31845=CIRCLE('',#97296,0.0999999999999994) ;
#31846=CIRCLE('',#97298,0.1) ;
#31847=CIRCLE('',#97299,0.1) ;
#31848=CIRCLE('',#97301,0.0999999999999994) ;
#31849=CIRCLE('',#97303,0.1) ;
#31850=CIRCLE('',#97305,0.1) ;
#31851=CIRCLE('',#97307,0.0999999999999998) ;
#31852=CIRCLE('',#97309,0.1) ;
#31853=CIRCLE('',#97310,0.1) ;
#31854=CIRCLE('',#97312,0.1) ;
#31855=CIRCLE('',#97314,0.1) ;
#31856=CIRCLE('',#97315,0.1) ;
#31857=CIRCLE('',#97317,0.1) ;
#31858=CIRCLE('',#97318,0.1) ;
#31859=CIRCLE('',#97320,0.0999999999999994) ;
#31860=CIRCLE('',#97321,0.1) ;
#31861=CIRCLE('',#97323,0.1) ;
#31862=CIRCLE('',#97324,0.1) ;
#31863=CIRCLE('',#97326,0.1) ;
#31864=CIRCLE('',#97328,0.1) ;
#31865=CIRCLE('',#97330,0.0999999999999994) ;
#31866=CIRCLE('',#97332,0.1) ;
#31867=CIRCLE('',#97333,0.1) ;
#31868=CIRCLE('',#97335,0.0999999999999994) ;
#31869=CIRCLE('',#97337,0.1) ;
#31870=CIRCLE('',#97339,0.1) ;
#31871=CIRCLE('',#97341,0.1) ;
#31872=CIRCLE('',#97343,0.1) ;
#31873=CIRCLE('',#97344,0.1) ;
#31874=CIRCLE('',#97346,0.100000000000001) ;
#31875=CIRCLE('',#97348,0.0999999999999999) ;
#31876=CIRCLE('',#97349,0.0999999999999999) ;
#31877=CIRCLE('',#97351,0.1) ;
#31878=CIRCLE('',#97352,0.1) ;
#31879=CIRCLE('',#97354,0.0999999999999994) ;
#31880=CIRCLE('',#97355,0.1) ;
#31881=CIRCLE('',#97357,0.1) ;
#31882=CIRCLE('',#97358,0.1) ;
#31883=CIRCLE('',#97360,0.1) ;
#31884=CIRCLE('',#97362,0.0999999999999994) ;
#31885=CIRCLE('',#97364,0.0999999999999994) ;
#31886=CIRCLE('',#97366,0.1) ;
#31887=CIRCLE('',#97367,0.1) ;
#31888=CIRCLE('',#97369,0.0999999999999994) ;
#31889=CIRCLE('',#97371,0.1) ;
#31890=CIRCLE('',#97373,0.1) ;
#31891=CIRCLE('',#97375,0.0999999999999999) ;
#31892=CIRCLE('',#97377,0.1) ;
#31893=CIRCLE('',#97378,0.1) ;
#31894=CIRCLE('',#97380,0.0999999999999998) ;
#31895=CIRCLE('',#97382,0.0999999999999999) ;
#31896=CIRCLE('',#97383,0.0999999999999998) ;
#31897=CIRCLE('',#97385,0.1) ;
#31898=CIRCLE('',#97386,0.1) ;
#31899=CIRCLE('',#97388,0.0999999999999994) ;
#31900=CIRCLE('',#97389,0.1) ;
#31901=CIRCLE('',#97391,0.1) ;
#31902=CIRCLE('',#97392,0.1) ;
#31903=CIRCLE('',#97394,0.1) ;
#31904=CIRCLE('',#97396,0.1) ;
#31905=CIRCLE('',#97398,0.0999999999999994) ;
#31906=CIRCLE('',#97400,0.1) ;
#31907=CIRCLE('',#97401,0.1) ;
#31908=CIRCLE('',#97403,0.0999999999999994) ;
#31909=CIRCLE('',#97405,0.1) ;
#31910=CIRCLE('',#97407,0.1) ;
#31911=CIRCLE('',#97409,0.0999999999999995) ;
#31912=CIRCLE('',#97411,0.1) ;
#31913=CIRCLE('',#97412,0.1) ;
#31914=CIRCLE('',#97414,0.1) ;
#31915=CIRCLE('',#97416,0.1) ;
#31916=CIRCLE('',#97417,0.0999999999999999) ;
#31917=CIRCLE('',#97419,0.1) ;
#31918=CIRCLE('',#97420,0.1) ;
#31919=CIRCLE('',#97422,0.0999999999999994) ;
#31920=CIRCLE('',#97423,0.1) ;
#31921=CIRCLE('',#97425,0.099999999999999) ;
#31922=CIRCLE('',#97426,0.1) ;
#31923=CIRCLE('',#97428,0.1) ;
#31924=CIRCLE('',#97430,0.0999999999999994) ;
#31925=CIRCLE('',#97432,0.0999999999999994) ;
#31926=CIRCLE('',#97434,0.0999999999999999) ;
#31927=CIRCLE('',#97435,0.1) ;
#31928=CIRCLE('',#97437,0.0999999999999994) ;
#31929=CIRCLE('',#97439,0.1) ;
#31930=CIRCLE('',#97441,0.099999999999999) ;
#31931=CIRCLE('',#97443,0.1) ;
#31932=CIRCLE('',#97445,0.1) ;
#31933=CIRCLE('',#97446,0.1) ;
#31934=CIRCLE('',#97448,0.0999999999999995) ;
#31935=CIRCLE('',#97450,0.0999999999999991) ;
#31936=CIRCLE('',#97451,0.0999999999999995) ;
#31937=CIRCLE('',#97453,0.1) ;
#31938=CIRCLE('',#97454,0.1) ;
#31939=CIRCLE('',#97456,0.0999999999999994) ;
#31940=CIRCLE('',#97457,0.1) ;
#31941=CIRCLE('',#97459,0.0999999999999989) ;
#31942=CIRCLE('',#97460,0.099999999999999) ;
#31943=CIRCLE('',#97462,0.1) ;
#31944=CIRCLE('',#97464,0.0999999999999994) ;
#31945=CIRCLE('',#97466,0.0999999999999994) ;
#31946=CIRCLE('',#97468,0.1) ;
#31947=CIRCLE('',#97469,0.1) ;
#31948=CIRCLE('',#97471,0.0999999999999994) ;
#31949=CIRCLE('',#97473,0.1) ;
#31950=CIRCLE('',#97475,0.0999999999999989) ;
#31951=CIRCLE('',#97477,0.0999999999999999) ;
#31952=CIRCLE('',#97479,0.1) ;
#31953=CIRCLE('',#97480,0.1) ;
#31954=CIRCLE('',#97482,0.0999999999999989) ;
#31955=CIRCLE('',#97484,0.1) ;
#31956=CIRCLE('',#97485,0.0999999999999999) ;
#31957=CIRCLE('',#97487,0.1) ;
#31958=CIRCLE('',#97488,0.1) ;
#31959=CIRCLE('',#97490,0.0999999999999994) ;
#31960=CIRCLE('',#97491,0.1) ;
#31961=CIRCLE('',#97493,0.099999999999999) ;
#31962=CIRCLE('',#97494,0.1) ;
#31963=CIRCLE('',#97496,0.1) ;
#31964=CIRCLE('',#97498,0.0999999999999994) ;
#31965=CIRCLE('',#97500,0.0999999999999994) ;
#31966=CIRCLE('',#97502,0.0999999999999999) ;
#31967=CIRCLE('',#97503,0.1) ;
#31968=CIRCLE('',#97505,0.0999999999999994) ;
#31969=CIRCLE('',#97507,0.1) ;
#31970=CIRCLE('',#97509,0.099999999999999) ;
#31971=CIRCLE('',#97511,0.1) ;
#31972=CIRCLE('',#97513,0.1) ;
#31973=CIRCLE('',#97514,0.1) ;
#31974=CIRCLE('',#97516,0.0999999999999995) ;
#31975=CIRCLE('',#97518,0.0999999999999991) ;
#31976=CIRCLE('',#97519,0.0999999999999995) ;
#31977=CIRCLE('',#97521,0.1) ;
#31978=CIRCLE('',#97522,0.1) ;
#31979=CIRCLE('',#97524,0.0999999999999994) ;
#31980=CIRCLE('',#97525,0.1) ;
#31981=CIRCLE('',#97527,0.0999999999999989) ;
#31982=CIRCLE('',#97528,0.099999999999999) ;
#31983=CIRCLE('',#97530,0.1) ;
#31984=CIRCLE('',#97532,0.0999999999999994) ;
#31985=CIRCLE('',#97534,0.0999999999999994) ;
#31986=CIRCLE('',#97536,0.1) ;
#31987=CIRCLE('',#97537,0.1) ;
#31988=CIRCLE('',#97539,0.0999999999999994) ;
#31989=CIRCLE('',#97541,0.1) ;
#31990=CIRCLE('',#97543,0.0999999999999989) ;
#31991=CIRCLE('',#97545,0.0999999999999999) ;
#31992=CIRCLE('',#97547,0.1) ;
#31993=CIRCLE('',#97548,0.1) ;
#31994=CIRCLE('',#97550,0.0999999999999989) ;
#31995=CIRCLE('',#97552,0.1) ;
#31996=CIRCLE('',#97553,0.0999999999999999) ;
#31997=CIRCLE('',#97555,0.1) ;
#31998=CIRCLE('',#97556,0.1) ;
#31999=CIRCLE('',#97558,0.0999999999999994) ;
#32000=CIRCLE('',#97559,0.1) ;
#32001=CIRCLE('',#97561,0.099999999999999) ;
#32002=CIRCLE('',#97562,0.1) ;
#32003=CIRCLE('',#97564,0.1) ;
#32004=CIRCLE('',#97566,0.0999999999999994) ;
#32005=CIRCLE('',#97568,0.0999999999999994) ;
#32006=CIRCLE('',#97570,0.0999999999999999) ;
#32007=CIRCLE('',#97571,0.1) ;
#32008=CIRCLE('',#97573,0.0999999999999994) ;
#32009=CIRCLE('',#97575,0.1) ;
#32010=CIRCLE('',#97577,0.099999999999999) ;
#32011=CIRCLE('',#97579,0.1) ;
#32012=CIRCLE('',#97581,0.1) ;
#32013=CIRCLE('',#97582,0.1) ;
#32014=CIRCLE('',#97584,0.0999999999999995) ;
#32015=CIRCLE('',#97586,0.0999999999999991) ;
#32016=CIRCLE('',#97587,0.0999999999999995) ;
#32017=CIRCLE('',#97589,0.1) ;
#32018=CIRCLE('',#97590,0.1) ;
#32019=CIRCLE('',#97592,0.0999999999999994) ;
#32020=CIRCLE('',#97593,0.1) ;
#32021=CIRCLE('',#97595,0.0999999999999989) ;
#32022=CIRCLE('',#97596,0.099999999999999) ;
#32023=CIRCLE('',#97598,0.1) ;
#32024=CIRCLE('',#97600,0.0999999999999994) ;
#32025=CIRCLE('',#97602,0.0999999999999994) ;
#32026=CIRCLE('',#97604,0.1) ;
#32027=CIRCLE('',#97605,0.1) ;
#32028=CIRCLE('',#97607,0.0999999999999994) ;
#32029=CIRCLE('',#97609,0.1) ;
#32030=CIRCLE('',#97611,0.0999999999999989) ;
#32031=CIRCLE('',#97613,0.0999999999999999) ;
#32032=CIRCLE('',#97615,0.1) ;
#32033=CIRCLE('',#97616,0.1) ;
#32034=CIRCLE('',#97618,0.0999999999999989) ;
#32035=CIRCLE('',#97620,0.1) ;
#32036=CIRCLE('',#97621,0.0999999999999999) ;
#32037=CIRCLE('',#97623,0.1) ;
#32038=CIRCLE('',#97624,0.1) ;
#32039=CIRCLE('',#97626,0.0999999999999994) ;
#32040=CIRCLE('',#97627,0.1) ;
#32041=CIRCLE('',#97629,0.099999999999999) ;
#32042=CIRCLE('',#97630,0.1) ;
#32043=CIRCLE('',#97632,0.1) ;
#32044=CIRCLE('',#97634,0.0999999999999994) ;
#32045=CIRCLE('',#97636,0.0999999999999994) ;
#32046=CIRCLE('',#97638,0.0999999999999999) ;
#32047=CIRCLE('',#97639,0.1) ;
#32048=CIRCLE('',#97641,0.0999999999999994) ;
#32049=CIRCLE('',#97643,0.1) ;
#32050=CIRCLE('',#97645,0.099999999999999) ;
#32051=CIRCLE('',#97647,0.1) ;
#32052=CIRCLE('',#97649,0.1) ;
#32053=CIRCLE('',#97650,0.1) ;
#32054=CIRCLE('',#97652,0.0999999999999995) ;
#32055=CIRCLE('',#97654,0.0999999999999991) ;
#32056=CIRCLE('',#97655,0.0999999999999995) ;
#32057=CIRCLE('',#97657,0.1) ;
#32058=CIRCLE('',#97658,0.1) ;
#32059=CIRCLE('',#97660,0.0999999999999994) ;
#32060=CIRCLE('',#97661,0.1) ;
#32061=CIRCLE('',#97663,0.0999999999999989) ;
#32062=CIRCLE('',#97664,0.099999999999999) ;
#32063=CIRCLE('',#97666,0.1) ;
#32064=CIRCLE('',#97668,0.0999999999999994) ;
#32065=CIRCLE('',#97670,0.0999999999999994) ;
#32066=CIRCLE('',#97672,0.1) ;
#32067=CIRCLE('',#97673,0.1) ;
#32068=CIRCLE('',#97675,0.0999999999999994) ;
#32069=CIRCLE('',#97677,0.1) ;
#32070=CIRCLE('',#97679,0.0999999999999989) ;
#32071=CIRCLE('',#97681,0.0999999999999999) ;
#32072=CIRCLE('',#97683,0.1) ;
#32073=CIRCLE('',#97684,0.1) ;
#32074=CIRCLE('',#97686,0.0999999999999989) ;
#32075=CIRCLE('',#97688,0.0999999999999997) ;
#32076=CIRCLE('',#97689,0.0999999999999995) ;
#32077=CIRCLE('',#97691,0.1) ;
#32078=CIRCLE('',#97692,0.1) ;
#32079=CIRCLE('',#97694,0.100000000000003) ;
#32080=CIRCLE('',#97695,0.1) ;
#32081=CIRCLE('',#97697,0.099999999999999) ;
#32082=CIRCLE('',#97698,0.100000000000001) ;
#32083=CIRCLE('',#97700,0.1) ;
#32084=CIRCLE('',#97702,0.100000000000003) ;
#32085=CIRCLE('',#97704,0.100000000000003) ;
#32086=CIRCLE('',#97706,0.0999999999999995) ;
#32087=CIRCLE('',#97707,0.1) ;
#32088=CIRCLE('',#97709,0.100000000000003) ;
#32089=CIRCLE('',#97711,0.1) ;
#32090=CIRCLE('',#97713,0.099999999999999) ;
#32091=CIRCLE('',#97715,0.1) ;
#32092=CIRCLE('',#97717,0.1) ;
#32093=CIRCLE('',#97718,0.1) ;
#32094=CIRCLE('',#97720,0.0999999999999999) ;
#32095=CIRCLE('',#97722,0.1) ;
#32096=CIRCLE('',#97723,0.0999999999999983) ;
#32097=CIRCLE('',#97725,0.1) ;
#32098=CIRCLE('',#97726,0.1) ;
#32099=CIRCLE('',#97728,0.100000000000003) ;
#32100=CIRCLE('',#97729,0.1) ;
#32101=CIRCLE('',#97731,0.0999999999999989) ;
#32102=CIRCLE('',#97732,0.0999999999999998) ;
#32103=CIRCLE('',#97734,0.1) ;
#32104=CIRCLE('',#97736,0.1) ;
#32105=CIRCLE('',#97738,0.100000000000003) ;
#32106=CIRCLE('',#97740,0.0999999999999998) ;
#32107=CIRCLE('',#97741,0.1) ;
#32108=CIRCLE('',#97743,0.100000000000003) ;
#32109=CIRCLE('',#97745,0.1) ;
#32110=CIRCLE('',#97747,0.0999999999999989) ;
#32111=CIRCLE('',#97749,0.1) ;
#32112=CIRCLE('',#97751,0.1) ;
#32113=CIRCLE('',#97752,0.1) ;
#32114=CIRCLE('',#97754,0.100000000000001) ;
#32115=CIRCLE('',#97756,0.1) ;
#32116=CIRCLE('',#97758,0.1) ;
#32117=CIRCLE('',#97760,0.1) ;
#32118=CIRCLE('',#97762,0.1) ;
#32119=CIRCLE('',#97764,0.1) ;
#32120=CIRCLE('',#97766,0.1) ;
#32121=CIRCLE('',#97769,0.0999999999999998) ;
#32122=CIRCLE('',#97771,0.0999999999999998) ;
#32123=CIRCLE('',#97773,0.1) ;
#32124=CIRCLE('',#97775,0.0999999999999998) ;
#32125=CIRCLE('',#97777,0.0999999999999998) ;
#32126=CIRCLE('',#97779,0.0999999999999998) ;
#32127=CIRCLE('',#97782,0.1) ;
#32128=CIRCLE('',#97784,0.1) ;
#32129=CIRCLE('',#97786,0.1) ;
#32130=CIRCLE('',#97788,0.1) ;
#32131=CIRCLE('',#97791,0.0999999999999998) ;
#32132=CIRCLE('',#97793,0.1) ;
#32133=CIRCLE('',#97795,0.0999999999999998) ;
#32134=CIRCLE('',#97797,0.0999999999999998) ;
#32135=CIRCLE('',#97800,0.0999999999999994) ;
#32136=CIRCLE('',#97802,0.0999999999999994) ;
#32137=CIRCLE('',#97804,0.1) ;
#32138=CIRCLE('',#97806,0.0999999999999994) ;
#32139=CIRCLE('',#97808,0.0999999999999994) ;
#32140=CIRCLE('',#97810,0.0999999999999994) ;
#32141=CIRCLE('',#97813,0.1) ;
#32142=CIRCLE('',#97815,0.1) ;
#32143=CIRCLE('',#97817,0.1) ;
#32144=CIRCLE('',#97819,0.1) ;
#32145=CIRCLE('',#97821,0.1) ;
#32146=CIRCLE('',#97823,0.1) ;
#32147=CIRCLE('',#97826,0.0999999999999994) ;
#32148=CIRCLE('',#97828,0.1) ;
#32149=CIRCLE('',#97830,0.0999999999999994) ;
#32150=CIRCLE('',#97832,0.0999999999999994) ;
#32151=CIRCLE('',#97835,0.1) ;
#32152=CIRCLE('',#97837,0.1) ;
#32153=CIRCLE('',#97839,0.1) ;
#32154=CIRCLE('',#97841,0.1) ;
#32155=CIRCLE('',#97844,0.0999999999999994) ;
#32156=CIRCLE('',#97846,0.0999999999999994) ;
#32157=CIRCLE('',#97848,0.1) ;
#32158=CIRCLE('',#97850,0.0999999999999994) ;
#32159=CIRCLE('',#97852,0.0999999999999994) ;
#32160=CIRCLE('',#97854,0.0999999999999994) ;
#32161=CIRCLE('',#97857,0.0999999999999994) ;
#32162=CIRCLE('',#97859,0.0999999999999994) ;
#32163=CIRCLE('',#97861,0.1) ;
#32164=CIRCLE('',#97863,0.0999999999999994) ;
#32165=CIRCLE('',#97865,0.0999999999999994) ;
#32166=CIRCLE('',#97867,0.0999999999999994) ;
#32167=CIRCLE('',#97870,0.0999999999999994) ;
#32168=CIRCLE('',#97872,0.1) ;
#32169=CIRCLE('',#97874,0.0999999999999994) ;
#32170=CIRCLE('',#97876,0.0999999999999994) ;
#32171=CIRCLE('',#97879,0.0999999999999994) ;
#32172=CIRCLE('',#97881,0.1) ;
#32173=CIRCLE('',#97883,0.0999999999999994) ;
#32174=CIRCLE('',#97885,0.0999999999999994) ;
#32175=CIRCLE('',#97888,0.0999999999999994) ;
#32176=CIRCLE('',#97890,0.0999999999999994) ;
#32177=CIRCLE('',#97892,0.0999999999999994) ;
#32178=CIRCLE('',#97894,0.0999999999999994) ;
#32179=CIRCLE('',#97896,0.0999999999999994) ;
#32180=CIRCLE('',#97898,0.0999999999999994) ;
#32181=CIRCLE('',#97901,0.0999999999999994) ;
#32182=CIRCLE('',#97903,0.0999999999999994) ;
#32183=CIRCLE('',#97905,0.1) ;
#32184=CIRCLE('',#97907,0.0999999999999994) ;
#32185=CIRCLE('',#97909,0.0999999999999994) ;
#32186=CIRCLE('',#97911,0.0999999999999994) ;
#32187=CIRCLE('',#97914,0.100000000000001) ;
#32188=CIRCLE('',#97916,0.1) ;
#32189=CIRCLE('',#97918,0.100000000000001) ;
#32190=CIRCLE('',#97920,0.0999999999999994) ;
#32191=CIRCLE('',#97923,0.0999999999999994) ;
#32192=CIRCLE('',#97925,0.1) ;
#32193=CIRCLE('',#97927,0.0999999999999994) ;
#32194=CIRCLE('',#97929,0.0999999999999994) ;
#32195=CIRCLE('',#97932,0.0999999999999994) ;
#32196=CIRCLE('',#97934,0.0999999999999994) ;
#32197=CIRCLE('',#97936,0.1) ;
#32198=CIRCLE('',#97938,0.0999999999999994) ;
#32199=CIRCLE('',#97940,0.0999999999999994) ;
#32200=CIRCLE('',#97942,0.0999999999999994) ;
#32201=CIRCLE('',#97945,0.0999999999999994) ;
#32202=CIRCLE('',#97947,0.0999999999999994) ;
#32203=CIRCLE('',#97949,0.1) ;
#32204=CIRCLE('',#97951,0.0999999999999994) ;
#32205=CIRCLE('',#97953,0.0999999999999994) ;
#32206=CIRCLE('',#97955,0.0999999999999994) ;
#32207=CIRCLE('',#97958,0.0999999999999994) ;
#32208=CIRCLE('',#97960,0.1) ;
#32209=CIRCLE('',#97962,0.0999999999999994) ;
#32210=CIRCLE('',#97964,0.0999999999999994) ;
#32211=CIRCLE('',#97967,0.0999999999999994) ;
#32212=CIRCLE('',#97969,0.1) ;
#32213=CIRCLE('',#97971,0.0999999999999994) ;
#32214=CIRCLE('',#97973,0.0999999999999994) ;
#32215=CIRCLE('',#97976,0.0999999999999994) ;
#32216=CIRCLE('',#97978,0.0999999999999994) ;
#32217=CIRCLE('',#97980,0.1) ;
#32218=CIRCLE('',#97982,0.0999999999999994) ;
#32219=CIRCLE('',#97984,0.0999999999999994) ;
#32220=CIRCLE('',#97986,0.0999999999999994) ;
#32221=CIRCLE('',#97989,0.0999999999999994) ;
#32222=CIRCLE('',#97991,0.0999999999999994) ;
#32223=CIRCLE('',#97993,0.1) ;
#32224=CIRCLE('',#97995,0.0999999999999994) ;
#32225=CIRCLE('',#97997,0.0999999999999994) ;
#32226=CIRCLE('',#97999,0.0999999999999994) ;
#32227=CIRCLE('',#98002,0.0999999999999994) ;
#32228=CIRCLE('',#98004,0.1) ;
#32229=CIRCLE('',#98006,0.0999999999999994) ;
#32230=CIRCLE('',#98008,0.0999999999999994) ;
#32231=CIRCLE('',#98011,0.0999999999999994) ;
#32232=CIRCLE('',#98013,0.1) ;
#32233=CIRCLE('',#98015,0.0999999999999994) ;
#32234=CIRCLE('',#98017,0.0999999999999994) ;
#32235=CIRCLE('',#98020,0.0999999999999994) ;
#32236=CIRCLE('',#98022,0.0999999999999994) ;
#32237=CIRCLE('',#98024,0.1) ;
#32238=CIRCLE('',#98026,0.0999999999999994) ;
#32239=CIRCLE('',#98028,0.0999999999999994) ;
#32240=CIRCLE('',#98030,0.0999999999999994) ;
#32241=CIRCLE('',#98033,0.0999999999999994) ;
#32242=CIRCLE('',#98035,0.0999999999999994) ;
#32243=CIRCLE('',#98037,0.1) ;
#32244=CIRCLE('',#98039,0.0999999999999994) ;
#32245=CIRCLE('',#98041,0.0999999999999994) ;
#32246=CIRCLE('',#98043,0.0999999999999994) ;
#32247=CIRCLE('',#98046,0.0999999999999994) ;
#32248=CIRCLE('',#98048,0.1) ;
#32249=CIRCLE('',#98050,0.0999999999999994) ;
#32250=CIRCLE('',#98052,0.0999999999999994) ;
#32251=CIRCLE('',#98055,0.0999999999999994) ;
#32252=CIRCLE('',#98057,0.1) ;
#32253=CIRCLE('',#98059,0.0999999999999994) ;
#32254=CIRCLE('',#98061,0.0999999999999994) ;
#32255=CIRCLE('',#98064,0.0999999999999994) ;
#32256=CIRCLE('',#98066,0.0999999999999994) ;
#32257=CIRCLE('',#98068,0.1) ;
#32258=CIRCLE('',#98070,0.0999999999999994) ;
#32259=CIRCLE('',#98072,0.0999999999999994) ;
#32260=CIRCLE('',#98074,0.0999999999999994) ;
#32261=CIRCLE('',#98077,0.0999999999999994) ;
#32262=CIRCLE('',#98079,0.0999999999999994) ;
#32263=CIRCLE('',#98081,0.1) ;
#32264=CIRCLE('',#98083,0.0999999999999994) ;
#32265=CIRCLE('',#98085,0.0999999999999994) ;
#32266=CIRCLE('',#98087,0.0999999999999994) ;
#32267=CIRCLE('',#98090,0.0999999999999994) ;
#32268=CIRCLE('',#98092,0.1) ;
#32269=CIRCLE('',#98094,0.0999999999999994) ;
#32270=CIRCLE('',#98096,0.0999999999999994) ;
#32271=CIRCLE('',#98099,0.0999999999999994) ;
#32272=CIRCLE('',#98101,0.1) ;
#32273=CIRCLE('',#98103,0.0999999999999994) ;
#32274=CIRCLE('',#98105,0.0999999999999994) ;
#32275=CIRCLE('',#98108,0.100000000000003) ;
#32276=CIRCLE('',#98110,0.100000000000003) ;
#32277=CIRCLE('',#98112,0.1) ;
#32278=CIRCLE('',#98114,0.100000000000003) ;
#32279=CIRCLE('',#98116,0.100000000000003) ;
#32280=CIRCLE('',#98118,0.100000000000003) ;
#32281=CIRCLE('',#98121,0.100000000000003) ;
#32282=CIRCLE('',#98123,0.100000000000003) ;
#32283=CIRCLE('',#98125,0.1) ;
#32284=CIRCLE('',#98127,0.100000000000003) ;
#32285=CIRCLE('',#98129,0.100000000000003) ;
#32286=CIRCLE('',#98131,0.100000000000003) ;
#32287=CIRCLE('',#98134,0.100000000000003) ;
#32288=CIRCLE('',#98136,0.1) ;
#32289=CIRCLE('',#98138,0.100000000000003) ;
#32290=CIRCLE('',#98140,0.100000000000003) ;
#32291=CIRCLE('',#98143,0.100000000000003) ;
#32292=CIRCLE('',#98145,0.1) ;
#32293=CIRCLE('',#98147,0.100000000000003) ;
#32294=CIRCLE('',#98149,0.100000000000003) ;
#36190=VERTEX_POINT('',#141828) ;
#36191=VERTEX_POINT('',#141830) ;
#36192=VERTEX_POINT('',#141832) ;
#36193=VERTEX_POINT('',#141836) ;
#36194=VERTEX_POINT('',#141838) ;
#36195=VERTEX_POINT('',#141842) ;
#36196=VERTEX_POINT('',#141843) ;
#36197=VERTEX_POINT('',#141845) ;
#36198=VERTEX_POINT('',#141849) ;
#36199=VERTEX_POINT('',#141850) ;
#36200=VERTEX_POINT('',#141852) ;
#36201=VERTEX_POINT('',#141854) ;
#36202=VERTEX_POINT('',#141856) ;
#36203=VERTEX_POINT('',#141858) ;
#36204=VERTEX_POINT('',#141860) ;
#36205=VERTEX_POINT('',#141871) ;
#36206=VERTEX_POINT('',#141873) ;
#36207=VERTEX_POINT('',#141875) ;
#36208=VERTEX_POINT('',#141879) ;
#36209=VERTEX_POINT('',#141881) ;
#36210=VERTEX_POINT('',#141885) ;
#36211=VERTEX_POINT('',#141886) ;
#36212=VERTEX_POINT('',#141888) ;
#36213=VERTEX_POINT('',#141892) ;
#36214=VERTEX_POINT('',#141893) ;
#36215=VERTEX_POINT('',#141895) ;
#36216=VERTEX_POINT('',#141897) ;
#36217=VERTEX_POINT('',#141899) ;
#36218=VERTEX_POINT('',#141901) ;
#36219=VERTEX_POINT('',#141903) ;
#36220=VERTEX_POINT('',#141914) ;
#36221=VERTEX_POINT('',#141916) ;
#36222=VERTEX_POINT('',#141918) ;
#36223=VERTEX_POINT('',#141922) ;
#36224=VERTEX_POINT('',#141924) ;
#36225=VERTEX_POINT('',#141928) ;
#36226=VERTEX_POINT('',#141929) ;
#36227=VERTEX_POINT('',#141931) ;
#36228=VERTEX_POINT('',#141935) ;
#36229=VERTEX_POINT('',#141936) ;
#36230=VERTEX_POINT('',#141938) ;
#36231=VERTEX_POINT('',#141940) ;
#36232=VERTEX_POINT('',#141942) ;
#36233=VERTEX_POINT('',#141944) ;
#36234=VERTEX_POINT('',#141946) ;
#36235=VERTEX_POINT('',#141957) ;
#36236=VERTEX_POINT('',#141959) ;
#36237=VERTEX_POINT('',#141961) ;
#36238=VERTEX_POINT('',#141965) ;
#36239=VERTEX_POINT('',#141967) ;
#36240=VERTEX_POINT('',#141971) ;
#36241=VERTEX_POINT('',#141972) ;
#36242=VERTEX_POINT('',#141974) ;
#36243=VERTEX_POINT('',#141978) ;
#36244=VERTEX_POINT('',#141979) ;
#36245=VERTEX_POINT('',#141981) ;
#36246=VERTEX_POINT('',#141983) ;
#36247=VERTEX_POINT('',#141985) ;
#36248=VERTEX_POINT('',#141987) ;
#36249=VERTEX_POINT('',#141989) ;
#36250=VERTEX_POINT('',#142000) ;
#36251=VERTEX_POINT('',#142002) ;
#36252=VERTEX_POINT('',#142004) ;
#36253=VERTEX_POINT('',#142008) ;
#36254=VERTEX_POINT('',#142010) ;
#36255=VERTEX_POINT('',#142014) ;
#36256=VERTEX_POINT('',#142015) ;
#36257=VERTEX_POINT('',#142017) ;
#36258=VERTEX_POINT('',#142021) ;
#36259=VERTEX_POINT('',#142022) ;
#36260=VERTEX_POINT('',#142024) ;
#36261=VERTEX_POINT('',#142026) ;
#36262=VERTEX_POINT('',#142028) ;
#36263=VERTEX_POINT('',#142030) ;
#36264=VERTEX_POINT('',#142032) ;
#36265=VERTEX_POINT('',#142043) ;
#36266=VERTEX_POINT('',#142045) ;
#36267=VERTEX_POINT('',#142047) ;
#36268=VERTEX_POINT('',#142051) ;
#36269=VERTEX_POINT('',#142053) ;
#36270=VERTEX_POINT('',#142057) ;
#36271=VERTEX_POINT('',#142058) ;
#36272=VERTEX_POINT('',#142060) ;
#36273=VERTEX_POINT('',#142064) ;
#36274=VERTEX_POINT('',#142065) ;
#36275=VERTEX_POINT('',#142067) ;
#36276=VERTEX_POINT('',#142069) ;
#36277=VERTEX_POINT('',#142071) ;
#36278=VERTEX_POINT('',#142073) ;
#36279=VERTEX_POINT('',#142075) ;
#36280=VERTEX_POINT('',#142086) ;
#36281=VERTEX_POINT('',#142088) ;
#36282=VERTEX_POINT('',#142090) ;
#36283=VERTEX_POINT('',#142094) ;
#36284=VERTEX_POINT('',#142096) ;
#36285=VERTEX_POINT('',#142100) ;
#36286=VERTEX_POINT('',#142101) ;
#36287=VERTEX_POINT('',#142103) ;
#36288=VERTEX_POINT('',#142107) ;
#36289=VERTEX_POINT('',#142108) ;
#36290=VERTEX_POINT('',#142110) ;
#36291=VERTEX_POINT('',#142112) ;
#36292=VERTEX_POINT('',#142114) ;
#36293=VERTEX_POINT('',#142116) ;
#36294=VERTEX_POINT('',#142118) ;
#36295=VERTEX_POINT('',#142129) ;
#36296=VERTEX_POINT('',#142131) ;
#36297=VERTEX_POINT('',#142133) ;
#36298=VERTEX_POINT('',#142137) ;
#36299=VERTEX_POINT('',#142139) ;
#36300=VERTEX_POINT('',#142143) ;
#36301=VERTEX_POINT('',#142144) ;
#36302=VERTEX_POINT('',#142146) ;
#36303=VERTEX_POINT('',#142150) ;
#36304=VERTEX_POINT('',#142151) ;
#36305=VERTEX_POINT('',#142153) ;
#36306=VERTEX_POINT('',#142155) ;
#36307=VERTEX_POINT('',#142157) ;
#36308=VERTEX_POINT('',#142159) ;
#36309=VERTEX_POINT('',#142161) ;
#36310=VERTEX_POINT('',#142172) ;
#36311=VERTEX_POINT('',#142174) ;
#36312=VERTEX_POINT('',#142176) ;
#36313=VERTEX_POINT('',#142180) ;
#36314=VERTEX_POINT('',#142181) ;
#36315=VERTEX_POINT('',#142183) ;
#36316=VERTEX_POINT('',#142185) ;
#36317=VERTEX_POINT('',#142189) ;
#36318=VERTEX_POINT('',#142190) ;
#36319=VERTEX_POINT('',#142192) ;
#36320=VERTEX_POINT('',#142194) ;
#36321=VERTEX_POINT('',#142198) ;
#36322=VERTEX_POINT('',#142199) ;
#36323=VERTEX_POINT('',#142201) ;
#36324=VERTEX_POINT('',#142203) ;
#36325=VERTEX_POINT('',#142207) ;
#36326=VERTEX_POINT('',#142208) ;
#36327=VERTEX_POINT('',#142210) ;
#36328=VERTEX_POINT('',#142212) ;
#36329=VERTEX_POINT('',#142216) ;
#36330=VERTEX_POINT('',#142217) ;
#36331=VERTEX_POINT('',#142219) ;
#36332=VERTEX_POINT('',#142221) ;
#36333=VERTEX_POINT('',#142225) ;
#36334=VERTEX_POINT('',#142226) ;
#36335=VERTEX_POINT('',#142228) ;
#36336=VERTEX_POINT('',#142230) ;
#36337=VERTEX_POINT('',#142234) ;
#36338=VERTEX_POINT('',#142235) ;
#36339=VERTEX_POINT('',#142237) ;
#36340=VERTEX_POINT('',#142239) ;
#36341=VERTEX_POINT('',#142243) ;
#36342=VERTEX_POINT('',#142244) ;
#36343=VERTEX_POINT('',#142246) ;
#36344=VERTEX_POINT('',#142248) ;
#36345=VERTEX_POINT('',#142252) ;
#36346=VERTEX_POINT('',#142253) ;
#36347=VERTEX_POINT('',#142255) ;
#36348=VERTEX_POINT('',#142257) ;
#36349=VERTEX_POINT('',#142261) ;
#36350=VERTEX_POINT('',#142263) ;
#36351=VERTEX_POINT('',#142267) ;
#36352=VERTEX_POINT('',#142268) ;
#36353=VERTEX_POINT('',#142270) ;
#36354=VERTEX_POINT('',#142274) ;
#36355=VERTEX_POINT('',#142275) ;
#36356=VERTEX_POINT('',#142277) ;
#36357=VERTEX_POINT('',#142279) ;
#36358=VERTEX_POINT('',#142281) ;
#36359=VERTEX_POINT('',#142283) ;
#36360=VERTEX_POINT('',#142285) ;
#36361=VERTEX_POINT('',#142314) ;
#36362=VERTEX_POINT('',#142315) ;
#36363=VERTEX_POINT('',#142320) ;
#36364=VERTEX_POINT('',#142321) ;
#36365=VERTEX_POINT('',#142326) ;
#36366=VERTEX_POINT('',#142327) ;
#36367=VERTEX_POINT('',#142332) ;
#36368=VERTEX_POINT('',#142333) ;
#36369=VERTEX_POINT('',#142338) ;
#36370=VERTEX_POINT('',#142339) ;
#36371=VERTEX_POINT('',#142344) ;
#36372=VERTEX_POINT('',#142345) ;
#36373=VERTEX_POINT('',#142350) ;
#36374=VERTEX_POINT('',#142351) ;
#36375=VERTEX_POINT('',#142356) ;
#36376=VERTEX_POINT('',#142357) ;
#36377=VERTEX_POINT('',#142362) ;
#36378=VERTEX_POINT('',#142363) ;
#36379=VERTEX_POINT('',#142368) ;
#36380=VERTEX_POINT('',#142370) ;
#36381=VERTEX_POINT('',#142372) ;
#36382=VERTEX_POINT('',#142376) ;
#36383=VERTEX_POINT('',#142377) ;
#36384=VERTEX_POINT('',#142379) ;
#36385=VERTEX_POINT('',#142381) ;
#36386=VERTEX_POINT('',#142385) ;
#36387=VERTEX_POINT('',#142387) ;
#36388=VERTEX_POINT('',#142391) ;
#36389=VERTEX_POINT('',#142392) ;
#36390=VERTEX_POINT('',#142394) ;
#36391=VERTEX_POINT('',#142398) ;
#36392=VERTEX_POINT('',#142399) ;
#36393=VERTEX_POINT('',#142401) ;
#36394=VERTEX_POINT('',#142403) ;
#36395=VERTEX_POINT('',#142405) ;
#36396=VERTEX_POINT('',#142407) ;
#36397=VERTEX_POINT('',#142409) ;
#36398=VERTEX_POINT('',#142422) ;
#36399=VERTEX_POINT('',#142423) ;
#36400=VERTEX_POINT('',#142428) ;
#36401=VERTEX_POINT('',#142429) ;
#36402=VERTEX_POINT('',#142431) ;
#36403=VERTEX_POINT('',#142433) ;
#36404=VERTEX_POINT('',#142436) ;
#36405=VERTEX_POINT('',#142438) ;
#36406=VERTEX_POINT('',#142440) ;
#36407=VERTEX_POINT('',#142442) ;
#36408=VERTEX_POINT('',#142444) ;
#36409=VERTEX_POINT('',#142446) ;
#36410=VERTEX_POINT('',#142450) ;
#36411=VERTEX_POINT('',#142451) ;
#36412=VERTEX_POINT('',#142453) ;
#36413=VERTEX_POINT('',#142455) ;
#36414=VERTEX_POINT('',#142458) ;
#36415=VERTEX_POINT('',#142460) ;
#36416=VERTEX_POINT('',#142462) ;
#36417=VERTEX_POINT('',#142464) ;
#36418=VERTEX_POINT('',#142466) ;
#36419=VERTEX_POINT('',#142468) ;
#36420=VERTEX_POINT('',#142472) ;
#36421=VERTEX_POINT('',#142473) ;
#36422=VERTEX_POINT('',#142475) ;
#36423=VERTEX_POINT('',#142477) ;
#36424=VERTEX_POINT('',#142480) ;
#36425=VERTEX_POINT('',#142482) ;
#36426=VERTEX_POINT('',#142484) ;
#36427=VERTEX_POINT('',#142486) ;
#36428=VERTEX_POINT('',#142488) ;
#36429=VERTEX_POINT('',#142490) ;
#36430=VERTEX_POINT('',#142494) ;
#36431=VERTEX_POINT('',#142495) ;
#36432=VERTEX_POINT('',#142497) ;
#36433=VERTEX_POINT('',#142499) ;
#36434=VERTEX_POINT('',#142502) ;
#36435=VERTEX_POINT('',#142504) ;
#36436=VERTEX_POINT('',#142506) ;
#36437=VERTEX_POINT('',#142508) ;
#36438=VERTEX_POINT('',#142510) ;
#36439=VERTEX_POINT('',#142512) ;
#36440=VERTEX_POINT('',#142516) ;
#36441=VERTEX_POINT('',#142517) ;
#36442=VERTEX_POINT('',#142519) ;
#36443=VERTEX_POINT('',#142521) ;
#36444=VERTEX_POINT('',#142524) ;
#36445=VERTEX_POINT('',#142526) ;
#36446=VERTEX_POINT('',#142528) ;
#36447=VERTEX_POINT('',#142530) ;
#36448=VERTEX_POINT('',#142532) ;
#36449=VERTEX_POINT('',#142534) ;
#36450=VERTEX_POINT('',#142538) ;
#36451=VERTEX_POINT('',#142539) ;
#36452=VERTEX_POINT('',#142541) ;
#36453=VERTEX_POINT('',#142543) ;
#36454=VERTEX_POINT('',#142546) ;
#36455=VERTEX_POINT('',#142548) ;
#36456=VERTEX_POINT('',#142550) ;
#36457=VERTEX_POINT('',#142552) ;
#36458=VERTEX_POINT('',#142554) ;
#36459=VERTEX_POINT('',#142556) ;
#36460=VERTEX_POINT('',#142560) ;
#36461=VERTEX_POINT('',#142561) ;
#36462=VERTEX_POINT('',#142563) ;
#36463=VERTEX_POINT('',#142565) ;
#36464=VERTEX_POINT('',#142568) ;
#36465=VERTEX_POINT('',#142570) ;
#36466=VERTEX_POINT('',#142572) ;
#36467=VERTEX_POINT('',#142574) ;
#36468=VERTEX_POINT('',#142576) ;
#36469=VERTEX_POINT('',#142578) ;
#36470=VERTEX_POINT('',#142582) ;
#36471=VERTEX_POINT('',#142583) ;
#36472=VERTEX_POINT('',#142585) ;
#36473=VERTEX_POINT('',#142587) ;
#36474=VERTEX_POINT('',#142590) ;
#36475=VERTEX_POINT('',#142592) ;
#36476=VERTEX_POINT('',#142594) ;
#36477=VERTEX_POINT('',#142596) ;
#36478=VERTEX_POINT('',#142598) ;
#36479=VERTEX_POINT('',#142600) ;
#36480=VERTEX_POINT('',#142604) ;
#36481=VERTEX_POINT('',#142605) ;
#36482=VERTEX_POINT('',#142607) ;
#36483=VERTEX_POINT('',#142609) ;
#36484=VERTEX_POINT('',#142612) ;
#36485=VERTEX_POINT('',#142614) ;
#36486=VERTEX_POINT('',#142616) ;
#36487=VERTEX_POINT('',#142618) ;
#36488=VERTEX_POINT('',#142620) ;
#36489=VERTEX_POINT('',#142622) ;
#36490=VERTEX_POINT('',#142626) ;
#36491=VERTEX_POINT('',#142627) ;
#36492=VERTEX_POINT('',#142629) ;
#36493=VERTEX_POINT('',#142631) ;
#36494=VERTEX_POINT('',#142633) ;
#36495=VERTEX_POINT('',#142637) ;
#36496=VERTEX_POINT('',#142638) ;
#36497=VERTEX_POINT('',#142640) ;
#36498=VERTEX_POINT('',#142642) ;
#36499=VERTEX_POINT('',#142644) ;
#36500=VERTEX_POINT('',#142648) ;
#36501=VERTEX_POINT('',#142649) ;
#36502=VERTEX_POINT('',#142651) ;
#36503=VERTEX_POINT('',#142653) ;
#36504=VERTEX_POINT('',#142655) ;
#36505=VERTEX_POINT('',#142659) ;
#36506=VERTEX_POINT('',#142660) ;
#36507=VERTEX_POINT('',#142662) ;
#36508=VERTEX_POINT('',#142664) ;
#36509=VERTEX_POINT('',#142666) ;
#36510=VERTEX_POINT('',#142670) ;
#36511=VERTEX_POINT('',#142671) ;
#36512=VERTEX_POINT('',#142673) ;
#36513=VERTEX_POINT('',#142675) ;
#36514=VERTEX_POINT('',#142677) ;
#36515=VERTEX_POINT('',#142681) ;
#36516=VERTEX_POINT('',#142682) ;
#36517=VERTEX_POINT('',#142684) ;
#36518=VERTEX_POINT('',#142686) ;
#36519=VERTEX_POINT('',#142688) ;
#36520=VERTEX_POINT('',#142692) ;
#36521=VERTEX_POINT('',#142693) ;
#36522=VERTEX_POINT('',#142695) ;
#36523=VERTEX_POINT('',#142697) ;
#36524=VERTEX_POINT('',#142699) ;
#36525=VERTEX_POINT('',#142703) ;
#36526=VERTEX_POINT('',#142704) ;
#36527=VERTEX_POINT('',#142706) ;
#36528=VERTEX_POINT('',#142708) ;
#36529=VERTEX_POINT('',#142710) ;
#36530=VERTEX_POINT('',#142714) ;
#36531=VERTEX_POINT('',#142715) ;
#36532=VERTEX_POINT('',#142717) ;
#36533=VERTEX_POINT('',#142719) ;
#36534=VERTEX_POINT('',#142721) ;
#36535=VERTEX_POINT('',#142725) ;
#36536=VERTEX_POINT('',#142726) ;
#36537=VERTEX_POINT('',#142728) ;
#36538=VERTEX_POINT('',#142730) ;
#36539=VERTEX_POINT('',#142732) ;
#36540=VERTEX_POINT('',#142736) ;
#36541=VERTEX_POINT('',#142737) ;
#36542=VERTEX_POINT('',#142739) ;
#36543=VERTEX_POINT('',#142741) ;
#36544=VERTEX_POINT('',#142743) ;
#36545=VERTEX_POINT('',#142747) ;
#36546=VERTEX_POINT('',#142748) ;
#36547=VERTEX_POINT('',#142750) ;
#36548=VERTEX_POINT('',#142752) ;
#36549=VERTEX_POINT('',#142754) ;
#36550=VERTEX_POINT('',#142758) ;
#36551=VERTEX_POINT('',#142759) ;
#36552=VERTEX_POINT('',#142761) ;
#36553=VERTEX_POINT('',#142763) ;
#36554=VERTEX_POINT('',#142765) ;
#36555=VERTEX_POINT('',#142769) ;
#36556=VERTEX_POINT('',#142770) ;
#36557=VERTEX_POINT('',#142772) ;
#36558=VERTEX_POINT('',#142774) ;
#36559=VERTEX_POINT('',#142776) ;
#36560=VERTEX_POINT('',#142780) ;
#36561=VERTEX_POINT('',#142781) ;
#36562=VERTEX_POINT('',#142783) ;
#36563=VERTEX_POINT('',#142785) ;
#36564=VERTEX_POINT('',#142787) ;
#36565=VERTEX_POINT('',#142791) ;
#36566=VERTEX_POINT('',#142792) ;
#36567=VERTEX_POINT('',#142794) ;
#36568=VERTEX_POINT('',#142796) ;
#36569=VERTEX_POINT('',#142798) ;
#36570=VERTEX_POINT('',#142802) ;
#36571=VERTEX_POINT('',#142803) ;
#36572=VERTEX_POINT('',#142805) ;
#36573=VERTEX_POINT('',#142807) ;
#36574=VERTEX_POINT('',#142809) ;
#36575=VERTEX_POINT('',#142813) ;
#36576=VERTEX_POINT('',#142814) ;
#36577=VERTEX_POINT('',#142816) ;
#36578=VERTEX_POINT('',#142818) ;
#36579=VERTEX_POINT('',#142820) ;
#36580=VERTEX_POINT('',#142824) ;
#36581=VERTEX_POINT('',#142825) ;
#36582=VERTEX_POINT('',#142827) ;
#36583=VERTEX_POINT('',#142829) ;
#36584=VERTEX_POINT('',#142833) ;
#36585=VERTEX_POINT('',#142834) ;
#36586=VERTEX_POINT('',#142836) ;
#36587=VERTEX_POINT('',#142838) ;
#36588=VERTEX_POINT('',#142842) ;
#36589=VERTEX_POINT('',#142843) ;
#36590=VERTEX_POINT('',#142845) ;
#36591=VERTEX_POINT('',#142847) ;
#36592=VERTEX_POINT('',#142851) ;
#36593=VERTEX_POINT('',#142852) ;
#36594=VERTEX_POINT('',#142854) ;
#36595=VERTEX_POINT('',#142856) ;
#36596=VERTEX_POINT('',#142860) ;
#36597=VERTEX_POINT('',#142861) ;
#36598=VERTEX_POINT('',#142863) ;
#36599=VERTEX_POINT('',#142865) ;
#36600=VERTEX_POINT('',#142869) ;
#36601=VERTEX_POINT('',#142870) ;
#36602=VERTEX_POINT('',#142872) ;
#36603=VERTEX_POINT('',#142874) ;
#36604=VERTEX_POINT('',#142878) ;
#36605=VERTEX_POINT('',#142879) ;
#36606=VERTEX_POINT('',#142881) ;
#36607=VERTEX_POINT('',#142883) ;
#36608=VERTEX_POINT('',#142887) ;
#36609=VERTEX_POINT('',#142888) ;
#36610=VERTEX_POINT('',#142890) ;
#36611=VERTEX_POINT('',#142892) ;
#36612=VERTEX_POINT('',#142896) ;
#36613=VERTEX_POINT('',#142897) ;
#36614=VERTEX_POINT('',#142899) ;
#36615=VERTEX_POINT('',#142901) ;
#36616=VERTEX_POINT('',#142905) ;
#36617=VERTEX_POINT('',#142906) ;
#36618=VERTEX_POINT('',#142908) ;
#36619=VERTEX_POINT('',#142910) ;
#36620=VERTEX_POINT('',#142913) ;
#36621=VERTEX_POINT('',#142915) ;
#36622=VERTEX_POINT('',#142917) ;
#36623=VERTEX_POINT('',#142919) ;
#36624=VERTEX_POINT('',#142921) ;
#36625=VERTEX_POINT('',#142923) ;
#36626=VERTEX_POINT('',#142927) ;
#36627=VERTEX_POINT('',#142928) ;
#36628=VERTEX_POINT('',#142930) ;
#36629=VERTEX_POINT('',#142932) ;
#36630=VERTEX_POINT('',#142934) ;
#36631=VERTEX_POINT('',#142938) ;
#36632=VERTEX_POINT('',#142939) ;
#36633=VERTEX_POINT('',#142941) ;
#36634=VERTEX_POINT('',#142943) ;
#36635=VERTEX_POINT('',#142945) ;
#36636=VERTEX_POINT('',#142949) ;
#36637=VERTEX_POINT('',#142950) ;
#36638=VERTEX_POINT('',#142952) ;
#36639=VERTEX_POINT('',#142954) ;
#36640=VERTEX_POINT('',#142958) ;
#36641=VERTEX_POINT('',#142959) ;
#36642=VERTEX_POINT('',#142961) ;
#36643=VERTEX_POINT('',#142963) ;
#36644=VERTEX_POINT('',#142967) ;
#36645=VERTEX_POINT('',#142968) ;
#36646=VERTEX_POINT('',#142970) ;
#36647=VERTEX_POINT('',#142972) ;
#36648=VERTEX_POINT('',#142976) ;
#36649=VERTEX_POINT('',#142978) ;
#36650=VERTEX_POINT('',#142980) ;
#36651=VERTEX_POINT('',#142982) ;
#36652=VERTEX_POINT('',#142985) ;
#36653=VERTEX_POINT('',#142987) ;
#36654=VERTEX_POINT('',#142989) ;
#36655=VERTEX_POINT('',#142991) ;
#36656=VERTEX_POINT('',#142994) ;
#36657=VERTEX_POINT('',#142996) ;
#36658=VERTEX_POINT('',#142998) ;
#36659=VERTEX_POINT('',#143000) ;
#36660=VERTEX_POINT('',#143003) ;
#36661=VERTEX_POINT('',#143005) ;
#36662=VERTEX_POINT('',#143007) ;
#36663=VERTEX_POINT('',#143009) ;
#36664=VERTEX_POINT('',#143012) ;
#36665=VERTEX_POINT('',#143014) ;
#36666=VERTEX_POINT('',#143016) ;
#36667=VERTEX_POINT('',#143018) ;
#36668=VERTEX_POINT('',#143021) ;
#36669=VERTEX_POINT('',#143023) ;
#36670=VERTEX_POINT('',#143025) ;
#36671=VERTEX_POINT('',#143027) ;
#36672=VERTEX_POINT('',#143030) ;
#36673=VERTEX_POINT('',#143032) ;
#36674=VERTEX_POINT('',#143034) ;
#36675=VERTEX_POINT('',#143036) ;
#36676=VERTEX_POINT('',#143039) ;
#36677=VERTEX_POINT('',#143041) ;
#36678=VERTEX_POINT('',#143043) ;
#36679=VERTEX_POINT('',#143045) ;
#36680=VERTEX_POINT('',#143048) ;
#36681=VERTEX_POINT('',#143050) ;
#36682=VERTEX_POINT('',#143052) ;
#36683=VERTEX_POINT('',#143054) ;
#36684=VERTEX_POINT('',#143057) ;
#36685=VERTEX_POINT('',#143059) ;
#36686=VERTEX_POINT('',#143063) ;
#36687=VERTEX_POINT('',#143065) ;
#36688=VERTEX_POINT('',#143069) ;
#36689=VERTEX_POINT('',#143070) ;
#36690=VERTEX_POINT('',#143073) ;
#36691=VERTEX_POINT('',#143075) ;
#36692=VERTEX_POINT('',#143077) ;
#36693=VERTEX_POINT('',#143079) ;
#36694=VERTEX_POINT('',#143082) ;
#36695=VERTEX_POINT('',#143084) ;
#36696=VERTEX_POINT('',#143086) ;
#36697=VERTEX_POINT('',#143088) ;
#36698=VERTEX_POINT('',#143091) ;
#36699=VERTEX_POINT('',#143093) ;
#36700=VERTEX_POINT('',#143095) ;
#36701=VERTEX_POINT('',#143097) ;
#36702=VERTEX_POINT('',#143100) ;
#36703=VERTEX_POINT('',#143102) ;
#36704=VERTEX_POINT('',#143104) ;
#36705=VERTEX_POINT('',#143106) ;
#36706=VERTEX_POINT('',#143109) ;
#36707=VERTEX_POINT('',#143111) ;
#36708=VERTEX_POINT('',#143113) ;
#36709=VERTEX_POINT('',#143115) ;
#36710=VERTEX_POINT('',#143118) ;
#36711=VERTEX_POINT('',#143120) ;
#36712=VERTEX_POINT('',#143122) ;
#36713=VERTEX_POINT('',#143124) ;
#36714=VERTEX_POINT('',#143127) ;
#36715=VERTEX_POINT('',#143129) ;
#36716=VERTEX_POINT('',#143131) ;
#36717=VERTEX_POINT('',#143133) ;
#36718=VERTEX_POINT('',#143136) ;
#36719=VERTEX_POINT('',#143138) ;
#36720=VERTEX_POINT('',#143140) ;
#36721=VERTEX_POINT('',#143142) ;
#36722=VERTEX_POINT('',#143145) ;
#36723=VERTEX_POINT('',#143147) ;
#36724=VERTEX_POINT('',#143149) ;
#36725=VERTEX_POINT('',#143151) ;
#36726=VERTEX_POINT('',#143154) ;
#36727=VERTEX_POINT('',#143156) ;
#36728=VERTEX_POINT('',#143159) ;
#36729=VERTEX_POINT('',#143161) ;
#36730=VERTEX_POINT('',#143165) ;
#36731=VERTEX_POINT('',#143166) ;
#36732=VERTEX_POINT('',#143171) ;
#36733=VERTEX_POINT('',#143172) ;
#36734=VERTEX_POINT('',#143177) ;
#36735=VERTEX_POINT('',#143178) ;
#36736=VERTEX_POINT('',#143183) ;
#36737=VERTEX_POINT('',#143184) ;
#36738=VERTEX_POINT('',#143189) ;
#36739=VERTEX_POINT('',#143190) ;
#36740=VERTEX_POINT('',#143195) ;
#36741=VERTEX_POINT('',#143196) ;
#36742=VERTEX_POINT('',#143201) ;
#36743=VERTEX_POINT('',#143202) ;
#36744=VERTEX_POINT('',#143207) ;
#36745=VERTEX_POINT('',#143208) ;
#36746=VERTEX_POINT('',#143213) ;
#36747=VERTEX_POINT('',#143214) ;
#36748=VERTEX_POINT('',#143219) ;
#36749=VERTEX_POINT('',#143220) ;
#36750=VERTEX_POINT('',#143225) ;
#36751=VERTEX_POINT('',#143226) ;
#36752=VERTEX_POINT('',#143233) ;
#36753=VERTEX_POINT('',#143234) ;
#36754=VERTEX_POINT('',#143236) ;
#36755=VERTEX_POINT('',#143238) ;
#36756=VERTEX_POINT('',#143240) ;
#36757=VERTEX_POINT('',#143242) ;
#36758=VERTEX_POINT('',#143244) ;
#36759=VERTEX_POINT('',#143246) ;
#36760=VERTEX_POINT('',#143249) ;
#36761=VERTEX_POINT('',#143251) ;
#36762=VERTEX_POINT('',#143253) ;
#36763=VERTEX_POINT('',#143255) ;
#36764=VERTEX_POINT('',#143257) ;
#36765=VERTEX_POINT('',#143259) ;
#36766=VERTEX_POINT('',#143261) ;
#36767=VERTEX_POINT('',#143263) ;
#36768=VERTEX_POINT('',#143265) ;
#36769=VERTEX_POINT('',#143267) ;
#36770=VERTEX_POINT('',#143269) ;
#36771=VERTEX_POINT('',#143271) ;
#36772=VERTEX_POINT('',#143273) ;
#36773=VERTEX_POINT('',#143275) ;
#36774=VERTEX_POINT('',#143278) ;
#36775=VERTEX_POINT('',#143279) ;
#36776=VERTEX_POINT('',#143281) ;
#36777=VERTEX_POINT('',#143283) ;
#36778=VERTEX_POINT('',#143285) ;
#36779=VERTEX_POINT('',#143287) ;
#36780=VERTEX_POINT('',#143289) ;
#36781=VERTEX_POINT('',#143291) ;
#36782=VERTEX_POINT('',#143294) ;
#36783=VERTEX_POINT('',#143296) ;
#36784=VERTEX_POINT('',#143298) ;
#36785=VERTEX_POINT('',#143300) ;
#36786=VERTEX_POINT('',#143302) ;
#36787=VERTEX_POINT('',#143304) ;
#36788=VERTEX_POINT('',#143306) ;
#36789=VERTEX_POINT('',#143308) ;
#36790=VERTEX_POINT('',#143310) ;
#36791=VERTEX_POINT('',#143312) ;
#36792=VERTEX_POINT('',#143314) ;
#36793=VERTEX_POINT('',#143316) ;
#36794=VERTEX_POINT('',#143318) ;
#36795=VERTEX_POINT('',#143320) ;
#36796=VERTEX_POINT('',#143323) ;
#36797=VERTEX_POINT('',#143324) ;
#36798=VERTEX_POINT('',#143326) ;
#36799=VERTEX_POINT('',#143328) ;
#36800=VERTEX_POINT('',#143330) ;
#36801=VERTEX_POINT('',#143332) ;
#36802=VERTEX_POINT('',#143334) ;
#36803=VERTEX_POINT('',#143336) ;
#36804=VERTEX_POINT('',#143339) ;
#36805=VERTEX_POINT('',#143341) ;
#36806=VERTEX_POINT('',#143343) ;
#36807=VERTEX_POINT('',#143345) ;
#36808=VERTEX_POINT('',#143347) ;
#36809=VERTEX_POINT('',#143349) ;
#36810=VERTEX_POINT('',#143351) ;
#36811=VERTEX_POINT('',#143353) ;
#36812=VERTEX_POINT('',#143355) ;
#36813=VERTEX_POINT('',#143357) ;
#36814=VERTEX_POINT('',#143359) ;
#36815=VERTEX_POINT('',#143361) ;
#36816=VERTEX_POINT('',#143363) ;
#36817=VERTEX_POINT('',#143365) ;
#36818=VERTEX_POINT('',#143368) ;
#36819=VERTEX_POINT('',#143369) ;
#36820=VERTEX_POINT('',#143371) ;
#36821=VERTEX_POINT('',#143373) ;
#36822=VERTEX_POINT('',#143375) ;
#36823=VERTEX_POINT('',#143377) ;
#36824=VERTEX_POINT('',#143379) ;
#36825=VERTEX_POINT('',#143381) ;
#36826=VERTEX_POINT('',#143384) ;
#36827=VERTEX_POINT('',#143386) ;
#36828=VERTEX_POINT('',#143388) ;
#36829=VERTEX_POINT('',#143390) ;
#36830=VERTEX_POINT('',#143392) ;
#36831=VERTEX_POINT('',#143394) ;
#36832=VERTEX_POINT('',#143396) ;
#36833=VERTEX_POINT('',#143398) ;
#36834=VERTEX_POINT('',#143400) ;
#36835=VERTEX_POINT('',#143402) ;
#36836=VERTEX_POINT('',#143404) ;
#36837=VERTEX_POINT('',#143406) ;
#36838=VERTEX_POINT('',#143408) ;
#36839=VERTEX_POINT('',#143410) ;
#36840=VERTEX_POINT('',#143413) ;
#36841=VERTEX_POINT('',#143414) ;
#36842=VERTEX_POINT('',#143416) ;
#36843=VERTEX_POINT('',#143418) ;
#36844=VERTEX_POINT('',#143420) ;
#36845=VERTEX_POINT('',#143422) ;
#36846=VERTEX_POINT('',#143424) ;
#36847=VERTEX_POINT('',#143426) ;
#36848=VERTEX_POINT('',#143429) ;
#36849=VERTEX_POINT('',#143431) ;
#36850=VERTEX_POINT('',#143433) ;
#36851=VERTEX_POINT('',#143435) ;
#36852=VERTEX_POINT('',#143437) ;
#36853=VERTEX_POINT('',#143439) ;
#36854=VERTEX_POINT('',#143441) ;
#36855=VERTEX_POINT('',#143443) ;
#36856=VERTEX_POINT('',#143445) ;
#36857=VERTEX_POINT('',#143447) ;
#36858=VERTEX_POINT('',#143449) ;
#36859=VERTEX_POINT('',#143451) ;
#36860=VERTEX_POINT('',#143453) ;
#36861=VERTEX_POINT('',#143455) ;
#36862=VERTEX_POINT('',#143458) ;
#36863=VERTEX_POINT('',#143459) ;
#36864=VERTEX_POINT('',#143461) ;
#36865=VERTEX_POINT('',#143463) ;
#36866=VERTEX_POINT('',#143465) ;
#36867=VERTEX_POINT('',#143467) ;
#36868=VERTEX_POINT('',#143469) ;
#36869=VERTEX_POINT('',#143471) ;
#36870=VERTEX_POINT('',#143474) ;
#36871=VERTEX_POINT('',#143476) ;
#36872=VERTEX_POINT('',#143478) ;
#36873=VERTEX_POINT('',#143480) ;
#36874=VERTEX_POINT('',#143482) ;
#36875=VERTEX_POINT('',#143484) ;
#36876=VERTEX_POINT('',#143486) ;
#36877=VERTEX_POINT('',#143488) ;
#36878=VERTEX_POINT('',#143490) ;
#36879=VERTEX_POINT('',#143492) ;
#36880=VERTEX_POINT('',#143494) ;
#36881=VERTEX_POINT('',#143496) ;
#36882=VERTEX_POINT('',#143498) ;
#36883=VERTEX_POINT('',#143500) ;
#36884=VERTEX_POINT('',#143503) ;
#36885=VERTEX_POINT('',#143504) ;
#36886=VERTEX_POINT('',#143506) ;
#36887=VERTEX_POINT('',#143508) ;
#36888=VERTEX_POINT('',#143510) ;
#36889=VERTEX_POINT('',#143512) ;
#36890=VERTEX_POINT('',#143514) ;
#36891=VERTEX_POINT('',#143516) ;
#36892=VERTEX_POINT('',#143519) ;
#36893=VERTEX_POINT('',#143521) ;
#36894=VERTEX_POINT('',#143523) ;
#36895=VERTEX_POINT('',#143525) ;
#36896=VERTEX_POINT('',#143527) ;
#36897=VERTEX_POINT('',#143529) ;
#36898=VERTEX_POINT('',#143531) ;
#36899=VERTEX_POINT('',#143533) ;
#36900=VERTEX_POINT('',#143535) ;
#36901=VERTEX_POINT('',#143537) ;
#36902=VERTEX_POINT('',#143539) ;
#36903=VERTEX_POINT('',#143541) ;
#36904=VERTEX_POINT('',#143543) ;
#36905=VERTEX_POINT('',#143545) ;
#36906=VERTEX_POINT('',#143548) ;
#36907=VERTEX_POINT('',#143549) ;
#36908=VERTEX_POINT('',#143551) ;
#36909=VERTEX_POINT('',#143553) ;
#36910=VERTEX_POINT('',#143555) ;
#36911=VERTEX_POINT('',#143557) ;
#36912=VERTEX_POINT('',#143559) ;
#36913=VERTEX_POINT('',#143561) ;
#36914=VERTEX_POINT('',#143564) ;
#36915=VERTEX_POINT('',#143566) ;
#36916=VERTEX_POINT('',#143568) ;
#36917=VERTEX_POINT('',#143570) ;
#36918=VERTEX_POINT('',#143572) ;
#36919=VERTEX_POINT('',#143574) ;
#36920=VERTEX_POINT('',#143576) ;
#36921=VERTEX_POINT('',#143578) ;
#36922=VERTEX_POINT('',#143580) ;
#36923=VERTEX_POINT('',#143582) ;
#36924=VERTEX_POINT('',#143584) ;
#36925=VERTEX_POINT('',#143586) ;
#36926=VERTEX_POINT('',#143588) ;
#36927=VERTEX_POINT('',#143590) ;
#36928=VERTEX_POINT('',#143593) ;
#36929=VERTEX_POINT('',#143594) ;
#36930=VERTEX_POINT('',#143596) ;
#36931=VERTEX_POINT('',#143598) ;
#36932=VERTEX_POINT('',#143600) ;
#36933=VERTEX_POINT('',#143602) ;
#36934=VERTEX_POINT('',#143604) ;
#36935=VERTEX_POINT('',#143606) ;
#36936=VERTEX_POINT('',#143609) ;
#36937=VERTEX_POINT('',#143611) ;
#36938=VERTEX_POINT('',#143613) ;
#36939=VERTEX_POINT('',#143615) ;
#36940=VERTEX_POINT('',#143617) ;
#36941=VERTEX_POINT('',#143619) ;
#36942=VERTEX_POINT('',#143621) ;
#36943=VERTEX_POINT('',#143623) ;
#36944=VERTEX_POINT('',#143625) ;
#36945=VERTEX_POINT('',#143627) ;
#36946=VERTEX_POINT('',#143629) ;
#36947=VERTEX_POINT('',#143631) ;
#36948=VERTEX_POINT('',#143633) ;
#36949=VERTEX_POINT('',#143635) ;
#36950=VERTEX_POINT('',#143638) ;
#36951=VERTEX_POINT('',#143639) ;
#36952=VERTEX_POINT('',#143641) ;
#36953=VERTEX_POINT('',#143643) ;
#36954=VERTEX_POINT('',#143645) ;
#36955=VERTEX_POINT('',#143647) ;
#36956=VERTEX_POINT('',#143649) ;
#36957=VERTEX_POINT('',#143651) ;
#36958=VERTEX_POINT('',#143654) ;
#36959=VERTEX_POINT('',#143656) ;
#36960=VERTEX_POINT('',#143658) ;
#36961=VERTEX_POINT('',#143660) ;
#36962=VERTEX_POINT('',#143662) ;
#36963=VERTEX_POINT('',#143664) ;
#36964=VERTEX_POINT('',#143666) ;
#36965=VERTEX_POINT('',#143668) ;
#36966=VERTEX_POINT('',#143670) ;
#36967=VERTEX_POINT('',#143672) ;
#36968=VERTEX_POINT('',#143674) ;
#36969=VERTEX_POINT('',#143676) ;
#36970=VERTEX_POINT('',#143678) ;
#36971=VERTEX_POINT('',#143680) ;
#36972=VERTEX_POINT('',#143684) ;
#36973=VERTEX_POINT('',#143685) ;
#36974=VERTEX_POINT('',#143687) ;
#36975=VERTEX_POINT('',#143689) ;
#36976=VERTEX_POINT('',#143691) ;
#36977=VERTEX_POINT('',#143693) ;
#36978=VERTEX_POINT('',#143695) ;
#36979=VERTEX_POINT('',#143697) ;
#36980=VERTEX_POINT('',#143699) ;
#36981=VERTEX_POINT('',#143701) ;
#36982=VERTEX_POINT('',#143705) ;
#36983=VERTEX_POINT('',#143706) ;
#36984=VERTEX_POINT('',#143708) ;
#36985=VERTEX_POINT('',#143710) ;
#36986=VERTEX_POINT('',#143712) ;
#36987=VERTEX_POINT('',#143714) ;
#36988=VERTEX_POINT('',#143716) ;
#36989=VERTEX_POINT('',#143718) ;
#36990=VERTEX_POINT('',#143720) ;
#36991=VERTEX_POINT('',#143722) ;
#36992=VERTEX_POINT('',#143726) ;
#36993=VERTEX_POINT('',#143727) ;
#36994=VERTEX_POINT('',#143729) ;
#36995=VERTEX_POINT('',#143731) ;
#36996=VERTEX_POINT('',#143733) ;
#36997=VERTEX_POINT('',#143735) ;
#36998=VERTEX_POINT('',#143737) ;
#36999=VERTEX_POINT('',#143739) ;
#37000=VERTEX_POINT('',#143741) ;
#37001=VERTEX_POINT('',#143743) ;
#37002=VERTEX_POINT('',#143747) ;
#37003=VERTEX_POINT('',#143748) ;
#37004=VERTEX_POINT('',#143750) ;
#37005=VERTEX_POINT('',#143752) ;
#37006=VERTEX_POINT('',#143756) ;
#37007=VERTEX_POINT('',#143758) ;
#37008=VERTEX_POINT('',#143762) ;
#37009=VERTEX_POINT('',#143763) ;
#37010=VERTEX_POINT('',#143765) ;
#37011=VERTEX_POINT('',#143767) ;
#37012=VERTEX_POINT('',#143771) ;
#37013=VERTEX_POINT('',#143772) ;
#37014=VERTEX_POINT('',#143774) ;
#37015=VERTEX_POINT('',#143776) ;
#37016=VERTEX_POINT('',#143780) ;
#37017=VERTEX_POINT('',#143781) ;
#37018=VERTEX_POINT('',#143783) ;
#37019=VERTEX_POINT('',#143785) ;
#37020=VERTEX_POINT('',#143789) ;
#37021=VERTEX_POINT('',#143790) ;
#37022=VERTEX_POINT('',#143792) ;
#37023=VERTEX_POINT('',#143794) ;
#37024=VERTEX_POINT('',#143798) ;
#37025=VERTEX_POINT('',#143800) ;
#37026=VERTEX_POINT('',#143804) ;
#37027=VERTEX_POINT('',#143806) ;
#37028=VERTEX_POINT('',#143810) ;
#37029=VERTEX_POINT('',#143812) ;
#37030=VERTEX_POINT('',#143816) ;
#37031=VERTEX_POINT('',#143818) ;
#37032=VERTEX_POINT('',#143823) ;
#37033=VERTEX_POINT('',#143827) ;
#37034=VERTEX_POINT('',#143834) ;
#37035=VERTEX_POINT('',#143836) ;
#37036=VERTEX_POINT('',#143840) ;
#37037=VERTEX_POINT('',#143842) ;
#37038=VERTEX_POINT('',#143846) ;
#37039=VERTEX_POINT('',#143848) ;
#37040=VERTEX_POINT('',#143852) ;
#37041=VERTEX_POINT('',#143854) ;
#37042=VERTEX_POINT('',#143858) ;
#37043=VERTEX_POINT('',#143860) ;
#37044=VERTEX_POINT('',#143864) ;
#37045=VERTEX_POINT('',#143866) ;
#37046=VERTEX_POINT('',#143870) ;
#37047=VERTEX_POINT('',#143872) ;
#37048=VERTEX_POINT('',#143876) ;
#37049=VERTEX_POINT('',#143878) ;
#37050=VERTEX_POINT('',#143882) ;
#37051=VERTEX_POINT('',#143884) ;
#37052=VERTEX_POINT('',#143888) ;
#37053=VERTEX_POINT('',#143890) ;
#37054=VERTEX_POINT('',#143894) ;
#37055=VERTEX_POINT('',#143896) ;
#37056=VERTEX_POINT('',#143900) ;
#37057=VERTEX_POINT('',#143902) ;
#37058=VERTEX_POINT('',#143906) ;
#37059=VERTEX_POINT('',#143908) ;
#37060=VERTEX_POINT('',#143912) ;
#37061=VERTEX_POINT('',#143914) ;
#37062=VERTEX_POINT('',#143918) ;
#37063=VERTEX_POINT('',#143920) ;
#37064=VERTEX_POINT('',#143924) ;
#37065=VERTEX_POINT('',#143926) ;
#37066=VERTEX_POINT('',#143930) ;
#37067=VERTEX_POINT('',#143932) ;
#37068=VERTEX_POINT('',#143936) ;
#37069=VERTEX_POINT('',#143938) ;
#37070=VERTEX_POINT('',#143945) ;
#37071=VERTEX_POINT('',#143946) ;
#37072=VERTEX_POINT('',#143948) ;
#37073=VERTEX_POINT('',#143950) ;
#37074=VERTEX_POINT('',#143952) ;
#37075=VERTEX_POINT('',#143954) ;
#37076=VERTEX_POINT('',#143956) ;
#37077=VERTEX_POINT('',#143958) ;
#37078=VERTEX_POINT('',#143960) ;
#37079=VERTEX_POINT('',#143962) ;
#37080=VERTEX_POINT('',#143964) ;
#37081=VERTEX_POINT('',#143966) ;
#37082=VERTEX_POINT('',#143968) ;
#37083=VERTEX_POINT('',#143970) ;
#37084=VERTEX_POINT('',#143972) ;
#37085=VERTEX_POINT('',#143974) ;
#37086=VERTEX_POINT('',#143977) ;
#37087=VERTEX_POINT('',#143981) ;
#37088=VERTEX_POINT('',#143982) ;
#37089=VERTEX_POINT('',#143984) ;
#37090=VERTEX_POINT('',#143986) ;
#37091=VERTEX_POINT('',#143988) ;
#37092=VERTEX_POINT('',#143990) ;
#37093=VERTEX_POINT('',#143992) ;
#37094=VERTEX_POINT('',#143994) ;
#37095=VERTEX_POINT('',#144004) ;
#37096=VERTEX_POINT('',#144014) ;
#37097=VERTEX_POINT('',#144025) ;
#37098=VERTEX_POINT('',#144057) ;
#37099=VERTEX_POINT('',#144104) ;
#37100=VERTEX_POINT('',#144122) ;
#37101=VERTEX_POINT('',#144136) ;
#37102=VERTEX_POINT('',#144151) ;
#37103=VERTEX_POINT('',#144342) ;
#37104=VERTEX_POINT('',#144343) ;
#37105=VERTEX_POINT('',#144345) ;
#37106=VERTEX_POINT('',#144347) ;
#37107=VERTEX_POINT('',#144351) ;
#37108=VERTEX_POINT('',#144352) ;
#37109=VERTEX_POINT('',#144354) ;
#37110=VERTEX_POINT('',#144356) ;
#37111=VERTEX_POINT('',#144360) ;
#37112=VERTEX_POINT('',#144361) ;
#37113=VERTEX_POINT('',#144363) ;
#37114=VERTEX_POINT('',#144365) ;
#37115=VERTEX_POINT('',#144369) ;
#37116=VERTEX_POINT('',#144370) ;
#37117=VERTEX_POINT('',#144372) ;
#37118=VERTEX_POINT('',#144374) ;
#37119=VERTEX_POINT('',#144378) ;
#37120=VERTEX_POINT('',#144379) ;
#37121=VERTEX_POINT('',#144381) ;
#37122=VERTEX_POINT('',#144383) ;
#37123=VERTEX_POINT('',#144387) ;
#37124=VERTEX_POINT('',#144388) ;
#37125=VERTEX_POINT('',#144391) ;
#37126=VERTEX_POINT('',#144393) ;
#37127=VERTEX_POINT('',#144397) ;
#37128=VERTEX_POINT('',#144398) ;
#37129=VERTEX_POINT('',#144401) ;
#37130=VERTEX_POINT('',#144403) ;
#37131=VERTEX_POINT('',#144413) ;
#37132=VERTEX_POINT('',#144414) ;
#37133=VERTEX_POINT('',#144416) ;
#37134=VERTEX_POINT('',#144418) ;
#37135=VERTEX_POINT('',#144422) ;
#37136=VERTEX_POINT('',#144423) ;
#37137=VERTEX_POINT('',#144428) ;
#37138=VERTEX_POINT('',#144430) ;
#37139=VERTEX_POINT('',#144434) ;
#37140=VERTEX_POINT('',#144435) ;
#37141=VERTEX_POINT('',#144437) ;
#37142=VERTEX_POINT('',#144439) ;
#37143=VERTEX_POINT('',#144443) ;
#37144=VERTEX_POINT('',#144444) ;
#37145=VERTEX_POINT('',#144446) ;
#37146=VERTEX_POINT('',#144448) ;
#37147=VERTEX_POINT('',#144452) ;
#37148=VERTEX_POINT('',#144453) ;
#37149=VERTEX_POINT('',#144458) ;
#37150=VERTEX_POINT('',#144460) ;
#37151=VERTEX_POINT('',#144464) ;
#37152=VERTEX_POINT('',#144465) ;
#37153=VERTEX_POINT('',#144467) ;
#37154=VERTEX_POINT('',#144469) ;
#37155=VERTEX_POINT('',#144473) ;
#37156=VERTEX_POINT('',#144474) ;
#37157=VERTEX_POINT('',#144476) ;
#37158=VERTEX_POINT('',#144478) ;
#37159=VERTEX_POINT('',#144482) ;
#37160=VERTEX_POINT('',#144483) ;
#37161=VERTEX_POINT('',#144485) ;
#37162=VERTEX_POINT('',#144487) ;
#37163=VERTEX_POINT('',#144491) ;
#37164=VERTEX_POINT('',#144492) ;
#37165=VERTEX_POINT('',#144494) ;
#37166=VERTEX_POINT('',#144496) ;
#37167=VERTEX_POINT('',#144612) ;
#37168=VERTEX_POINT('',#144613) ;
#37169=VERTEX_POINT('',#144615) ;
#37170=VERTEX_POINT('',#144617) ;
#37171=VERTEX_POINT('',#144619) ;
#37172=VERTEX_POINT('',#144621) ;
#37173=VERTEX_POINT('',#144623) ;
#37174=VERTEX_POINT('',#144625) ;
#37175=VERTEX_POINT('',#144627) ;
#37176=VERTEX_POINT('',#144629) ;
#37177=VERTEX_POINT('',#144633) ;
#37178=VERTEX_POINT('',#144634) ;
#37179=VERTEX_POINT('',#144636) ;
#37180=VERTEX_POINT('',#144638) ;
#37181=VERTEX_POINT('',#144640) ;
#37182=VERTEX_POINT('',#144642) ;
#37183=VERTEX_POINT('',#144644) ;
#37184=VERTEX_POINT('',#144646) ;
#37185=VERTEX_POINT('',#144648) ;
#37186=VERTEX_POINT('',#144650) ;
#37187=VERTEX_POINT('',#144654) ;
#37188=VERTEX_POINT('',#144655) ;
#37189=VERTEX_POINT('',#144657) ;
#37190=VERTEX_POINT('',#144659) ;
#37191=VERTEX_POINT('',#144661) ;
#37192=VERTEX_POINT('',#144663) ;
#37193=VERTEX_POINT('',#144665) ;
#37194=VERTEX_POINT('',#144667) ;
#37195=VERTEX_POINT('',#144669) ;
#37196=VERTEX_POINT('',#144671) ;
#37197=VERTEX_POINT('',#144675) ;
#37198=VERTEX_POINT('',#144676) ;
#37199=VERTEX_POINT('',#144678) ;
#37200=VERTEX_POINT('',#144680) ;
#37201=VERTEX_POINT('',#144682) ;
#37202=VERTEX_POINT('',#144684) ;
#37203=VERTEX_POINT('',#144686) ;
#37204=VERTEX_POINT('',#144688) ;
#37205=VERTEX_POINT('',#144690) ;
#37206=VERTEX_POINT('',#144692) ;
#37207=VERTEX_POINT('',#144696) ;
#37208=VERTEX_POINT('',#144697) ;
#37209=VERTEX_POINT('',#144699) ;
#37210=VERTEX_POINT('',#144701) ;
#37211=VERTEX_POINT('',#144703) ;
#37212=VERTEX_POINT('',#144705) ;
#37213=VERTEX_POINT('',#144707) ;
#37214=VERTEX_POINT('',#144709) ;
#37215=VERTEX_POINT('',#144711) ;
#37216=VERTEX_POINT('',#144713) ;
#37217=VERTEX_POINT('',#144717) ;
#37218=VERTEX_POINT('',#144718) ;
#37219=VERTEX_POINT('',#144720) ;
#37220=VERTEX_POINT('',#144722) ;
#37221=VERTEX_POINT('',#144724) ;
#37222=VERTEX_POINT('',#144726) ;
#37223=VERTEX_POINT('',#144728) ;
#37224=VERTEX_POINT('',#144730) ;
#37225=VERTEX_POINT('',#144732) ;
#37226=VERTEX_POINT('',#144734) ;
#37227=VERTEX_POINT('',#144738) ;
#37228=VERTEX_POINT('',#144739) ;
#37229=VERTEX_POINT('',#144741) ;
#37230=VERTEX_POINT('',#144743) ;
#37231=VERTEX_POINT('',#144745) ;
#37232=VERTEX_POINT('',#144747) ;
#37233=VERTEX_POINT('',#144749) ;
#37234=VERTEX_POINT('',#144751) ;
#37235=VERTEX_POINT('',#144753) ;
#37236=VERTEX_POINT('',#144755) ;
#37237=VERTEX_POINT('',#144759) ;
#37238=VERTEX_POINT('',#144760) ;
#37239=VERTEX_POINT('',#144762) ;
#37240=VERTEX_POINT('',#144764) ;
#37241=VERTEX_POINT('',#144766) ;
#37242=VERTEX_POINT('',#144768) ;
#37243=VERTEX_POINT('',#144770) ;
#37244=VERTEX_POINT('',#144772) ;
#37245=VERTEX_POINT('',#144774) ;
#37246=VERTEX_POINT('',#144776) ;
#37247=VERTEX_POINT('',#144780) ;
#37248=VERTEX_POINT('',#144781) ;
#37249=VERTEX_POINT('',#144783) ;
#37250=VERTEX_POINT('',#144785) ;
#37251=VERTEX_POINT('',#144787) ;
#37252=VERTEX_POINT('',#144789) ;
#37253=VERTEX_POINT('',#144791) ;
#37254=VERTEX_POINT('',#144793) ;
#37255=VERTEX_POINT('',#144795) ;
#37256=VERTEX_POINT('',#144797) ;
#37257=VERTEX_POINT('',#144801) ;
#37258=VERTEX_POINT('',#144802) ;
#37259=VERTEX_POINT('',#144804) ;
#37260=VERTEX_POINT('',#144806) ;
#37261=VERTEX_POINT('',#144810) ;
#37262=VERTEX_POINT('',#144812) ;
#37263=VERTEX_POINT('',#144816) ;
#37264=VERTEX_POINT('',#144817) ;
#37265=VERTEX_POINT('',#144819) ;
#37266=VERTEX_POINT('',#144821) ;
#37267=VERTEX_POINT('',#144825) ;
#37268=VERTEX_POINT('',#144826) ;
#37269=VERTEX_POINT('',#144828) ;
#37270=VERTEX_POINT('',#144830) ;
#37271=VERTEX_POINT('',#144834) ;
#37272=VERTEX_POINT('',#144835) ;
#37273=VERTEX_POINT('',#144837) ;
#37274=VERTEX_POINT('',#144839) ;
#37275=VERTEX_POINT('',#144843) ;
#37276=VERTEX_POINT('',#144844) ;
#37277=VERTEX_POINT('',#144846) ;
#37278=VERTEX_POINT('',#144848) ;
#37279=VERTEX_POINT('',#144852) ;
#37280=VERTEX_POINT('',#144854) ;
#37281=VERTEX_POINT('',#144858) ;
#37282=VERTEX_POINT('',#144859) ;
#37283=VERTEX_POINT('',#144861) ;
#37284=VERTEX_POINT('',#144863) ;
#37285=VERTEX_POINT('',#144867) ;
#37286=VERTEX_POINT('',#144868) ;
#37287=VERTEX_POINT('',#144870) ;
#37288=VERTEX_POINT('',#144872) ;
#37289=VERTEX_POINT('',#144876) ;
#37290=VERTEX_POINT('',#144877) ;
#37291=VERTEX_POINT('',#144879) ;
#37292=VERTEX_POINT('',#144881) ;
#37293=VERTEX_POINT('',#144885) ;
#37294=VERTEX_POINT('',#144886) ;
#37295=VERTEX_POINT('',#144888) ;
#37296=VERTEX_POINT('',#144890) ;
#37297=VERTEX_POINT('',#144894) ;
#37298=VERTEX_POINT('',#144896) ;
#37299=VERTEX_POINT('',#144900) ;
#37300=VERTEX_POINT('',#144901) ;
#37301=VERTEX_POINT('',#144903) ;
#37302=VERTEX_POINT('',#144905) ;
#37303=VERTEX_POINT('',#144909) ;
#37304=VERTEX_POINT('',#144910) ;
#37305=VERTEX_POINT('',#144912) ;
#37306=VERTEX_POINT('',#144914) ;
#37307=VERTEX_POINT('',#144918) ;
#37308=VERTEX_POINT('',#144919) ;
#37309=VERTEX_POINT('',#144921) ;
#37310=VERTEX_POINT('',#144923) ;
#37311=VERTEX_POINT('',#144927) ;
#37312=VERTEX_POINT('',#144928) ;
#37313=VERTEX_POINT('',#144930) ;
#37314=VERTEX_POINT('',#144932) ;
#37315=VERTEX_POINT('',#144936) ;
#37316=VERTEX_POINT('',#144938) ;
#37317=VERTEX_POINT('',#144942) ;
#37318=VERTEX_POINT('',#144943) ;
#37319=VERTEX_POINT('',#144945) ;
#37320=VERTEX_POINT('',#144947) ;
#37321=VERTEX_POINT('',#144951) ;
#37322=VERTEX_POINT('',#144952) ;
#37323=VERTEX_POINT('',#144954) ;
#37324=VERTEX_POINT('',#144956) ;
#37325=VERTEX_POINT('',#144960) ;
#37326=VERTEX_POINT('',#144961) ;
#37327=VERTEX_POINT('',#144963) ;
#37328=VERTEX_POINT('',#144965) ;
#37329=VERTEX_POINT('',#144969) ;
#37330=VERTEX_POINT('',#144970) ;
#37331=VERTEX_POINT('',#144972) ;
#37332=VERTEX_POINT('',#144974) ;
#37333=VERTEX_POINT('',#144978) ;
#37334=VERTEX_POINT('',#144980) ;
#37335=VERTEX_POINT('',#144984) ;
#37336=VERTEX_POINT('',#144985) ;
#37337=VERTEX_POINT('',#144987) ;
#37338=VERTEX_POINT('',#144989) ;
#37339=VERTEX_POINT('',#144993) ;
#37340=VERTEX_POINT('',#144994) ;
#37341=VERTEX_POINT('',#144996) ;
#37342=VERTEX_POINT('',#144998) ;
#37343=VERTEX_POINT('',#145002) ;
#37344=VERTEX_POINT('',#145003) ;
#37345=VERTEX_POINT('',#145005) ;
#37346=VERTEX_POINT('',#145007) ;
#37347=VERTEX_POINT('',#145011) ;
#37348=VERTEX_POINT('',#145012) ;
#37349=VERTEX_POINT('',#145014) ;
#37350=VERTEX_POINT('',#145016) ;
#37351=VERTEX_POINT('',#145020) ;
#37352=VERTEX_POINT('',#145022) ;
#37353=VERTEX_POINT('',#145026) ;
#37354=VERTEX_POINT('',#145027) ;
#37355=VERTEX_POINT('',#145029) ;
#37356=VERTEX_POINT('',#145031) ;
#37357=VERTEX_POINT('',#145035) ;
#37358=VERTEX_POINT('',#145036) ;
#37359=VERTEX_POINT('',#145038) ;
#37360=VERTEX_POINT('',#145040) ;
#37361=VERTEX_POINT('',#145044) ;
#37362=VERTEX_POINT('',#145045) ;
#37363=VERTEX_POINT('',#145047) ;
#37364=VERTEX_POINT('',#145049) ;
#37365=VERTEX_POINT('',#145053) ;
#37366=VERTEX_POINT('',#145054) ;
#37367=VERTEX_POINT('',#145056) ;
#37368=VERTEX_POINT('',#145058) ;
#37369=VERTEX_POINT('',#145062) ;
#37370=VERTEX_POINT('',#145064) ;
#37371=VERTEX_POINT('',#145068) ;
#37372=VERTEX_POINT('',#145069) ;
#37373=VERTEX_POINT('',#145071) ;
#37374=VERTEX_POINT('',#145073) ;
#37375=VERTEX_POINT('',#145077) ;
#37376=VERTEX_POINT('',#145078) ;
#37377=VERTEX_POINT('',#145080) ;
#37378=VERTEX_POINT('',#145082) ;
#37379=VERTEX_POINT('',#145086) ;
#37380=VERTEX_POINT('',#145087) ;
#37381=VERTEX_POINT('',#145089) ;
#37382=VERTEX_POINT('',#145091) ;
#37383=VERTEX_POINT('',#145095) ;
#37384=VERTEX_POINT('',#145096) ;
#37385=VERTEX_POINT('',#145098) ;
#37386=VERTEX_POINT('',#145100) ;
#37387=VERTEX_POINT('',#145104) ;
#37388=VERTEX_POINT('',#145106) ;
#37389=VERTEX_POINT('',#145110) ;
#37390=VERTEX_POINT('',#145111) ;
#37391=VERTEX_POINT('',#145113) ;
#37392=VERTEX_POINT('',#145115) ;
#37393=VERTEX_POINT('',#145119) ;
#37394=VERTEX_POINT('',#145120) ;
#37395=VERTEX_POINT('',#145122) ;
#37396=VERTEX_POINT('',#145124) ;
#37397=VERTEX_POINT('',#145128) ;
#37398=VERTEX_POINT('',#145129) ;
#37399=VERTEX_POINT('',#145131) ;
#37400=VERTEX_POINT('',#145133) ;
#37401=VERTEX_POINT('',#145137) ;
#37402=VERTEX_POINT('',#145138) ;
#37403=VERTEX_POINT('',#145140) ;
#37404=VERTEX_POINT('',#145142) ;
#37405=VERTEX_POINT('',#145146) ;
#37406=VERTEX_POINT('',#145148) ;
#37407=VERTEX_POINT('',#145152) ;
#37408=VERTEX_POINT('',#145153) ;
#37409=VERTEX_POINT('',#145155) ;
#37410=VERTEX_POINT('',#145157) ;
#37411=VERTEX_POINT('',#145161) ;
#37412=VERTEX_POINT('',#145162) ;
#37413=VERTEX_POINT('',#145164) ;
#37414=VERTEX_POINT('',#145166) ;
#37415=VERTEX_POINT('',#145170) ;
#37416=VERTEX_POINT('',#145171) ;
#37417=VERTEX_POINT('',#145173) ;
#37418=VERTEX_POINT('',#145175) ;
#37419=VERTEX_POINT('',#145179) ;
#37420=VERTEX_POINT('',#145180) ;
#37421=VERTEX_POINT('',#145182) ;
#37422=VERTEX_POINT('',#145184) ;
#37423=VERTEX_POINT('',#145188) ;
#37424=VERTEX_POINT('',#145190) ;
#37425=VERTEX_POINT('',#145194) ;
#37426=VERTEX_POINT('',#145196) ;
#37427=VERTEX_POINT('',#145200) ;
#37428=VERTEX_POINT('',#145202) ;
#37429=VERTEX_POINT('',#145206) ;
#37430=VERTEX_POINT('',#145208) ;
#37431=VERTEX_POINT('',#145213) ;
#37432=VERTEX_POINT('',#145217) ;
#37433=VERTEX_POINT('',#145224) ;
#37434=VERTEX_POINT('',#145226) ;
#37435=VERTEX_POINT('',#145230) ;
#37436=VERTEX_POINT('',#145232) ;
#37437=VERTEX_POINT('',#145236) ;
#37438=VERTEX_POINT('',#145238) ;
#37439=VERTEX_POINT('',#145242) ;
#37440=VERTEX_POINT('',#145244) ;
#37441=VERTEX_POINT('',#145248) ;
#37442=VERTEX_POINT('',#145250) ;
#37443=VERTEX_POINT('',#145254) ;
#37444=VERTEX_POINT('',#145256) ;
#37445=VERTEX_POINT('',#145260) ;
#37446=VERTEX_POINT('',#145262) ;
#37447=VERTEX_POINT('',#145266) ;
#37448=VERTEX_POINT('',#145268) ;
#37449=VERTEX_POINT('',#145272) ;
#37450=VERTEX_POINT('',#145274) ;
#37451=VERTEX_POINT('',#145278) ;
#37452=VERTEX_POINT('',#145280) ;
#37453=VERTEX_POINT('',#145284) ;
#37454=VERTEX_POINT('',#145286) ;
#37455=VERTEX_POINT('',#145290) ;
#37456=VERTEX_POINT('',#145292) ;
#37457=VERTEX_POINT('',#145296) ;
#37458=VERTEX_POINT('',#145298) ;
#37459=VERTEX_POINT('',#145302) ;
#37460=VERTEX_POINT('',#145304) ;
#37461=VERTEX_POINT('',#145308) ;
#37462=VERTEX_POINT('',#145310) ;
#37463=VERTEX_POINT('',#145314) ;
#37464=VERTEX_POINT('',#145316) ;
#37465=VERTEX_POINT('',#145320) ;
#37466=VERTEX_POINT('',#145322) ;
#37467=VERTEX_POINT('',#145326) ;
#37468=VERTEX_POINT('',#145328) ;
#37469=VERTEX_POINT('',#145335) ;
#37470=VERTEX_POINT('',#145336) ;
#37471=VERTEX_POINT('',#145338) ;
#37472=VERTEX_POINT('',#145340) ;
#37473=VERTEX_POINT('',#145342) ;
#37474=VERTEX_POINT('',#145344) ;
#37475=VERTEX_POINT('',#145346) ;
#37476=VERTEX_POINT('',#145348) ;
#37477=VERTEX_POINT('',#145350) ;
#37478=VERTEX_POINT('',#145352) ;
#37479=VERTEX_POINT('',#145354) ;
#37480=VERTEX_POINT('',#145356) ;
#37481=VERTEX_POINT('',#145358) ;
#37482=VERTEX_POINT('',#145360) ;
#37483=VERTEX_POINT('',#145362) ;
#37484=VERTEX_POINT('',#145364) ;
#37485=VERTEX_POINT('',#145367) ;
#37486=VERTEX_POINT('',#145371) ;
#37487=VERTEX_POINT('',#145372) ;
#37488=VERTEX_POINT('',#145374) ;
#37489=VERTEX_POINT('',#145376) ;
#37490=VERTEX_POINT('',#145380) ;
#37491=VERTEX_POINT('',#145382) ;
#37492=VERTEX_POINT('',#145386) ;
#37493=VERTEX_POINT('',#145388) ;
#37494=VERTEX_POINT('',#145392) ;
#37495=VERTEX_POINT('',#145394) ;
#37496=VERTEX_POINT('',#145398) ;
#37497=VERTEX_POINT('',#145400) ;
#37498=VERTEX_POINT('',#145405) ;
#37499=VERTEX_POINT('',#145409) ;
#37500=VERTEX_POINT('',#145416) ;
#37501=VERTEX_POINT('',#145418) ;
#37502=VERTEX_POINT('',#145422) ;
#37503=VERTEX_POINT('',#145424) ;
#37504=VERTEX_POINT('',#145428) ;
#37505=VERTEX_POINT('',#145430) ;
#37506=VERTEX_POINT('',#145434) ;
#37507=VERTEX_POINT('',#145436) ;
#37508=VERTEX_POINT('',#145440) ;
#37509=VERTEX_POINT('',#145442) ;
#37510=VERTEX_POINT('',#145446) ;
#37511=VERTEX_POINT('',#145448) ;
#37512=VERTEX_POINT('',#145452) ;
#37513=VERTEX_POINT('',#145454) ;
#37514=VERTEX_POINT('',#145458) ;
#37515=VERTEX_POINT('',#145460) ;
#37516=VERTEX_POINT('',#145464) ;
#37517=VERTEX_POINT('',#145466) ;
#37518=VERTEX_POINT('',#145470) ;
#37519=VERTEX_POINT('',#145472) ;
#37520=VERTEX_POINT('',#145476) ;
#37521=VERTEX_POINT('',#145478) ;
#37522=VERTEX_POINT('',#145482) ;
#37523=VERTEX_POINT('',#145484) ;
#37524=VERTEX_POINT('',#145488) ;
#37525=VERTEX_POINT('',#145490) ;
#37526=VERTEX_POINT('',#145494) ;
#37527=VERTEX_POINT('',#145496) ;
#37528=VERTEX_POINT('',#145500) ;
#37529=VERTEX_POINT('',#145502) ;
#37530=VERTEX_POINT('',#145506) ;
#37531=VERTEX_POINT('',#145508) ;
#37532=VERTEX_POINT('',#145512) ;
#37533=VERTEX_POINT('',#145514) ;
#37534=VERTEX_POINT('',#145518) ;
#37535=VERTEX_POINT('',#145520) ;
#37536=VERTEX_POINT('',#145527) ;
#37537=VERTEX_POINT('',#145528) ;
#37538=VERTEX_POINT('',#145530) ;
#37539=VERTEX_POINT('',#145532) ;
#37540=VERTEX_POINT('',#145534) ;
#37541=VERTEX_POINT('',#145536) ;
#37542=VERTEX_POINT('',#145538) ;
#37543=VERTEX_POINT('',#145540) ;
#37544=VERTEX_POINT('',#145542) ;
#37545=VERTEX_POINT('',#145544) ;
#37546=VERTEX_POINT('',#145546) ;
#37547=VERTEX_POINT('',#145548) ;
#37548=VERTEX_POINT('',#145550) ;
#37549=VERTEX_POINT('',#145552) ;
#37550=VERTEX_POINT('',#145554) ;
#37551=VERTEX_POINT('',#145556) ;
#37552=VERTEX_POINT('',#145559) ;
#37553=VERTEX_POINT('',#145563) ;
#37554=VERTEX_POINT('',#145564) ;
#37555=VERTEX_POINT('',#145566) ;
#37556=VERTEX_POINT('',#145568) ;
#37557=VERTEX_POINT('',#145572) ;
#37558=VERTEX_POINT('',#145574) ;
#37559=VERTEX_POINT('',#145578) ;
#37560=VERTEX_POINT('',#145580) ;
#37561=VERTEX_POINT('',#145584) ;
#37562=VERTEX_POINT('',#145586) ;
#37563=VERTEX_POINT('',#145590) ;
#37564=VERTEX_POINT('',#145592) ;
#37565=VERTEX_POINT('',#145597) ;
#37566=VERTEX_POINT('',#145601) ;
#37567=VERTEX_POINT('',#145608) ;
#37568=VERTEX_POINT('',#145610) ;
#37569=VERTEX_POINT('',#145614) ;
#37570=VERTEX_POINT('',#145616) ;
#37571=VERTEX_POINT('',#145620) ;
#37572=VERTEX_POINT('',#145622) ;
#37573=VERTEX_POINT('',#145626) ;
#37574=VERTEX_POINT('',#145628) ;
#37575=VERTEX_POINT('',#145632) ;
#37576=VERTEX_POINT('',#145634) ;
#37577=VERTEX_POINT('',#145638) ;
#37578=VERTEX_POINT('',#145640) ;
#37579=VERTEX_POINT('',#145644) ;
#37580=VERTEX_POINT('',#145646) ;
#37581=VERTEX_POINT('',#145650) ;
#37582=VERTEX_POINT('',#145652) ;
#37583=VERTEX_POINT('',#145656) ;
#37584=VERTEX_POINT('',#145658) ;
#37585=VERTEX_POINT('',#145662) ;
#37586=VERTEX_POINT('',#145664) ;
#37587=VERTEX_POINT('',#145668) ;
#37588=VERTEX_POINT('',#145670) ;
#37589=VERTEX_POINT('',#145674) ;
#37590=VERTEX_POINT('',#145676) ;
#37591=VERTEX_POINT('',#145680) ;
#37592=VERTEX_POINT('',#145682) ;
#37593=VERTEX_POINT('',#145686) ;
#37594=VERTEX_POINT('',#145688) ;
#37595=VERTEX_POINT('',#145692) ;
#37596=VERTEX_POINT('',#145694) ;
#37597=VERTEX_POINT('',#145698) ;
#37598=VERTEX_POINT('',#145700) ;
#37599=VERTEX_POINT('',#145704) ;
#37600=VERTEX_POINT('',#145706) ;
#37601=VERTEX_POINT('',#145710) ;
#37602=VERTEX_POINT('',#145712) ;
#37603=VERTEX_POINT('',#145719) ;
#37604=VERTEX_POINT('',#145720) ;
#37605=VERTEX_POINT('',#145722) ;
#37606=VERTEX_POINT('',#145724) ;
#37607=VERTEX_POINT('',#145726) ;
#37608=VERTEX_POINT('',#145728) ;
#37609=VERTEX_POINT('',#145730) ;
#37610=VERTEX_POINT('',#145732) ;
#37611=VERTEX_POINT('',#145734) ;
#37612=VERTEX_POINT('',#145736) ;
#37613=VERTEX_POINT('',#145738) ;
#37614=VERTEX_POINT('',#145740) ;
#37615=VERTEX_POINT('',#145742) ;
#37616=VERTEX_POINT('',#145744) ;
#37617=VERTEX_POINT('',#145746) ;
#37618=VERTEX_POINT('',#145748) ;
#37619=VERTEX_POINT('',#145751) ;
#37620=VERTEX_POINT('',#145755) ;
#37621=VERTEX_POINT('',#145756) ;
#37622=VERTEX_POINT('',#145758) ;
#37623=VERTEX_POINT('',#145760) ;
#37624=VERTEX_POINT('',#145764) ;
#37625=VERTEX_POINT('',#145766) ;
#37626=VERTEX_POINT('',#145770) ;
#37627=VERTEX_POINT('',#145772) ;
#37628=VERTEX_POINT('',#145776) ;
#37629=VERTEX_POINT('',#145778) ;
#37630=VERTEX_POINT('',#145782) ;
#37631=VERTEX_POINT('',#145784) ;
#37632=VERTEX_POINT('',#145789) ;
#37633=VERTEX_POINT('',#145793) ;
#37634=VERTEX_POINT('',#145800) ;
#37635=VERTEX_POINT('',#145802) ;
#37636=VERTEX_POINT('',#145806) ;
#37637=VERTEX_POINT('',#145808) ;
#37638=VERTEX_POINT('',#145812) ;
#37639=VERTEX_POINT('',#145814) ;
#37640=VERTEX_POINT('',#145818) ;
#37641=VERTEX_POINT('',#145820) ;
#37642=VERTEX_POINT('',#145824) ;
#37643=VERTEX_POINT('',#145826) ;
#37644=VERTEX_POINT('',#145830) ;
#37645=VERTEX_POINT('',#145832) ;
#37646=VERTEX_POINT('',#145836) ;
#37647=VERTEX_POINT('',#145838) ;
#37648=VERTEX_POINT('',#145842) ;
#37649=VERTEX_POINT('',#145844) ;
#37650=VERTEX_POINT('',#145848) ;
#37651=VERTEX_POINT('',#145850) ;
#37652=VERTEX_POINT('',#145854) ;
#37653=VERTEX_POINT('',#145856) ;
#37654=VERTEX_POINT('',#145860) ;
#37655=VERTEX_POINT('',#145862) ;
#37656=VERTEX_POINT('',#145866) ;
#37657=VERTEX_POINT('',#145868) ;
#37658=VERTEX_POINT('',#145872) ;
#37659=VERTEX_POINT('',#145874) ;
#37660=VERTEX_POINT('',#145878) ;
#37661=VERTEX_POINT('',#145880) ;
#37662=VERTEX_POINT('',#145884) ;
#37663=VERTEX_POINT('',#145886) ;
#37664=VERTEX_POINT('',#145890) ;
#37665=VERTEX_POINT('',#145892) ;
#37666=VERTEX_POINT('',#145896) ;
#37667=VERTEX_POINT('',#145898) ;
#37668=VERTEX_POINT('',#145902) ;
#37669=VERTEX_POINT('',#145904) ;
#37670=VERTEX_POINT('',#145911) ;
#37671=VERTEX_POINT('',#145912) ;
#37672=VERTEX_POINT('',#145914) ;
#37673=VERTEX_POINT('',#145916) ;
#37674=VERTEX_POINT('',#145918) ;
#37675=VERTEX_POINT('',#145920) ;
#37676=VERTEX_POINT('',#145922) ;
#37677=VERTEX_POINT('',#145924) ;
#37678=VERTEX_POINT('',#145926) ;
#37679=VERTEX_POINT('',#145928) ;
#37680=VERTEX_POINT('',#145930) ;
#37681=VERTEX_POINT('',#145932) ;
#37682=VERTEX_POINT('',#145934) ;
#37683=VERTEX_POINT('',#145936) ;
#37684=VERTEX_POINT('',#145938) ;
#37685=VERTEX_POINT('',#145940) ;
#37686=VERTEX_POINT('',#145943) ;
#37687=VERTEX_POINT('',#145947) ;
#37688=VERTEX_POINT('',#145948) ;
#37689=VERTEX_POINT('',#145950) ;
#37690=VERTEX_POINT('',#145952) ;
#37691=VERTEX_POINT('',#145956) ;
#37692=VERTEX_POINT('',#145958) ;
#37693=VERTEX_POINT('',#145962) ;
#37694=VERTEX_POINT('',#145964) ;
#37695=VERTEX_POINT('',#145968) ;
#37696=VERTEX_POINT('',#145970) ;
#37697=VERTEX_POINT('',#145974) ;
#37698=VERTEX_POINT('',#145976) ;
#37699=VERTEX_POINT('',#145981) ;
#37700=VERTEX_POINT('',#145985) ;
#37701=VERTEX_POINT('',#145992) ;
#37702=VERTEX_POINT('',#145994) ;
#37703=VERTEX_POINT('',#145998) ;
#37704=VERTEX_POINT('',#146000) ;
#37705=VERTEX_POINT('',#146004) ;
#37706=VERTEX_POINT('',#146006) ;
#37707=VERTEX_POINT('',#146010) ;
#37708=VERTEX_POINT('',#146012) ;
#37709=VERTEX_POINT('',#146016) ;
#37710=VERTEX_POINT('',#146018) ;
#37711=VERTEX_POINT('',#146022) ;
#37712=VERTEX_POINT('',#146024) ;
#37713=VERTEX_POINT('',#146028) ;
#37714=VERTEX_POINT('',#146030) ;
#37715=VERTEX_POINT('',#146034) ;
#37716=VERTEX_POINT('',#146036) ;
#37717=VERTEX_POINT('',#146040) ;
#37718=VERTEX_POINT('',#146042) ;
#37719=VERTEX_POINT('',#146046) ;
#37720=VERTEX_POINT('',#146048) ;
#37721=VERTEX_POINT('',#146052) ;
#37722=VERTEX_POINT('',#146054) ;
#37723=VERTEX_POINT('',#146058) ;
#37724=VERTEX_POINT('',#146060) ;
#37725=VERTEX_POINT('',#146064) ;
#37726=VERTEX_POINT('',#146066) ;
#37727=VERTEX_POINT('',#146070) ;
#37728=VERTEX_POINT('',#146072) ;
#37729=VERTEX_POINT('',#146076) ;
#37730=VERTEX_POINT('',#146078) ;
#37731=VERTEX_POINT('',#146082) ;
#37732=VERTEX_POINT('',#146084) ;
#37733=VERTEX_POINT('',#146088) ;
#37734=VERTEX_POINT('',#146090) ;
#37735=VERTEX_POINT('',#146094) ;
#37736=VERTEX_POINT('',#146096) ;
#37737=VERTEX_POINT('',#146103) ;
#37738=VERTEX_POINT('',#146104) ;
#37739=VERTEX_POINT('',#146106) ;
#37740=VERTEX_POINT('',#146108) ;
#37741=VERTEX_POINT('',#146110) ;
#37742=VERTEX_POINT('',#146112) ;
#37743=VERTEX_POINT('',#146114) ;
#37744=VERTEX_POINT('',#146116) ;
#37745=VERTEX_POINT('',#146118) ;
#37746=VERTEX_POINT('',#146120) ;
#37747=VERTEX_POINT('',#146122) ;
#37748=VERTEX_POINT('',#146124) ;
#37749=VERTEX_POINT('',#146126) ;
#37750=VERTEX_POINT('',#146128) ;
#37751=VERTEX_POINT('',#146130) ;
#37752=VERTEX_POINT('',#146132) ;
#37753=VERTEX_POINT('',#146135) ;
#37754=VERTEX_POINT('',#146139) ;
#37755=VERTEX_POINT('',#146140) ;
#37756=VERTEX_POINT('',#146142) ;
#37757=VERTEX_POINT('',#146144) ;
#37758=VERTEX_POINT('',#146148) ;
#37759=VERTEX_POINT('',#146150) ;
#37760=VERTEX_POINT('',#146154) ;
#37761=VERTEX_POINT('',#146156) ;
#37762=VERTEX_POINT('',#146160) ;
#37763=VERTEX_POINT('',#146162) ;
#37764=VERTEX_POINT('',#146166) ;
#37765=VERTEX_POINT('',#146168) ;
#37766=VERTEX_POINT('',#146173) ;
#37767=VERTEX_POINT('',#146177) ;
#37768=VERTEX_POINT('',#146184) ;
#37769=VERTEX_POINT('',#146186) ;
#37770=VERTEX_POINT('',#146190) ;
#37771=VERTEX_POINT('',#146192) ;
#37772=VERTEX_POINT('',#146196) ;
#37773=VERTEX_POINT('',#146198) ;
#37774=VERTEX_POINT('',#146202) ;
#37775=VERTEX_POINT('',#146204) ;
#37776=VERTEX_POINT('',#146208) ;
#37777=VERTEX_POINT('',#146210) ;
#37778=VERTEX_POINT('',#146214) ;
#37779=VERTEX_POINT('',#146216) ;
#37780=VERTEX_POINT('',#146220) ;
#37781=VERTEX_POINT('',#146222) ;
#37782=VERTEX_POINT('',#146226) ;
#37783=VERTEX_POINT('',#146228) ;
#37784=VERTEX_POINT('',#146232) ;
#37785=VERTEX_POINT('',#146234) ;
#37786=VERTEX_POINT('',#146238) ;
#37787=VERTEX_POINT('',#146240) ;
#37788=VERTEX_POINT('',#146244) ;
#37789=VERTEX_POINT('',#146246) ;
#37790=VERTEX_POINT('',#146250) ;
#37791=VERTEX_POINT('',#146252) ;
#37792=VERTEX_POINT('',#146256) ;
#37793=VERTEX_POINT('',#146258) ;
#37794=VERTEX_POINT('',#146262) ;
#37795=VERTEX_POINT('',#146264) ;
#37796=VERTEX_POINT('',#146268) ;
#37797=VERTEX_POINT('',#146270) ;
#37798=VERTEX_POINT('',#146274) ;
#37799=VERTEX_POINT('',#146276) ;
#37800=VERTEX_POINT('',#146280) ;
#37801=VERTEX_POINT('',#146282) ;
#37802=VERTEX_POINT('',#146286) ;
#37803=VERTEX_POINT('',#146288) ;
#37804=VERTEX_POINT('',#146295) ;
#37805=VERTEX_POINT('',#146296) ;
#37806=VERTEX_POINT('',#146298) ;
#37807=VERTEX_POINT('',#146300) ;
#37808=VERTEX_POINT('',#146302) ;
#37809=VERTEX_POINT('',#146304) ;
#37810=VERTEX_POINT('',#146306) ;
#37811=VERTEX_POINT('',#146308) ;
#37812=VERTEX_POINT('',#146310) ;
#37813=VERTEX_POINT('',#146312) ;
#37814=VERTEX_POINT('',#146314) ;
#37815=VERTEX_POINT('',#146316) ;
#37816=VERTEX_POINT('',#146318) ;
#37817=VERTEX_POINT('',#146320) ;
#37818=VERTEX_POINT('',#146322) ;
#37819=VERTEX_POINT('',#146324) ;
#37820=VERTEX_POINT('',#146327) ;
#37821=VERTEX_POINT('',#146331) ;
#37822=VERTEX_POINT('',#146332) ;
#37823=VERTEX_POINT('',#146334) ;
#37824=VERTEX_POINT('',#146336) ;
#37825=VERTEX_POINT('',#146340) ;
#37826=VERTEX_POINT('',#146342) ;
#37827=VERTEX_POINT('',#146346) ;
#37828=VERTEX_POINT('',#146348) ;
#37829=VERTEX_POINT('',#146352) ;
#37830=VERTEX_POINT('',#146354) ;
#37831=VERTEX_POINT('',#146358) ;
#37832=VERTEX_POINT('',#146360) ;
#37833=VERTEX_POINT('',#146365) ;
#37834=VERTEX_POINT('',#146369) ;
#37835=VERTEX_POINT('',#146376) ;
#37836=VERTEX_POINT('',#146378) ;
#37837=VERTEX_POINT('',#146382) ;
#37838=VERTEX_POINT('',#146384) ;
#37839=VERTEX_POINT('',#146388) ;
#37840=VERTEX_POINT('',#146390) ;
#37841=VERTEX_POINT('',#146394) ;
#37842=VERTEX_POINT('',#146396) ;
#37843=VERTEX_POINT('',#146400) ;
#37844=VERTEX_POINT('',#146402) ;
#37845=VERTEX_POINT('',#146406) ;
#37846=VERTEX_POINT('',#146408) ;
#37847=VERTEX_POINT('',#146412) ;
#37848=VERTEX_POINT('',#146414) ;
#37849=VERTEX_POINT('',#146418) ;
#37850=VERTEX_POINT('',#146420) ;
#37851=VERTEX_POINT('',#146424) ;
#37852=VERTEX_POINT('',#146426) ;
#37853=VERTEX_POINT('',#146430) ;
#37854=VERTEX_POINT('',#146432) ;
#37855=VERTEX_POINT('',#146436) ;
#37856=VERTEX_POINT('',#146438) ;
#37857=VERTEX_POINT('',#146442) ;
#37858=VERTEX_POINT('',#146444) ;
#37859=VERTEX_POINT('',#146448) ;
#37860=VERTEX_POINT('',#146450) ;
#37861=VERTEX_POINT('',#146454) ;
#37862=VERTEX_POINT('',#146456) ;
#37863=VERTEX_POINT('',#146460) ;
#37864=VERTEX_POINT('',#146462) ;
#37865=VERTEX_POINT('',#146466) ;
#37866=VERTEX_POINT('',#146468) ;
#37867=VERTEX_POINT('',#146472) ;
#37868=VERTEX_POINT('',#146474) ;
#37869=VERTEX_POINT('',#146478) ;
#37870=VERTEX_POINT('',#146480) ;
#37871=VERTEX_POINT('',#146487) ;
#37872=VERTEX_POINT('',#146488) ;
#37873=VERTEX_POINT('',#146490) ;
#37874=VERTEX_POINT('',#146492) ;
#37875=VERTEX_POINT('',#146494) ;
#37876=VERTEX_POINT('',#146496) ;
#37877=VERTEX_POINT('',#146498) ;
#37878=VERTEX_POINT('',#146500) ;
#37879=VERTEX_POINT('',#146502) ;
#37880=VERTEX_POINT('',#146504) ;
#37881=VERTEX_POINT('',#146506) ;
#37882=VERTEX_POINT('',#146508) ;
#37883=VERTEX_POINT('',#146510) ;
#37884=VERTEX_POINT('',#146512) ;
#37885=VERTEX_POINT('',#146514) ;
#37886=VERTEX_POINT('',#146516) ;
#37887=VERTEX_POINT('',#146519) ;
#37888=VERTEX_POINT('',#146523) ;
#37889=VERTEX_POINT('',#146524) ;
#37890=VERTEX_POINT('',#146526) ;
#37891=VERTEX_POINT('',#146528) ;
#37892=VERTEX_POINT('',#146532) ;
#37893=VERTEX_POINT('',#146534) ;
#37894=VERTEX_POINT('',#146538) ;
#37895=VERTEX_POINT('',#146540) ;
#37896=VERTEX_POINT('',#146544) ;
#37897=VERTEX_POINT('',#146546) ;
#37898=VERTEX_POINT('',#146550) ;
#37899=VERTEX_POINT('',#146552) ;
#37900=VERTEX_POINT('',#146557) ;
#37901=VERTEX_POINT('',#146561) ;
#37902=VERTEX_POINT('',#146568) ;
#37903=VERTEX_POINT('',#146570) ;
#37904=VERTEX_POINT('',#146574) ;
#37905=VERTEX_POINT('',#146576) ;
#37906=VERTEX_POINT('',#146580) ;
#37907=VERTEX_POINT('',#146582) ;
#37908=VERTEX_POINT('',#146586) ;
#37909=VERTEX_POINT('',#146588) ;
#37910=VERTEX_POINT('',#146592) ;
#37911=VERTEX_POINT('',#146594) ;
#37912=VERTEX_POINT('',#146598) ;
#37913=VERTEX_POINT('',#146600) ;
#37914=VERTEX_POINT('',#146604) ;
#37915=VERTEX_POINT('',#146606) ;
#37916=VERTEX_POINT('',#146610) ;
#37917=VERTEX_POINT('',#146612) ;
#37918=VERTEX_POINT('',#146616) ;
#37919=VERTEX_POINT('',#146618) ;
#37920=VERTEX_POINT('',#146622) ;
#37921=VERTEX_POINT('',#146624) ;
#37922=VERTEX_POINT('',#146628) ;
#37923=VERTEX_POINT('',#146630) ;
#37924=VERTEX_POINT('',#146634) ;
#37925=VERTEX_POINT('',#146636) ;
#37926=VERTEX_POINT('',#146640) ;
#37927=VERTEX_POINT('',#146642) ;
#37928=VERTEX_POINT('',#146646) ;
#37929=VERTEX_POINT('',#146648) ;
#37930=VERTEX_POINT('',#146652) ;
#37931=VERTEX_POINT('',#146654) ;
#37932=VERTEX_POINT('',#146658) ;
#37933=VERTEX_POINT('',#146660) ;
#37934=VERTEX_POINT('',#146664) ;
#37935=VERTEX_POINT('',#146666) ;
#37936=VERTEX_POINT('',#146670) ;
#37937=VERTEX_POINT('',#146672) ;
#37938=VERTEX_POINT('',#146679) ;
#37939=VERTEX_POINT('',#146680) ;
#37940=VERTEX_POINT('',#146682) ;
#37941=VERTEX_POINT('',#146684) ;
#37942=VERTEX_POINT('',#146686) ;
#37943=VERTEX_POINT('',#146688) ;
#37944=VERTEX_POINT('',#146690) ;
#37945=VERTEX_POINT('',#146692) ;
#37946=VERTEX_POINT('',#146694) ;
#37947=VERTEX_POINT('',#146696) ;
#37948=VERTEX_POINT('',#146698) ;
#37949=VERTEX_POINT('',#146700) ;
#37950=VERTEX_POINT('',#146702) ;
#37951=VERTEX_POINT('',#146704) ;
#37952=VERTEX_POINT('',#146706) ;
#37953=VERTEX_POINT('',#146708) ;
#37954=VERTEX_POINT('',#146711) ;
#37955=VERTEX_POINT('',#146715) ;
#37956=VERTEX_POINT('',#146716) ;
#37957=VERTEX_POINT('',#146718) ;
#37958=VERTEX_POINT('',#146720) ;
#37959=VERTEX_POINT('',#146724) ;
#37960=VERTEX_POINT('',#146726) ;
#37961=VERTEX_POINT('',#146730) ;
#37962=VERTEX_POINT('',#146732) ;
#37963=VERTEX_POINT('',#146736) ;
#37964=VERTEX_POINT('',#146738) ;
#37965=VERTEX_POINT('',#146742) ;
#37966=VERTEX_POINT('',#146744) ;
#37967=VERTEX_POINT('',#146749) ;
#37968=VERTEX_POINT('',#146753) ;
#37969=VERTEX_POINT('',#146760) ;
#37970=VERTEX_POINT('',#146762) ;
#37971=VERTEX_POINT('',#146766) ;
#37972=VERTEX_POINT('',#146768) ;
#37973=VERTEX_POINT('',#146772) ;
#37974=VERTEX_POINT('',#146774) ;
#37975=VERTEX_POINT('',#146778) ;
#37976=VERTEX_POINT('',#146780) ;
#37977=VERTEX_POINT('',#146784) ;
#37978=VERTEX_POINT('',#146786) ;
#37979=VERTEX_POINT('',#146790) ;
#37980=VERTEX_POINT('',#146792) ;
#37981=VERTEX_POINT('',#146796) ;
#37982=VERTEX_POINT('',#146798) ;
#37983=VERTEX_POINT('',#146802) ;
#37984=VERTEX_POINT('',#146804) ;
#37985=VERTEX_POINT('',#146808) ;
#37986=VERTEX_POINT('',#146810) ;
#37987=VERTEX_POINT('',#146814) ;
#37988=VERTEX_POINT('',#146816) ;
#37989=VERTEX_POINT('',#146820) ;
#37990=VERTEX_POINT('',#146822) ;
#37991=VERTEX_POINT('',#146826) ;
#37992=VERTEX_POINT('',#146828) ;
#37993=VERTEX_POINT('',#146832) ;
#37994=VERTEX_POINT('',#146834) ;
#37995=VERTEX_POINT('',#146838) ;
#37996=VERTEX_POINT('',#146840) ;
#37997=VERTEX_POINT('',#146844) ;
#37998=VERTEX_POINT('',#146846) ;
#37999=VERTEX_POINT('',#146850) ;
#38000=VERTEX_POINT('',#146852) ;
#38001=VERTEX_POINT('',#146856) ;
#38002=VERTEX_POINT('',#146858) ;
#38003=VERTEX_POINT('',#146862) ;
#38004=VERTEX_POINT('',#146864) ;
#38005=VERTEX_POINT('',#146871) ;
#38006=VERTEX_POINT('',#146872) ;
#38007=VERTEX_POINT('',#146874) ;
#38008=VERTEX_POINT('',#146876) ;
#38009=VERTEX_POINT('',#146878) ;
#38010=VERTEX_POINT('',#146880) ;
#38011=VERTEX_POINT('',#146882) ;
#38012=VERTEX_POINT('',#146884) ;
#38013=VERTEX_POINT('',#146886) ;
#38014=VERTEX_POINT('',#146888) ;
#38015=VERTEX_POINT('',#146890) ;
#38016=VERTEX_POINT('',#146892) ;
#38017=VERTEX_POINT('',#146894) ;
#38018=VERTEX_POINT('',#146896) ;
#38019=VERTEX_POINT('',#146898) ;
#38020=VERTEX_POINT('',#146900) ;
#38021=VERTEX_POINT('',#146903) ;
#38022=VERTEX_POINT('',#146907) ;
#38023=VERTEX_POINT('',#146908) ;
#38024=VERTEX_POINT('',#146910) ;
#38025=VERTEX_POINT('',#146912) ;
#38026=VERTEX_POINT('',#146914) ;
#38027=VERTEX_POINT('',#146916) ;
#38028=VERTEX_POINT('',#146918) ;
#38029=VERTEX_POINT('',#146920) ;
#38030=VERTEX_POINT('',#146924) ;
#38031=VERTEX_POINT('',#146925) ;
#38032=VERTEX_POINT('',#146927) ;
#38033=VERTEX_POINT('',#146929) ;
#38034=VERTEX_POINT('',#146931) ;
#38035=VERTEX_POINT('',#146933) ;
#38036=VERTEX_POINT('',#146935) ;
#38037=VERTEX_POINT('',#146937) ;
#38038=VERTEX_POINT('',#146941) ;
#38039=VERTEX_POINT('',#146942) ;
#38040=VERTEX_POINT('',#146944) ;
#38041=VERTEX_POINT('',#146946) ;
#38042=VERTEX_POINT('',#146948) ;
#38043=VERTEX_POINT('',#146950) ;
#38044=VERTEX_POINT('',#146952) ;
#38045=VERTEX_POINT('',#146954) ;
#38046=VERTEX_POINT('',#146958) ;
#38047=VERTEX_POINT('',#146959) ;
#38048=VERTEX_POINT('',#146961) ;
#38049=VERTEX_POINT('',#146963) ;
#38050=VERTEX_POINT('',#146965) ;
#38051=VERTEX_POINT('',#146967) ;
#38052=VERTEX_POINT('',#146969) ;
#38053=VERTEX_POINT('',#146971) ;
#38054=VERTEX_POINT('',#146975) ;
#38055=VERTEX_POINT('',#146976) ;
#38056=VERTEX_POINT('',#146978) ;
#38057=VERTEX_POINT('',#146980) ;
#38058=VERTEX_POINT('',#146982) ;
#38059=VERTEX_POINT('',#146984) ;
#38060=VERTEX_POINT('',#146986) ;
#38061=VERTEX_POINT('',#146988) ;
#38062=VERTEX_POINT('',#146992) ;
#38063=VERTEX_POINT('',#146993) ;
#38064=VERTEX_POINT('',#146995) ;
#38065=VERTEX_POINT('',#146997) ;
#38066=VERTEX_POINT('',#146999) ;
#38067=VERTEX_POINT('',#147001) ;
#38068=VERTEX_POINT('',#147003) ;
#38069=VERTEX_POINT('',#147005) ;
#38070=VERTEX_POINT('',#147009) ;
#38071=VERTEX_POINT('',#147010) ;
#38072=VERTEX_POINT('',#147012) ;
#38073=VERTEX_POINT('',#147014) ;
#38074=VERTEX_POINT('',#147016) ;
#38075=VERTEX_POINT('',#147018) ;
#38076=VERTEX_POINT('',#147020) ;
#38077=VERTEX_POINT('',#147022) ;
#38078=VERTEX_POINT('',#147026) ;
#38079=VERTEX_POINT('',#147027) ;
#38080=VERTEX_POINT('',#147029) ;
#38081=VERTEX_POINT('',#147031) ;
#38082=VERTEX_POINT('',#147033) ;
#38083=VERTEX_POINT('',#147035) ;
#38084=VERTEX_POINT('',#147037) ;
#38085=VERTEX_POINT('',#147039) ;
#38086=VERTEX_POINT('',#147043) ;
#38087=VERTEX_POINT('',#147044) ;
#38088=VERTEX_POINT('',#147046) ;
#38089=VERTEX_POINT('',#147048) ;
#38090=VERTEX_POINT('',#147050) ;
#38091=VERTEX_POINT('',#147052) ;
#38092=VERTEX_POINT('',#147054) ;
#38093=VERTEX_POINT('',#147056) ;
#38094=VERTEX_POINT('',#147066) ;
#38095=VERTEX_POINT('',#147076) ;
#38096=VERTEX_POINT('',#147087) ;
#38097=VERTEX_POINT('',#147119) ;
#38098=VERTEX_POINT('',#147166) ;
#38099=VERTEX_POINT('',#147184) ;
#38100=VERTEX_POINT('',#147198) ;
#38101=VERTEX_POINT('',#147213) ;
#38102=VERTEX_POINT('',#147770) ;
#38103=VERTEX_POINT('',#147780) ;
#38104=VERTEX_POINT('',#147791) ;
#38105=VERTEX_POINT('',#147823) ;
#38106=VERTEX_POINT('',#147870) ;
#38107=VERTEX_POINT('',#147888) ;
#38108=VERTEX_POINT('',#147902) ;
#38109=VERTEX_POINT('',#147917) ;
#38110=VERTEX_POINT('',#147997) ;
#38111=VERTEX_POINT('',#148007) ;
#38112=VERTEX_POINT('',#148018) ;
#38113=VERTEX_POINT('',#148050) ;
#38114=VERTEX_POINT('',#148097) ;
#38115=VERTEX_POINT('',#148115) ;
#38116=VERTEX_POINT('',#148129) ;
#38117=VERTEX_POINT('',#148144) ;
#38118=VERTEX_POINT('',#148224) ;
#38119=VERTEX_POINT('',#148234) ;
#38120=VERTEX_POINT('',#148245) ;
#38121=VERTEX_POINT('',#148277) ;
#38122=VERTEX_POINT('',#148324) ;
#38123=VERTEX_POINT('',#148342) ;
#38124=VERTEX_POINT('',#148356) ;
#38125=VERTEX_POINT('',#148371) ;
#38126=VERTEX_POINT('',#148451) ;
#38127=VERTEX_POINT('',#148461) ;
#38128=VERTEX_POINT('',#148472) ;
#38129=VERTEX_POINT('',#148504) ;
#38130=VERTEX_POINT('',#148551) ;
#38131=VERTEX_POINT('',#148569) ;
#38132=VERTEX_POINT('',#148583) ;
#38133=VERTEX_POINT('',#148598) ;
#38134=VERTEX_POINT('',#148678) ;
#38135=VERTEX_POINT('',#148688) ;
#38136=VERTEX_POINT('',#148699) ;
#38137=VERTEX_POINT('',#148731) ;
#38138=VERTEX_POINT('',#148778) ;
#38139=VERTEX_POINT('',#148796) ;
#38140=VERTEX_POINT('',#148810) ;
#38141=VERTEX_POINT('',#148825) ;
#38142=VERTEX_POINT('',#148905) ;
#38143=VERTEX_POINT('',#148915) ;
#38144=VERTEX_POINT('',#148926) ;
#38145=VERTEX_POINT('',#148958) ;
#38146=VERTEX_POINT('',#149005) ;
#38147=VERTEX_POINT('',#149023) ;
#38148=VERTEX_POINT('',#149037) ;
#38149=VERTEX_POINT('',#149052) ;
#38150=VERTEX_POINT('',#149132) ;
#38151=VERTEX_POINT('',#149142) ;
#38152=VERTEX_POINT('',#149153) ;
#38153=VERTEX_POINT('',#149185) ;
#38154=VERTEX_POINT('',#149232) ;
#38155=VERTEX_POINT('',#149250) ;
#38156=VERTEX_POINT('',#149264) ;
#38157=VERTEX_POINT('',#149279) ;
#38158=VERTEX_POINT('',#149359) ;
#38159=VERTEX_POINT('',#149369) ;
#38160=VERTEX_POINT('',#149380) ;
#38161=VERTEX_POINT('',#149412) ;
#38162=VERTEX_POINT('',#149459) ;
#38163=VERTEX_POINT('',#149477) ;
#38164=VERTEX_POINT('',#149491) ;
#38165=VERTEX_POINT('',#149506) ;
#38166=VERTEX_POINT('',#149580) ;
#38167=VERTEX_POINT('',#149581) ;
#38168=VERTEX_POINT('',#149583) ;
#38169=VERTEX_POINT('',#149585) ;
#38170=VERTEX_POINT('',#149589) ;
#38171=VERTEX_POINT('',#149590) ;
#38172=VERTEX_POINT('',#149592) ;
#38173=VERTEX_POINT('',#149594) ;
#38174=VERTEX_POINT('',#149598) ;
#38175=VERTEX_POINT('',#149599) ;
#38176=VERTEX_POINT('',#149601) ;
#38177=VERTEX_POINT('',#149603) ;
#38178=VERTEX_POINT('',#149607) ;
#38179=VERTEX_POINT('',#149608) ;
#38180=VERTEX_POINT('',#149610) ;
#38181=VERTEX_POINT('',#149612) ;
#38182=VERTEX_POINT('',#149616) ;
#38183=VERTEX_POINT('',#149617) ;
#38184=VERTEX_POINT('',#149619) ;
#38185=VERTEX_POINT('',#149621) ;
#38186=VERTEX_POINT('',#149625) ;
#38187=VERTEX_POINT('',#149626) ;
#38188=VERTEX_POINT('',#149629) ;
#38189=VERTEX_POINT('',#149631) ;
#38190=VERTEX_POINT('',#149635) ;
#38191=VERTEX_POINT('',#149636) ;
#38192=VERTEX_POINT('',#149639) ;
#38193=VERTEX_POINT('',#149641) ;
#38194=VERTEX_POINT('',#149651) ;
#38195=VERTEX_POINT('',#149652) ;
#38196=VERTEX_POINT('',#149654) ;
#38197=VERTEX_POINT('',#149656) ;
#38198=VERTEX_POINT('',#149660) ;
#38199=VERTEX_POINT('',#149661) ;
#38200=VERTEX_POINT('',#149666) ;
#38201=VERTEX_POINT('',#149668) ;
#38202=VERTEX_POINT('',#149672) ;
#38203=VERTEX_POINT('',#149673) ;
#38204=VERTEX_POINT('',#149675) ;
#38205=VERTEX_POINT('',#149677) ;
#38206=VERTEX_POINT('',#149681) ;
#38207=VERTEX_POINT('',#149682) ;
#38208=VERTEX_POINT('',#149684) ;
#38209=VERTEX_POINT('',#149686) ;
#38210=VERTEX_POINT('',#149690) ;
#38211=VERTEX_POINT('',#149691) ;
#38212=VERTEX_POINT('',#149696) ;
#38213=VERTEX_POINT('',#149698) ;
#38214=VERTEX_POINT('',#149702) ;
#38215=VERTEX_POINT('',#149703) ;
#38216=VERTEX_POINT('',#149705) ;
#38217=VERTEX_POINT('',#149707) ;
#38218=VERTEX_POINT('',#149711) ;
#38219=VERTEX_POINT('',#149712) ;
#38220=VERTEX_POINT('',#149714) ;
#38221=VERTEX_POINT('',#149716) ;
#38222=VERTEX_POINT('',#149720) ;
#38223=VERTEX_POINT('',#149721) ;
#38224=VERTEX_POINT('',#149723) ;
#38225=VERTEX_POINT('',#149725) ;
#38226=VERTEX_POINT('',#149729) ;
#38227=VERTEX_POINT('',#149730) ;
#38228=VERTEX_POINT('',#149732) ;
#38229=VERTEX_POINT('',#149734) ;
#38230=VERTEX_POINT('',#149738) ;
#38231=VERTEX_POINT('',#149739) ;
#38232=VERTEX_POINT('',#149741) ;
#38233=VERTEX_POINT('',#149743) ;
#38234=VERTEX_POINT('',#149747) ;
#38235=VERTEX_POINT('',#149748) ;
#38236=VERTEX_POINT('',#149751) ;
#38237=VERTEX_POINT('',#149753) ;
#38238=VERTEX_POINT('',#149757) ;
#38239=VERTEX_POINT('',#149758) ;
#38240=VERTEX_POINT('',#149761) ;
#38241=VERTEX_POINT('',#149763) ;
#38242=VERTEX_POINT('',#149773) ;
#38243=VERTEX_POINT('',#149774) ;
#38244=VERTEX_POINT('',#149776) ;
#38245=VERTEX_POINT('',#149778) ;
#38246=VERTEX_POINT('',#149782) ;
#38247=VERTEX_POINT('',#149783) ;
#38248=VERTEX_POINT('',#149788) ;
#38249=VERTEX_POINT('',#149790) ;
#38250=VERTEX_POINT('',#149794) ;
#38251=VERTEX_POINT('',#149795) ;
#38252=VERTEX_POINT('',#149797) ;
#38253=VERTEX_POINT('',#149799) ;
#38254=VERTEX_POINT('',#149803) ;
#38255=VERTEX_POINT('',#149804) ;
#38256=VERTEX_POINT('',#149806) ;
#38257=VERTEX_POINT('',#149808) ;
#38258=VERTEX_POINT('',#149812) ;
#38259=VERTEX_POINT('',#149813) ;
#38260=VERTEX_POINT('',#149818) ;
#38261=VERTEX_POINT('',#149820) ;
#38262=VERTEX_POINT('',#149824) ;
#38263=VERTEX_POINT('',#149825) ;
#38264=VERTEX_POINT('',#149827) ;
#38265=VERTEX_POINT('',#149829) ;
#38266=VERTEX_POINT('',#149833) ;
#38267=VERTEX_POINT('',#149834) ;
#38268=VERTEX_POINT('',#149836) ;
#38269=VERTEX_POINT('',#149838) ;
#38270=VERTEX_POINT('',#149842) ;
#38271=VERTEX_POINT('',#149843) ;
#38272=VERTEX_POINT('',#149845) ;
#38273=VERTEX_POINT('',#149847) ;
#38274=VERTEX_POINT('',#149851) ;
#38275=VERTEX_POINT('',#149852) ;
#38276=VERTEX_POINT('',#149854) ;
#38277=VERTEX_POINT('',#149856) ;
#38278=VERTEX_POINT('',#149860) ;
#38279=VERTEX_POINT('',#149861) ;
#38280=VERTEX_POINT('',#149863) ;
#38281=VERTEX_POINT('',#149865) ;
#38282=VERTEX_POINT('',#149869) ;
#38283=VERTEX_POINT('',#149870) ;
#38284=VERTEX_POINT('',#149873) ;
#38285=VERTEX_POINT('',#149875) ;
#38286=VERTEX_POINT('',#149879) ;
#38287=VERTEX_POINT('',#149880) ;
#38288=VERTEX_POINT('',#149883) ;
#38289=VERTEX_POINT('',#149885) ;
#38290=VERTEX_POINT('',#149895) ;
#38291=VERTEX_POINT('',#149896) ;
#38292=VERTEX_POINT('',#149898) ;
#38293=VERTEX_POINT('',#149900) ;
#38294=VERTEX_POINT('',#149904) ;
#38295=VERTEX_POINT('',#149905) ;
#38296=VERTEX_POINT('',#149910) ;
#38297=VERTEX_POINT('',#149912) ;
#38298=VERTEX_POINT('',#149916) ;
#38299=VERTEX_POINT('',#149917) ;
#38300=VERTEX_POINT('',#149919) ;
#38301=VERTEX_POINT('',#149921) ;
#38302=VERTEX_POINT('',#149925) ;
#38303=VERTEX_POINT('',#149926) ;
#38304=VERTEX_POINT('',#149928) ;
#38305=VERTEX_POINT('',#149930) ;
#38306=VERTEX_POINT('',#149934) ;
#38307=VERTEX_POINT('',#149935) ;
#38308=VERTEX_POINT('',#149940) ;
#38309=VERTEX_POINT('',#149942) ;
#38310=VERTEX_POINT('',#149946) ;
#38311=VERTEX_POINT('',#149947) ;
#38312=VERTEX_POINT('',#149949) ;
#38313=VERTEX_POINT('',#149951) ;
#38314=VERTEX_POINT('',#149955) ;
#38315=VERTEX_POINT('',#149956) ;
#38316=VERTEX_POINT('',#149958) ;
#38317=VERTEX_POINT('',#149960) ;
#38318=VERTEX_POINT('',#149964) ;
#38319=VERTEX_POINT('',#149965) ;
#38320=VERTEX_POINT('',#149967) ;
#38321=VERTEX_POINT('',#149969) ;
#38322=VERTEX_POINT('',#149973) ;
#38323=VERTEX_POINT('',#149974) ;
#38324=VERTEX_POINT('',#149976) ;
#38325=VERTEX_POINT('',#149978) ;
#38326=VERTEX_POINT('',#149982) ;
#38327=VERTEX_POINT('',#149983) ;
#38328=VERTEX_POINT('',#149985) ;
#38329=VERTEX_POINT('',#149987) ;
#38330=VERTEX_POINT('',#149991) ;
#38331=VERTEX_POINT('',#149992) ;
#38332=VERTEX_POINT('',#149995) ;
#38333=VERTEX_POINT('',#149997) ;
#38334=VERTEX_POINT('',#150001) ;
#38335=VERTEX_POINT('',#150002) ;
#38336=VERTEX_POINT('',#150005) ;
#38337=VERTEX_POINT('',#150007) ;
#38338=VERTEX_POINT('',#150017) ;
#38339=VERTEX_POINT('',#150018) ;
#38340=VERTEX_POINT('',#150020) ;
#38341=VERTEX_POINT('',#150022) ;
#38342=VERTEX_POINT('',#150026) ;
#38343=VERTEX_POINT('',#150027) ;
#38344=VERTEX_POINT('',#150032) ;
#38345=VERTEX_POINT('',#150034) ;
#38346=VERTEX_POINT('',#150038) ;
#38347=VERTEX_POINT('',#150039) ;
#38348=VERTEX_POINT('',#150041) ;
#38349=VERTEX_POINT('',#150043) ;
#38350=VERTEX_POINT('',#150047) ;
#38351=VERTEX_POINT('',#150048) ;
#38352=VERTEX_POINT('',#150050) ;
#38353=VERTEX_POINT('',#150052) ;
#38354=VERTEX_POINT('',#150056) ;
#38355=VERTEX_POINT('',#150057) ;
#38356=VERTEX_POINT('',#150062) ;
#38357=VERTEX_POINT('',#150064) ;
#38358=VERTEX_POINT('',#150068) ;
#38359=VERTEX_POINT('',#150069) ;
#38360=VERTEX_POINT('',#150071) ;
#38361=VERTEX_POINT('',#150073) ;
#38362=VERTEX_POINT('',#150077) ;
#38363=VERTEX_POINT('',#150078) ;
#38364=VERTEX_POINT('',#150080) ;
#38365=VERTEX_POINT('',#150082) ;
#38366=VERTEX_POINT('',#150086) ;
#38367=VERTEX_POINT('',#150087) ;
#38368=VERTEX_POINT('',#150089) ;
#38369=VERTEX_POINT('',#150091) ;
#38370=VERTEX_POINT('',#150095) ;
#38371=VERTEX_POINT('',#150096) ;
#38372=VERTEX_POINT('',#150098) ;
#38373=VERTEX_POINT('',#150100) ;
#38374=VERTEX_POINT('',#150104) ;
#38375=VERTEX_POINT('',#150105) ;
#38376=VERTEX_POINT('',#150107) ;
#38377=VERTEX_POINT('',#150109) ;
#38378=VERTEX_POINT('',#150113) ;
#38379=VERTEX_POINT('',#150114) ;
#38380=VERTEX_POINT('',#150117) ;
#38381=VERTEX_POINT('',#150119) ;
#38382=VERTEX_POINT('',#150123) ;
#38383=VERTEX_POINT('',#150124) ;
#38384=VERTEX_POINT('',#150127) ;
#38385=VERTEX_POINT('',#150129) ;
#38386=VERTEX_POINT('',#150139) ;
#38387=VERTEX_POINT('',#150140) ;
#38388=VERTEX_POINT('',#150142) ;
#38389=VERTEX_POINT('',#150144) ;
#38390=VERTEX_POINT('',#150148) ;
#38391=VERTEX_POINT('',#150149) ;
#38392=VERTEX_POINT('',#150154) ;
#38393=VERTEX_POINT('',#150156) ;
#38394=VERTEX_POINT('',#150160) ;
#38395=VERTEX_POINT('',#150161) ;
#38396=VERTEX_POINT('',#150163) ;
#38397=VERTEX_POINT('',#150165) ;
#38398=VERTEX_POINT('',#150169) ;
#38399=VERTEX_POINT('',#150170) ;
#38400=VERTEX_POINT('',#150172) ;
#38401=VERTEX_POINT('',#150174) ;
#38402=VERTEX_POINT('',#150178) ;
#38403=VERTEX_POINT('',#150179) ;
#38404=VERTEX_POINT('',#150184) ;
#38405=VERTEX_POINT('',#150186) ;
#38406=VERTEX_POINT('',#150190) ;
#38407=VERTEX_POINT('',#150191) ;
#38408=VERTEX_POINT('',#150193) ;
#38409=VERTEX_POINT('',#150195) ;
#38410=VERTEX_POINT('',#150199) ;
#38411=VERTEX_POINT('',#150200) ;
#38412=VERTEX_POINT('',#150202) ;
#38413=VERTEX_POINT('',#150204) ;
#38414=VERTEX_POINT('',#150208) ;
#38415=VERTEX_POINT('',#150209) ;
#38416=VERTEX_POINT('',#150211) ;
#38417=VERTEX_POINT('',#150213) ;
#38418=VERTEX_POINT('',#150217) ;
#38419=VERTEX_POINT('',#150218) ;
#38420=VERTEX_POINT('',#150220) ;
#38421=VERTEX_POINT('',#150222) ;
#38422=VERTEX_POINT('',#150226) ;
#38423=VERTEX_POINT('',#150227) ;
#38424=VERTEX_POINT('',#150229) ;
#38425=VERTEX_POINT('',#150231) ;
#38426=VERTEX_POINT('',#150235) ;
#38427=VERTEX_POINT('',#150236) ;
#38428=VERTEX_POINT('',#150239) ;
#38429=VERTEX_POINT('',#150241) ;
#38430=VERTEX_POINT('',#150245) ;
#38431=VERTEX_POINT('',#150246) ;
#38432=VERTEX_POINT('',#150249) ;
#38433=VERTEX_POINT('',#150251) ;
#38434=VERTEX_POINT('',#150261) ;
#38435=VERTEX_POINT('',#150262) ;
#38436=VERTEX_POINT('',#150264) ;
#38437=VERTEX_POINT('',#150266) ;
#38438=VERTEX_POINT('',#150270) ;
#38439=VERTEX_POINT('',#150271) ;
#38440=VERTEX_POINT('',#150276) ;
#38441=VERTEX_POINT('',#150278) ;
#38442=VERTEX_POINT('',#150282) ;
#38443=VERTEX_POINT('',#150283) ;
#38444=VERTEX_POINT('',#150285) ;
#38445=VERTEX_POINT('',#150287) ;
#38446=VERTEX_POINT('',#150291) ;
#38447=VERTEX_POINT('',#150292) ;
#38448=VERTEX_POINT('',#150294) ;
#38449=VERTEX_POINT('',#150296) ;
#38450=VERTEX_POINT('',#150300) ;
#38451=VERTEX_POINT('',#150301) ;
#38452=VERTEX_POINT('',#150306) ;
#38453=VERTEX_POINT('',#150308) ;
#38454=VERTEX_POINT('',#150312) ;
#38455=VERTEX_POINT('',#150313) ;
#38456=VERTEX_POINT('',#150315) ;
#38457=VERTEX_POINT('',#150317) ;
#38458=VERTEX_POINT('',#150321) ;
#38459=VERTEX_POINT('',#150322) ;
#38460=VERTEX_POINT('',#150324) ;
#38461=VERTEX_POINT('',#150326) ;
#38462=VERTEX_POINT('',#150330) ;
#38463=VERTEX_POINT('',#150331) ;
#38464=VERTEX_POINT('',#150333) ;
#38465=VERTEX_POINT('',#150335) ;
#38466=VERTEX_POINT('',#150339) ;
#38467=VERTEX_POINT('',#150340) ;
#38468=VERTEX_POINT('',#150342) ;
#38469=VERTEX_POINT('',#150344) ;
#38470=VERTEX_POINT('',#150348) ;
#38471=VERTEX_POINT('',#150349) ;
#38472=VERTEX_POINT('',#150351) ;
#38473=VERTEX_POINT('',#150353) ;
#38474=VERTEX_POINT('',#150357) ;
#38475=VERTEX_POINT('',#150358) ;
#38476=VERTEX_POINT('',#150361) ;
#38477=VERTEX_POINT('',#150363) ;
#38478=VERTEX_POINT('',#150367) ;
#38479=VERTEX_POINT('',#150368) ;
#38480=VERTEX_POINT('',#150371) ;
#38481=VERTEX_POINT('',#150373) ;
#38482=VERTEX_POINT('',#150383) ;
#38483=VERTEX_POINT('',#150384) ;
#38484=VERTEX_POINT('',#150386) ;
#38485=VERTEX_POINT('',#150388) ;
#38486=VERTEX_POINT('',#150392) ;
#38487=VERTEX_POINT('',#150393) ;
#38488=VERTEX_POINT('',#150398) ;
#38489=VERTEX_POINT('',#150400) ;
#38490=VERTEX_POINT('',#150404) ;
#38491=VERTEX_POINT('',#150405) ;
#38492=VERTEX_POINT('',#150407) ;
#38493=VERTEX_POINT('',#150409) ;
#38494=VERTEX_POINT('',#150413) ;
#38495=VERTEX_POINT('',#150414) ;
#38496=VERTEX_POINT('',#150416) ;
#38497=VERTEX_POINT('',#150418) ;
#38498=VERTEX_POINT('',#150422) ;
#38499=VERTEX_POINT('',#150423) ;
#38500=VERTEX_POINT('',#150428) ;
#38501=VERTEX_POINT('',#150430) ;
#38502=VERTEX_POINT('',#150434) ;
#38503=VERTEX_POINT('',#150435) ;
#38504=VERTEX_POINT('',#150437) ;
#38505=VERTEX_POINT('',#150439) ;
#38506=VERTEX_POINT('',#150443) ;
#38507=VERTEX_POINT('',#150444) ;
#38508=VERTEX_POINT('',#150446) ;
#38509=VERTEX_POINT('',#150448) ;
#38510=VERTEX_POINT('',#150452) ;
#38511=VERTEX_POINT('',#150453) ;
#38512=VERTEX_POINT('',#150455) ;
#38513=VERTEX_POINT('',#150457) ;
#38514=VERTEX_POINT('',#150461) ;
#38515=VERTEX_POINT('',#150462) ;
#38516=VERTEX_POINT('',#150464) ;
#38517=VERTEX_POINT('',#150466) ;
#38518=VERTEX_POINT('',#150470) ;
#38519=VERTEX_POINT('',#150471) ;
#38520=VERTEX_POINT('',#150473) ;
#38521=VERTEX_POINT('',#150475) ;
#38522=VERTEX_POINT('',#150479) ;
#38523=VERTEX_POINT('',#150480) ;
#38524=VERTEX_POINT('',#150483) ;
#38525=VERTEX_POINT('',#150485) ;
#38526=VERTEX_POINT('',#150489) ;
#38527=VERTEX_POINT('',#150490) ;
#38528=VERTEX_POINT('',#150493) ;
#38529=VERTEX_POINT('',#150495) ;
#38530=VERTEX_POINT('',#150505) ;
#38531=VERTEX_POINT('',#150506) ;
#38532=VERTEX_POINT('',#150508) ;
#38533=VERTEX_POINT('',#150510) ;
#38534=VERTEX_POINT('',#150514) ;
#38535=VERTEX_POINT('',#150515) ;
#38536=VERTEX_POINT('',#150520) ;
#38537=VERTEX_POINT('',#150522) ;
#38538=VERTEX_POINT('',#150526) ;
#38539=VERTEX_POINT('',#150527) ;
#38540=VERTEX_POINT('',#150529) ;
#38541=VERTEX_POINT('',#150531) ;
#38542=VERTEX_POINT('',#150535) ;
#38543=VERTEX_POINT('',#150536) ;
#38544=VERTEX_POINT('',#150538) ;
#38545=VERTEX_POINT('',#150540) ;
#38546=VERTEX_POINT('',#150544) ;
#38547=VERTEX_POINT('',#150545) ;
#38548=VERTEX_POINT('',#150550) ;
#38549=VERTEX_POINT('',#150552) ;
#38550=VERTEX_POINT('',#150556) ;
#38551=VERTEX_POINT('',#150557) ;
#38552=VERTEX_POINT('',#150559) ;
#38553=VERTEX_POINT('',#150561) ;
#38554=VERTEX_POINT('',#150565) ;
#38555=VERTEX_POINT('',#150566) ;
#38556=VERTEX_POINT('',#150568) ;
#38557=VERTEX_POINT('',#150570) ;
#38558=VERTEX_POINT('',#150574) ;
#38559=VERTEX_POINT('',#150575) ;
#38560=VERTEX_POINT('',#150577) ;
#38561=VERTEX_POINT('',#150579) ;
#38562=VERTEX_POINT('',#150583) ;
#38563=VERTEX_POINT('',#150584) ;
#38564=VERTEX_POINT('',#150586) ;
#38565=VERTEX_POINT('',#150588) ;
#38566=VERTEX_POINT('',#150592) ;
#38567=VERTEX_POINT('',#150593) ;
#38568=VERTEX_POINT('',#150595) ;
#38569=VERTEX_POINT('',#150597) ;
#38570=VERTEX_POINT('',#150601) ;
#38571=VERTEX_POINT('',#150602) ;
#38572=VERTEX_POINT('',#150605) ;
#38573=VERTEX_POINT('',#150607) ;
#38574=VERTEX_POINT('',#150611) ;
#38575=VERTEX_POINT('',#150612) ;
#38576=VERTEX_POINT('',#150615) ;
#38577=VERTEX_POINT('',#150617) ;
#38578=VERTEX_POINT('',#150627) ;
#38579=VERTEX_POINT('',#150628) ;
#38580=VERTEX_POINT('',#150630) ;
#38581=VERTEX_POINT('',#150632) ;
#38582=VERTEX_POINT('',#150636) ;
#38583=VERTEX_POINT('',#150637) ;
#38584=VERTEX_POINT('',#150642) ;
#38585=VERTEX_POINT('',#150644) ;
#38586=VERTEX_POINT('',#150648) ;
#38587=VERTEX_POINT('',#150649) ;
#38588=VERTEX_POINT('',#150651) ;
#38589=VERTEX_POINT('',#150653) ;
#38590=VERTEX_POINT('',#150657) ;
#38591=VERTEX_POINT('',#150658) ;
#38592=VERTEX_POINT('',#150660) ;
#38593=VERTEX_POINT('',#150662) ;
#38594=VERTEX_POINT('',#150666) ;
#38595=VERTEX_POINT('',#150667) ;
#38596=VERTEX_POINT('',#150672) ;
#38597=VERTEX_POINT('',#150674) ;
#38598=VERTEX_POINT('',#150678) ;
#38599=VERTEX_POINT('',#150679) ;
#38600=VERTEX_POINT('',#150681) ;
#38601=VERTEX_POINT('',#150683) ;
#38602=VERTEX_POINT('',#150687) ;
#38603=VERTEX_POINT('',#150688) ;
#38604=VERTEX_POINT('',#150690) ;
#38605=VERTEX_POINT('',#150692) ;
#38606=VERTEX_POINT('',#150696) ;
#38607=VERTEX_POINT('',#150697) ;
#38608=VERTEX_POINT('',#150699) ;
#38609=VERTEX_POINT('',#150701) ;
#38610=VERTEX_POINT('',#150705) ;
#38611=VERTEX_POINT('',#150706) ;
#38612=VERTEX_POINT('',#150708) ;
#38613=VERTEX_POINT('',#150710) ;
#38614=VERTEX_POINT('',#150714) ;
#38615=VERTEX_POINT('',#150715) ;
#38616=VERTEX_POINT('',#150717) ;
#38617=VERTEX_POINT('',#150719) ;
#38618=VERTEX_POINT('',#150723) ;
#38619=VERTEX_POINT('',#150724) ;
#38620=VERTEX_POINT('',#150726) ;
#38621=VERTEX_POINT('',#150728) ;
#38622=VERTEX_POINT('',#150732) ;
#38623=VERTEX_POINT('',#150733) ;
#38624=VERTEX_POINT('',#150735) ;
#38625=VERTEX_POINT('',#150737) ;
#38626=VERTEX_POINT('',#150741) ;
#38627=VERTEX_POINT('',#150742) ;
#38628=VERTEX_POINT('',#150744) ;
#38629=VERTEX_POINT('',#150746) ;
#38630=VERTEX_POINT('',#150750) ;
#38631=VERTEX_POINT('',#150751) ;
#38632=VERTEX_POINT('',#150753) ;
#38633=VERTEX_POINT('',#150755) ;
#38634=VERTEX_POINT('',#150759) ;
#38635=VERTEX_POINT('',#150760) ;
#38636=VERTEX_POINT('',#150762) ;
#38637=VERTEX_POINT('',#150764) ;
#38638=VERTEX_POINT('',#150768) ;
#38639=VERTEX_POINT('',#150769) ;
#38640=VERTEX_POINT('',#150771) ;
#38641=VERTEX_POINT('',#150773) ;
#38642=VERTEX_POINT('',#150777) ;
#38643=VERTEX_POINT('',#150778) ;
#38644=VERTEX_POINT('',#150780) ;
#38645=VERTEX_POINT('',#150782) ;
#38646=VERTEX_POINT('',#150786) ;
#38647=VERTEX_POINT('',#150787) ;
#38648=VERTEX_POINT('',#150789) ;
#38649=VERTEX_POINT('',#150791) ;
#38650=VERTEX_POINT('',#150795) ;
#38651=VERTEX_POINT('',#150796) ;
#38652=VERTEX_POINT('',#150798) ;
#38653=VERTEX_POINT('',#150800) ;
#38654=VERTEX_POINT('',#150804) ;
#38655=VERTEX_POINT('',#150805) ;
#38656=VERTEX_POINT('',#150807) ;
#38657=VERTEX_POINT('',#150809) ;
#38658=VERTEX_POINT('',#150813) ;
#38659=VERTEX_POINT('',#150814) ;
#38660=VERTEX_POINT('',#150816) ;
#38661=VERTEX_POINT('',#150818) ;
#38662=VERTEX_POINT('',#150822) ;
#38663=VERTEX_POINT('',#150823) ;
#38664=VERTEX_POINT('',#150825) ;
#38665=VERTEX_POINT('',#150827) ;
#38666=VERTEX_POINT('',#150831) ;
#38667=VERTEX_POINT('',#150832) ;
#38668=VERTEX_POINT('',#150834) ;
#38669=VERTEX_POINT('',#150836) ;
#38670=VERTEX_POINT('',#150840) ;
#38671=VERTEX_POINT('',#150841) ;
#38672=VERTEX_POINT('',#150843) ;
#38673=VERTEX_POINT('',#150845) ;
#38674=VERTEX_POINT('',#150849) ;
#38675=VERTEX_POINT('',#150850) ;
#38676=VERTEX_POINT('',#150852) ;
#38677=VERTEX_POINT('',#150854) ;
#38678=VERTEX_POINT('',#150858) ;
#38679=VERTEX_POINT('',#150859) ;
#38680=VERTEX_POINT('',#150861) ;
#38681=VERTEX_POINT('',#150863) ;
#38682=VERTEX_POINT('',#150867) ;
#38683=VERTEX_POINT('',#150868) ;
#38684=VERTEX_POINT('',#150870) ;
#38685=VERTEX_POINT('',#150872) ;
#38686=VERTEX_POINT('',#150876) ;
#38687=VERTEX_POINT('',#150877) ;
#38688=VERTEX_POINT('',#150879) ;
#38689=VERTEX_POINT('',#150881) ;
#38690=VERTEX_POINT('',#150885) ;
#38691=VERTEX_POINT('',#150886) ;
#38692=VERTEX_POINT('',#150888) ;
#38693=VERTEX_POINT('',#150890) ;
#38694=VERTEX_POINT('',#150894) ;
#38695=VERTEX_POINT('',#150895) ;
#38696=VERTEX_POINT('',#150897) ;
#38697=VERTEX_POINT('',#150899) ;
#38698=VERTEX_POINT('',#150903) ;
#38699=VERTEX_POINT('',#150904) ;
#38700=VERTEX_POINT('',#150906) ;
#38701=VERTEX_POINT('',#150908) ;
#38702=VERTEX_POINT('',#150912) ;
#38703=VERTEX_POINT('',#150913) ;
#38704=VERTEX_POINT('',#150915) ;
#38705=VERTEX_POINT('',#150917) ;
#38706=VERTEX_POINT('',#150921) ;
#38707=VERTEX_POINT('',#150922) ;
#38708=VERTEX_POINT('',#150924) ;
#38709=VERTEX_POINT('',#150926) ;
#38710=VERTEX_POINT('',#150930) ;
#38711=VERTEX_POINT('',#150931) ;
#38712=VERTEX_POINT('',#150933) ;
#38713=VERTEX_POINT('',#150935) ;
#38714=VERTEX_POINT('',#150939) ;
#38715=VERTEX_POINT('',#150940) ;
#38716=VERTEX_POINT('',#150942) ;
#38717=VERTEX_POINT('',#150944) ;
#38718=VERTEX_POINT('',#150948) ;
#38719=VERTEX_POINT('',#150949) ;
#38720=VERTEX_POINT('',#150951) ;
#38721=VERTEX_POINT('',#150953) ;
#38722=VERTEX_POINT('',#150957) ;
#38723=VERTEX_POINT('',#150958) ;
#38724=VERTEX_POINT('',#150960) ;
#38725=VERTEX_POINT('',#150962) ;
#38726=VERTEX_POINT('',#150966) ;
#38727=VERTEX_POINT('',#150967) ;
#38728=VERTEX_POINT('',#150969) ;
#38729=VERTEX_POINT('',#150971) ;
#38730=VERTEX_POINT('',#150975) ;
#38731=VERTEX_POINT('',#150976) ;
#38732=VERTEX_POINT('',#150978) ;
#38733=VERTEX_POINT('',#150980) ;
#38734=VERTEX_POINT('',#150984) ;
#38735=VERTEX_POINT('',#150985) ;
#38736=VERTEX_POINT('',#150987) ;
#38737=VERTEX_POINT('',#150989) ;
#38738=VERTEX_POINT('',#150993) ;
#38739=VERTEX_POINT('',#150994) ;
#38740=VERTEX_POINT('',#150996) ;
#38741=VERTEX_POINT('',#150998) ;
#44147=EDGE_CURVE('',#36190,#36190,#29733,.T.) ;
#44148=EDGE_CURVE('',#36190,#36191,#29734,.T.) ;
#44149=EDGE_CURVE('',#36192,#36191,#29735,.T.) ;
#44150=EDGE_CURVE('',#36191,#36192,#29736,.T.) ;
#44151=EDGE_CURVE('',#36193,#36193,#29737,.T.) ;
#44152=EDGE_CURVE('',#36193,#36194,#29738,.T.) ;
#44153=EDGE_CURVE('',#36194,#36194,#29739,.T.) ;
#44154=EDGE_CURVE('',#36195,#36196,#29740,.T.) ;
#44155=EDGE_CURVE('',#36197,#36195,#29741,.T.) ;
#44156=EDGE_CURVE('',#36197,#36196,#29742,.T.) ;
#44157=EDGE_CURVE('',#36198,#36199,#357,.T.) ;
#44158=EDGE_CURVE('',#36198,#36200,#29743,.T.) ;
#44159=EDGE_CURVE('',#36201,#36200,#3629,.T.) ;
#44160=EDGE_CURVE('',#36202,#36201,#29744,.T.) ;
#44161=EDGE_CURVE('',#36203,#36202,#3630,.T.) ;
#44162=EDGE_CURVE('',#36204,#36203,#3631,.T.) ;
#44163=EDGE_CURVE('',#36204,#36199,#2157,.T.) ;
#44164=EDGE_CURVE('',#36205,#36205,#29745,.T.) ;
#44165=EDGE_CURVE('',#36205,#36206,#29746,.T.) ;
#44166=EDGE_CURVE('',#36207,#36206,#29747,.T.) ;
#44167=EDGE_CURVE('',#36206,#36207,#29748,.T.) ;
#44168=EDGE_CURVE('',#36208,#36208,#29749,.T.) ;
#44169=EDGE_CURVE('',#36208,#36209,#29750,.T.) ;
#44170=EDGE_CURVE('',#36209,#36209,#29751,.T.) ;
#44171=EDGE_CURVE('',#36210,#36211,#29752,.T.) ;
#44172=EDGE_CURVE('',#36212,#36210,#29753,.T.) ;
#44173=EDGE_CURVE('',#36212,#36211,#29754,.T.) ;
#44174=EDGE_CURVE('',#36213,#36214,#358,.T.) ;
#44175=EDGE_CURVE('',#36213,#36215,#29755,.T.) ;
#44176=EDGE_CURVE('',#36216,#36215,#3632,.T.) ;
#44177=EDGE_CURVE('',#36217,#36216,#29756,.T.) ;
#44178=EDGE_CURVE('',#36218,#36217,#3633,.T.) ;
#44179=EDGE_CURVE('',#36219,#36218,#3634,.T.) ;
#44180=EDGE_CURVE('',#36219,#36214,#2158,.T.) ;
#44181=EDGE_CURVE('',#36220,#36220,#29757,.T.) ;
#44182=EDGE_CURVE('',#36220,#36221,#29758,.T.) ;
#44183=EDGE_CURVE('',#36222,#36221,#29759,.T.) ;
#44184=EDGE_CURVE('',#36221,#36222,#29760,.T.) ;
#44185=EDGE_CURVE('',#36223,#36223,#29761,.T.) ;
#44186=EDGE_CURVE('',#36223,#36224,#29762,.T.) ;
#44187=EDGE_CURVE('',#36224,#36224,#29763,.T.) ;
#44188=EDGE_CURVE('',#36225,#36226,#29764,.T.) ;
#44189=EDGE_CURVE('',#36227,#36225,#29765,.T.) ;
#44190=EDGE_CURVE('',#36227,#36226,#29766,.T.) ;
#44191=EDGE_CURVE('',#36228,#36229,#359,.T.) ;
#44192=EDGE_CURVE('',#36228,#36230,#29767,.T.) ;
#44193=EDGE_CURVE('',#36231,#36230,#3635,.T.) ;
#44194=EDGE_CURVE('',#36232,#36231,#29768,.T.) ;
#44195=EDGE_CURVE('',#36233,#36232,#3636,.T.) ;
#44196=EDGE_CURVE('',#36234,#36233,#3637,.T.) ;
#44197=EDGE_CURVE('',#36234,#36229,#2159,.T.) ;
#44198=EDGE_CURVE('',#36235,#36235,#29769,.T.) ;
#44199=EDGE_CURVE('',#36235,#36236,#29770,.T.) ;
#44200=EDGE_CURVE('',#36237,#36236,#29771,.T.) ;
#44201=EDGE_CURVE('',#36236,#36237,#29772,.T.) ;
#44202=EDGE_CURVE('',#36238,#36238,#29773,.T.) ;
#44203=EDGE_CURVE('',#36238,#36239,#29774,.T.) ;
#44204=EDGE_CURVE('',#36239,#36239,#29775,.T.) ;
#44205=EDGE_CURVE('',#36240,#36241,#29776,.T.) ;
#44206=EDGE_CURVE('',#36242,#36240,#29777,.T.) ;
#44207=EDGE_CURVE('',#36242,#36241,#29778,.T.) ;
#44208=EDGE_CURVE('',#36243,#36244,#360,.T.) ;
#44209=EDGE_CURVE('',#36243,#36245,#29779,.T.) ;
#44210=EDGE_CURVE('',#36246,#36245,#3638,.T.) ;
#44211=EDGE_CURVE('',#36247,#36246,#29780,.T.) ;
#44212=EDGE_CURVE('',#36248,#36247,#3639,.T.) ;
#44213=EDGE_CURVE('',#36249,#36248,#3640,.T.) ;
#44214=EDGE_CURVE('',#36249,#36244,#2160,.T.) ;
#44215=EDGE_CURVE('',#36250,#36250,#29781,.T.) ;
#44216=EDGE_CURVE('',#36250,#36251,#29782,.T.) ;
#44217=EDGE_CURVE('',#36252,#36251,#29783,.T.) ;
#44218=EDGE_CURVE('',#36251,#36252,#29784,.T.) ;
#44219=EDGE_CURVE('',#36253,#36253,#29785,.T.) ;
#44220=EDGE_CURVE('',#36253,#36254,#29786,.T.) ;
#44221=EDGE_CURVE('',#36254,#36254,#29787,.T.) ;
#44222=EDGE_CURVE('',#36255,#36256,#29788,.T.) ;
#44223=EDGE_CURVE('',#36257,#36255,#29789,.T.) ;
#44224=EDGE_CURVE('',#36257,#36256,#29790,.T.) ;
#44225=EDGE_CURVE('',#36258,#36259,#361,.T.) ;
#44226=EDGE_CURVE('',#36258,#36260,#29791,.T.) ;
#44227=EDGE_CURVE('',#36261,#36260,#3641,.T.) ;
#44228=EDGE_CURVE('',#36262,#36261,#29792,.T.) ;
#44229=EDGE_CURVE('',#36263,#36262,#3642,.T.) ;
#44230=EDGE_CURVE('',#36264,#36263,#3643,.T.) ;
#44231=EDGE_CURVE('',#36264,#36259,#2161,.T.) ;
#44232=EDGE_CURVE('',#36265,#36265,#29793,.T.) ;
#44233=EDGE_CURVE('',#36265,#36266,#29794,.T.) ;
#44234=EDGE_CURVE('',#36267,#36266,#29795,.T.) ;
#44235=EDGE_CURVE('',#36266,#36267,#29796,.T.) ;
#44236=EDGE_CURVE('',#36268,#36268,#29797,.T.) ;
#44237=EDGE_CURVE('',#36268,#36269,#29798,.T.) ;
#44238=EDGE_CURVE('',#36269,#36269,#29799,.T.) ;
#44239=EDGE_CURVE('',#36270,#36271,#29800,.T.) ;
#44240=EDGE_CURVE('',#36272,#36270,#29801,.T.) ;
#44241=EDGE_CURVE('',#36272,#36271,#29802,.T.) ;
#44242=EDGE_CURVE('',#36273,#36274,#362,.T.) ;
#44243=EDGE_CURVE('',#36273,#36275,#29803,.T.) ;
#44244=EDGE_CURVE('',#36276,#36275,#3644,.T.) ;
#44245=EDGE_CURVE('',#36277,#36276,#29804,.T.) ;
#44246=EDGE_CURVE('',#36278,#36277,#3645,.T.) ;
#44247=EDGE_CURVE('',#36279,#36278,#3646,.T.) ;
#44248=EDGE_CURVE('',#36279,#36274,#2162,.T.) ;
#44249=EDGE_CURVE('',#36280,#36280,#29805,.T.) ;
#44250=EDGE_CURVE('',#36280,#36281,#29806,.T.) ;
#44251=EDGE_CURVE('',#36282,#36281,#29807,.T.) ;
#44252=EDGE_CURVE('',#36281,#36282,#29808,.T.) ;
#44253=EDGE_CURVE('',#36283,#36283,#29809,.T.) ;
#44254=EDGE_CURVE('',#36283,#36284,#29810,.T.) ;
#44255=EDGE_CURVE('',#36284,#36284,#29811,.T.) ;
#44256=EDGE_CURVE('',#36285,#36286,#29812,.T.) ;
#44257=EDGE_CURVE('',#36287,#36285,#29813,.T.) ;
#44258=EDGE_CURVE('',#36287,#36286,#29814,.T.) ;
#44259=EDGE_CURVE('',#36288,#36289,#363,.T.) ;
#44260=EDGE_CURVE('',#36288,#36290,#29815,.T.) ;
#44261=EDGE_CURVE('',#36291,#36290,#3647,.T.) ;
#44262=EDGE_CURVE('',#36292,#36291,#29816,.T.) ;
#44263=EDGE_CURVE('',#36293,#36292,#3648,.T.) ;
#44264=EDGE_CURVE('',#36294,#36293,#3649,.T.) ;
#44265=EDGE_CURVE('',#36294,#36289,#2163,.T.) ;
#44266=EDGE_CURVE('',#36295,#36295,#29817,.T.) ;
#44267=EDGE_CURVE('',#36295,#36296,#29818,.T.) ;
#44268=EDGE_CURVE('',#36297,#36296,#29819,.T.) ;
#44269=EDGE_CURVE('',#36296,#36297,#29820,.T.) ;
#44270=EDGE_CURVE('',#36298,#36298,#29821,.T.) ;
#44271=EDGE_CURVE('',#36298,#36299,#29822,.T.) ;
#44272=EDGE_CURVE('',#36299,#36299,#29823,.T.) ;
#44273=EDGE_CURVE('',#36300,#36301,#29824,.T.) ;
#44274=EDGE_CURVE('',#36302,#36300,#29825,.T.) ;
#44275=EDGE_CURVE('',#36302,#36301,#29826,.T.) ;
#44276=EDGE_CURVE('',#36303,#36304,#364,.T.) ;
#44277=EDGE_CURVE('',#36303,#36305,#29827,.T.) ;
#44278=EDGE_CURVE('',#36306,#36305,#3650,.T.) ;
#44279=EDGE_CURVE('',#36307,#36306,#29828,.T.) ;
#44280=EDGE_CURVE('',#36308,#36307,#3651,.T.) ;
#44281=EDGE_CURVE('',#36309,#36308,#3652,.T.) ;
#44282=EDGE_CURVE('',#36309,#36304,#2164,.T.) ;
#44283=EDGE_CURVE('',#36310,#36310,#29829,.T.) ;
#44284=EDGE_CURVE('',#36310,#36311,#29830,.T.) ;
#44285=EDGE_CURVE('',#36312,#36311,#29831,.T.) ;
#44286=EDGE_CURVE('',#36311,#36312,#29832,.T.) ;
#44287=EDGE_CURVE('',#36313,#36314,#29833,.T.) ;
#44288=EDGE_CURVE('',#36315,#36313,#29834,.T.) ;
#44289=EDGE_CURVE('',#36316,#36315,#29835,.T.) ;
#44290=EDGE_CURVE('',#36316,#36314,#29836,.T.) ;
#44291=EDGE_CURVE('',#36317,#36318,#29837,.T.) ;
#44292=EDGE_CURVE('',#36319,#36317,#29838,.T.) ;
#44293=EDGE_CURVE('',#36320,#36319,#29839,.T.) ;
#44294=EDGE_CURVE('',#36320,#36318,#29840,.T.) ;
#44295=EDGE_CURVE('',#36321,#36322,#29841,.T.) ;
#44296=EDGE_CURVE('',#36323,#36321,#29842,.T.) ;
#44297=EDGE_CURVE('',#36324,#36323,#29843,.T.) ;
#44298=EDGE_CURVE('',#36324,#36322,#29844,.T.) ;
#44299=EDGE_CURVE('',#36325,#36326,#29845,.T.) ;
#44300=EDGE_CURVE('',#36327,#36325,#29846,.T.) ;
#44301=EDGE_CURVE('',#36328,#36327,#29847,.T.) ;
#44302=EDGE_CURVE('',#36328,#36326,#29848,.T.) ;
#44303=EDGE_CURVE('',#36329,#36330,#29849,.T.) ;
#44304=EDGE_CURVE('',#36331,#36329,#29850,.T.) ;
#44305=EDGE_CURVE('',#36332,#36331,#29851,.T.) ;
#44306=EDGE_CURVE('',#36332,#36330,#29852,.T.) ;
#44307=EDGE_CURVE('',#36333,#36334,#29853,.T.) ;
#44308=EDGE_CURVE('',#36335,#36333,#29854,.T.) ;
#44309=EDGE_CURVE('',#36336,#36335,#29855,.T.) ;
#44310=EDGE_CURVE('',#36336,#36334,#29856,.T.) ;
#44311=EDGE_CURVE('',#36337,#36338,#29857,.T.) ;
#44312=EDGE_CURVE('',#36339,#36337,#29858,.T.) ;
#44313=EDGE_CURVE('',#36340,#36339,#29859,.T.) ;
#44314=EDGE_CURVE('',#36340,#36338,#29860,.T.) ;
#44315=EDGE_CURVE('',#36341,#36342,#29861,.T.) ;
#44316=EDGE_CURVE('',#36343,#36341,#29862,.T.) ;
#44317=EDGE_CURVE('',#36344,#36343,#29863,.T.) ;
#44318=EDGE_CURVE('',#36344,#36342,#29864,.T.) ;
#44319=EDGE_CURVE('',#36345,#36346,#29865,.T.) ;
#44320=EDGE_CURVE('',#36347,#36345,#29866,.T.) ;
#44321=EDGE_CURVE('',#36348,#36347,#29867,.T.) ;
#44322=EDGE_CURVE('',#36348,#36346,#29868,.T.) ;
#44323=EDGE_CURVE('',#36349,#36349,#29869,.T.) ;
#44324=EDGE_CURVE('',#36349,#36350,#29870,.T.) ;
#44325=EDGE_CURVE('',#36350,#36350,#29871,.T.) ;
#44326=EDGE_CURVE('',#36351,#36352,#29872,.T.) ;
#44327=EDGE_CURVE('',#36353,#36351,#29873,.T.) ;
#44328=EDGE_CURVE('',#36353,#36352,#29874,.T.) ;
#44329=EDGE_CURVE('',#36354,#36355,#365,.T.) ;
#44330=EDGE_CURVE('',#36354,#36356,#29875,.T.) ;
#44331=EDGE_CURVE('',#36357,#36356,#3653,.T.) ;
#44332=EDGE_CURVE('',#36358,#36357,#29876,.T.) ;
#44333=EDGE_CURVE('',#36359,#36358,#3654,.T.) ;
#44334=EDGE_CURVE('',#36360,#36359,#3655,.T.) ;
#44335=EDGE_CURVE('',#36360,#36355,#2165,.T.) ;
#44336=EDGE_CURVE('',#36194,#36192,#3656,.T.) ;
#44337=EDGE_CURVE('',#36209,#36207,#3657,.T.) ;
#44338=EDGE_CURVE('',#36224,#36222,#3658,.T.) ;
#44339=EDGE_CURVE('',#36239,#36237,#3659,.T.) ;
#44340=EDGE_CURVE('',#36254,#36252,#3660,.T.) ;
#44341=EDGE_CURVE('',#36269,#36267,#3661,.T.) ;
#44342=EDGE_CURVE('',#36284,#36282,#3662,.T.) ;
#44343=EDGE_CURVE('',#36299,#36297,#3663,.T.) ;
#44344=EDGE_CURVE('',#36350,#36312,#3664,.T.) ;
#44345=EDGE_CURVE('',#36361,#36362,#29877,.T.) ;
#44346=EDGE_CURVE('',#36362,#36316,#3665,.T.) ;
#44347=EDGE_CURVE('',#36361,#36315,#3666,.T.) ;
#44348=EDGE_CURVE('',#36363,#36364,#29878,.T.) ;
#44349=EDGE_CURVE('',#36364,#36320,#3667,.T.) ;
#44350=EDGE_CURVE('',#36363,#36319,#3668,.T.) ;
#44351=EDGE_CURVE('',#36365,#36366,#29879,.T.) ;
#44352=EDGE_CURVE('',#36366,#36324,#3669,.T.) ;
#44353=EDGE_CURVE('',#36365,#36323,#3670,.T.) ;
#44354=EDGE_CURVE('',#36367,#36368,#29880,.T.) ;
#44355=EDGE_CURVE('',#36368,#36328,#3671,.T.) ;
#44356=EDGE_CURVE('',#36367,#36327,#3672,.T.) ;
#44357=EDGE_CURVE('',#36369,#36370,#29881,.T.) ;
#44358=EDGE_CURVE('',#36370,#36332,#3673,.T.) ;
#44359=EDGE_CURVE('',#36369,#36331,#3674,.T.) ;
#44360=EDGE_CURVE('',#36371,#36372,#29882,.T.) ;
#44361=EDGE_CURVE('',#36372,#36336,#3675,.T.) ;
#44362=EDGE_CURVE('',#36371,#36335,#3676,.T.) ;
#44363=EDGE_CURVE('',#36373,#36374,#29883,.T.) ;
#44364=EDGE_CURVE('',#36374,#36340,#3677,.T.) ;
#44365=EDGE_CURVE('',#36373,#36339,#3678,.T.) ;
#44366=EDGE_CURVE('',#36375,#36376,#29884,.T.) ;
#44367=EDGE_CURVE('',#36376,#36344,#3679,.T.) ;
#44368=EDGE_CURVE('',#36375,#36343,#3680,.T.) ;
#44369=EDGE_CURVE('',#36377,#36378,#29885,.T.) ;
#44370=EDGE_CURVE('',#36378,#36348,#3681,.T.) ;
#44371=EDGE_CURVE('',#36377,#36347,#3682,.T.) ;
#44372=EDGE_CURVE('',#36379,#36379,#29886,.T.) ;
#44373=EDGE_CURVE('',#36379,#36380,#29887,.T.) ;
#44374=EDGE_CURVE('',#36381,#36380,#29888,.T.) ;
#44375=EDGE_CURVE('',#36380,#36381,#29889,.T.) ;
#44376=EDGE_CURVE('',#36382,#36383,#29890,.T.) ;
#44377=EDGE_CURVE('',#36384,#36382,#29891,.T.) ;
#44378=EDGE_CURVE('',#36385,#36384,#29892,.T.) ;
#44379=EDGE_CURVE('',#36385,#36383,#29893,.T.) ;
#44380=EDGE_CURVE('',#36386,#36386,#29894,.T.) ;
#44381=EDGE_CURVE('',#36386,#36387,#29895,.T.) ;
#44382=EDGE_CURVE('',#36387,#36387,#29896,.T.) ;
#44383=EDGE_CURVE('',#36388,#36389,#29897,.T.) ;
#44384=EDGE_CURVE('',#36390,#36388,#29898,.T.) ;
#44385=EDGE_CURVE('',#36390,#36389,#29899,.T.) ;
#44386=EDGE_CURVE('',#36391,#36392,#366,.T.) ;
#44387=EDGE_CURVE('',#36391,#36393,#29900,.T.) ;
#44388=EDGE_CURVE('',#36394,#36393,#3683,.T.) ;
#44389=EDGE_CURVE('',#36395,#36394,#29901,.T.) ;
#44390=EDGE_CURVE('',#36396,#36395,#3684,.T.) ;
#44391=EDGE_CURVE('',#36397,#36396,#3685,.T.) ;
#44392=EDGE_CURVE('',#36397,#36392,#2166,.T.) ;
#44393=EDGE_CURVE('',#36387,#36381,#3686,.T.) ;
#44394=EDGE_CURVE('',#36398,#36399,#29902,.T.) ;
#44395=EDGE_CURVE('',#36399,#36385,#3687,.T.) ;
#44396=EDGE_CURVE('',#36398,#36384,#3688,.T.) ;
#44397=EDGE_CURVE('',#36400,#36401,#3689,.T.) ;
#44398=EDGE_CURVE('',#36401,#36402,#29903,.T.) ;
#44399=EDGE_CURVE('',#36402,#36403,#3690,.T.) ;
#44400=EDGE_CURVE('',#36403,#36203,#29904,.T.) ;
#44401=EDGE_CURVE('',#36404,#36202,#29905,.T.) ;
#44402=EDGE_CURVE('',#36404,#36405,#3691,.T.) ;
#44403=EDGE_CURVE('',#36405,#36406,#3692,.T.) ;
#44404=EDGE_CURVE('',#36406,#36407,#3693,.T.) ;
#44405=EDGE_CURVE('',#36407,#36408,#3694,.T.) ;
#44406=EDGE_CURVE('',#36408,#36409,#3695,.T.) ;
#44407=EDGE_CURVE('',#36400,#36409,#29906,.T.) ;
#44408=EDGE_CURVE('',#36410,#36411,#3696,.T.) ;
#44409=EDGE_CURVE('',#36411,#36412,#29907,.T.) ;
#44410=EDGE_CURVE('',#36412,#36413,#3697,.T.) ;
#44411=EDGE_CURVE('',#36413,#36218,#29908,.T.) ;
#44412=EDGE_CURVE('',#36414,#36217,#29909,.T.) ;
#44413=EDGE_CURVE('',#36414,#36415,#3698,.T.) ;
#44414=EDGE_CURVE('',#36415,#36416,#3699,.T.) ;
#44415=EDGE_CURVE('',#36416,#36417,#3700,.T.) ;
#44416=EDGE_CURVE('',#36417,#36418,#3701,.T.) ;
#44417=EDGE_CURVE('',#36418,#36419,#3702,.T.) ;
#44418=EDGE_CURVE('',#36410,#36419,#29910,.T.) ;
#44419=EDGE_CURVE('',#36420,#36421,#3703,.T.) ;
#44420=EDGE_CURVE('',#36421,#36422,#29911,.T.) ;
#44421=EDGE_CURVE('',#36422,#36423,#3704,.T.) ;
#44422=EDGE_CURVE('',#36423,#36233,#29912,.T.) ;
#44423=EDGE_CURVE('',#36424,#36232,#29913,.T.) ;
#44424=EDGE_CURVE('',#36424,#36425,#3705,.T.) ;
#44425=EDGE_CURVE('',#36425,#36426,#3706,.T.) ;
#44426=EDGE_CURVE('',#36426,#36427,#3707,.T.) ;
#44427=EDGE_CURVE('',#36427,#36428,#3708,.T.) ;
#44428=EDGE_CURVE('',#36428,#36429,#3709,.T.) ;
#44429=EDGE_CURVE('',#36420,#36429,#29914,.T.) ;
#44430=EDGE_CURVE('',#36430,#36431,#3710,.T.) ;
#44431=EDGE_CURVE('',#36431,#36432,#29915,.T.) ;
#44432=EDGE_CURVE('',#36432,#36433,#3711,.T.) ;
#44433=EDGE_CURVE('',#36433,#36248,#29916,.T.) ;
#44434=EDGE_CURVE('',#36434,#36247,#29917,.T.) ;
#44435=EDGE_CURVE('',#36434,#36435,#3712,.T.) ;
#44436=EDGE_CURVE('',#36435,#36436,#3713,.T.) ;
#44437=EDGE_CURVE('',#36436,#36437,#3714,.T.) ;
#44438=EDGE_CURVE('',#36437,#36438,#3715,.T.) ;
#44439=EDGE_CURVE('',#36438,#36439,#3716,.T.) ;
#44440=EDGE_CURVE('',#36430,#36439,#29918,.T.) ;
#44441=EDGE_CURVE('',#36440,#36441,#3717,.T.) ;
#44442=EDGE_CURVE('',#36441,#36442,#29919,.T.) ;
#44443=EDGE_CURVE('',#36442,#36443,#3718,.T.) ;
#44444=EDGE_CURVE('',#36443,#36263,#29920,.T.) ;
#44445=EDGE_CURVE('',#36444,#36262,#29921,.T.) ;
#44446=EDGE_CURVE('',#36444,#36445,#3719,.T.) ;
#44447=EDGE_CURVE('',#36445,#36446,#3720,.T.) ;
#44448=EDGE_CURVE('',#36446,#36447,#3721,.T.) ;
#44449=EDGE_CURVE('',#36447,#36448,#3722,.T.) ;
#44450=EDGE_CURVE('',#36448,#36449,#3723,.T.) ;
#44451=EDGE_CURVE('',#36440,#36449,#29922,.T.) ;
#44452=EDGE_CURVE('',#36450,#36451,#3724,.T.) ;
#44453=EDGE_CURVE('',#36451,#36452,#29923,.T.) ;
#44454=EDGE_CURVE('',#36452,#36453,#3725,.T.) ;
#44455=EDGE_CURVE('',#36453,#36278,#29924,.T.) ;
#44456=EDGE_CURVE('',#36454,#36277,#29925,.T.) ;
#44457=EDGE_CURVE('',#36454,#36455,#3726,.T.) ;
#44458=EDGE_CURVE('',#36455,#36456,#3727,.T.) ;
#44459=EDGE_CURVE('',#36456,#36457,#3728,.T.) ;
#44460=EDGE_CURVE('',#36457,#36458,#3729,.T.) ;
#44461=EDGE_CURVE('',#36458,#36459,#3730,.T.) ;
#44462=EDGE_CURVE('',#36450,#36459,#29926,.T.) ;
#44463=EDGE_CURVE('',#36460,#36461,#3731,.T.) ;
#44464=EDGE_CURVE('',#36461,#36462,#29927,.T.) ;
#44465=EDGE_CURVE('',#36462,#36463,#3732,.T.) ;
#44466=EDGE_CURVE('',#36463,#36293,#29928,.T.) ;
#44467=EDGE_CURVE('',#36464,#36292,#29929,.T.) ;
#44468=EDGE_CURVE('',#36464,#36465,#3733,.T.) ;
#44469=EDGE_CURVE('',#36465,#36466,#3734,.T.) ;
#44470=EDGE_CURVE('',#36466,#36467,#3735,.T.) ;
#44471=EDGE_CURVE('',#36467,#36468,#3736,.T.) ;
#44472=EDGE_CURVE('',#36468,#36469,#3737,.T.) ;
#44473=EDGE_CURVE('',#36460,#36469,#29930,.T.) ;
#44474=EDGE_CURVE('',#36470,#36471,#3738,.T.) ;
#44475=EDGE_CURVE('',#36471,#36472,#29931,.T.) ;
#44476=EDGE_CURVE('',#36472,#36473,#3739,.T.) ;
#44477=EDGE_CURVE('',#36473,#36308,#29932,.T.) ;
#44478=EDGE_CURVE('',#36474,#36307,#29933,.T.) ;
#44479=EDGE_CURVE('',#36474,#36475,#3740,.T.) ;
#44480=EDGE_CURVE('',#36475,#36476,#3741,.T.) ;
#44481=EDGE_CURVE('',#36476,#36477,#3742,.T.) ;
#44482=EDGE_CURVE('',#36477,#36478,#3743,.T.) ;
#44483=EDGE_CURVE('',#36478,#36479,#3744,.T.) ;
#44484=EDGE_CURVE('',#36470,#36479,#29934,.T.) ;
#44485=EDGE_CURVE('',#36480,#36481,#3745,.T.) ;
#44486=EDGE_CURVE('',#36481,#36482,#29935,.T.) ;
#44487=EDGE_CURVE('',#36482,#36483,#3746,.T.) ;
#44488=EDGE_CURVE('',#36483,#36359,#29936,.T.) ;
#44489=EDGE_CURVE('',#36484,#36358,#29937,.T.) ;
#44490=EDGE_CURVE('',#36484,#36485,#3747,.T.) ;
#44491=EDGE_CURVE('',#36485,#36486,#3748,.T.) ;
#44492=EDGE_CURVE('',#36486,#36487,#3749,.T.) ;
#44493=EDGE_CURVE('',#36487,#36488,#3750,.T.) ;
#44494=EDGE_CURVE('',#36488,#36489,#3751,.T.) ;
#44495=EDGE_CURVE('',#36480,#36489,#29938,.T.) ;
#44496=EDGE_CURVE('',#36490,#36491,#29939,.T.) ;
#44497=EDGE_CURVE('',#36490,#36492,#3752,.T.) ;
#44498=EDGE_CURVE('',#36492,#36493,#3753,.T.) ;
#44499=EDGE_CURVE('',#36493,#36494,#3754,.T.) ;
#44500=EDGE_CURVE('',#36494,#36491,#3755,.T.) ;
#44501=EDGE_CURVE('',#36495,#36496,#29940,.T.) ;
#44502=EDGE_CURVE('',#36495,#36497,#3756,.T.) ;
#44503=EDGE_CURVE('',#36497,#36498,#3757,.T.) ;
#44504=EDGE_CURVE('',#36498,#36499,#3758,.T.) ;
#44505=EDGE_CURVE('',#36499,#36496,#3759,.T.) ;
#44506=EDGE_CURVE('',#36500,#36501,#29941,.T.) ;
#44507=EDGE_CURVE('',#36500,#36502,#3760,.T.) ;
#44508=EDGE_CURVE('',#36502,#36503,#3761,.T.) ;
#44509=EDGE_CURVE('',#36503,#36504,#3762,.T.) ;
#44510=EDGE_CURVE('',#36504,#36501,#3763,.T.) ;
#44511=EDGE_CURVE('',#36505,#36506,#29942,.T.) ;
#44512=EDGE_CURVE('',#36505,#36507,#3764,.T.) ;
#44513=EDGE_CURVE('',#36507,#36508,#3765,.T.) ;
#44514=EDGE_CURVE('',#36508,#36509,#3766,.T.) ;
#44515=EDGE_CURVE('',#36509,#36506,#3767,.T.) ;
#44516=EDGE_CURVE('',#36510,#36511,#29943,.T.) ;
#44517=EDGE_CURVE('',#36510,#36512,#3768,.T.) ;
#44518=EDGE_CURVE('',#36512,#36513,#3769,.T.) ;
#44519=EDGE_CURVE('',#36513,#36514,#3770,.T.) ;
#44520=EDGE_CURVE('',#36514,#36511,#3771,.T.) ;
#44521=EDGE_CURVE('',#36515,#36516,#29944,.T.) ;
#44522=EDGE_CURVE('',#36515,#36517,#3772,.T.) ;
#44523=EDGE_CURVE('',#36517,#36518,#3773,.T.) ;
#44524=EDGE_CURVE('',#36518,#36519,#3774,.T.) ;
#44525=EDGE_CURVE('',#36519,#36516,#3775,.T.) ;
#44526=EDGE_CURVE('',#36520,#36521,#29945,.T.) ;
#44527=EDGE_CURVE('',#36520,#36522,#3776,.T.) ;
#44528=EDGE_CURVE('',#36522,#36523,#3777,.T.) ;
#44529=EDGE_CURVE('',#36523,#36524,#3778,.T.) ;
#44530=EDGE_CURVE('',#36524,#36521,#3779,.T.) ;
#44531=EDGE_CURVE('',#36525,#36526,#29946,.T.) ;
#44532=EDGE_CURVE('',#36525,#36527,#3780,.T.) ;
#44533=EDGE_CURVE('',#36527,#36528,#3781,.T.) ;
#44534=EDGE_CURVE('',#36528,#36529,#3782,.T.) ;
#44535=EDGE_CURVE('',#36529,#36526,#3783,.T.) ;
#44536=EDGE_CURVE('',#36530,#36531,#29947,.T.) ;
#44537=EDGE_CURVE('',#36530,#36532,#3784,.T.) ;
#44538=EDGE_CURVE('',#36532,#36533,#3785,.T.) ;
#44539=EDGE_CURVE('',#36533,#36534,#3786,.T.) ;
#44540=EDGE_CURVE('',#36534,#36531,#3787,.T.) ;
#44541=EDGE_CURVE('',#36535,#36536,#29948,.T.) ;
#44542=EDGE_CURVE('',#36535,#36537,#3788,.T.) ;
#44543=EDGE_CURVE('',#36537,#36538,#3789,.T.) ;
#44544=EDGE_CURVE('',#36538,#36539,#3790,.T.) ;
#44545=EDGE_CURVE('',#36539,#36536,#3791,.T.) ;
#44546=EDGE_CURVE('',#36540,#36541,#29949,.T.) ;
#44547=EDGE_CURVE('',#36540,#36542,#3792,.T.) ;
#44548=EDGE_CURVE('',#36542,#36543,#3793,.T.) ;
#44549=EDGE_CURVE('',#36543,#36544,#3794,.T.) ;
#44550=EDGE_CURVE('',#36544,#36541,#3795,.T.) ;
#44551=EDGE_CURVE('',#36545,#36546,#29950,.T.) ;
#44552=EDGE_CURVE('',#36545,#36547,#3796,.T.) ;
#44553=EDGE_CURVE('',#36547,#36548,#3797,.T.) ;
#44554=EDGE_CURVE('',#36548,#36549,#3798,.T.) ;
#44555=EDGE_CURVE('',#36549,#36546,#3799,.T.) ;
#44556=EDGE_CURVE('',#36550,#36551,#29951,.T.) ;
#44557=EDGE_CURVE('',#36550,#36552,#3800,.T.) ;
#44558=EDGE_CURVE('',#36552,#36553,#3801,.T.) ;
#44559=EDGE_CURVE('',#36553,#36554,#3802,.T.) ;
#44560=EDGE_CURVE('',#36554,#36551,#3803,.T.) ;
#44561=EDGE_CURVE('',#36555,#36556,#29952,.T.) ;
#44562=EDGE_CURVE('',#36555,#36557,#3804,.T.) ;
#44563=EDGE_CURVE('',#36557,#36558,#3805,.T.) ;
#44564=EDGE_CURVE('',#36558,#36559,#3806,.T.) ;
#44565=EDGE_CURVE('',#36559,#36556,#3807,.T.) ;
#44566=EDGE_CURVE('',#36560,#36561,#29953,.T.) ;
#44567=EDGE_CURVE('',#36560,#36562,#3808,.T.) ;
#44568=EDGE_CURVE('',#36562,#36563,#3809,.T.) ;
#44569=EDGE_CURVE('',#36563,#36564,#3810,.T.) ;
#44570=EDGE_CURVE('',#36564,#36561,#3811,.T.) ;
#44571=EDGE_CURVE('',#36565,#36566,#29954,.T.) ;
#44572=EDGE_CURVE('',#36565,#36567,#3812,.T.) ;
#44573=EDGE_CURVE('',#36567,#36568,#3813,.T.) ;
#44574=EDGE_CURVE('',#36568,#36569,#3814,.T.) ;
#44575=EDGE_CURVE('',#36569,#36566,#3815,.T.) ;
#44576=EDGE_CURVE('',#36570,#36571,#29955,.T.) ;
#44577=EDGE_CURVE('',#36570,#36572,#3816,.T.) ;
#44578=EDGE_CURVE('',#36572,#36573,#3817,.T.) ;
#44579=EDGE_CURVE('',#36573,#36574,#3818,.T.) ;
#44580=EDGE_CURVE('',#36574,#36571,#3819,.T.) ;
#44581=EDGE_CURVE('',#36575,#36576,#29956,.T.) ;
#44582=EDGE_CURVE('',#36575,#36577,#3820,.T.) ;
#44583=EDGE_CURVE('',#36577,#36578,#3821,.T.) ;
#44584=EDGE_CURVE('',#36578,#36579,#3822,.T.) ;
#44585=EDGE_CURVE('',#36579,#36576,#3823,.T.) ;
#44586=EDGE_CURVE('',#36580,#36581,#3824,.T.) ;
#44587=EDGE_CURVE('',#36580,#36582,#29957,.T.) ;
#44588=EDGE_CURVE('',#36582,#36583,#3825,.T.) ;
#44589=EDGE_CURVE('',#36583,#36581,#29958,.T.) ;
#44590=EDGE_CURVE('',#36584,#36585,#3826,.T.) ;
#44591=EDGE_CURVE('',#36584,#36586,#29959,.T.) ;
#44592=EDGE_CURVE('',#36586,#36587,#3827,.T.) ;
#44593=EDGE_CURVE('',#36587,#36585,#29960,.T.) ;
#44594=EDGE_CURVE('',#36588,#36589,#3828,.T.) ;
#44595=EDGE_CURVE('',#36588,#36590,#29961,.T.) ;
#44596=EDGE_CURVE('',#36590,#36591,#3829,.T.) ;
#44597=EDGE_CURVE('',#36591,#36589,#29962,.T.) ;
#44598=EDGE_CURVE('',#36592,#36593,#3830,.T.) ;
#44599=EDGE_CURVE('',#36592,#36594,#29963,.T.) ;
#44600=EDGE_CURVE('',#36594,#36595,#3831,.T.) ;
#44601=EDGE_CURVE('',#36595,#36593,#29964,.T.) ;
#44602=EDGE_CURVE('',#36596,#36597,#3832,.T.) ;
#44603=EDGE_CURVE('',#36596,#36598,#29965,.T.) ;
#44604=EDGE_CURVE('',#36598,#36599,#3833,.T.) ;
#44605=EDGE_CURVE('',#36599,#36597,#29966,.T.) ;
#44606=EDGE_CURVE('',#36600,#36601,#3834,.T.) ;
#44607=EDGE_CURVE('',#36600,#36602,#29967,.T.) ;
#44608=EDGE_CURVE('',#36602,#36603,#3835,.T.) ;
#44609=EDGE_CURVE('',#36603,#36601,#29968,.T.) ;
#44610=EDGE_CURVE('',#36604,#36605,#3836,.T.) ;
#44611=EDGE_CURVE('',#36604,#36606,#29969,.T.) ;
#44612=EDGE_CURVE('',#36606,#36607,#3837,.T.) ;
#44613=EDGE_CURVE('',#36607,#36605,#29970,.T.) ;
#44614=EDGE_CURVE('',#36608,#36609,#3838,.T.) ;
#44615=EDGE_CURVE('',#36608,#36610,#29971,.T.) ;
#44616=EDGE_CURVE('',#36610,#36611,#3839,.T.) ;
#44617=EDGE_CURVE('',#36611,#36609,#29972,.T.) ;
#44618=EDGE_CURVE('',#36612,#36613,#3840,.T.) ;
#44619=EDGE_CURVE('',#36612,#36614,#29973,.T.) ;
#44620=EDGE_CURVE('',#36614,#36615,#3841,.T.) ;
#44621=EDGE_CURVE('',#36615,#36613,#29974,.T.) ;
#44622=EDGE_CURVE('',#36616,#36617,#3842,.T.) ;
#44623=EDGE_CURVE('',#36617,#36618,#29975,.T.) ;
#44624=EDGE_CURVE('',#36618,#36619,#3843,.T.) ;
#44625=EDGE_CURVE('',#36619,#36396,#29976,.T.) ;
#44626=EDGE_CURVE('',#36620,#36395,#29977,.T.) ;
#44627=EDGE_CURVE('',#36620,#36621,#3844,.T.) ;
#44628=EDGE_CURVE('',#36621,#36622,#3845,.T.) ;
#44629=EDGE_CURVE('',#36622,#36623,#3846,.T.) ;
#44630=EDGE_CURVE('',#36623,#36624,#3847,.T.) ;
#44631=EDGE_CURVE('',#36624,#36625,#3848,.T.) ;
#44632=EDGE_CURVE('',#36616,#36625,#29978,.T.) ;
#44633=EDGE_CURVE('',#36626,#36627,#29979,.T.) ;
#44634=EDGE_CURVE('',#36626,#36628,#3849,.T.) ;
#44635=EDGE_CURVE('',#36628,#36629,#3850,.T.) ;
#44636=EDGE_CURVE('',#36629,#36630,#3851,.T.) ;
#44637=EDGE_CURVE('',#36630,#36627,#3852,.T.) ;
#44638=EDGE_CURVE('',#36631,#36632,#29980,.T.) ;
#44639=EDGE_CURVE('',#36631,#36633,#3853,.T.) ;
#44640=EDGE_CURVE('',#36633,#36634,#3854,.T.) ;
#44641=EDGE_CURVE('',#36634,#36635,#3855,.T.) ;
#44642=EDGE_CURVE('',#36635,#36632,#3856,.T.) ;
#44643=EDGE_CURVE('',#36636,#36637,#3857,.T.) ;
#44644=EDGE_CURVE('',#36636,#36638,#29981,.T.) ;
#44645=EDGE_CURVE('',#36638,#36639,#3858,.T.) ;
#44646=EDGE_CURVE('',#36639,#36637,#29982,.T.) ;
#44647=EDGE_CURVE('',#36640,#36641,#3859,.T.) ;
#44648=EDGE_CURVE('',#36640,#36642,#29983,.T.) ;
#44649=EDGE_CURVE('',#36642,#36643,#3860,.T.) ;
#44650=EDGE_CURVE('',#36643,#36641,#29984,.T.) ;
#44651=EDGE_CURVE('',#36644,#36645,#29985,.T.) ;
#44652=EDGE_CURVE('',#36644,#36646,#3861,.T.) ;
#44653=EDGE_CURVE('',#36647,#36646,#3862,.T.) ;
#44654=EDGE_CURVE('',#36647,#36640,#3863,.T.) ;
#44655=EDGE_CURVE('',#36641,#36639,#3864,.T.) ;
#44656=EDGE_CURVE('',#36638,#36648,#3865,.T.) ;
#44657=EDGE_CURVE('',#36649,#36648,#29986,.T.) ;
#44658=EDGE_CURVE('',#36649,#36650,#3866,.T.) ;
#44659=EDGE_CURVE('',#36651,#36650,#29987,.T.) ;
#44660=EDGE_CURVE('',#36651,#36583,#3867,.T.) ;
#44661=EDGE_CURVE('',#36582,#36652,#3868,.T.) ;
#44662=EDGE_CURVE('',#36653,#36652,#29988,.T.) ;
#44663=EDGE_CURVE('',#36653,#36654,#3869,.T.) ;
#44664=EDGE_CURVE('',#36655,#36654,#29989,.T.) ;
#44665=EDGE_CURVE('',#36655,#36587,#3870,.T.) ;
#44666=EDGE_CURVE('',#36586,#36656,#3871,.T.) ;
#44667=EDGE_CURVE('',#36657,#36656,#29990,.T.) ;
#44668=EDGE_CURVE('',#36657,#36658,#3872,.T.) ;
#44669=EDGE_CURVE('',#36659,#36658,#29991,.T.) ;
#44670=EDGE_CURVE('',#36659,#36591,#3873,.T.) ;
#44671=EDGE_CURVE('',#36590,#36660,#3874,.T.) ;
#44672=EDGE_CURVE('',#36661,#36660,#29992,.T.) ;
#44673=EDGE_CURVE('',#36661,#36662,#3875,.T.) ;
#44674=EDGE_CURVE('',#36663,#36662,#29993,.T.) ;
#44675=EDGE_CURVE('',#36663,#36595,#3876,.T.) ;
#44676=EDGE_CURVE('',#36594,#36664,#3877,.T.) ;
#44677=EDGE_CURVE('',#36665,#36664,#29994,.T.) ;
#44678=EDGE_CURVE('',#36665,#36666,#3878,.T.) ;
#44679=EDGE_CURVE('',#36667,#36666,#29995,.T.) ;
#44680=EDGE_CURVE('',#36667,#36599,#3879,.T.) ;
#44681=EDGE_CURVE('',#36598,#36668,#3880,.T.) ;
#44682=EDGE_CURVE('',#36669,#36668,#29996,.T.) ;
#44683=EDGE_CURVE('',#36669,#36670,#3881,.T.) ;
#44684=EDGE_CURVE('',#36671,#36670,#29997,.T.) ;
#44685=EDGE_CURVE('',#36671,#36603,#3882,.T.) ;
#44686=EDGE_CURVE('',#36602,#36672,#3883,.T.) ;
#44687=EDGE_CURVE('',#36673,#36672,#29998,.T.) ;
#44688=EDGE_CURVE('',#36673,#36674,#3884,.T.) ;
#44689=EDGE_CURVE('',#36675,#36674,#29999,.T.) ;
#44690=EDGE_CURVE('',#36675,#36607,#3885,.T.) ;
#44691=EDGE_CURVE('',#36606,#36676,#3886,.T.) ;
#44692=EDGE_CURVE('',#36677,#36676,#30000,.T.) ;
#44693=EDGE_CURVE('',#36677,#36678,#3887,.T.) ;
#44694=EDGE_CURVE('',#36679,#36678,#30001,.T.) ;
#44695=EDGE_CURVE('',#36679,#36611,#3888,.T.) ;
#44696=EDGE_CURVE('',#36610,#36680,#3889,.T.) ;
#44697=EDGE_CURVE('',#36681,#36680,#30002,.T.) ;
#44698=EDGE_CURVE('',#36681,#36682,#3890,.T.) ;
#44699=EDGE_CURVE('',#36683,#36682,#30003,.T.) ;
#44700=EDGE_CURVE('',#36683,#36615,#3891,.T.) ;
#44701=EDGE_CURVE('',#36614,#36684,#3892,.T.) ;
#44702=EDGE_CURVE('',#36685,#36684,#30004,.T.) ;
#44703=EDGE_CURVE('',#36685,#36645,#3893,.T.) ;
#44704=EDGE_CURVE('',#36646,#36686,#30005,.T.) ;
#44705=EDGE_CURVE('',#36687,#36686,#3894,.T.) ;
#44706=EDGE_CURVE('',#36687,#36647,#30006,.T.) ;
#44707=EDGE_CURVE('',#36688,#36689,#30007,.T.) ;
#44708=EDGE_CURVE('',#36688,#36612,#3895,.T.) ;
#44709=EDGE_CURVE('',#36613,#36690,#3896,.T.) ;
#44710=EDGE_CURVE('',#36691,#36690,#30008,.T.) ;
#44711=EDGE_CURVE('',#36691,#36692,#3897,.T.) ;
#44712=EDGE_CURVE('',#36693,#36692,#30009,.T.) ;
#44713=EDGE_CURVE('',#36693,#36608,#3898,.T.) ;
#44714=EDGE_CURVE('',#36609,#36694,#3899,.T.) ;
#44715=EDGE_CURVE('',#36695,#36694,#30010,.T.) ;
#44716=EDGE_CURVE('',#36695,#36696,#3900,.T.) ;
#44717=EDGE_CURVE('',#36697,#36696,#30011,.T.) ;
#44718=EDGE_CURVE('',#36697,#36604,#3901,.T.) ;
#44719=EDGE_CURVE('',#36605,#36698,#3902,.T.) ;
#44720=EDGE_CURVE('',#36699,#36698,#30012,.T.) ;
#44721=EDGE_CURVE('',#36699,#36700,#3903,.T.) ;
#44722=EDGE_CURVE('',#36701,#36700,#30013,.T.) ;
#44723=EDGE_CURVE('',#36701,#36600,#3904,.T.) ;
#44724=EDGE_CURVE('',#36601,#36702,#3905,.T.) ;
#44725=EDGE_CURVE('',#36703,#36702,#30014,.T.) ;
#44726=EDGE_CURVE('',#36703,#36704,#3906,.T.) ;
#44727=EDGE_CURVE('',#36705,#36704,#30015,.T.) ;
#44728=EDGE_CURVE('',#36705,#36596,#3907,.T.) ;
#44729=EDGE_CURVE('',#36597,#36706,#3908,.T.) ;
#44730=EDGE_CURVE('',#36707,#36706,#30016,.T.) ;
#44731=EDGE_CURVE('',#36707,#36708,#3909,.T.) ;
#44732=EDGE_CURVE('',#36709,#36708,#30017,.T.) ;
#44733=EDGE_CURVE('',#36709,#36592,#3910,.T.) ;
#44734=EDGE_CURVE('',#36593,#36710,#3911,.T.) ;
#44735=EDGE_CURVE('',#36711,#36710,#30018,.T.) ;
#44736=EDGE_CURVE('',#36711,#36712,#3912,.T.) ;
#44737=EDGE_CURVE('',#36713,#36712,#30019,.T.) ;
#44738=EDGE_CURVE('',#36713,#36588,#3913,.T.) ;
#44739=EDGE_CURVE('',#36589,#36714,#3914,.T.) ;
#44740=EDGE_CURVE('',#36715,#36714,#30020,.T.) ;
#44741=EDGE_CURVE('',#36715,#36716,#3915,.T.) ;
#44742=EDGE_CURVE('',#36717,#36716,#30021,.T.) ;
#44743=EDGE_CURVE('',#36717,#36584,#3916,.T.) ;
#44744=EDGE_CURVE('',#36585,#36718,#3917,.T.) ;
#44745=EDGE_CURVE('',#36719,#36718,#30022,.T.) ;
#44746=EDGE_CURVE('',#36719,#36720,#3918,.T.) ;
#44747=EDGE_CURVE('',#36721,#36720,#30023,.T.) ;
#44748=EDGE_CURVE('',#36721,#36580,#3919,.T.) ;
#44749=EDGE_CURVE('',#36581,#36722,#3920,.T.) ;
#44750=EDGE_CURVE('',#36723,#36722,#30024,.T.) ;
#44751=EDGE_CURVE('',#36723,#36724,#3921,.T.) ;
#44752=EDGE_CURVE('',#36725,#36724,#30025,.T.) ;
#44753=EDGE_CURVE('',#36725,#36636,#3922,.T.) ;
#44754=EDGE_CURVE('',#36637,#36726,#3923,.T.) ;
#44755=EDGE_CURVE('',#36727,#36726,#3924,.T.) ;
#44756=EDGE_CURVE('',#36727,#36687,#3925,.T.) ;
#44757=EDGE_CURVE('',#36686,#36728,#3926,.T.) ;
#44758=EDGE_CURVE('',#36729,#36728,#30026,.T.) ;
#44759=EDGE_CURVE('',#36729,#36689,#3927,.T.) ;
#44760=EDGE_CURVE('',#36730,#36731,#3928,.T.) ;
#44761=EDGE_CURVE('',#36730,#36727,#30027,.T.) ;
#44762=EDGE_CURVE('',#36726,#36731,#30028,.T.) ;
#44763=EDGE_CURVE('',#36732,#36733,#3929,.T.) ;
#44764=EDGE_CURVE('',#36732,#36730,#3930,.T.) ;
#44765=EDGE_CURVE('',#36731,#36733,#3931,.T.) ;
#44766=EDGE_CURVE('',#36734,#36735,#3932,.T.) ;
#44767=EDGE_CURVE('',#36734,#36732,#30029,.T.) ;
#44768=EDGE_CURVE('',#36733,#36735,#30030,.T.) ;
#44769=EDGE_CURVE('',#36736,#36737,#3933,.T.) ;
#44770=EDGE_CURVE('',#36736,#36734,#3934,.T.) ;
#44771=EDGE_CURVE('',#36735,#36737,#3935,.T.) ;
#44772=EDGE_CURVE('',#36738,#36739,#3936,.T.) ;
#44773=EDGE_CURVE('',#36738,#36736,#30031,.T.) ;
#44774=EDGE_CURVE('',#36737,#36739,#30032,.T.) ;
#44775=EDGE_CURVE('',#36740,#36741,#3937,.T.) ;
#44776=EDGE_CURVE('',#36740,#36738,#3938,.T.) ;
#44777=EDGE_CURVE('',#36739,#36741,#3939,.T.) ;
#44778=EDGE_CURVE('',#36742,#36743,#3940,.T.) ;
#44779=EDGE_CURVE('',#36742,#36740,#30033,.T.) ;
#44780=EDGE_CURVE('',#36741,#36743,#30034,.T.) ;
#44781=EDGE_CURVE('',#36744,#36745,#3941,.T.) ;
#44782=EDGE_CURVE('',#36744,#36742,#3942,.T.) ;
#44783=EDGE_CURVE('',#36743,#36745,#3943,.T.) ;
#44784=EDGE_CURVE('',#36746,#36747,#3944,.T.) ;
#44785=EDGE_CURVE('',#36746,#36744,#30035,.T.) ;
#44786=EDGE_CURVE('',#36745,#36747,#30036,.T.) ;
#44787=EDGE_CURVE('',#36748,#36749,#3945,.T.) ;
#44788=EDGE_CURVE('',#36748,#36746,#3946,.T.) ;
#44789=EDGE_CURVE('',#36747,#36749,#3947,.T.) ;
#44790=EDGE_CURVE('',#36750,#36751,#3948,.T.) ;
#44791=EDGE_CURVE('',#36750,#36748,#30037,.T.) ;
#44792=EDGE_CURVE('',#36749,#36751,#30038,.T.) ;
#44793=EDGE_CURVE('',#36642,#36750,#3949,.T.) ;
#44794=EDGE_CURVE('',#36751,#36643,#3950,.T.) ;
#44795=EDGE_CURVE('',#36752,#36753,#30039,.T.) ;
#44796=EDGE_CURVE('',#36753,#36754,#3951,.T.) ;
#44797=EDGE_CURVE('',#36754,#36755,#3952,.T.) ;
#44798=EDGE_CURVE('',#36755,#36756,#3953,.T.) ;
#44799=EDGE_CURVE('',#36756,#36757,#30040,.T.) ;
#44800=EDGE_CURVE('',#36757,#36758,#3954,.T.) ;
#44801=EDGE_CURVE('',#36758,#36759,#30041,.T.) ;
#44802=EDGE_CURVE('',#36759,#36345,#3955,.T.) ;
#44803=EDGE_CURVE('',#36346,#36760,#3956,.T.) ;
#44804=EDGE_CURVE('',#36760,#36761,#30042,.T.) ;
#44805=EDGE_CURVE('',#36761,#36762,#3957,.T.) ;
#44806=EDGE_CURVE('',#36762,#36763,#3958,.T.) ;
#44807=EDGE_CURVE('',#36763,#36764,#3959,.T.) ;
#44808=EDGE_CURVE('',#36764,#36765,#30043,.T.) ;
#44809=EDGE_CURVE('',#36765,#36766,#3960,.T.) ;
#44810=EDGE_CURVE('',#36766,#36767,#30044,.T.) ;
#44811=EDGE_CURVE('',#36767,#36768,#3961,.T.) ;
#44812=EDGE_CURVE('',#36768,#36769,#30045,.T.) ;
#44813=EDGE_CURVE('',#36769,#36770,#30046,.T.) ;
#44814=EDGE_CURVE('',#36770,#36771,#30047,.T.) ;
#44815=EDGE_CURVE('',#36771,#36772,#3962,.T.) ;
#44816=EDGE_CURVE('',#36772,#36773,#30048,.T.) ;
#44817=EDGE_CURVE('',#36773,#36752,#3963,.T.) ;
#44818=EDGE_CURVE('',#36774,#36775,#30049,.T.) ;
#44819=EDGE_CURVE('',#36775,#36776,#3964,.T.) ;
#44820=EDGE_CURVE('',#36776,#36777,#3965,.T.) ;
#44821=EDGE_CURVE('',#36777,#36778,#3966,.T.) ;
#44822=EDGE_CURVE('',#36778,#36779,#30050,.T.) ;
#44823=EDGE_CURVE('',#36779,#36780,#3967,.T.) ;
#44824=EDGE_CURVE('',#36780,#36781,#30051,.T.) ;
#44825=EDGE_CURVE('',#36781,#36341,#3968,.T.) ;
#44826=EDGE_CURVE('',#36342,#36782,#3969,.T.) ;
#44827=EDGE_CURVE('',#36782,#36783,#30052,.T.) ;
#44828=EDGE_CURVE('',#36783,#36784,#3970,.T.) ;
#44829=EDGE_CURVE('',#36784,#36785,#3971,.T.) ;
#44830=EDGE_CURVE('',#36785,#36786,#3972,.T.) ;
#44831=EDGE_CURVE('',#36786,#36787,#30053,.T.) ;
#44832=EDGE_CURVE('',#36787,#36788,#3973,.T.) ;
#44833=EDGE_CURVE('',#36788,#36789,#30054,.T.) ;
#44834=EDGE_CURVE('',#36789,#36790,#3974,.T.) ;
#44835=EDGE_CURVE('',#36790,#36791,#30055,.T.) ;
#44836=EDGE_CURVE('',#36791,#36792,#30056,.T.) ;
#44837=EDGE_CURVE('',#36792,#36793,#30057,.T.) ;
#44838=EDGE_CURVE('',#36793,#36794,#3975,.T.) ;
#44839=EDGE_CURVE('',#36794,#36795,#30058,.T.) ;
#44840=EDGE_CURVE('',#36795,#36774,#3976,.T.) ;
#44841=EDGE_CURVE('',#36796,#36797,#30059,.T.) ;
#44842=EDGE_CURVE('',#36797,#36798,#3977,.T.) ;
#44843=EDGE_CURVE('',#36798,#36799,#3978,.T.) ;
#44844=EDGE_CURVE('',#36799,#36800,#3979,.T.) ;
#44845=EDGE_CURVE('',#36800,#36801,#30060,.T.) ;
#44846=EDGE_CURVE('',#36801,#36802,#3980,.T.) ;
#44847=EDGE_CURVE('',#36802,#36803,#30061,.T.) ;
#44848=EDGE_CURVE('',#36803,#36337,#3981,.T.) ;
#44849=EDGE_CURVE('',#36338,#36804,#3982,.T.) ;
#44850=EDGE_CURVE('',#36804,#36805,#30062,.T.) ;
#44851=EDGE_CURVE('',#36805,#36806,#3983,.T.) ;
#44852=EDGE_CURVE('',#36806,#36807,#3984,.T.) ;
#44853=EDGE_CURVE('',#36807,#36808,#3985,.T.) ;
#44854=EDGE_CURVE('',#36808,#36809,#30063,.T.) ;
#44855=EDGE_CURVE('',#36809,#36810,#3986,.T.) ;
#44856=EDGE_CURVE('',#36810,#36811,#30064,.T.) ;
#44857=EDGE_CURVE('',#36811,#36812,#3987,.T.) ;
#44858=EDGE_CURVE('',#36812,#36813,#30065,.T.) ;
#44859=EDGE_CURVE('',#36813,#36814,#30066,.T.) ;
#44860=EDGE_CURVE('',#36814,#36815,#30067,.T.) ;
#44861=EDGE_CURVE('',#36815,#36816,#3988,.T.) ;
#44862=EDGE_CURVE('',#36816,#36817,#30068,.T.) ;
#44863=EDGE_CURVE('',#36817,#36796,#3989,.T.) ;
#44864=EDGE_CURVE('',#36818,#36819,#30069,.T.) ;
#44865=EDGE_CURVE('',#36819,#36820,#3990,.T.) ;
#44866=EDGE_CURVE('',#36820,#36821,#3991,.T.) ;
#44867=EDGE_CURVE('',#36821,#36822,#3992,.T.) ;
#44868=EDGE_CURVE('',#36822,#36823,#30070,.T.) ;
#44869=EDGE_CURVE('',#36823,#36824,#3993,.T.) ;
#44870=EDGE_CURVE('',#36824,#36825,#30071,.T.) ;
#44871=EDGE_CURVE('',#36825,#36333,#3994,.T.) ;
#44872=EDGE_CURVE('',#36334,#36826,#3995,.T.) ;
#44873=EDGE_CURVE('',#36826,#36827,#30072,.T.) ;
#44874=EDGE_CURVE('',#36827,#36828,#3996,.T.) ;
#44875=EDGE_CURVE('',#36828,#36829,#3997,.T.) ;
#44876=EDGE_CURVE('',#36829,#36830,#3998,.T.) ;
#44877=EDGE_CURVE('',#36830,#36831,#30073,.T.) ;
#44878=EDGE_CURVE('',#36831,#36832,#3999,.T.) ;
#44879=EDGE_CURVE('',#36832,#36833,#30074,.T.) ;
#44880=EDGE_CURVE('',#36833,#36834,#4000,.T.) ;
#44881=EDGE_CURVE('',#36834,#36835,#30075,.T.) ;
#44882=EDGE_CURVE('',#36835,#36836,#30076,.T.) ;
#44883=EDGE_CURVE('',#36836,#36837,#30077,.T.) ;
#44884=EDGE_CURVE('',#36837,#36838,#4001,.T.) ;
#44885=EDGE_CURVE('',#36838,#36839,#30078,.T.) ;
#44886=EDGE_CURVE('',#36839,#36818,#4002,.T.) ;
#44887=EDGE_CURVE('',#36840,#36841,#30079,.T.) ;
#44888=EDGE_CURVE('',#36841,#36842,#4003,.T.) ;
#44889=EDGE_CURVE('',#36842,#36843,#4004,.T.) ;
#44890=EDGE_CURVE('',#36843,#36844,#4005,.T.) ;
#44891=EDGE_CURVE('',#36844,#36845,#30080,.T.) ;
#44892=EDGE_CURVE('',#36845,#36846,#4006,.T.) ;
#44893=EDGE_CURVE('',#36846,#36847,#30081,.T.) ;
#44894=EDGE_CURVE('',#36847,#36329,#4007,.T.) ;
#44895=EDGE_CURVE('',#36330,#36848,#4008,.T.) ;
#44896=EDGE_CURVE('',#36848,#36849,#30082,.T.) ;
#44897=EDGE_CURVE('',#36849,#36850,#4009,.T.) ;
#44898=EDGE_CURVE('',#36850,#36851,#4010,.T.) ;
#44899=EDGE_CURVE('',#36851,#36852,#4011,.T.) ;
#44900=EDGE_CURVE('',#36852,#36853,#30083,.T.) ;
#44901=EDGE_CURVE('',#36853,#36854,#4012,.T.) ;
#44902=EDGE_CURVE('',#36854,#36855,#30084,.T.) ;
#44903=EDGE_CURVE('',#36855,#36856,#4013,.T.) ;
#44904=EDGE_CURVE('',#36856,#36857,#30085,.T.) ;
#44905=EDGE_CURVE('',#36857,#36858,#30086,.T.) ;
#44906=EDGE_CURVE('',#36858,#36859,#30087,.T.) ;
#44907=EDGE_CURVE('',#36859,#36860,#4014,.T.) ;
#44908=EDGE_CURVE('',#36860,#36861,#30088,.T.) ;
#44909=EDGE_CURVE('',#36861,#36840,#4015,.T.) ;
#44910=EDGE_CURVE('',#36862,#36863,#30089,.T.) ;
#44911=EDGE_CURVE('',#36863,#36864,#4016,.T.) ;
#44912=EDGE_CURVE('',#36864,#36865,#4017,.T.) ;
#44913=EDGE_CURVE('',#36865,#36866,#4018,.T.) ;
#44914=EDGE_CURVE('',#36866,#36867,#30090,.T.) ;
#44915=EDGE_CURVE('',#36867,#36868,#4019,.T.) ;
#44916=EDGE_CURVE('',#36868,#36869,#30091,.T.) ;
#44917=EDGE_CURVE('',#36869,#36325,#4020,.T.) ;
#44918=EDGE_CURVE('',#36326,#36870,#4021,.T.) ;
#44919=EDGE_CURVE('',#36870,#36871,#30092,.T.) ;
#44920=EDGE_CURVE('',#36871,#36872,#4022,.T.) ;
#44921=EDGE_CURVE('',#36872,#36873,#4023,.T.) ;
#44922=EDGE_CURVE('',#36873,#36874,#4024,.T.) ;
#44923=EDGE_CURVE('',#36874,#36875,#30093,.T.) ;
#44924=EDGE_CURVE('',#36875,#36876,#4025,.T.) ;
#44925=EDGE_CURVE('',#36876,#36877,#30094,.T.) ;
#44926=EDGE_CURVE('',#36877,#36878,#4026,.T.) ;
#44927=EDGE_CURVE('',#36878,#36879,#30095,.T.) ;
#44928=EDGE_CURVE('',#36879,#36880,#30096,.T.) ;
#44929=EDGE_CURVE('',#36880,#36881,#30097,.T.) ;
#44930=EDGE_CURVE('',#36881,#36882,#4027,.T.) ;
#44931=EDGE_CURVE('',#36882,#36883,#30098,.T.) ;
#44932=EDGE_CURVE('',#36883,#36862,#4028,.T.) ;
#44933=EDGE_CURVE('',#36884,#36885,#30099,.T.) ;
#44934=EDGE_CURVE('',#36885,#36886,#4029,.T.) ;
#44935=EDGE_CURVE('',#36886,#36887,#4030,.T.) ;
#44936=EDGE_CURVE('',#36887,#36888,#4031,.T.) ;
#44937=EDGE_CURVE('',#36888,#36889,#30100,.T.) ;
#44938=EDGE_CURVE('',#36889,#36890,#4032,.T.) ;
#44939=EDGE_CURVE('',#36890,#36891,#30101,.T.) ;
#44940=EDGE_CURVE('',#36891,#36321,#4033,.T.) ;
#44941=EDGE_CURVE('',#36322,#36892,#4034,.T.) ;
#44942=EDGE_CURVE('',#36892,#36893,#30102,.T.) ;
#44943=EDGE_CURVE('',#36893,#36894,#4035,.T.) ;
#44944=EDGE_CURVE('',#36894,#36895,#4036,.T.) ;
#44945=EDGE_CURVE('',#36895,#36896,#4037,.T.) ;
#44946=EDGE_CURVE('',#36896,#36897,#30103,.T.) ;
#44947=EDGE_CURVE('',#36897,#36898,#4038,.T.) ;
#44948=EDGE_CURVE('',#36898,#36899,#30104,.T.) ;
#44949=EDGE_CURVE('',#36899,#36900,#4039,.T.) ;
#44950=EDGE_CURVE('',#36900,#36901,#30105,.T.) ;
#44951=EDGE_CURVE('',#36901,#36902,#30106,.T.) ;
#44952=EDGE_CURVE('',#36902,#36903,#30107,.T.) ;
#44953=EDGE_CURVE('',#36903,#36904,#4040,.T.) ;
#44954=EDGE_CURVE('',#36904,#36905,#30108,.T.) ;
#44955=EDGE_CURVE('',#36905,#36884,#4041,.T.) ;
#44956=EDGE_CURVE('',#36906,#36907,#30109,.T.) ;
#44957=EDGE_CURVE('',#36907,#36908,#4042,.T.) ;
#44958=EDGE_CURVE('',#36908,#36909,#4043,.T.) ;
#44959=EDGE_CURVE('',#36909,#36910,#4044,.T.) ;
#44960=EDGE_CURVE('',#36910,#36911,#30110,.T.) ;
#44961=EDGE_CURVE('',#36911,#36912,#4045,.T.) ;
#44962=EDGE_CURVE('',#36912,#36913,#30111,.T.) ;
#44963=EDGE_CURVE('',#36913,#36317,#4046,.T.) ;
#44964=EDGE_CURVE('',#36318,#36914,#4047,.T.) ;
#44965=EDGE_CURVE('',#36914,#36915,#30112,.T.) ;
#44966=EDGE_CURVE('',#36915,#36916,#4048,.T.) ;
#44967=EDGE_CURVE('',#36916,#36917,#4049,.T.) ;
#44968=EDGE_CURVE('',#36917,#36918,#4050,.T.) ;
#44969=EDGE_CURVE('',#36918,#36919,#30113,.T.) ;
#44970=EDGE_CURVE('',#36919,#36920,#4051,.T.) ;
#44971=EDGE_CURVE('',#36920,#36921,#30114,.T.) ;
#44972=EDGE_CURVE('',#36921,#36922,#4052,.T.) ;
#44973=EDGE_CURVE('',#36922,#36923,#30115,.T.) ;
#44974=EDGE_CURVE('',#36923,#36924,#30116,.T.) ;
#44975=EDGE_CURVE('',#36924,#36925,#30117,.T.) ;
#44976=EDGE_CURVE('',#36925,#36926,#4053,.T.) ;
#44977=EDGE_CURVE('',#36926,#36927,#30118,.T.) ;
#44978=EDGE_CURVE('',#36927,#36906,#4054,.T.) ;
#44979=EDGE_CURVE('',#36928,#36929,#30119,.T.) ;
#44980=EDGE_CURVE('',#36929,#36930,#4055,.T.) ;
#44981=EDGE_CURVE('',#36930,#36931,#4056,.T.) ;
#44982=EDGE_CURVE('',#36931,#36932,#4057,.T.) ;
#44983=EDGE_CURVE('',#36932,#36933,#30120,.T.) ;
#44984=EDGE_CURVE('',#36933,#36934,#4058,.T.) ;
#44985=EDGE_CURVE('',#36934,#36935,#30121,.T.) ;
#44986=EDGE_CURVE('',#36935,#36313,#4059,.T.) ;
#44987=EDGE_CURVE('',#36314,#36936,#4060,.T.) ;
#44988=EDGE_CURVE('',#36936,#36937,#30122,.T.) ;
#44989=EDGE_CURVE('',#36937,#36938,#4061,.T.) ;
#44990=EDGE_CURVE('',#36938,#36939,#4062,.T.) ;
#44991=EDGE_CURVE('',#36939,#36940,#4063,.T.) ;
#44992=EDGE_CURVE('',#36940,#36941,#30123,.T.) ;
#44993=EDGE_CURVE('',#36941,#36942,#4064,.T.) ;
#44994=EDGE_CURVE('',#36942,#36943,#30124,.T.) ;
#44995=EDGE_CURVE('',#36943,#36944,#4065,.T.) ;
#44996=EDGE_CURVE('',#36944,#36945,#30125,.T.) ;
#44997=EDGE_CURVE('',#36945,#36946,#30126,.T.) ;
#44998=EDGE_CURVE('',#36946,#36947,#30127,.T.) ;
#44999=EDGE_CURVE('',#36947,#36948,#4066,.T.) ;
#45000=EDGE_CURVE('',#36948,#36949,#30128,.T.) ;
#45001=EDGE_CURVE('',#36949,#36928,#4067,.T.) ;
#45002=EDGE_CURVE('',#36950,#36951,#30129,.T.) ;
#45003=EDGE_CURVE('',#36951,#36952,#4068,.T.) ;
#45004=EDGE_CURVE('',#36952,#36953,#4069,.T.) ;
#45005=EDGE_CURVE('',#36953,#36954,#4070,.T.) ;
#45006=EDGE_CURVE('',#36954,#36955,#30130,.T.) ;
#45007=EDGE_CURVE('',#36955,#36956,#4071,.T.) ;
#45008=EDGE_CURVE('',#36956,#36957,#30131,.T.) ;
#45009=EDGE_CURVE('',#36957,#36382,#4072,.T.) ;
#45010=EDGE_CURVE('',#36383,#36958,#4073,.T.) ;
#45011=EDGE_CURVE('',#36958,#36959,#30132,.T.) ;
#45012=EDGE_CURVE('',#36959,#36960,#4074,.T.) ;
#45013=EDGE_CURVE('',#36960,#36961,#4075,.T.) ;
#45014=EDGE_CURVE('',#36961,#36962,#4076,.T.) ;
#45015=EDGE_CURVE('',#36962,#36963,#30133,.T.) ;
#45016=EDGE_CURVE('',#36963,#36964,#4077,.T.) ;
#45017=EDGE_CURVE('',#36964,#36965,#30134,.T.) ;
#45018=EDGE_CURVE('',#36965,#36966,#4078,.T.) ;
#45019=EDGE_CURVE('',#36966,#36967,#30135,.T.) ;
#45020=EDGE_CURVE('',#36967,#36968,#30136,.T.) ;
#45021=EDGE_CURVE('',#36968,#36969,#30137,.T.) ;
#45022=EDGE_CURVE('',#36969,#36970,#4079,.T.) ;
#45023=EDGE_CURVE('',#36970,#36971,#30138,.T.) ;
#45024=EDGE_CURVE('',#36971,#36950,#4080,.T.) ;
#45025=EDGE_CURVE('',#36972,#36973,#4081,.T.) ;
#45026=EDGE_CURVE('',#36973,#36974,#4082,.T.) ;
#45027=EDGE_CURVE('',#36974,#36975,#4083,.T.) ;
#45028=EDGE_CURVE('',#36975,#36976,#4084,.T.) ;
#45029=EDGE_CURVE('',#36976,#36977,#30139,.T.) ;
#45030=EDGE_CURVE('',#36977,#36978,#4085,.T.) ;
#45031=EDGE_CURVE('',#36978,#36979,#4086,.T.) ;
#45032=EDGE_CURVE('',#36979,#36980,#4087,.T.) ;
#45033=EDGE_CURVE('',#36980,#36981,#30140,.T.) ;
#45034=EDGE_CURVE('',#36981,#36972,#4088,.T.) ;
#45035=EDGE_CURVE('',#36982,#36983,#4089,.T.) ;
#45036=EDGE_CURVE('',#36983,#36984,#4090,.T.) ;
#45037=EDGE_CURVE('',#36984,#36985,#4091,.T.) ;
#45038=EDGE_CURVE('',#36985,#36986,#4092,.T.) ;
#45039=EDGE_CURVE('',#36986,#36987,#30141,.T.) ;
#45040=EDGE_CURVE('',#36987,#36988,#4093,.T.) ;
#45041=EDGE_CURVE('',#36988,#36989,#4094,.T.) ;
#45042=EDGE_CURVE('',#36989,#36990,#4095,.T.) ;
#45043=EDGE_CURVE('',#36990,#36991,#30142,.T.) ;
#45044=EDGE_CURVE('',#36991,#36982,#4096,.T.) ;
#45045=EDGE_CURVE('',#36992,#36993,#4097,.T.) ;
#45046=EDGE_CURVE('',#36993,#36994,#4098,.T.) ;
#45047=EDGE_CURVE('',#36994,#36995,#4099,.T.) ;
#45048=EDGE_CURVE('',#36995,#36996,#4100,.T.) ;
#45049=EDGE_CURVE('',#36996,#36997,#4101,.T.) ;
#45050=EDGE_CURVE('',#36997,#36998,#4102,.T.) ;
#45051=EDGE_CURVE('',#36999,#36998,#30143,.T.) ;
#45052=EDGE_CURVE('',#36999,#37000,#4103,.T.) ;
#45053=EDGE_CURVE('',#37001,#37000,#30144,.T.) ;
#45054=EDGE_CURVE('',#37001,#36992,#4104,.T.) ;
#45055=EDGE_CURVE('',#37002,#37003,#4105,.T.) ;
#45056=EDGE_CURVE('',#37003,#37004,#4106,.T.) ;
#45057=EDGE_CURVE('',#37004,#37005,#4107,.T.) ;
#45058=EDGE_CURVE('',#37005,#37002,#4108,.T.) ;
#45059=EDGE_CURVE('',#36393,#37006,#4109,.T.) ;
#45060=EDGE_CURVE('',#37006,#37007,#4110,.T.) ;
#45061=EDGE_CURVE('',#37007,#36394,#4111,.T.) ;
#45062=EDGE_CURVE('',#37008,#37009,#4112,.T.) ;
#45063=EDGE_CURVE('',#37009,#37010,#4113,.T.) ;
#45064=EDGE_CURVE('',#37010,#37011,#4114,.T.) ;
#45065=EDGE_CURVE('',#37011,#37008,#4115,.T.) ;
#45066=EDGE_CURVE('',#37012,#37013,#4116,.T.) ;
#45067=EDGE_CURVE('',#37013,#37014,#4117,.T.) ;
#45068=EDGE_CURVE('',#37014,#37015,#4118,.T.) ;
#45069=EDGE_CURVE('',#37015,#37012,#4119,.T.) ;
#45070=EDGE_CURVE('',#37016,#37017,#4120,.T.) ;
#45071=EDGE_CURVE('',#37017,#37018,#4121,.T.) ;
#45072=EDGE_CURVE('',#37018,#37019,#4122,.T.) ;
#45073=EDGE_CURVE('',#37019,#37016,#4123,.T.) ;
#45074=EDGE_CURVE('',#37020,#37021,#4124,.T.) ;
#45075=EDGE_CURVE('',#37020,#37022,#30145,.T.) ;
#45076=EDGE_CURVE('',#37022,#37023,#4125,.T.) ;
#45077=EDGE_CURVE('',#37023,#37021,#30146,.T.) ;
#45078=EDGE_CURVE('',#37022,#37024,#4126,.T.) ;
#45079=EDGE_CURVE('',#37024,#37025,#4127,.T.) ;
#45080=EDGE_CURVE('',#37025,#37023,#4128,.T.) ;
#45081=EDGE_CURVE('',#37024,#37026,#30147,.T.) ;
#45082=EDGE_CURVE('',#37026,#37027,#4129,.T.) ;
#45083=EDGE_CURVE('',#37027,#37025,#30148,.T.) ;
#45084=EDGE_CURVE('',#37026,#37028,#4130,.T.) ;
#45085=EDGE_CURVE('',#37028,#37029,#4131,.T.) ;
#45086=EDGE_CURVE('',#37029,#37027,#4132,.T.) ;
#45087=EDGE_CURVE('',#37028,#37030,#30149,.T.) ;
#45088=EDGE_CURVE('',#37030,#37031,#4133,.T.) ;
#45089=EDGE_CURVE('',#37031,#37029,#30150,.T.) ;
#45090=EDGE_CURVE('',#37030,#36388,#4134,.T.) ;
#45091=EDGE_CURVE('',#36388,#37032,#4135,.T.) ;
#45092=EDGE_CURVE('',#37032,#37031,#4136,.T.) ;
#45093=EDGE_CURVE('',#36389,#37033,#4137,.T.) ;
#45094=EDGE_CURVE('',#37033,#37032,#30151,.T.) ;
#45095=EDGE_CURVE('',#36389,#36398,#4138,.T.) ;
#45096=EDGE_CURVE('',#36384,#37033,#4139,.T.) ;
#45097=EDGE_CURVE('',#36399,#37034,#4140,.T.) ;
#45098=EDGE_CURVE('',#37034,#37035,#4141,.T.) ;
#45099=EDGE_CURVE('',#37035,#36385,#4142,.T.) ;
#45100=EDGE_CURVE('',#37034,#37036,#30152,.T.) ;
#45101=EDGE_CURVE('',#37036,#37037,#4143,.T.) ;
#45102=EDGE_CURVE('',#37037,#37035,#30153,.T.) ;
#45103=EDGE_CURVE('',#37036,#37038,#4144,.T.) ;
#45104=EDGE_CURVE('',#37038,#37039,#4145,.T.) ;
#45105=EDGE_CURVE('',#37039,#37037,#4146,.T.) ;
#45106=EDGE_CURVE('',#37038,#37040,#30154,.T.) ;
#45107=EDGE_CURVE('',#37040,#37041,#4147,.T.) ;
#45108=EDGE_CURVE('',#37041,#37039,#30155,.T.) ;
#45109=EDGE_CURVE('',#37040,#37042,#4148,.T.) ;
#45110=EDGE_CURVE('',#37042,#37043,#4149,.T.) ;
#45111=EDGE_CURVE('',#37043,#37041,#4150,.T.) ;
#45112=EDGE_CURVE('',#37042,#37044,#30156,.T.) ;
#45113=EDGE_CURVE('',#37044,#37045,#4151,.T.) ;
#45114=EDGE_CURVE('',#37045,#37043,#30157,.T.) ;
#45115=EDGE_CURVE('',#37044,#37046,#4152,.T.) ;
#45116=EDGE_CURVE('',#37046,#37047,#4153,.T.) ;
#45117=EDGE_CURVE('',#37047,#37045,#4154,.T.) ;
#45118=EDGE_CURVE('',#37046,#37048,#30158,.T.) ;
#45119=EDGE_CURVE('',#37048,#37049,#4155,.T.) ;
#45120=EDGE_CURVE('',#37049,#37047,#30159,.T.) ;
#45121=EDGE_CURVE('',#37048,#37050,#4156,.T.) ;
#45122=EDGE_CURVE('',#37050,#37051,#4157,.T.) ;
#45123=EDGE_CURVE('',#37051,#37049,#4158,.T.) ;
#45124=EDGE_CURVE('',#37050,#37052,#30160,.T.) ;
#45125=EDGE_CURVE('',#37052,#37053,#4159,.T.) ;
#45126=EDGE_CURVE('',#37053,#37051,#30161,.T.) ;
#45127=EDGE_CURVE('',#37052,#37054,#4160,.T.) ;
#45128=EDGE_CURVE('',#37054,#37055,#4161,.T.) ;
#45129=EDGE_CURVE('',#37055,#37053,#4162,.T.) ;
#45130=EDGE_CURVE('',#37054,#37056,#30162,.T.) ;
#45131=EDGE_CURVE('',#37056,#37057,#4163,.T.) ;
#45132=EDGE_CURVE('',#37057,#37055,#30163,.T.) ;
#45133=EDGE_CURVE('',#37056,#37058,#30164,.T.) ;
#45134=EDGE_CURVE('',#37058,#37059,#4164,.T.) ;
#45135=EDGE_CURVE('',#37059,#37057,#30165,.T.) ;
#45136=EDGE_CURVE('',#37058,#37060,#30166,.T.) ;
#45137=EDGE_CURVE('',#37060,#37061,#4165,.T.) ;
#45138=EDGE_CURVE('',#37061,#37059,#30167,.T.) ;
#45139=EDGE_CURVE('',#37060,#37062,#4166,.T.) ;
#45140=EDGE_CURVE('',#37062,#37063,#4167,.T.) ;
#45141=EDGE_CURVE('',#37063,#37061,#4168,.T.) ;
#45142=EDGE_CURVE('',#37062,#37064,#30168,.T.) ;
#45143=EDGE_CURVE('',#37064,#37065,#4169,.T.) ;
#45144=EDGE_CURVE('',#37065,#37063,#30169,.T.) ;
#45145=EDGE_CURVE('',#37064,#37066,#4170,.T.) ;
#45146=EDGE_CURVE('',#37066,#37067,#4171,.T.) ;
#45147=EDGE_CURVE('',#37067,#37065,#4172,.T.) ;
#45148=EDGE_CURVE('',#37066,#37068,#30170,.T.) ;
#45149=EDGE_CURVE('',#37068,#37069,#4173,.T.) ;
#45150=EDGE_CURVE('',#37069,#37067,#30171,.T.) ;
#45151=EDGE_CURVE('',#37068,#37020,#4174,.T.) ;
#45152=EDGE_CURVE('',#37021,#37069,#4175,.T.) ;
#45153=EDGE_CURVE('',#37070,#37071,#30172,.T.) ;
#45154=EDGE_CURVE('',#37071,#37072,#4176,.T.) ;
#45155=EDGE_CURVE('',#37072,#37073,#30173,.T.) ;
#45156=EDGE_CURVE('',#37073,#37074,#4177,.T.) ;
#45157=EDGE_CURVE('',#37074,#37075,#4178,.T.) ;
#45158=EDGE_CURVE('',#37075,#37076,#4179,.T.) ;
#45159=EDGE_CURVE('',#37076,#37077,#30174,.T.) ;
#45160=EDGE_CURVE('',#37077,#37078,#4180,.T.) ;
#45161=EDGE_CURVE('',#37078,#37079,#4181,.T.) ;
#45162=EDGE_CURVE('',#37079,#37080,#4182,.T.) ;
#45163=EDGE_CURVE('',#37080,#37081,#30175,.T.) ;
#45164=EDGE_CURVE('',#37081,#37082,#4183,.T.) ;
#45165=EDGE_CURVE('',#37082,#37083,#30176,.T.) ;
#45166=EDGE_CURVE('',#37083,#37084,#4184,.T.) ;
#45167=EDGE_CURVE('',#37084,#37085,#4185,.T.) ;
#45168=EDGE_CURVE('',#37085,#36390,#4186,.T.) ;
#45169=EDGE_CURVE('',#36390,#37086,#4187,.T.) ;
#45170=EDGE_CURVE('',#37086,#37070,#4188,.T.) ;
#45171=EDGE_CURVE('',#37087,#37088,#4189,.T.) ;
#45172=EDGE_CURVE('',#37087,#37089,#30177,.T.) ;
#45173=EDGE_CURVE('',#37089,#37090,#4190,.T.) ;
#45174=EDGE_CURVE('',#37090,#37091,#30178,.T.) ;
#45175=EDGE_CURVE('',#37091,#37092,#4191,.T.) ;
#45176=EDGE_CURVE('',#37092,#37093,#30179,.T.) ;
#45177=EDGE_CURVE('',#37093,#37094,#4192,.T.) ;
#45178=EDGE_CURVE('',#37094,#37088,#30180,.T.) ;
#45179=EDGE_CURVE('',#37014,#37001,#30181,.T.) ;
#45180=EDGE_CURVE('',#36992,#37013,#30182,.T.) ;
#45181=EDGE_CURVE('',#37015,#37008,#30183,.T.) ;
#45182=EDGE_CURVE('',#37009,#37014,#30184,.T.) ;
#45183=EDGE_CURVE('',#37015,#37095,#30185,.T.) ;
#45184=EDGE_CURVE('',#37095,#37008,#30186,.T.) ;
#45185=EDGE_CURVE('',#36992,#37018,#30187,.T.) ;
#45186=EDGE_CURVE('',#37018,#37013,#30188,.T.) ;
#45187=EDGE_CURVE('',#37009,#37000,#30189,.T.) ;
#45188=EDGE_CURVE('',#36391,#37011,#30190,.T.) ;
#45189=EDGE_CURVE('',#36392,#37096,#2167,.T.) ;
#45190=EDGE_CURVE('',#37095,#37096,#4193,.T.) ;
#45191=EDGE_CURVE('',#37097,#37095,#2168,.T.) ;
#45192=EDGE_CURVE('',#37097,#37098,#2169,.T.) ;
#45193=EDGE_CURVE('',#36617,#37098,#4194,.T.) ;
#45194=EDGE_CURVE('',#37012,#36616,#30191,.T.) ;
#45195=EDGE_CURVE('',#37019,#37012,#30192,.T.) ;
#45196=EDGE_CURVE('',#36993,#37017,#30193,.T.) ;
#45197=EDGE_CURVE('',#37010,#36999,#30194,.T.) ;
#45198=EDGE_CURVE('',#37011,#36393,#30195,.T.) ;
#45199=EDGE_CURVE('',#37006,#37010,#30196,.T.) ;
#45200=EDGE_CURVE('',#37019,#36625,#30197,.T.) ;
#45201=EDGE_CURVE('',#36993,#36632,#30198,.T.) ;
#45202=EDGE_CURVE('',#36631,#37017,#30199,.T.) ;
#45203=EDGE_CURVE('',#37006,#36998,#30200,.T.) ;
#45204=EDGE_CURVE('',#37016,#36624,#30201,.T.) ;
#45205=EDGE_CURVE('',#36633,#37016,#30202,.T.) ;
#45206=EDGE_CURVE('',#37099,#36632,#4195,.T.) ;
#45207=EDGE_CURVE('',#36994,#37099,#30203,.T.) ;
#45208=EDGE_CURVE('',#37007,#36997,#30204,.T.) ;
#45209=EDGE_CURVE('',#36394,#37002,#30205,.T.) ;
#45210=EDGE_CURVE('',#37003,#37007,#30206,.T.) ;
#45211=EDGE_CURVE('',#36620,#37002,#30207,.T.) ;
#45212=EDGE_CURVE('',#36633,#36624,#30208,.T.) ;
#45213=EDGE_CURVE('',#36638,#36635,#30209,.T.) ;
#45214=EDGE_CURVE('',#36635,#36636,#30210,.T.) ;
#45215=EDGE_CURVE('',#37099,#36725,#30211,.T.) ;
#45216=EDGE_CURVE('',#37100,#37099,#30212,.T.) ;
#45217=EDGE_CURVE('',#36994,#37100,#30213,.T.) ;
#45218=EDGE_CURVE('',#37003,#36997,#30214,.T.) ;
#45219=EDGE_CURVE('',#36621,#37005,#30215,.T.) ;
#45220=EDGE_CURVE('',#36634,#36623,#30216,.T.) ;
#45221=EDGE_CURVE('',#36648,#36634,#30217,.T.) ;
#45222=EDGE_CURVE('',#37100,#36724,#30218,.T.) ;
#45223=EDGE_CURVE('',#37101,#37100,#4196,.T.) ;
#45224=EDGE_CURVE('',#36995,#37101,#30219,.T.) ;
#45225=EDGE_CURVE('',#37004,#36996,#30220,.T.) ;
#45226=EDGE_CURVE('',#37005,#36630,#30221,.T.) ;
#45227=EDGE_CURVE('',#36627,#37004,#30222,.T.) ;
#45228=EDGE_CURVE('',#36621,#36630,#30223,.T.) ;
#45229=EDGE_CURVE('',#36649,#36623,#30224,.T.) ;
#45230=EDGE_CURVE('',#37101,#36723,#30225,.T.) ;
#45231=EDGE_CURVE('',#37102,#37101,#30226,.T.) ;
#45232=EDGE_CURVE('',#36995,#37102,#30227,.T.) ;
#45233=EDGE_CURVE('',#36626,#36996,#30228,.T.) ;
#45234=EDGE_CURVE('',#36622,#36629,#30229,.T.) ;
#45235=EDGE_CURVE('',#36650,#36622,#30230,.T.) ;
#45236=EDGE_CURVE('',#37102,#36722,#30231,.T.) ;
#45237=EDGE_CURVE('',#36626,#37102,#4197,.T.) ;
#45238=EDGE_CURVE('',#36651,#36629,#30232,.T.) ;
#45239=EDGE_CURVE('',#36628,#36581,#30233,.T.) ;
#45240=EDGE_CURVE('',#36583,#36628,#30234,.T.) ;
#45241=EDGE_CURVE('',#36978,#36738,#30235,.T.) ;
#45242=EDGE_CURVE('',#36736,#36978,#30236,.T.) ;
#45243=EDGE_CURVE('',#36734,#36977,#30237,.T.) ;
#45244=EDGE_CURVE('',#36979,#36740,#30238,.T.) ;
#45245=EDGE_CURVE('',#36732,#36976,#30239,.T.) ;
#45246=EDGE_CURVE('',#36979,#36742,#30240,.T.) ;
#45247=EDGE_CURVE('',#36730,#36975,#30241,.T.) ;
#45248=EDGE_CURVE('',#36980,#36744,#30242,.T.) ;
#45249=EDGE_CURVE('',#36727,#36975,#30243,.T.) ;
#45250=EDGE_CURVE('',#36981,#36746,#30244,.T.) ;
#45251=EDGE_CURVE('',#36687,#36974,#30245,.T.) ;
#45252=EDGE_CURVE('',#36972,#36748,#30246,.T.) ;
#45253=EDGE_CURVE('',#36647,#36974,#30247,.T.) ;
#45254=EDGE_CURVE('',#36972,#36750,#30248,.T.) ;
#45255=EDGE_CURVE('',#36640,#36973,#30249,.T.) ;
#45256=EDGE_CURVE('',#36973,#36642,#30250,.T.) ;
#45257=EDGE_CURVE('',#36739,#36989,#30251,.T.) ;
#45258=EDGE_CURVE('',#36989,#36737,#30252,.T.) ;
#45259=EDGE_CURVE('',#36990,#36735,#30253,.T.) ;
#45260=EDGE_CURVE('',#36741,#36988,#30254,.T.) ;
#45261=EDGE_CURVE('',#36991,#36733,#30255,.T.) ;
#45262=EDGE_CURVE('',#36743,#36988,#30256,.T.) ;
#45263=EDGE_CURVE('',#36982,#36731,#30257,.T.) ;
#45264=EDGE_CURVE('',#36745,#36987,#30258,.T.) ;
#45265=EDGE_CURVE('',#36982,#36726,#30259,.T.) ;
#45266=EDGE_CURVE('',#36747,#36986,#30260,.T.) ;
#45267=EDGE_CURVE('',#36983,#36637,#30261,.T.) ;
#45268=EDGE_CURVE('',#36749,#36985,#30262,.T.) ;
#45269=EDGE_CURVE('',#36983,#36639,#30263,.T.) ;
#45270=EDGE_CURVE('',#36751,#36985,#30264,.T.) ;
#45271=EDGE_CURVE('',#36984,#36641,#30265,.T.) ;
#45272=EDGE_CURVE('',#36643,#36984,#30266,.T.) ;
#45273=EDGE_CURVE('',#37046,#37079,#30267,.T.) ;
#45274=EDGE_CURVE('',#37080,#37044,#30268,.T.) ;
#45275=EDGE_CURVE('',#37081,#37042,#30269,.T.) ;
#45276=EDGE_CURVE('',#37048,#37079,#30270,.T.) ;
#45277=EDGE_CURVE('',#37082,#37040,#30271,.T.) ;
#45278=EDGE_CURVE('',#37050,#37078,#30272,.T.) ;
#45279=EDGE_CURVE('',#37083,#37038,#30273,.T.) ;
#45280=EDGE_CURVE('',#37052,#37078,#30274,.T.) ;
#45281=EDGE_CURVE('',#37084,#37036,#30275,.T.) ;
#45282=EDGE_CURVE('',#37054,#37077,#30276,.T.) ;
#45283=EDGE_CURVE('',#37084,#37034,#30277,.T.) ;
#45284=EDGE_CURVE('',#37056,#37077,#30278,.T.) ;
#45285=EDGE_CURVE('',#37085,#36399,#30279,.T.) ;
#45286=EDGE_CURVE('',#37058,#37076,#30280,.T.) ;
#45287=EDGE_CURVE('',#37085,#36398,#30281,.T.) ;
#45288=EDGE_CURVE('',#37060,#37076,#30282,.T.) ;
#45289=EDGE_CURVE('',#37062,#37075,#30283,.T.) ;
#45290=EDGE_CURVE('',#37064,#37075,#30284,.T.) ;
#45291=EDGE_CURVE('',#37086,#37030,#30285,.T.) ;
#45292=EDGE_CURVE('',#37066,#37074,#30286,.T.) ;
#45293=EDGE_CURVE('',#37086,#37028,#30287,.T.) ;
#45294=EDGE_CURVE('',#37068,#37074,#30288,.T.) ;
#45295=EDGE_CURVE('',#37070,#37026,#30289,.T.) ;
#45296=EDGE_CURVE('',#37020,#37073,#30290,.T.) ;
#45297=EDGE_CURVE('',#37071,#37024,#30291,.T.) ;
#45298=EDGE_CURVE('',#37022,#37072,#30292,.T.) ;
#45299=EDGE_CURVE('',#37041,#36960,#30293,.T.) ;
#45300=EDGE_CURVE('',#36961,#37043,#30294,.T.) ;
#45301=EDGE_CURVE('',#37039,#36960,#30295,.T.) ;
#45302=EDGE_CURVE('',#36961,#37045,#30296,.T.) ;
#45303=EDGE_CURVE('',#37037,#36959,#30297,.T.) ;
#45304=EDGE_CURVE('',#36962,#37047,#30298,.T.) ;
#45305=EDGE_CURVE('',#37035,#36958,#30299,.T.) ;
#45306=EDGE_CURVE('',#36963,#37049,#30300,.T.) ;
#45307=EDGE_CURVE('',#36964,#37051,#30301,.T.) ;
#45308=EDGE_CURVE('',#36965,#37053,#30302,.T.) ;
#45309=EDGE_CURVE('',#37033,#36957,#30303,.T.) ;
#45310=EDGE_CURVE('',#36966,#37055,#30304,.T.) ;
#45311=EDGE_CURVE('',#37032,#36956,#30305,.T.) ;
#45312=EDGE_CURVE('',#36967,#37057,#30306,.T.) ;
#45313=EDGE_CURVE('',#37031,#36955,#30307,.T.) ;
#45314=EDGE_CURVE('',#36968,#37059,#30308,.T.) ;
#45315=EDGE_CURVE('',#37029,#36954,#30309,.T.) ;
#45316=EDGE_CURVE('',#36969,#37061,#30310,.T.) ;
#45317=EDGE_CURVE('',#37027,#36953,#30311,.T.) ;
#45318=EDGE_CURVE('',#36970,#37063,#30312,.T.) ;
#45319=EDGE_CURVE('',#37025,#36953,#30313,.T.) ;
#45320=EDGE_CURVE('',#36971,#37065,#30314,.T.) ;
#45321=EDGE_CURVE('',#37023,#36952,#30315,.T.) ;
#45322=EDGE_CURVE('',#36950,#37067,#30316,.T.) ;
#45323=EDGE_CURVE('',#37021,#36952,#30317,.T.) ;
#45324=EDGE_CURVE('',#36951,#37069,#30318,.T.) ;
#45325=EDGE_CURVE('',#37103,#37104,#4198,.T.) ;
#45326=EDGE_CURVE('',#37104,#37105,#4199,.T.) ;
#45327=EDGE_CURVE('',#37105,#37106,#4200,.T.) ;
#45328=EDGE_CURVE('',#37106,#37103,#4201,.T.) ;
#45329=EDGE_CURVE('',#37107,#37108,#4202,.T.) ;
#45330=EDGE_CURVE('',#37108,#37109,#4203,.T.) ;
#45331=EDGE_CURVE('',#37109,#37110,#4204,.T.) ;
#45332=EDGE_CURVE('',#37110,#37107,#4205,.T.) ;
#45333=EDGE_CURVE('',#37111,#37112,#4206,.T.) ;
#45334=EDGE_CURVE('',#37112,#37113,#4207,.T.) ;
#45335=EDGE_CURVE('',#37113,#37114,#4208,.T.) ;
#45336=EDGE_CURVE('',#37114,#37111,#4209,.T.) ;
#45337=EDGE_CURVE('',#37115,#37116,#4210,.T.) ;
#45338=EDGE_CURVE('',#37116,#37117,#4211,.T.) ;
#45339=EDGE_CURVE('',#37117,#37118,#4212,.T.) ;
#45340=EDGE_CURVE('',#37118,#37115,#4213,.T.) ;
#45341=EDGE_CURVE('',#37119,#37120,#4214,.T.) ;
#45342=EDGE_CURVE('',#37120,#37121,#4215,.T.) ;
#45343=EDGE_CURVE('',#37122,#37121,#4216,.T.) ;
#45344=EDGE_CURVE('',#37122,#37119,#4217,.T.) ;
#45345=EDGE_CURVE('',#37123,#37124,#4218,.T.) ;
#45346=EDGE_CURVE('',#37124,#36617,#30319,.T.) ;
#45347=EDGE_CURVE('',#37098,#37125,#30320,.T.) ;
#45348=EDGE_CURVE('',#37125,#37126,#4219,.T.) ;
#45349=EDGE_CURVE('',#37126,#37123,#4220,.T.) ;
#45350=EDGE_CURVE('',#37127,#37128,#4221,.T.) ;
#45351=EDGE_CURVE('',#37128,#36397,#30321,.T.) ;
#45352=EDGE_CURVE('',#36396,#37129,#30322,.T.) ;
#45353=EDGE_CURVE('',#37129,#37130,#4222,.T.) ;
#45354=EDGE_CURVE('',#37130,#37127,#4223,.T.) ;
#45355=EDGE_CURVE('',#37096,#37104,#30323,.T.) ;
#45356=EDGE_CURVE('',#37103,#37097,#30324,.T.) ;
#45357=EDGE_CURVE('',#37121,#36619,#30325,.T.) ;
#45358=EDGE_CURVE('',#36618,#37122,#30326,.T.) ;
#45359=EDGE_CURVE('',#37131,#37132,#4224,.T.) ;
#45360=EDGE_CURVE('',#37132,#37133,#4225,.T.) ;
#45361=EDGE_CURVE('',#37133,#37134,#4226,.T.) ;
#45362=EDGE_CURVE('',#37134,#37131,#4227,.T.) ;
#45363=EDGE_CURVE('',#37135,#37136,#4228,.T.) ;
#45364=EDGE_CURVE('',#37136,#37090,#4229,.T.) ;
#45365=EDGE_CURVE('',#37089,#37135,#4230,.T.) ;
#45366=EDGE_CURVE('',#37093,#37137,#4231,.T.) ;
#45367=EDGE_CURVE('',#37137,#37138,#4232,.T.) ;
#45368=EDGE_CURVE('',#37138,#37094,#4233,.T.) ;
#45369=EDGE_CURVE('',#37139,#37140,#4234,.T.) ;
#45370=EDGE_CURVE('',#37140,#37141,#4235,.T.) ;
#45371=EDGE_CURVE('',#37141,#37142,#4236,.T.) ;
#45372=EDGE_CURVE('',#37142,#37139,#4237,.T.) ;
#45373=EDGE_CURVE('',#37143,#37144,#4238,.T.) ;
#45374=EDGE_CURVE('',#37144,#37145,#4239,.T.) ;
#45375=EDGE_CURVE('',#37145,#37146,#4240,.T.) ;
#45376=EDGE_CURVE('',#37146,#37143,#4241,.T.) ;
#45377=EDGE_CURVE('',#37147,#37148,#4242,.T.) ;
#45378=EDGE_CURVE('',#37148,#37087,#4243,.T.) ;
#45379=EDGE_CURVE('',#37088,#37147,#4244,.T.) ;
#45380=EDGE_CURVE('',#37091,#37149,#4245,.T.) ;
#45381=EDGE_CURVE('',#37149,#37150,#4246,.T.) ;
#45382=EDGE_CURVE('',#37150,#37092,#4247,.T.) ;
#45383=EDGE_CURVE('',#37151,#37152,#4248,.T.) ;
#45384=EDGE_CURVE('',#37152,#37153,#4249,.T.) ;
#45385=EDGE_CURVE('',#37153,#37154,#4250,.T.) ;
#45386=EDGE_CURVE('',#37154,#37151,#4251,.T.) ;
#45387=EDGE_CURVE('',#37155,#37156,#4252,.T.) ;
#45388=EDGE_CURVE('',#37156,#37157,#4253,.T.) ;
#45389=EDGE_CURVE('',#37157,#37158,#4254,.T.) ;
#45390=EDGE_CURVE('',#37158,#37155,#4255,.T.) ;
#45391=EDGE_CURVE('',#37159,#37160,#4256,.T.) ;
#45392=EDGE_CURVE('',#37160,#37161,#4257,.T.) ;
#45393=EDGE_CURVE('',#37161,#37162,#4258,.T.) ;
#45394=EDGE_CURVE('',#37162,#37159,#4259,.T.) ;
#45395=EDGE_CURVE('',#37163,#37164,#4260,.T.) ;
#45396=EDGE_CURVE('',#37164,#37165,#4261,.T.) ;
#45397=EDGE_CURVE('',#37165,#37166,#4262,.T.) ;
#45398=EDGE_CURVE('',#37166,#37163,#4263,.T.) ;
#45399=EDGE_CURVE('',#37153,#37115,#30327,.T.) ;
#45400=EDGE_CURVE('',#37154,#37118,#30328,.T.) ;
#45401=EDGE_CURVE('',#37115,#37120,#30329,.T.) ;
#45402=EDGE_CURVE('',#37119,#37116,#30330,.T.) ;
#45403=EDGE_CURVE('',#37154,#37111,#30331,.T.) ;
#45404=EDGE_CURVE('',#37111,#37118,#30332,.T.) ;
#45405=EDGE_CURVE('',#37116,#37156,#30333,.T.) ;
#45406=EDGE_CURVE('',#37117,#37155,#30334,.T.) ;
#45407=EDGE_CURVE('',#37112,#37117,#30335,.T.) ;
#45408=EDGE_CURVE('',#37151,#37114,#30336,.T.) ;
#45409=EDGE_CURVE('',#37112,#37155,#30337,.T.) ;
#45410=EDGE_CURVE('',#37151,#37107,#30338,.T.) ;
#45411=EDGE_CURVE('',#37107,#37114,#30339,.T.) ;
#45412=EDGE_CURVE('',#37113,#37158,#30340,.T.) ;
#45413=EDGE_CURVE('',#37108,#37113,#30341,.T.) ;
#45414=EDGE_CURVE('',#37110,#37152,#30342,.T.) ;
#45415=EDGE_CURVE('',#37108,#37158,#30343,.T.) ;
#45416=EDGE_CURVE('',#37105,#37110,#30344,.T.) ;
#45417=EDGE_CURVE('',#37109,#37106,#30345,.T.) ;
#45418=EDGE_CURVE('',#37157,#37109,#30346,.T.) ;
#45419=EDGE_CURVE('',#37161,#37131,#30347,.T.) ;
#45420=EDGE_CURVE('',#37162,#37134,#30348,.T.) ;
#45421=EDGE_CURVE('',#37131,#37136,#30349,.T.) ;
#45422=EDGE_CURVE('',#37135,#37132,#30350,.T.) ;
#45423=EDGE_CURVE('',#37162,#37145,#30351,.T.) ;
#45424=EDGE_CURVE('',#37145,#37134,#30352,.T.) ;
#45425=EDGE_CURVE('',#37132,#37164,#30353,.T.) ;
#45426=EDGE_CURVE('',#37133,#37163,#30354,.T.) ;
#45427=EDGE_CURVE('',#37146,#37133,#30355,.T.) ;
#45428=EDGE_CURVE('',#37159,#37144,#30356,.T.) ;
#45429=EDGE_CURVE('',#37146,#37163,#30357,.T.) ;
#45430=EDGE_CURVE('',#37159,#37139,#30358,.T.) ;
#45431=EDGE_CURVE('',#37139,#37144,#30359,.T.) ;
#45432=EDGE_CURVE('',#37143,#37166,#30360,.T.) ;
#45433=EDGE_CURVE('',#37140,#37143,#30361,.T.) ;
#45434=EDGE_CURVE('',#37142,#37160,#30362,.T.) ;
#45435=EDGE_CURVE('',#37140,#37166,#30363,.T.) ;
#45436=EDGE_CURVE('',#37137,#37142,#30364,.T.) ;
#45437=EDGE_CURVE('',#37141,#37138,#30365,.T.) ;
#45438=EDGE_CURVE('',#37165,#37141,#30366,.T.) ;
#45439=EDGE_CURVE('',#37129,#37121,#30367,.T.) ;
#45440=EDGE_CURVE('',#37130,#37120,#30368,.T.) ;
#45441=EDGE_CURVE('',#37130,#37153,#30369,.T.) ;
#45442=EDGE_CURVE('',#37127,#37152,#30370,.T.) ;
#45443=EDGE_CURVE('',#37127,#37105,#30371,.T.) ;
#45444=EDGE_CURVE('',#37128,#37104,#30372,.T.) ;
#45445=EDGE_CURVE('',#37125,#37103,#30373,.T.) ;
#45446=EDGE_CURVE('',#37126,#37106,#30374,.T.) ;
#45447=EDGE_CURVE('',#37126,#37157,#30375,.T.) ;
#45448=EDGE_CURVE('',#37123,#37156,#30376,.T.) ;
#45449=EDGE_CURVE('',#37123,#37119,#30377,.T.) ;
#45450=EDGE_CURVE('',#37124,#37122,#30378,.T.) ;
#45451=EDGE_CURVE('',#37149,#37136,#30379,.T.) ;
#45452=EDGE_CURVE('',#37149,#37161,#30380,.T.) ;
#45453=EDGE_CURVE('',#37150,#37160,#30381,.T.) ;
#45454=EDGE_CURVE('',#37150,#37137,#30382,.T.) ;
#45455=EDGE_CURVE('',#37135,#37148,#30383,.T.) ;
#45456=EDGE_CURVE('',#37164,#37148,#30384,.T.) ;
#45457=EDGE_CURVE('',#37165,#37147,#30385,.T.) ;
#45458=EDGE_CURVE('',#37147,#37138,#30386,.T.) ;
#45459=EDGE_CURVE('',#37167,#37168,#4264,.T.) ;
#45460=EDGE_CURVE('',#37168,#37169,#4265,.T.) ;
#45461=EDGE_CURVE('',#37169,#37170,#4266,.T.) ;
#45462=EDGE_CURVE('',#37170,#37171,#4267,.T.) ;
#45463=EDGE_CURVE('',#37171,#37172,#4268,.T.) ;
#45464=EDGE_CURVE('',#37172,#37173,#4269,.T.) ;
#45465=EDGE_CURVE('',#37174,#37173,#30387,.T.) ;
#45466=EDGE_CURVE('',#37174,#37175,#4270,.T.) ;
#45467=EDGE_CURVE('',#37176,#37175,#30388,.T.) ;
#45468=EDGE_CURVE('',#37176,#37167,#4271,.T.) ;
#45469=EDGE_CURVE('',#37177,#37178,#4272,.T.) ;
#45470=EDGE_CURVE('',#37178,#37179,#4273,.T.) ;
#45471=EDGE_CURVE('',#37179,#37180,#4274,.T.) ;
#45472=EDGE_CURVE('',#37180,#37181,#4275,.T.) ;
#45473=EDGE_CURVE('',#37181,#37182,#4276,.T.) ;
#45474=EDGE_CURVE('',#37182,#37183,#4277,.T.) ;
#45475=EDGE_CURVE('',#37184,#37183,#30389,.T.) ;
#45476=EDGE_CURVE('',#37184,#37185,#4278,.T.) ;
#45477=EDGE_CURVE('',#37186,#37185,#30390,.T.) ;
#45478=EDGE_CURVE('',#37186,#37177,#4279,.T.) ;
#45479=EDGE_CURVE('',#37187,#37188,#4280,.T.) ;
#45480=EDGE_CURVE('',#37188,#37189,#4281,.T.) ;
#45481=EDGE_CURVE('',#37189,#37190,#4282,.T.) ;
#45482=EDGE_CURVE('',#37190,#37191,#4283,.T.) ;
#45483=EDGE_CURVE('',#37191,#37192,#4284,.T.) ;
#45484=EDGE_CURVE('',#37192,#37193,#4285,.T.) ;
#45485=EDGE_CURVE('',#37194,#37193,#30391,.T.) ;
#45486=EDGE_CURVE('',#37194,#37195,#4286,.T.) ;
#45487=EDGE_CURVE('',#37196,#37195,#30392,.T.) ;
#45488=EDGE_CURVE('',#37196,#37187,#4287,.T.) ;
#45489=EDGE_CURVE('',#37197,#37198,#4288,.T.) ;
#45490=EDGE_CURVE('',#37198,#37199,#4289,.T.) ;
#45491=EDGE_CURVE('',#37199,#37200,#4290,.T.) ;
#45492=EDGE_CURVE('',#37200,#37201,#4291,.T.) ;
#45493=EDGE_CURVE('',#37201,#37202,#4292,.T.) ;
#45494=EDGE_CURVE('',#37202,#37203,#4293,.T.) ;
#45495=EDGE_CURVE('',#37204,#37203,#30393,.T.) ;
#45496=EDGE_CURVE('',#37204,#37205,#4294,.T.) ;
#45497=EDGE_CURVE('',#37206,#37205,#30394,.T.) ;
#45498=EDGE_CURVE('',#37206,#37197,#4295,.T.) ;
#45499=EDGE_CURVE('',#37207,#37208,#4296,.T.) ;
#45500=EDGE_CURVE('',#37208,#37209,#4297,.T.) ;
#45501=EDGE_CURVE('',#37209,#37210,#4298,.T.) ;
#45502=EDGE_CURVE('',#37210,#37211,#4299,.T.) ;
#45503=EDGE_CURVE('',#37211,#37212,#4300,.T.) ;
#45504=EDGE_CURVE('',#37212,#37213,#4301,.T.) ;
#45505=EDGE_CURVE('',#37214,#37213,#30395,.T.) ;
#45506=EDGE_CURVE('',#37214,#37215,#4302,.T.) ;
#45507=EDGE_CURVE('',#37216,#37215,#30396,.T.) ;
#45508=EDGE_CURVE('',#37216,#37207,#4303,.T.) ;
#45509=EDGE_CURVE('',#37217,#37218,#4304,.T.) ;
#45510=EDGE_CURVE('',#37218,#37219,#4305,.T.) ;
#45511=EDGE_CURVE('',#37219,#37220,#4306,.T.) ;
#45512=EDGE_CURVE('',#37220,#37221,#4307,.T.) ;
#45513=EDGE_CURVE('',#37221,#37222,#4308,.T.) ;
#45514=EDGE_CURVE('',#37222,#37223,#4309,.T.) ;
#45515=EDGE_CURVE('',#37224,#37223,#30397,.T.) ;
#45516=EDGE_CURVE('',#37224,#37225,#4310,.T.) ;
#45517=EDGE_CURVE('',#37226,#37225,#30398,.T.) ;
#45518=EDGE_CURVE('',#37226,#37217,#4311,.T.) ;
#45519=EDGE_CURVE('',#37227,#37228,#4312,.T.) ;
#45520=EDGE_CURVE('',#37228,#37229,#4313,.T.) ;
#45521=EDGE_CURVE('',#37229,#37230,#4314,.T.) ;
#45522=EDGE_CURVE('',#37230,#37231,#4315,.T.) ;
#45523=EDGE_CURVE('',#37231,#37232,#4316,.T.) ;
#45524=EDGE_CURVE('',#37232,#37233,#4317,.T.) ;
#45525=EDGE_CURVE('',#37234,#37233,#30399,.T.) ;
#45526=EDGE_CURVE('',#37234,#37235,#4318,.T.) ;
#45527=EDGE_CURVE('',#37236,#37235,#30400,.T.) ;
#45528=EDGE_CURVE('',#37236,#37227,#4319,.T.) ;
#45529=EDGE_CURVE('',#37237,#37238,#4320,.T.) ;
#45530=EDGE_CURVE('',#37238,#37239,#4321,.T.) ;
#45531=EDGE_CURVE('',#37239,#37240,#4322,.T.) ;
#45532=EDGE_CURVE('',#37240,#37241,#4323,.T.) ;
#45533=EDGE_CURVE('',#37241,#37242,#4324,.T.) ;
#45534=EDGE_CURVE('',#37242,#37243,#4325,.T.) ;
#45535=EDGE_CURVE('',#37244,#37243,#30401,.T.) ;
#45536=EDGE_CURVE('',#37244,#37245,#4326,.T.) ;
#45537=EDGE_CURVE('',#37246,#37245,#30402,.T.) ;
#45538=EDGE_CURVE('',#37246,#37237,#4327,.T.) ;
#45539=EDGE_CURVE('',#37247,#37248,#4328,.T.) ;
#45540=EDGE_CURVE('',#37248,#37249,#4329,.T.) ;
#45541=EDGE_CURVE('',#37249,#37250,#4330,.T.) ;
#45542=EDGE_CURVE('',#37250,#37251,#4331,.T.) ;
#45543=EDGE_CURVE('',#37251,#37252,#4332,.T.) ;
#45544=EDGE_CURVE('',#37252,#37253,#4333,.T.) ;
#45545=EDGE_CURVE('',#37254,#37253,#30403,.T.) ;
#45546=EDGE_CURVE('',#37254,#37255,#4334,.T.) ;
#45547=EDGE_CURVE('',#37256,#37255,#30404,.T.) ;
#45548=EDGE_CURVE('',#37256,#37247,#4335,.T.) ;
#45549=EDGE_CURVE('',#37257,#37258,#4336,.T.) ;
#45550=EDGE_CURVE('',#37258,#37259,#4337,.T.) ;
#45551=EDGE_CURVE('',#37259,#37260,#4338,.T.) ;
#45552=EDGE_CURVE('',#37260,#37257,#4339,.T.) ;
#45553=EDGE_CURVE('',#36356,#37261,#4340,.T.) ;
#45554=EDGE_CURVE('',#37261,#37262,#4341,.T.) ;
#45555=EDGE_CURVE('',#37262,#36357,#4342,.T.) ;
#45556=EDGE_CURVE('',#37263,#37264,#4343,.T.) ;
#45557=EDGE_CURVE('',#37264,#37265,#4344,.T.) ;
#45558=EDGE_CURVE('',#37265,#37266,#4345,.T.) ;
#45559=EDGE_CURVE('',#37266,#37263,#4346,.T.) ;
#45560=EDGE_CURVE('',#37267,#37268,#4347,.T.) ;
#45561=EDGE_CURVE('',#37268,#37269,#4348,.T.) ;
#45562=EDGE_CURVE('',#37269,#37270,#4349,.T.) ;
#45563=EDGE_CURVE('',#37270,#37267,#4350,.T.) ;
#45564=EDGE_CURVE('',#37271,#37272,#4351,.T.) ;
#45565=EDGE_CURVE('',#37272,#37273,#4352,.T.) ;
#45566=EDGE_CURVE('',#37273,#37274,#4353,.T.) ;
#45567=EDGE_CURVE('',#37274,#37271,#4354,.T.) ;
#45568=EDGE_CURVE('',#37275,#37276,#4355,.T.) ;
#45569=EDGE_CURVE('',#37276,#37277,#4356,.T.) ;
#45570=EDGE_CURVE('',#37277,#37278,#4357,.T.) ;
#45571=EDGE_CURVE('',#37278,#37275,#4358,.T.) ;
#45572=EDGE_CURVE('',#36305,#37279,#4359,.T.) ;
#45573=EDGE_CURVE('',#37279,#37280,#4360,.T.) ;
#45574=EDGE_CURVE('',#37280,#36306,#4361,.T.) ;
#45575=EDGE_CURVE('',#37281,#37282,#4362,.T.) ;
#45576=EDGE_CURVE('',#37282,#37283,#4363,.T.) ;
#45577=EDGE_CURVE('',#37283,#37284,#4364,.T.) ;
#45578=EDGE_CURVE('',#37284,#37281,#4365,.T.) ;
#45579=EDGE_CURVE('',#37285,#37286,#4366,.T.) ;
#45580=EDGE_CURVE('',#37286,#37287,#4367,.T.) ;
#45581=EDGE_CURVE('',#37287,#37288,#4368,.T.) ;
#45582=EDGE_CURVE('',#37288,#37285,#4369,.T.) ;
#45583=EDGE_CURVE('',#37289,#37290,#4370,.T.) ;
#45584=EDGE_CURVE('',#37290,#37291,#4371,.T.) ;
#45585=EDGE_CURVE('',#37291,#37292,#4372,.T.) ;
#45586=EDGE_CURVE('',#37292,#37289,#4373,.T.) ;
#45587=EDGE_CURVE('',#37293,#37294,#4374,.T.) ;
#45588=EDGE_CURVE('',#37294,#37295,#4375,.T.) ;
#45589=EDGE_CURVE('',#37295,#37296,#4376,.T.) ;
#45590=EDGE_CURVE('',#37296,#37293,#4377,.T.) ;
#45591=EDGE_CURVE('',#36290,#37297,#4378,.T.) ;
#45592=EDGE_CURVE('',#37297,#37298,#4379,.T.) ;
#45593=EDGE_CURVE('',#37298,#36291,#4380,.T.) ;
#45594=EDGE_CURVE('',#37299,#37300,#4381,.T.) ;
#45595=EDGE_CURVE('',#37300,#37301,#4382,.T.) ;
#45596=EDGE_CURVE('',#37301,#37302,#4383,.T.) ;
#45597=EDGE_CURVE('',#37302,#37299,#4384,.T.) ;
#45598=EDGE_CURVE('',#37303,#37304,#4385,.T.) ;
#45599=EDGE_CURVE('',#37304,#37305,#4386,.T.) ;
#45600=EDGE_CURVE('',#37305,#37306,#4387,.T.) ;
#45601=EDGE_CURVE('',#37306,#37303,#4388,.T.) ;
#45602=EDGE_CURVE('',#37307,#37308,#4389,.T.) ;
#45603=EDGE_CURVE('',#37308,#37309,#4390,.T.) ;
#45604=EDGE_CURVE('',#37309,#37310,#4391,.T.) ;
#45605=EDGE_CURVE('',#37310,#37307,#4392,.T.) ;
#45606=EDGE_CURVE('',#37311,#37312,#4393,.T.) ;
#45607=EDGE_CURVE('',#37312,#37313,#4394,.T.) ;
#45608=EDGE_CURVE('',#37313,#37314,#4395,.T.) ;
#45609=EDGE_CURVE('',#37314,#37311,#4396,.T.) ;
#45610=EDGE_CURVE('',#36275,#37315,#4397,.T.) ;
#45611=EDGE_CURVE('',#37315,#37316,#4398,.T.) ;
#45612=EDGE_CURVE('',#37316,#36276,#4399,.T.) ;
#45613=EDGE_CURVE('',#37317,#37318,#4400,.T.) ;
#45614=EDGE_CURVE('',#37318,#37319,#4401,.T.) ;
#45615=EDGE_CURVE('',#37319,#37320,#4402,.T.) ;
#45616=EDGE_CURVE('',#37320,#37317,#4403,.T.) ;
#45617=EDGE_CURVE('',#37321,#37322,#4404,.T.) ;
#45618=EDGE_CURVE('',#37322,#37323,#4405,.T.) ;
#45619=EDGE_CURVE('',#37323,#37324,#4406,.T.) ;
#45620=EDGE_CURVE('',#37324,#37321,#4407,.T.) ;
#45621=EDGE_CURVE('',#37325,#37326,#4408,.T.) ;
#45622=EDGE_CURVE('',#37326,#37327,#4409,.T.) ;
#45623=EDGE_CURVE('',#37327,#37328,#4410,.T.) ;
#45624=EDGE_CURVE('',#37328,#37325,#4411,.T.) ;
#45625=EDGE_CURVE('',#37329,#37330,#4412,.T.) ;
#45626=EDGE_CURVE('',#37330,#37331,#4413,.T.) ;
#45627=EDGE_CURVE('',#37331,#37332,#4414,.T.) ;
#45628=EDGE_CURVE('',#37332,#37329,#4415,.T.) ;
#45629=EDGE_CURVE('',#36260,#37333,#4416,.T.) ;
#45630=EDGE_CURVE('',#37333,#37334,#4417,.T.) ;
#45631=EDGE_CURVE('',#37334,#36261,#4418,.T.) ;
#45632=EDGE_CURVE('',#37335,#37336,#4419,.T.) ;
#45633=EDGE_CURVE('',#37336,#37337,#4420,.T.) ;
#45634=EDGE_CURVE('',#37337,#37338,#4421,.T.) ;
#45635=EDGE_CURVE('',#37338,#37335,#4422,.T.) ;
#45636=EDGE_CURVE('',#37339,#37340,#4423,.T.) ;
#45637=EDGE_CURVE('',#37340,#37341,#4424,.T.) ;
#45638=EDGE_CURVE('',#37341,#37342,#4425,.T.) ;
#45639=EDGE_CURVE('',#37342,#37339,#4426,.T.) ;
#45640=EDGE_CURVE('',#37343,#37344,#4427,.T.) ;
#45641=EDGE_CURVE('',#37344,#37345,#4428,.T.) ;
#45642=EDGE_CURVE('',#37345,#37346,#4429,.T.) ;
#45643=EDGE_CURVE('',#37346,#37343,#4430,.T.) ;
#45644=EDGE_CURVE('',#37347,#37348,#4431,.T.) ;
#45645=EDGE_CURVE('',#37348,#37349,#4432,.T.) ;
#45646=EDGE_CURVE('',#37349,#37350,#4433,.T.) ;
#45647=EDGE_CURVE('',#37350,#37347,#4434,.T.) ;
#45648=EDGE_CURVE('',#36245,#37351,#4435,.T.) ;
#45649=EDGE_CURVE('',#37351,#37352,#4436,.T.) ;
#45650=EDGE_CURVE('',#37352,#36246,#4437,.T.) ;
#45651=EDGE_CURVE('',#37353,#37354,#4438,.T.) ;
#45652=EDGE_CURVE('',#37354,#37355,#4439,.T.) ;
#45653=EDGE_CURVE('',#37355,#37356,#4440,.T.) ;
#45654=EDGE_CURVE('',#37356,#37353,#4441,.T.) ;
#45655=EDGE_CURVE('',#37357,#37358,#4442,.T.) ;
#45656=EDGE_CURVE('',#37358,#37359,#4443,.T.) ;
#45657=EDGE_CURVE('',#37359,#37360,#4444,.T.) ;
#45658=EDGE_CURVE('',#37360,#37357,#4445,.T.) ;
#45659=EDGE_CURVE('',#37361,#37362,#4446,.T.) ;
#45660=EDGE_CURVE('',#37362,#37363,#4447,.T.) ;
#45661=EDGE_CURVE('',#37363,#37364,#4448,.T.) ;
#45662=EDGE_CURVE('',#37364,#37361,#4449,.T.) ;
#45663=EDGE_CURVE('',#37365,#37366,#4450,.T.) ;
#45664=EDGE_CURVE('',#37366,#37367,#4451,.T.) ;
#45665=EDGE_CURVE('',#37367,#37368,#4452,.T.) ;
#45666=EDGE_CURVE('',#37368,#37365,#4453,.T.) ;
#45667=EDGE_CURVE('',#36230,#37369,#4454,.T.) ;
#45668=EDGE_CURVE('',#37369,#37370,#4455,.T.) ;
#45669=EDGE_CURVE('',#37370,#36231,#4456,.T.) ;
#45670=EDGE_CURVE('',#37371,#37372,#4457,.T.) ;
#45671=EDGE_CURVE('',#37372,#37373,#4458,.T.) ;
#45672=EDGE_CURVE('',#37373,#37374,#4459,.T.) ;
#45673=EDGE_CURVE('',#37374,#37371,#4460,.T.) ;
#45674=EDGE_CURVE('',#37375,#37376,#4461,.T.) ;
#45675=EDGE_CURVE('',#37376,#37377,#4462,.T.) ;
#45676=EDGE_CURVE('',#37377,#37378,#4463,.T.) ;
#45677=EDGE_CURVE('',#37378,#37375,#4464,.T.) ;
#45678=EDGE_CURVE('',#37379,#37380,#4465,.T.) ;
#45679=EDGE_CURVE('',#37380,#37381,#4466,.T.) ;
#45680=EDGE_CURVE('',#37381,#37382,#4467,.T.) ;
#45681=EDGE_CURVE('',#37382,#37379,#4468,.T.) ;
#45682=EDGE_CURVE('',#37383,#37384,#4469,.T.) ;
#45683=EDGE_CURVE('',#37384,#37385,#4470,.T.) ;
#45684=EDGE_CURVE('',#37385,#37386,#4471,.T.) ;
#45685=EDGE_CURVE('',#37386,#37383,#4472,.T.) ;
#45686=EDGE_CURVE('',#36215,#37387,#4473,.T.) ;
#45687=EDGE_CURVE('',#37387,#37388,#4474,.T.) ;
#45688=EDGE_CURVE('',#37388,#36216,#4475,.T.) ;
#45689=EDGE_CURVE('',#37389,#37390,#4476,.T.) ;
#45690=EDGE_CURVE('',#37390,#37391,#4477,.T.) ;
#45691=EDGE_CURVE('',#37391,#37392,#4478,.T.) ;
#45692=EDGE_CURVE('',#37392,#37389,#4479,.T.) ;
#45693=EDGE_CURVE('',#37393,#37394,#4480,.T.) ;
#45694=EDGE_CURVE('',#37394,#37395,#4481,.T.) ;
#45695=EDGE_CURVE('',#37395,#37396,#4482,.T.) ;
#45696=EDGE_CURVE('',#37396,#37393,#4483,.T.) ;
#45697=EDGE_CURVE('',#37397,#37398,#4484,.T.) ;
#45698=EDGE_CURVE('',#37398,#37399,#4485,.T.) ;
#45699=EDGE_CURVE('',#37399,#37400,#4486,.T.) ;
#45700=EDGE_CURVE('',#37400,#37397,#4487,.T.) ;
#45701=EDGE_CURVE('',#37401,#37402,#4488,.T.) ;
#45702=EDGE_CURVE('',#37402,#37403,#4489,.T.) ;
#45703=EDGE_CURVE('',#37403,#37404,#4490,.T.) ;
#45704=EDGE_CURVE('',#37404,#37401,#4491,.T.) ;
#45705=EDGE_CURVE('',#36200,#37405,#4492,.T.) ;
#45706=EDGE_CURVE('',#37405,#37406,#4493,.T.) ;
#45707=EDGE_CURVE('',#37406,#36201,#4494,.T.) ;
#45708=EDGE_CURVE('',#37407,#37408,#4495,.T.) ;
#45709=EDGE_CURVE('',#37408,#37409,#4496,.T.) ;
#45710=EDGE_CURVE('',#37409,#37410,#4497,.T.) ;
#45711=EDGE_CURVE('',#37410,#37407,#4498,.T.) ;
#45712=EDGE_CURVE('',#37411,#37412,#4499,.T.) ;
#45713=EDGE_CURVE('',#37412,#37413,#4500,.T.) ;
#45714=EDGE_CURVE('',#37413,#37414,#4501,.T.) ;
#45715=EDGE_CURVE('',#37414,#37411,#4502,.T.) ;
#45716=EDGE_CURVE('',#37415,#37416,#4503,.T.) ;
#45717=EDGE_CURVE('',#37416,#37417,#4504,.T.) ;
#45718=EDGE_CURVE('',#37417,#37418,#4505,.T.) ;
#45719=EDGE_CURVE('',#37418,#37415,#4506,.T.) ;
#45720=EDGE_CURVE('',#37419,#37420,#4507,.T.) ;
#45721=EDGE_CURVE('',#37419,#37421,#30405,.T.) ;
#45722=EDGE_CURVE('',#37421,#37422,#4508,.T.) ;
#45723=EDGE_CURVE('',#37422,#37420,#30406,.T.) ;
#45724=EDGE_CURVE('',#37421,#37423,#4509,.T.) ;
#45725=EDGE_CURVE('',#37423,#37424,#4510,.T.) ;
#45726=EDGE_CURVE('',#37424,#37422,#4511,.T.) ;
#45727=EDGE_CURVE('',#37423,#37425,#30407,.T.) ;
#45728=EDGE_CURVE('',#37425,#37426,#4512,.T.) ;
#45729=EDGE_CURVE('',#37426,#37424,#30408,.T.) ;
#45730=EDGE_CURVE('',#37425,#37427,#4513,.T.) ;
#45731=EDGE_CURVE('',#37427,#37428,#4514,.T.) ;
#45732=EDGE_CURVE('',#37428,#37426,#4515,.T.) ;
#45733=EDGE_CURVE('',#37427,#37429,#30409,.T.) ;
#45734=EDGE_CURVE('',#37429,#37430,#4516,.T.) ;
#45735=EDGE_CURVE('',#37430,#37428,#30410,.T.) ;
#45736=EDGE_CURVE('',#37429,#36195,#4517,.T.) ;
#45737=EDGE_CURVE('',#36195,#37431,#4518,.T.) ;
#45738=EDGE_CURVE('',#37431,#37430,#4519,.T.) ;
#45739=EDGE_CURVE('',#36196,#37432,#4520,.T.) ;
#45740=EDGE_CURVE('',#37432,#37431,#30411,.T.) ;
#45741=EDGE_CURVE('',#36196,#36377,#4521,.T.) ;
#45742=EDGE_CURVE('',#36347,#37432,#4522,.T.) ;
#45743=EDGE_CURVE('',#36378,#37433,#4523,.T.) ;
#45744=EDGE_CURVE('',#37433,#37434,#4524,.T.) ;
#45745=EDGE_CURVE('',#37434,#36348,#4525,.T.) ;
#45746=EDGE_CURVE('',#37433,#37435,#30412,.T.) ;
#45747=EDGE_CURVE('',#37435,#37436,#4526,.T.) ;
#45748=EDGE_CURVE('',#37436,#37434,#30413,.T.) ;
#45749=EDGE_CURVE('',#37435,#37437,#4527,.T.) ;
#45750=EDGE_CURVE('',#37437,#37438,#4528,.T.) ;
#45751=EDGE_CURVE('',#37438,#37436,#4529,.T.) ;
#45752=EDGE_CURVE('',#37437,#37439,#30414,.T.) ;
#45753=EDGE_CURVE('',#37439,#37440,#4530,.T.) ;
#45754=EDGE_CURVE('',#37440,#37438,#30415,.T.) ;
#45755=EDGE_CURVE('',#37439,#37441,#4531,.T.) ;
#45756=EDGE_CURVE('',#37441,#37442,#4532,.T.) ;
#45757=EDGE_CURVE('',#37442,#37440,#4533,.T.) ;
#45758=EDGE_CURVE('',#37441,#37443,#30416,.T.) ;
#45759=EDGE_CURVE('',#37443,#37444,#4534,.T.) ;
#45760=EDGE_CURVE('',#37444,#37442,#30417,.T.) ;
#45761=EDGE_CURVE('',#37443,#37445,#4535,.T.) ;
#45762=EDGE_CURVE('',#37445,#37446,#4536,.T.) ;
#45763=EDGE_CURVE('',#37446,#37444,#4537,.T.) ;
#45764=EDGE_CURVE('',#37445,#37447,#30418,.T.) ;
#45765=EDGE_CURVE('',#37447,#37448,#4538,.T.) ;
#45766=EDGE_CURVE('',#37448,#37446,#30419,.T.) ;
#45767=EDGE_CURVE('',#37447,#37449,#4539,.T.) ;
#45768=EDGE_CURVE('',#37449,#37450,#4540,.T.) ;
#45769=EDGE_CURVE('',#37450,#37448,#4541,.T.) ;
#45770=EDGE_CURVE('',#37449,#37451,#30420,.T.) ;
#45771=EDGE_CURVE('',#37451,#37452,#4542,.T.) ;
#45772=EDGE_CURVE('',#37452,#37450,#30421,.T.) ;
#45773=EDGE_CURVE('',#37451,#37453,#4543,.T.) ;
#45774=EDGE_CURVE('',#37453,#37454,#4544,.T.) ;
#45775=EDGE_CURVE('',#37454,#37452,#4545,.T.) ;
#45776=EDGE_CURVE('',#37453,#37455,#30422,.T.) ;
#45777=EDGE_CURVE('',#37455,#37456,#4546,.T.) ;
#45778=EDGE_CURVE('',#37456,#37454,#30423,.T.) ;
#45779=EDGE_CURVE('',#37455,#37457,#30424,.T.) ;
#45780=EDGE_CURVE('',#37457,#37458,#4547,.T.) ;
#45781=EDGE_CURVE('',#37458,#37456,#30425,.T.) ;
#45782=EDGE_CURVE('',#37457,#37459,#30426,.T.) ;
#45783=EDGE_CURVE('',#37459,#37460,#4548,.T.) ;
#45784=EDGE_CURVE('',#37460,#37458,#30427,.T.) ;
#45785=EDGE_CURVE('',#37459,#37461,#4549,.T.) ;
#45786=EDGE_CURVE('',#37461,#37462,#4550,.T.) ;
#45787=EDGE_CURVE('',#37462,#37460,#4551,.T.) ;
#45788=EDGE_CURVE('',#37461,#37463,#30428,.T.) ;
#45789=EDGE_CURVE('',#37463,#37464,#4552,.T.) ;
#45790=EDGE_CURVE('',#37464,#37462,#30429,.T.) ;
#45791=EDGE_CURVE('',#37463,#37465,#4553,.T.) ;
#45792=EDGE_CURVE('',#37465,#37466,#4554,.T.) ;
#45793=EDGE_CURVE('',#37466,#37464,#4555,.T.) ;
#45794=EDGE_CURVE('',#37465,#37467,#30430,.T.) ;
#45795=EDGE_CURVE('',#37467,#37468,#4556,.T.) ;
#45796=EDGE_CURVE('',#37468,#37466,#30431,.T.) ;
#45797=EDGE_CURVE('',#37467,#37419,#4557,.T.) ;
#45798=EDGE_CURVE('',#37420,#37468,#4558,.T.) ;
#45799=EDGE_CURVE('',#37469,#37470,#30432,.T.) ;
#45800=EDGE_CURVE('',#37470,#37471,#4559,.T.) ;
#45801=EDGE_CURVE('',#37471,#37472,#30433,.T.) ;
#45802=EDGE_CURVE('',#37472,#37473,#4560,.T.) ;
#45803=EDGE_CURVE('',#37473,#37474,#4561,.T.) ;
#45804=EDGE_CURVE('',#37474,#37475,#4562,.T.) ;
#45805=EDGE_CURVE('',#37475,#37476,#30434,.T.) ;
#45806=EDGE_CURVE('',#37476,#37477,#4563,.T.) ;
#45807=EDGE_CURVE('',#37477,#37478,#4564,.T.) ;
#45808=EDGE_CURVE('',#37478,#37479,#4565,.T.) ;
#45809=EDGE_CURVE('',#37479,#37480,#30435,.T.) ;
#45810=EDGE_CURVE('',#37480,#37481,#4566,.T.) ;
#45811=EDGE_CURVE('',#37481,#37482,#30436,.T.) ;
#45812=EDGE_CURVE('',#37482,#37483,#4567,.T.) ;
#45813=EDGE_CURVE('',#37483,#37484,#4568,.T.) ;
#45814=EDGE_CURVE('',#37484,#36197,#4569,.T.) ;
#45815=EDGE_CURVE('',#36197,#37485,#4570,.T.) ;
#45816=EDGE_CURVE('',#37485,#37469,#4571,.T.) ;
#45817=EDGE_CURVE('',#37486,#37487,#4572,.T.) ;
#45818=EDGE_CURVE('',#37486,#37488,#30437,.T.) ;
#45819=EDGE_CURVE('',#37488,#37489,#4573,.T.) ;
#45820=EDGE_CURVE('',#37489,#37487,#30438,.T.) ;
#45821=EDGE_CURVE('',#37488,#37490,#4574,.T.) ;
#45822=EDGE_CURVE('',#37490,#37491,#4575,.T.) ;
#45823=EDGE_CURVE('',#37491,#37489,#4576,.T.) ;
#45824=EDGE_CURVE('',#37490,#37492,#30439,.T.) ;
#45825=EDGE_CURVE('',#37492,#37493,#4577,.T.) ;
#45826=EDGE_CURVE('',#37493,#37491,#30440,.T.) ;
#45827=EDGE_CURVE('',#37492,#37494,#4578,.T.) ;
#45828=EDGE_CURVE('',#37494,#37495,#4579,.T.) ;
#45829=EDGE_CURVE('',#37495,#37493,#4580,.T.) ;
#45830=EDGE_CURVE('',#37494,#37496,#30441,.T.) ;
#45831=EDGE_CURVE('',#37496,#37497,#4581,.T.) ;
#45832=EDGE_CURVE('',#37497,#37495,#30442,.T.) ;
#45833=EDGE_CURVE('',#37496,#36210,#4582,.T.) ;
#45834=EDGE_CURVE('',#36210,#37498,#4583,.T.) ;
#45835=EDGE_CURVE('',#37498,#37497,#4584,.T.) ;
#45836=EDGE_CURVE('',#36211,#37499,#4585,.T.) ;
#45837=EDGE_CURVE('',#37499,#37498,#30443,.T.) ;
#45838=EDGE_CURVE('',#36211,#36375,#4586,.T.) ;
#45839=EDGE_CURVE('',#36343,#37499,#4587,.T.) ;
#45840=EDGE_CURVE('',#36376,#37500,#4588,.T.) ;
#45841=EDGE_CURVE('',#37500,#37501,#4589,.T.) ;
#45842=EDGE_CURVE('',#37501,#36344,#4590,.T.) ;
#45843=EDGE_CURVE('',#37500,#37502,#30444,.T.) ;
#45844=EDGE_CURVE('',#37502,#37503,#4591,.T.) ;
#45845=EDGE_CURVE('',#37503,#37501,#30445,.T.) ;
#45846=EDGE_CURVE('',#37502,#37504,#4592,.T.) ;
#45847=EDGE_CURVE('',#37504,#37505,#4593,.T.) ;
#45848=EDGE_CURVE('',#37505,#37503,#4594,.T.) ;
#45849=EDGE_CURVE('',#37504,#37506,#30446,.T.) ;
#45850=EDGE_CURVE('',#37506,#37507,#4595,.T.) ;
#45851=EDGE_CURVE('',#37507,#37505,#30447,.T.) ;
#45852=EDGE_CURVE('',#37506,#37508,#4596,.T.) ;
#45853=EDGE_CURVE('',#37508,#37509,#4597,.T.) ;
#45854=EDGE_CURVE('',#37509,#37507,#4598,.T.) ;
#45855=EDGE_CURVE('',#37508,#37510,#30448,.T.) ;
#45856=EDGE_CURVE('',#37510,#37511,#4599,.T.) ;
#45857=EDGE_CURVE('',#37511,#37509,#30449,.T.) ;
#45858=EDGE_CURVE('',#37510,#37512,#4600,.T.) ;
#45859=EDGE_CURVE('',#37512,#37513,#4601,.T.) ;
#45860=EDGE_CURVE('',#37513,#37511,#4602,.T.) ;
#45861=EDGE_CURVE('',#37512,#37514,#30450,.T.) ;
#45862=EDGE_CURVE('',#37514,#37515,#4603,.T.) ;
#45863=EDGE_CURVE('',#37515,#37513,#30451,.T.) ;
#45864=EDGE_CURVE('',#37514,#37516,#4604,.T.) ;
#45865=EDGE_CURVE('',#37516,#37517,#4605,.T.) ;
#45866=EDGE_CURVE('',#37517,#37515,#4606,.T.) ;
#45867=EDGE_CURVE('',#37516,#37518,#30452,.T.) ;
#45868=EDGE_CURVE('',#37518,#37519,#4607,.T.) ;
#45869=EDGE_CURVE('',#37519,#37517,#30453,.T.) ;
#45870=EDGE_CURVE('',#37518,#37520,#4608,.T.) ;
#45871=EDGE_CURVE('',#37520,#37521,#4609,.T.) ;
#45872=EDGE_CURVE('',#37521,#37519,#4610,.T.) ;
#45873=EDGE_CURVE('',#37520,#37522,#30454,.T.) ;
#45874=EDGE_CURVE('',#37522,#37523,#4611,.T.) ;
#45875=EDGE_CURVE('',#37523,#37521,#30455,.T.) ;
#45876=EDGE_CURVE('',#37522,#37524,#30456,.T.) ;
#45877=EDGE_CURVE('',#37524,#37525,#4612,.T.) ;
#45878=EDGE_CURVE('',#37525,#37523,#30457,.T.) ;
#45879=EDGE_CURVE('',#37524,#37526,#30458,.T.) ;
#45880=EDGE_CURVE('',#37526,#37527,#4613,.T.) ;
#45881=EDGE_CURVE('',#37527,#37525,#30459,.T.) ;
#45882=EDGE_CURVE('',#37526,#37528,#4614,.T.) ;
#45883=EDGE_CURVE('',#37528,#37529,#4615,.T.) ;
#45884=EDGE_CURVE('',#37529,#37527,#4616,.T.) ;
#45885=EDGE_CURVE('',#37528,#37530,#30460,.T.) ;
#45886=EDGE_CURVE('',#37530,#37531,#4617,.T.) ;
#45887=EDGE_CURVE('',#37531,#37529,#30461,.T.) ;
#45888=EDGE_CURVE('',#37530,#37532,#4618,.T.) ;
#45889=EDGE_CURVE('',#37532,#37533,#4619,.T.) ;
#45890=EDGE_CURVE('',#37533,#37531,#4620,.T.) ;
#45891=EDGE_CURVE('',#37532,#37534,#30462,.T.) ;
#45892=EDGE_CURVE('',#37534,#37535,#4621,.T.) ;
#45893=EDGE_CURVE('',#37535,#37533,#30463,.T.) ;
#45894=EDGE_CURVE('',#37534,#37486,#4622,.T.) ;
#45895=EDGE_CURVE('',#37487,#37535,#4623,.T.) ;
#45896=EDGE_CURVE('',#37536,#37537,#30464,.T.) ;
#45897=EDGE_CURVE('',#37537,#37538,#4624,.T.) ;
#45898=EDGE_CURVE('',#37538,#37539,#30465,.T.) ;
#45899=EDGE_CURVE('',#37539,#37540,#4625,.T.) ;
#45900=EDGE_CURVE('',#37540,#37541,#4626,.T.) ;
#45901=EDGE_CURVE('',#37541,#37542,#4627,.T.) ;
#45902=EDGE_CURVE('',#37542,#37543,#30466,.T.) ;
#45903=EDGE_CURVE('',#37543,#37544,#4628,.T.) ;
#45904=EDGE_CURVE('',#37544,#37545,#4629,.T.) ;
#45905=EDGE_CURVE('',#37545,#37546,#4630,.T.) ;
#45906=EDGE_CURVE('',#37546,#37547,#30467,.T.) ;
#45907=EDGE_CURVE('',#37547,#37548,#4631,.T.) ;
#45908=EDGE_CURVE('',#37548,#37549,#30468,.T.) ;
#45909=EDGE_CURVE('',#37549,#37550,#4632,.T.) ;
#45910=EDGE_CURVE('',#37550,#37551,#4633,.T.) ;
#45911=EDGE_CURVE('',#37551,#36212,#4634,.T.) ;
#45912=EDGE_CURVE('',#36212,#37552,#4635,.T.) ;
#45913=EDGE_CURVE('',#37552,#37536,#4636,.T.) ;
#45914=EDGE_CURVE('',#37553,#37554,#4637,.T.) ;
#45915=EDGE_CURVE('',#37553,#37555,#30469,.T.) ;
#45916=EDGE_CURVE('',#37555,#37556,#4638,.T.) ;
#45917=EDGE_CURVE('',#37556,#37554,#30470,.T.) ;
#45918=EDGE_CURVE('',#37555,#37557,#4639,.T.) ;
#45919=EDGE_CURVE('',#37557,#37558,#4640,.T.) ;
#45920=EDGE_CURVE('',#37558,#37556,#4641,.T.) ;
#45921=EDGE_CURVE('',#37557,#37559,#30471,.T.) ;
#45922=EDGE_CURVE('',#37559,#37560,#4642,.T.) ;
#45923=EDGE_CURVE('',#37560,#37558,#30472,.T.) ;
#45924=EDGE_CURVE('',#37559,#37561,#4643,.T.) ;
#45925=EDGE_CURVE('',#37561,#37562,#4644,.T.) ;
#45926=EDGE_CURVE('',#37562,#37560,#4645,.T.) ;
#45927=EDGE_CURVE('',#37561,#37563,#30473,.T.) ;
#45928=EDGE_CURVE('',#37563,#37564,#4646,.T.) ;
#45929=EDGE_CURVE('',#37564,#37562,#30474,.T.) ;
#45930=EDGE_CURVE('',#37563,#36225,#4647,.T.) ;
#45931=EDGE_CURVE('',#36225,#37565,#4648,.T.) ;
#45932=EDGE_CURVE('',#37565,#37564,#4649,.T.) ;
#45933=EDGE_CURVE('',#36226,#37566,#4650,.T.) ;
#45934=EDGE_CURVE('',#37566,#37565,#30475,.T.) ;
#45935=EDGE_CURVE('',#36226,#36373,#4651,.T.) ;
#45936=EDGE_CURVE('',#36339,#37566,#4652,.T.) ;
#45937=EDGE_CURVE('',#36374,#37567,#4653,.T.) ;
#45938=EDGE_CURVE('',#37567,#37568,#4654,.T.) ;
#45939=EDGE_CURVE('',#37568,#36340,#4655,.T.) ;
#45940=EDGE_CURVE('',#37567,#37569,#30476,.T.) ;
#45941=EDGE_CURVE('',#37569,#37570,#4656,.T.) ;
#45942=EDGE_CURVE('',#37570,#37568,#30477,.T.) ;
#45943=EDGE_CURVE('',#37569,#37571,#4657,.T.) ;
#45944=EDGE_CURVE('',#37571,#37572,#4658,.T.) ;
#45945=EDGE_CURVE('',#37572,#37570,#4659,.T.) ;
#45946=EDGE_CURVE('',#37571,#37573,#30478,.T.) ;
#45947=EDGE_CURVE('',#37573,#37574,#4660,.T.) ;
#45948=EDGE_CURVE('',#37574,#37572,#30479,.T.) ;
#45949=EDGE_CURVE('',#37573,#37575,#4661,.T.) ;
#45950=EDGE_CURVE('',#37575,#37576,#4662,.T.) ;
#45951=EDGE_CURVE('',#37576,#37574,#4663,.T.) ;
#45952=EDGE_CURVE('',#37575,#37577,#30480,.T.) ;
#45953=EDGE_CURVE('',#37577,#37578,#4664,.T.) ;
#45954=EDGE_CURVE('',#37578,#37576,#30481,.T.) ;
#45955=EDGE_CURVE('',#37577,#37579,#4665,.T.) ;
#45956=EDGE_CURVE('',#37579,#37580,#4666,.T.) ;
#45957=EDGE_CURVE('',#37580,#37578,#4667,.T.) ;
#45958=EDGE_CURVE('',#37579,#37581,#30482,.T.) ;
#45959=EDGE_CURVE('',#37581,#37582,#4668,.T.) ;
#45960=EDGE_CURVE('',#37582,#37580,#30483,.T.) ;
#45961=EDGE_CURVE('',#37581,#37583,#4669,.T.) ;
#45962=EDGE_CURVE('',#37583,#37584,#4670,.T.) ;
#45963=EDGE_CURVE('',#37584,#37582,#4671,.T.) ;
#45964=EDGE_CURVE('',#37583,#37585,#30484,.T.) ;
#45965=EDGE_CURVE('',#37585,#37586,#4672,.T.) ;
#45966=EDGE_CURVE('',#37586,#37584,#30485,.T.) ;
#45967=EDGE_CURVE('',#37585,#37587,#4673,.T.) ;
#45968=EDGE_CURVE('',#37587,#37588,#4674,.T.) ;
#45969=EDGE_CURVE('',#37588,#37586,#4675,.T.) ;
#45970=EDGE_CURVE('',#37587,#37589,#30486,.T.) ;
#45971=EDGE_CURVE('',#37589,#37590,#4676,.T.) ;
#45972=EDGE_CURVE('',#37590,#37588,#30487,.T.) ;
#45973=EDGE_CURVE('',#37589,#37591,#30488,.T.) ;
#45974=EDGE_CURVE('',#37591,#37592,#4677,.T.) ;
#45975=EDGE_CURVE('',#37592,#37590,#30489,.T.) ;
#45976=EDGE_CURVE('',#37591,#37593,#30490,.T.) ;
#45977=EDGE_CURVE('',#37593,#37594,#4678,.T.) ;
#45978=EDGE_CURVE('',#37594,#37592,#30491,.T.) ;
#45979=EDGE_CURVE('',#37593,#37595,#4679,.T.) ;
#45980=EDGE_CURVE('',#37595,#37596,#4680,.T.) ;
#45981=EDGE_CURVE('',#37596,#37594,#4681,.T.) ;
#45982=EDGE_CURVE('',#37595,#37597,#30492,.T.) ;
#45983=EDGE_CURVE('',#37597,#37598,#4682,.T.) ;
#45984=EDGE_CURVE('',#37598,#37596,#30493,.T.) ;
#45985=EDGE_CURVE('',#37597,#37599,#4683,.T.) ;
#45986=EDGE_CURVE('',#37599,#37600,#4684,.T.) ;
#45987=EDGE_CURVE('',#37600,#37598,#4685,.T.) ;
#45988=EDGE_CURVE('',#37599,#37601,#30494,.T.) ;
#45989=EDGE_CURVE('',#37601,#37602,#4686,.T.) ;
#45990=EDGE_CURVE('',#37602,#37600,#30495,.T.) ;
#45991=EDGE_CURVE('',#37601,#37553,#4687,.T.) ;
#45992=EDGE_CURVE('',#37554,#37602,#4688,.T.) ;
#45993=EDGE_CURVE('',#37603,#37604,#30496,.T.) ;
#45994=EDGE_CURVE('',#37604,#37605,#4689,.T.) ;
#45995=EDGE_CURVE('',#37605,#37606,#30497,.T.) ;
#45996=EDGE_CURVE('',#37606,#37607,#4690,.T.) ;
#45997=EDGE_CURVE('',#37607,#37608,#4691,.T.) ;
#45998=EDGE_CURVE('',#37608,#37609,#4692,.T.) ;
#45999=EDGE_CURVE('',#37609,#37610,#30498,.T.) ;
#46000=EDGE_CURVE('',#37610,#37611,#4693,.T.) ;
#46001=EDGE_CURVE('',#37611,#37612,#4694,.T.) ;
#46002=EDGE_CURVE('',#37612,#37613,#4695,.T.) ;
#46003=EDGE_CURVE('',#37613,#37614,#30499,.T.) ;
#46004=EDGE_CURVE('',#37614,#37615,#4696,.T.) ;
#46005=EDGE_CURVE('',#37615,#37616,#30500,.T.) ;
#46006=EDGE_CURVE('',#37616,#37617,#4697,.T.) ;
#46007=EDGE_CURVE('',#37617,#37618,#4698,.T.) ;
#46008=EDGE_CURVE('',#37618,#36227,#4699,.T.) ;
#46009=EDGE_CURVE('',#36227,#37619,#4700,.T.) ;
#46010=EDGE_CURVE('',#37619,#37603,#4701,.T.) ;
#46011=EDGE_CURVE('',#37620,#37621,#4702,.T.) ;
#46012=EDGE_CURVE('',#37620,#37622,#30501,.T.) ;
#46013=EDGE_CURVE('',#37622,#37623,#4703,.T.) ;
#46014=EDGE_CURVE('',#37623,#37621,#30502,.T.) ;
#46015=EDGE_CURVE('',#37622,#37624,#4704,.T.) ;
#46016=EDGE_CURVE('',#37624,#37625,#4705,.T.) ;
#46017=EDGE_CURVE('',#37625,#37623,#4706,.T.) ;
#46018=EDGE_CURVE('',#37624,#37626,#30503,.T.) ;
#46019=EDGE_CURVE('',#37626,#37627,#4707,.T.) ;
#46020=EDGE_CURVE('',#37627,#37625,#30504,.T.) ;
#46021=EDGE_CURVE('',#37626,#37628,#4708,.T.) ;
#46022=EDGE_CURVE('',#37628,#37629,#4709,.T.) ;
#46023=EDGE_CURVE('',#37629,#37627,#4710,.T.) ;
#46024=EDGE_CURVE('',#37628,#37630,#30505,.T.) ;
#46025=EDGE_CURVE('',#37630,#37631,#4711,.T.) ;
#46026=EDGE_CURVE('',#37631,#37629,#30506,.T.) ;
#46027=EDGE_CURVE('',#37630,#36240,#4712,.T.) ;
#46028=EDGE_CURVE('',#36240,#37632,#4713,.T.) ;
#46029=EDGE_CURVE('',#37632,#37631,#4714,.T.) ;
#46030=EDGE_CURVE('',#36241,#37633,#4715,.T.) ;
#46031=EDGE_CURVE('',#37633,#37632,#30507,.T.) ;
#46032=EDGE_CURVE('',#36241,#36371,#4716,.T.) ;
#46033=EDGE_CURVE('',#36335,#37633,#4717,.T.) ;
#46034=EDGE_CURVE('',#36372,#37634,#4718,.T.) ;
#46035=EDGE_CURVE('',#37634,#37635,#4719,.T.) ;
#46036=EDGE_CURVE('',#37635,#36336,#4720,.T.) ;
#46037=EDGE_CURVE('',#37634,#37636,#30508,.T.) ;
#46038=EDGE_CURVE('',#37636,#37637,#4721,.T.) ;
#46039=EDGE_CURVE('',#37637,#37635,#30509,.T.) ;
#46040=EDGE_CURVE('',#37636,#37638,#4722,.T.) ;
#46041=EDGE_CURVE('',#37638,#37639,#4723,.T.) ;
#46042=EDGE_CURVE('',#37639,#37637,#4724,.T.) ;
#46043=EDGE_CURVE('',#37638,#37640,#30510,.T.) ;
#46044=EDGE_CURVE('',#37640,#37641,#4725,.T.) ;
#46045=EDGE_CURVE('',#37641,#37639,#30511,.T.) ;
#46046=EDGE_CURVE('',#37640,#37642,#4726,.T.) ;
#46047=EDGE_CURVE('',#37642,#37643,#4727,.T.) ;
#46048=EDGE_CURVE('',#37643,#37641,#4728,.T.) ;
#46049=EDGE_CURVE('',#37642,#37644,#30512,.T.) ;
#46050=EDGE_CURVE('',#37644,#37645,#4729,.T.) ;
#46051=EDGE_CURVE('',#37645,#37643,#30513,.T.) ;
#46052=EDGE_CURVE('',#37644,#37646,#4730,.T.) ;
#46053=EDGE_CURVE('',#37646,#37647,#4731,.T.) ;
#46054=EDGE_CURVE('',#37647,#37645,#4732,.T.) ;
#46055=EDGE_CURVE('',#37646,#37648,#30514,.T.) ;
#46056=EDGE_CURVE('',#37648,#37649,#4733,.T.) ;
#46057=EDGE_CURVE('',#37649,#37647,#30515,.T.) ;
#46058=EDGE_CURVE('',#37648,#37650,#4734,.T.) ;
#46059=EDGE_CURVE('',#37650,#37651,#4735,.T.) ;
#46060=EDGE_CURVE('',#37651,#37649,#4736,.T.) ;
#46061=EDGE_CURVE('',#37650,#37652,#30516,.T.) ;
#46062=EDGE_CURVE('',#37652,#37653,#4737,.T.) ;
#46063=EDGE_CURVE('',#37653,#37651,#30517,.T.) ;
#46064=EDGE_CURVE('',#37652,#37654,#4738,.T.) ;
#46065=EDGE_CURVE('',#37654,#37655,#4739,.T.) ;
#46066=EDGE_CURVE('',#37655,#37653,#4740,.T.) ;
#46067=EDGE_CURVE('',#37654,#37656,#30518,.T.) ;
#46068=EDGE_CURVE('',#37656,#37657,#4741,.T.) ;
#46069=EDGE_CURVE('',#37657,#37655,#30519,.T.) ;
#46070=EDGE_CURVE('',#37656,#37658,#30520,.T.) ;
#46071=EDGE_CURVE('',#37658,#37659,#4742,.T.) ;
#46072=EDGE_CURVE('',#37659,#37657,#30521,.T.) ;
#46073=EDGE_CURVE('',#37658,#37660,#30522,.T.) ;
#46074=EDGE_CURVE('',#37660,#37661,#4743,.T.) ;
#46075=EDGE_CURVE('',#37661,#37659,#30523,.T.) ;
#46076=EDGE_CURVE('',#37660,#37662,#4744,.T.) ;
#46077=EDGE_CURVE('',#37662,#37663,#4745,.T.) ;
#46078=EDGE_CURVE('',#37663,#37661,#4746,.T.) ;
#46079=EDGE_CURVE('',#37662,#37664,#30524,.T.) ;
#46080=EDGE_CURVE('',#37664,#37665,#4747,.T.) ;
#46081=EDGE_CURVE('',#37665,#37663,#30525,.T.) ;
#46082=EDGE_CURVE('',#37664,#37666,#4748,.T.) ;
#46083=EDGE_CURVE('',#37666,#37667,#4749,.T.) ;
#46084=EDGE_CURVE('',#37667,#37665,#4750,.T.) ;
#46085=EDGE_CURVE('',#37666,#37668,#30526,.T.) ;
#46086=EDGE_CURVE('',#37668,#37669,#4751,.T.) ;
#46087=EDGE_CURVE('',#37669,#37667,#30527,.T.) ;
#46088=EDGE_CURVE('',#37668,#37620,#4752,.T.) ;
#46089=EDGE_CURVE('',#37621,#37669,#4753,.T.) ;
#46090=EDGE_CURVE('',#37670,#37671,#30528,.T.) ;
#46091=EDGE_CURVE('',#37671,#37672,#4754,.T.) ;
#46092=EDGE_CURVE('',#37672,#37673,#30529,.T.) ;
#46093=EDGE_CURVE('',#37673,#37674,#4755,.T.) ;
#46094=EDGE_CURVE('',#37674,#37675,#4756,.T.) ;
#46095=EDGE_CURVE('',#37675,#37676,#4757,.T.) ;
#46096=EDGE_CURVE('',#37676,#37677,#30530,.T.) ;
#46097=EDGE_CURVE('',#37677,#37678,#4758,.T.) ;
#46098=EDGE_CURVE('',#37678,#37679,#4759,.T.) ;
#46099=EDGE_CURVE('',#37679,#37680,#4760,.T.) ;
#46100=EDGE_CURVE('',#37680,#37681,#30531,.T.) ;
#46101=EDGE_CURVE('',#37681,#37682,#4761,.T.) ;
#46102=EDGE_CURVE('',#37682,#37683,#30532,.T.) ;
#46103=EDGE_CURVE('',#37683,#37684,#4762,.T.) ;
#46104=EDGE_CURVE('',#37684,#37685,#4763,.T.) ;
#46105=EDGE_CURVE('',#37685,#36242,#4764,.T.) ;
#46106=EDGE_CURVE('',#36242,#37686,#4765,.T.) ;
#46107=EDGE_CURVE('',#37686,#37670,#4766,.T.) ;
#46108=EDGE_CURVE('',#37687,#37688,#4767,.T.) ;
#46109=EDGE_CURVE('',#37687,#37689,#30533,.T.) ;
#46110=EDGE_CURVE('',#37689,#37690,#4768,.T.) ;
#46111=EDGE_CURVE('',#37690,#37688,#30534,.T.) ;
#46112=EDGE_CURVE('',#37689,#37691,#4769,.T.) ;
#46113=EDGE_CURVE('',#37691,#37692,#4770,.T.) ;
#46114=EDGE_CURVE('',#37692,#37690,#4771,.T.) ;
#46115=EDGE_CURVE('',#37691,#37693,#30535,.T.) ;
#46116=EDGE_CURVE('',#37693,#37694,#4772,.T.) ;
#46117=EDGE_CURVE('',#37694,#37692,#30536,.T.) ;
#46118=EDGE_CURVE('',#37693,#37695,#4773,.T.) ;
#46119=EDGE_CURVE('',#37695,#37696,#4774,.T.) ;
#46120=EDGE_CURVE('',#37696,#37694,#4775,.T.) ;
#46121=EDGE_CURVE('',#37695,#37697,#30537,.T.) ;
#46122=EDGE_CURVE('',#37697,#37698,#4776,.T.) ;
#46123=EDGE_CURVE('',#37698,#37696,#30538,.T.) ;
#46124=EDGE_CURVE('',#37697,#36255,#4777,.T.) ;
#46125=EDGE_CURVE('',#36255,#37699,#4778,.T.) ;
#46126=EDGE_CURVE('',#37699,#37698,#4779,.T.) ;
#46127=EDGE_CURVE('',#36256,#37700,#4780,.T.) ;
#46128=EDGE_CURVE('',#37700,#37699,#30539,.T.) ;
#46129=EDGE_CURVE('',#36256,#36369,#4781,.T.) ;
#46130=EDGE_CURVE('',#36331,#37700,#4782,.T.) ;
#46131=EDGE_CURVE('',#36370,#37701,#4783,.T.) ;
#46132=EDGE_CURVE('',#37701,#37702,#4784,.T.) ;
#46133=EDGE_CURVE('',#37702,#36332,#4785,.T.) ;
#46134=EDGE_CURVE('',#37701,#37703,#30540,.T.) ;
#46135=EDGE_CURVE('',#37703,#37704,#4786,.T.) ;
#46136=EDGE_CURVE('',#37704,#37702,#30541,.T.) ;
#46137=EDGE_CURVE('',#37703,#37705,#4787,.T.) ;
#46138=EDGE_CURVE('',#37705,#37706,#4788,.T.) ;
#46139=EDGE_CURVE('',#37706,#37704,#4789,.T.) ;
#46140=EDGE_CURVE('',#37705,#37707,#30542,.T.) ;
#46141=EDGE_CURVE('',#37707,#37708,#4790,.T.) ;
#46142=EDGE_CURVE('',#37708,#37706,#30543,.T.) ;
#46143=EDGE_CURVE('',#37707,#37709,#4791,.T.) ;
#46144=EDGE_CURVE('',#37709,#37710,#4792,.T.) ;
#46145=EDGE_CURVE('',#37710,#37708,#4793,.T.) ;
#46146=EDGE_CURVE('',#37709,#37711,#30544,.T.) ;
#46147=EDGE_CURVE('',#37711,#37712,#4794,.T.) ;
#46148=EDGE_CURVE('',#37712,#37710,#30545,.T.) ;
#46149=EDGE_CURVE('',#37711,#37713,#4795,.T.) ;
#46150=EDGE_CURVE('',#37713,#37714,#4796,.T.) ;
#46151=EDGE_CURVE('',#37714,#37712,#4797,.T.) ;
#46152=EDGE_CURVE('',#37713,#37715,#30546,.T.) ;
#46153=EDGE_CURVE('',#37715,#37716,#4798,.T.) ;
#46154=EDGE_CURVE('',#37716,#37714,#30547,.T.) ;
#46155=EDGE_CURVE('',#37715,#37717,#4799,.T.) ;
#46156=EDGE_CURVE('',#37717,#37718,#4800,.T.) ;
#46157=EDGE_CURVE('',#37718,#37716,#4801,.T.) ;
#46158=EDGE_CURVE('',#37717,#37719,#30548,.T.) ;
#46159=EDGE_CURVE('',#37719,#37720,#4802,.T.) ;
#46160=EDGE_CURVE('',#37720,#37718,#30549,.T.) ;
#46161=EDGE_CURVE('',#37719,#37721,#4803,.T.) ;
#46162=EDGE_CURVE('',#37721,#37722,#4804,.T.) ;
#46163=EDGE_CURVE('',#37722,#37720,#4805,.T.) ;
#46164=EDGE_CURVE('',#37721,#37723,#30550,.T.) ;
#46165=EDGE_CURVE('',#37723,#37724,#4806,.T.) ;
#46166=EDGE_CURVE('',#37724,#37722,#30551,.T.) ;
#46167=EDGE_CURVE('',#37723,#37725,#30552,.T.) ;
#46168=EDGE_CURVE('',#37725,#37726,#4807,.T.) ;
#46169=EDGE_CURVE('',#37726,#37724,#30553,.T.) ;
#46170=EDGE_CURVE('',#37725,#37727,#30554,.T.) ;
#46171=EDGE_CURVE('',#37727,#37728,#4808,.T.) ;
#46172=EDGE_CURVE('',#37728,#37726,#30555,.T.) ;
#46173=EDGE_CURVE('',#37727,#37729,#4809,.T.) ;
#46174=EDGE_CURVE('',#37729,#37730,#4810,.T.) ;
#46175=EDGE_CURVE('',#37730,#37728,#4811,.T.) ;
#46176=EDGE_CURVE('',#37729,#37731,#30556,.T.) ;
#46177=EDGE_CURVE('',#37731,#37732,#4812,.T.) ;
#46178=EDGE_CURVE('',#37732,#37730,#30557,.T.) ;
#46179=EDGE_CURVE('',#37731,#37733,#4813,.T.) ;
#46180=EDGE_CURVE('',#37733,#37734,#4814,.T.) ;
#46181=EDGE_CURVE('',#37734,#37732,#4815,.T.) ;
#46182=EDGE_CURVE('',#37733,#37735,#30558,.T.) ;
#46183=EDGE_CURVE('',#37735,#37736,#4816,.T.) ;
#46184=EDGE_CURVE('',#37736,#37734,#30559,.T.) ;
#46185=EDGE_CURVE('',#37735,#37687,#4817,.T.) ;
#46186=EDGE_CURVE('',#37688,#37736,#4818,.T.) ;
#46187=EDGE_CURVE('',#37737,#37738,#30560,.T.) ;
#46188=EDGE_CURVE('',#37738,#37739,#4819,.T.) ;
#46189=EDGE_CURVE('',#37739,#37740,#30561,.T.) ;
#46190=EDGE_CURVE('',#37740,#37741,#4820,.T.) ;
#46191=EDGE_CURVE('',#37741,#37742,#4821,.T.) ;
#46192=EDGE_CURVE('',#37742,#37743,#4822,.T.) ;
#46193=EDGE_CURVE('',#37743,#37744,#30562,.T.) ;
#46194=EDGE_CURVE('',#37744,#37745,#4823,.T.) ;
#46195=EDGE_CURVE('',#37745,#37746,#4824,.T.) ;
#46196=EDGE_CURVE('',#37746,#37747,#4825,.T.) ;
#46197=EDGE_CURVE('',#37747,#37748,#30563,.T.) ;
#46198=EDGE_CURVE('',#37748,#37749,#4826,.T.) ;
#46199=EDGE_CURVE('',#37749,#37750,#30564,.T.) ;
#46200=EDGE_CURVE('',#37750,#37751,#4827,.T.) ;
#46201=EDGE_CURVE('',#37751,#37752,#4828,.T.) ;
#46202=EDGE_CURVE('',#37752,#36257,#4829,.T.) ;
#46203=EDGE_CURVE('',#36257,#37753,#4830,.T.) ;
#46204=EDGE_CURVE('',#37753,#37737,#4831,.T.) ;
#46205=EDGE_CURVE('',#37754,#37755,#4832,.T.) ;
#46206=EDGE_CURVE('',#37754,#37756,#30565,.T.) ;
#46207=EDGE_CURVE('',#37756,#37757,#4833,.T.) ;
#46208=EDGE_CURVE('',#37757,#37755,#30566,.T.) ;
#46209=EDGE_CURVE('',#37756,#37758,#4834,.T.) ;
#46210=EDGE_CURVE('',#37758,#37759,#4835,.T.) ;
#46211=EDGE_CURVE('',#37759,#37757,#4836,.T.) ;
#46212=EDGE_CURVE('',#37758,#37760,#30567,.T.) ;
#46213=EDGE_CURVE('',#37760,#37761,#4837,.T.) ;
#46214=EDGE_CURVE('',#37761,#37759,#30568,.T.) ;
#46215=EDGE_CURVE('',#37760,#37762,#4838,.T.) ;
#46216=EDGE_CURVE('',#37762,#37763,#4839,.T.) ;
#46217=EDGE_CURVE('',#37763,#37761,#4840,.T.) ;
#46218=EDGE_CURVE('',#37762,#37764,#30569,.T.) ;
#46219=EDGE_CURVE('',#37764,#37765,#4841,.T.) ;
#46220=EDGE_CURVE('',#37765,#37763,#30570,.T.) ;
#46221=EDGE_CURVE('',#37764,#36270,#4842,.T.) ;
#46222=EDGE_CURVE('',#36270,#37766,#4843,.T.) ;
#46223=EDGE_CURVE('',#37766,#37765,#4844,.T.) ;
#46224=EDGE_CURVE('',#36271,#37767,#4845,.T.) ;
#46225=EDGE_CURVE('',#37767,#37766,#30571,.T.) ;
#46226=EDGE_CURVE('',#36271,#36367,#4846,.T.) ;
#46227=EDGE_CURVE('',#36327,#37767,#4847,.T.) ;
#46228=EDGE_CURVE('',#36368,#37768,#4848,.T.) ;
#46229=EDGE_CURVE('',#37768,#37769,#4849,.T.) ;
#46230=EDGE_CURVE('',#37769,#36328,#4850,.T.) ;
#46231=EDGE_CURVE('',#37768,#37770,#30572,.T.) ;
#46232=EDGE_CURVE('',#37770,#37771,#4851,.T.) ;
#46233=EDGE_CURVE('',#37771,#37769,#30573,.T.) ;
#46234=EDGE_CURVE('',#37770,#37772,#4852,.T.) ;
#46235=EDGE_CURVE('',#37772,#37773,#4853,.T.) ;
#46236=EDGE_CURVE('',#37773,#37771,#4854,.T.) ;
#46237=EDGE_CURVE('',#37772,#37774,#30574,.T.) ;
#46238=EDGE_CURVE('',#37774,#37775,#4855,.T.) ;
#46239=EDGE_CURVE('',#37775,#37773,#30575,.T.) ;
#46240=EDGE_CURVE('',#37774,#37776,#4856,.T.) ;
#46241=EDGE_CURVE('',#37776,#37777,#4857,.T.) ;
#46242=EDGE_CURVE('',#37777,#37775,#4858,.T.) ;
#46243=EDGE_CURVE('',#37776,#37778,#30576,.T.) ;
#46244=EDGE_CURVE('',#37778,#37779,#4859,.T.) ;
#46245=EDGE_CURVE('',#37779,#37777,#30577,.T.) ;
#46246=EDGE_CURVE('',#37778,#37780,#4860,.T.) ;
#46247=EDGE_CURVE('',#37780,#37781,#4861,.T.) ;
#46248=EDGE_CURVE('',#37781,#37779,#4862,.T.) ;
#46249=EDGE_CURVE('',#37780,#37782,#30578,.T.) ;
#46250=EDGE_CURVE('',#37782,#37783,#4863,.T.) ;
#46251=EDGE_CURVE('',#37783,#37781,#30579,.T.) ;
#46252=EDGE_CURVE('',#37782,#37784,#4864,.T.) ;
#46253=EDGE_CURVE('',#37784,#37785,#4865,.T.) ;
#46254=EDGE_CURVE('',#37785,#37783,#4866,.T.) ;
#46255=EDGE_CURVE('',#37784,#37786,#30580,.T.) ;
#46256=EDGE_CURVE('',#37786,#37787,#4867,.T.) ;
#46257=EDGE_CURVE('',#37787,#37785,#30581,.T.) ;
#46258=EDGE_CURVE('',#37786,#37788,#4868,.T.) ;
#46259=EDGE_CURVE('',#37788,#37789,#4869,.T.) ;
#46260=EDGE_CURVE('',#37789,#37787,#4870,.T.) ;
#46261=EDGE_CURVE('',#37788,#37790,#30582,.T.) ;
#46262=EDGE_CURVE('',#37790,#37791,#4871,.T.) ;
#46263=EDGE_CURVE('',#37791,#37789,#30583,.T.) ;
#46264=EDGE_CURVE('',#37790,#37792,#30584,.T.) ;
#46265=EDGE_CURVE('',#37792,#37793,#4872,.T.) ;
#46266=EDGE_CURVE('',#37793,#37791,#30585,.T.) ;
#46267=EDGE_CURVE('',#37792,#37794,#30586,.T.) ;
#46268=EDGE_CURVE('',#37794,#37795,#4873,.T.) ;
#46269=EDGE_CURVE('',#37795,#37793,#30587,.T.) ;
#46270=EDGE_CURVE('',#37794,#37796,#4874,.T.) ;
#46271=EDGE_CURVE('',#37796,#37797,#4875,.T.) ;
#46272=EDGE_CURVE('',#37797,#37795,#4876,.T.) ;
#46273=EDGE_CURVE('',#37796,#37798,#30588,.T.) ;
#46274=EDGE_CURVE('',#37798,#37799,#4877,.T.) ;
#46275=EDGE_CURVE('',#37799,#37797,#30589,.T.) ;
#46276=EDGE_CURVE('',#37798,#37800,#4878,.T.) ;
#46277=EDGE_CURVE('',#37800,#37801,#4879,.T.) ;
#46278=EDGE_CURVE('',#37801,#37799,#4880,.T.) ;
#46279=EDGE_CURVE('',#37800,#37802,#30590,.T.) ;
#46280=EDGE_CURVE('',#37802,#37803,#4881,.T.) ;
#46281=EDGE_CURVE('',#37803,#37801,#30591,.T.) ;
#46282=EDGE_CURVE('',#37802,#37754,#4882,.T.) ;
#46283=EDGE_CURVE('',#37755,#37803,#4883,.T.) ;
#46284=EDGE_CURVE('',#37804,#37805,#30592,.T.) ;
#46285=EDGE_CURVE('',#37805,#37806,#4884,.T.) ;
#46286=EDGE_CURVE('',#37806,#37807,#30593,.T.) ;
#46287=EDGE_CURVE('',#37807,#37808,#4885,.T.) ;
#46288=EDGE_CURVE('',#37808,#37809,#4886,.T.) ;
#46289=EDGE_CURVE('',#37809,#37810,#4887,.T.) ;
#46290=EDGE_CURVE('',#37810,#37811,#30594,.T.) ;
#46291=EDGE_CURVE('',#37811,#37812,#4888,.T.) ;
#46292=EDGE_CURVE('',#37812,#37813,#4889,.T.) ;
#46293=EDGE_CURVE('',#37813,#37814,#4890,.T.) ;
#46294=EDGE_CURVE('',#37814,#37815,#30595,.T.) ;
#46295=EDGE_CURVE('',#37815,#37816,#4891,.T.) ;
#46296=EDGE_CURVE('',#37816,#37817,#30596,.T.) ;
#46297=EDGE_CURVE('',#37817,#37818,#4892,.T.) ;
#46298=EDGE_CURVE('',#37818,#37819,#4893,.T.) ;
#46299=EDGE_CURVE('',#37819,#36272,#4894,.T.) ;
#46300=EDGE_CURVE('',#36272,#37820,#4895,.T.) ;
#46301=EDGE_CURVE('',#37820,#37804,#4896,.T.) ;
#46302=EDGE_CURVE('',#37821,#37822,#4897,.T.) ;
#46303=EDGE_CURVE('',#37821,#37823,#30597,.T.) ;
#46304=EDGE_CURVE('',#37823,#37824,#4898,.T.) ;
#46305=EDGE_CURVE('',#37824,#37822,#30598,.T.) ;
#46306=EDGE_CURVE('',#37823,#37825,#4899,.T.) ;
#46307=EDGE_CURVE('',#37825,#37826,#4900,.T.) ;
#46308=EDGE_CURVE('',#37826,#37824,#4901,.T.) ;
#46309=EDGE_CURVE('',#37825,#37827,#30599,.T.) ;
#46310=EDGE_CURVE('',#37827,#37828,#4902,.T.) ;
#46311=EDGE_CURVE('',#37828,#37826,#30600,.T.) ;
#46312=EDGE_CURVE('',#37827,#37829,#4903,.T.) ;
#46313=EDGE_CURVE('',#37829,#37830,#4904,.T.) ;
#46314=EDGE_CURVE('',#37830,#37828,#4905,.T.) ;
#46315=EDGE_CURVE('',#37829,#37831,#30601,.T.) ;
#46316=EDGE_CURVE('',#37831,#37832,#4906,.T.) ;
#46317=EDGE_CURVE('',#37832,#37830,#30602,.T.) ;
#46318=EDGE_CURVE('',#37831,#36285,#4907,.T.) ;
#46319=EDGE_CURVE('',#36285,#37833,#4908,.T.) ;
#46320=EDGE_CURVE('',#37833,#37832,#4909,.T.) ;
#46321=EDGE_CURVE('',#36286,#37834,#4910,.T.) ;
#46322=EDGE_CURVE('',#37834,#37833,#30603,.T.) ;
#46323=EDGE_CURVE('',#36286,#36365,#4911,.T.) ;
#46324=EDGE_CURVE('',#36323,#37834,#4912,.T.) ;
#46325=EDGE_CURVE('',#36366,#37835,#4913,.T.) ;
#46326=EDGE_CURVE('',#37835,#37836,#4914,.T.) ;
#46327=EDGE_CURVE('',#37836,#36324,#4915,.T.) ;
#46328=EDGE_CURVE('',#37835,#37837,#30604,.T.) ;
#46329=EDGE_CURVE('',#37837,#37838,#4916,.T.) ;
#46330=EDGE_CURVE('',#37838,#37836,#30605,.T.) ;
#46331=EDGE_CURVE('',#37837,#37839,#4917,.T.) ;
#46332=EDGE_CURVE('',#37839,#37840,#4918,.T.) ;
#46333=EDGE_CURVE('',#37840,#37838,#4919,.T.) ;
#46334=EDGE_CURVE('',#37839,#37841,#30606,.T.) ;
#46335=EDGE_CURVE('',#37841,#37842,#4920,.T.) ;
#46336=EDGE_CURVE('',#37842,#37840,#30607,.T.) ;
#46337=EDGE_CURVE('',#37841,#37843,#4921,.T.) ;
#46338=EDGE_CURVE('',#37843,#37844,#4922,.T.) ;
#46339=EDGE_CURVE('',#37844,#37842,#4923,.T.) ;
#46340=EDGE_CURVE('',#37843,#37845,#30608,.T.) ;
#46341=EDGE_CURVE('',#37845,#37846,#4924,.T.) ;
#46342=EDGE_CURVE('',#37846,#37844,#30609,.T.) ;
#46343=EDGE_CURVE('',#37845,#37847,#4925,.T.) ;
#46344=EDGE_CURVE('',#37847,#37848,#4926,.T.) ;
#46345=EDGE_CURVE('',#37848,#37846,#4927,.T.) ;
#46346=EDGE_CURVE('',#37847,#37849,#30610,.T.) ;
#46347=EDGE_CURVE('',#37849,#37850,#4928,.T.) ;
#46348=EDGE_CURVE('',#37850,#37848,#30611,.T.) ;
#46349=EDGE_CURVE('',#37849,#37851,#4929,.T.) ;
#46350=EDGE_CURVE('',#37851,#37852,#4930,.T.) ;
#46351=EDGE_CURVE('',#37852,#37850,#4931,.T.) ;
#46352=EDGE_CURVE('',#37851,#37853,#30612,.T.) ;
#46353=EDGE_CURVE('',#37853,#37854,#4932,.T.) ;
#46354=EDGE_CURVE('',#37854,#37852,#30613,.T.) ;
#46355=EDGE_CURVE('',#37853,#37855,#4933,.T.) ;
#46356=EDGE_CURVE('',#37855,#37856,#4934,.T.) ;
#46357=EDGE_CURVE('',#37856,#37854,#4935,.T.) ;
#46358=EDGE_CURVE('',#37855,#37857,#30614,.T.) ;
#46359=EDGE_CURVE('',#37857,#37858,#4936,.T.) ;
#46360=EDGE_CURVE('',#37858,#37856,#30615,.T.) ;
#46361=EDGE_CURVE('',#37857,#37859,#30616,.T.) ;
#46362=EDGE_CURVE('',#37859,#37860,#4937,.T.) ;
#46363=EDGE_CURVE('',#37860,#37858,#30617,.T.) ;
#46364=EDGE_CURVE('',#37859,#37861,#30618,.T.) ;
#46365=EDGE_CURVE('',#37861,#37862,#4938,.T.) ;
#46366=EDGE_CURVE('',#37862,#37860,#30619,.T.) ;
#46367=EDGE_CURVE('',#37861,#37863,#4939,.T.) ;
#46368=EDGE_CURVE('',#37863,#37864,#4940,.T.) ;
#46369=EDGE_CURVE('',#37864,#37862,#4941,.T.) ;
#46370=EDGE_CURVE('',#37863,#37865,#30620,.T.) ;
#46371=EDGE_CURVE('',#37865,#37866,#4942,.T.) ;
#46372=EDGE_CURVE('',#37866,#37864,#30621,.T.) ;
#46373=EDGE_CURVE('',#37865,#37867,#4943,.T.) ;
#46374=EDGE_CURVE('',#37867,#37868,#4944,.T.) ;
#46375=EDGE_CURVE('',#37868,#37866,#4945,.T.) ;
#46376=EDGE_CURVE('',#37867,#37869,#30622,.T.) ;
#46377=EDGE_CURVE('',#37869,#37870,#4946,.T.) ;
#46378=EDGE_CURVE('',#37870,#37868,#30623,.T.) ;
#46379=EDGE_CURVE('',#37869,#37821,#4947,.T.) ;
#46380=EDGE_CURVE('',#37822,#37870,#4948,.T.) ;
#46381=EDGE_CURVE('',#37871,#37872,#30624,.T.) ;
#46382=EDGE_CURVE('',#37872,#37873,#4949,.T.) ;
#46383=EDGE_CURVE('',#37873,#37874,#30625,.T.) ;
#46384=EDGE_CURVE('',#37874,#37875,#4950,.T.) ;
#46385=EDGE_CURVE('',#37875,#37876,#4951,.T.) ;
#46386=EDGE_CURVE('',#37876,#37877,#4952,.T.) ;
#46387=EDGE_CURVE('',#37877,#37878,#30626,.T.) ;
#46388=EDGE_CURVE('',#37878,#37879,#4953,.T.) ;
#46389=EDGE_CURVE('',#37879,#37880,#4954,.T.) ;
#46390=EDGE_CURVE('',#37880,#37881,#4955,.T.) ;
#46391=EDGE_CURVE('',#37881,#37882,#30627,.T.) ;
#46392=EDGE_CURVE('',#37882,#37883,#4956,.T.) ;
#46393=EDGE_CURVE('',#37883,#37884,#30628,.T.) ;
#46394=EDGE_CURVE('',#37884,#37885,#4957,.T.) ;
#46395=EDGE_CURVE('',#37885,#37886,#4958,.T.) ;
#46396=EDGE_CURVE('',#37886,#36287,#4959,.T.) ;
#46397=EDGE_CURVE('',#36287,#37887,#4960,.T.) ;
#46398=EDGE_CURVE('',#37887,#37871,#4961,.T.) ;
#46399=EDGE_CURVE('',#37888,#37889,#4962,.T.) ;
#46400=EDGE_CURVE('',#37888,#37890,#30629,.T.) ;
#46401=EDGE_CURVE('',#37890,#37891,#4963,.T.) ;
#46402=EDGE_CURVE('',#37891,#37889,#30630,.T.) ;
#46403=EDGE_CURVE('',#37890,#37892,#4964,.T.) ;
#46404=EDGE_CURVE('',#37892,#37893,#4965,.T.) ;
#46405=EDGE_CURVE('',#37893,#37891,#4966,.T.) ;
#46406=EDGE_CURVE('',#37892,#37894,#30631,.T.) ;
#46407=EDGE_CURVE('',#37894,#37895,#4967,.T.) ;
#46408=EDGE_CURVE('',#37895,#37893,#30632,.T.) ;
#46409=EDGE_CURVE('',#37894,#37896,#4968,.T.) ;
#46410=EDGE_CURVE('',#37896,#37897,#4969,.T.) ;
#46411=EDGE_CURVE('',#37897,#37895,#4970,.T.) ;
#46412=EDGE_CURVE('',#37896,#37898,#30633,.T.) ;
#46413=EDGE_CURVE('',#37898,#37899,#4971,.T.) ;
#46414=EDGE_CURVE('',#37899,#37897,#30634,.T.) ;
#46415=EDGE_CURVE('',#37898,#36300,#4972,.T.) ;
#46416=EDGE_CURVE('',#36300,#37900,#4973,.T.) ;
#46417=EDGE_CURVE('',#37900,#37899,#4974,.T.) ;
#46418=EDGE_CURVE('',#36301,#37901,#4975,.T.) ;
#46419=EDGE_CURVE('',#37901,#37900,#30635,.T.) ;
#46420=EDGE_CURVE('',#36301,#36363,#4976,.T.) ;
#46421=EDGE_CURVE('',#36319,#37901,#4977,.T.) ;
#46422=EDGE_CURVE('',#36364,#37902,#4978,.T.) ;
#46423=EDGE_CURVE('',#37902,#37903,#4979,.T.) ;
#46424=EDGE_CURVE('',#37903,#36320,#4980,.T.) ;
#46425=EDGE_CURVE('',#37902,#37904,#30636,.T.) ;
#46426=EDGE_CURVE('',#37904,#37905,#4981,.T.) ;
#46427=EDGE_CURVE('',#37905,#37903,#30637,.T.) ;
#46428=EDGE_CURVE('',#37904,#37906,#4982,.T.) ;
#46429=EDGE_CURVE('',#37906,#37907,#4983,.T.) ;
#46430=EDGE_CURVE('',#37907,#37905,#4984,.T.) ;
#46431=EDGE_CURVE('',#37906,#37908,#30638,.T.) ;
#46432=EDGE_CURVE('',#37908,#37909,#4985,.T.) ;
#46433=EDGE_CURVE('',#37909,#37907,#30639,.T.) ;
#46434=EDGE_CURVE('',#37908,#37910,#4986,.T.) ;
#46435=EDGE_CURVE('',#37910,#37911,#4987,.T.) ;
#46436=EDGE_CURVE('',#37911,#37909,#4988,.T.) ;
#46437=EDGE_CURVE('',#37910,#37912,#30640,.T.) ;
#46438=EDGE_CURVE('',#37912,#37913,#4989,.T.) ;
#46439=EDGE_CURVE('',#37913,#37911,#30641,.T.) ;
#46440=EDGE_CURVE('',#37912,#37914,#4990,.T.) ;
#46441=EDGE_CURVE('',#37914,#37915,#4991,.T.) ;
#46442=EDGE_CURVE('',#37915,#37913,#4992,.T.) ;
#46443=EDGE_CURVE('',#37914,#37916,#30642,.T.) ;
#46444=EDGE_CURVE('',#37916,#37917,#4993,.T.) ;
#46445=EDGE_CURVE('',#37917,#37915,#30643,.T.) ;
#46446=EDGE_CURVE('',#37916,#37918,#4994,.T.) ;
#46447=EDGE_CURVE('',#37918,#37919,#4995,.T.) ;
#46448=EDGE_CURVE('',#37919,#37917,#4996,.T.) ;
#46449=EDGE_CURVE('',#37918,#37920,#30644,.T.) ;
#46450=EDGE_CURVE('',#37920,#37921,#4997,.T.) ;
#46451=EDGE_CURVE('',#37921,#37919,#30645,.T.) ;
#46452=EDGE_CURVE('',#37920,#37922,#4998,.T.) ;
#46453=EDGE_CURVE('',#37922,#37923,#4999,.T.) ;
#46454=EDGE_CURVE('',#37923,#37921,#5000,.T.) ;
#46455=EDGE_CURVE('',#37922,#37924,#30646,.T.) ;
#46456=EDGE_CURVE('',#37924,#37925,#5001,.T.) ;
#46457=EDGE_CURVE('',#37925,#37923,#30647,.T.) ;
#46458=EDGE_CURVE('',#37924,#37926,#30648,.T.) ;
#46459=EDGE_CURVE('',#37926,#37927,#5002,.T.) ;
#46460=EDGE_CURVE('',#37927,#37925,#30649,.T.) ;
#46461=EDGE_CURVE('',#37926,#37928,#30650,.T.) ;
#46462=EDGE_CURVE('',#37928,#37929,#5003,.T.) ;
#46463=EDGE_CURVE('',#37929,#37927,#30651,.T.) ;
#46464=EDGE_CURVE('',#37928,#37930,#5004,.T.) ;
#46465=EDGE_CURVE('',#37930,#37931,#5005,.T.) ;
#46466=EDGE_CURVE('',#37931,#37929,#5006,.T.) ;
#46467=EDGE_CURVE('',#37930,#37932,#30652,.T.) ;
#46468=EDGE_CURVE('',#37932,#37933,#5007,.T.) ;
#46469=EDGE_CURVE('',#37933,#37931,#30653,.T.) ;
#46470=EDGE_CURVE('',#37932,#37934,#5008,.T.) ;
#46471=EDGE_CURVE('',#37934,#37935,#5009,.T.) ;
#46472=EDGE_CURVE('',#37935,#37933,#5010,.T.) ;
#46473=EDGE_CURVE('',#37934,#37936,#30654,.T.) ;
#46474=EDGE_CURVE('',#37936,#37937,#5011,.T.) ;
#46475=EDGE_CURVE('',#37937,#37935,#30655,.T.) ;
#46476=EDGE_CURVE('',#37936,#37888,#5012,.T.) ;
#46477=EDGE_CURVE('',#37889,#37937,#5013,.T.) ;
#46478=EDGE_CURVE('',#37938,#37939,#30656,.T.) ;
#46479=EDGE_CURVE('',#37939,#37940,#5014,.T.) ;
#46480=EDGE_CURVE('',#37940,#37941,#30657,.T.) ;
#46481=EDGE_CURVE('',#37941,#37942,#5015,.T.) ;
#46482=EDGE_CURVE('',#37942,#37943,#5016,.T.) ;
#46483=EDGE_CURVE('',#37943,#37944,#5017,.T.) ;
#46484=EDGE_CURVE('',#37944,#37945,#30658,.T.) ;
#46485=EDGE_CURVE('',#37945,#37946,#5018,.T.) ;
#46486=EDGE_CURVE('',#37946,#37947,#5019,.T.) ;
#46487=EDGE_CURVE('',#37947,#37948,#5020,.T.) ;
#46488=EDGE_CURVE('',#37948,#37949,#30659,.T.) ;
#46489=EDGE_CURVE('',#37949,#37950,#5021,.T.) ;
#46490=EDGE_CURVE('',#37950,#37951,#30660,.T.) ;
#46491=EDGE_CURVE('',#37951,#37952,#5022,.T.) ;
#46492=EDGE_CURVE('',#37952,#37953,#5023,.T.) ;
#46493=EDGE_CURVE('',#37953,#36302,#5024,.T.) ;
#46494=EDGE_CURVE('',#36302,#37954,#5025,.T.) ;
#46495=EDGE_CURVE('',#37954,#37938,#5026,.T.) ;
#46496=EDGE_CURVE('',#37955,#37956,#5027,.T.) ;
#46497=EDGE_CURVE('',#37955,#37957,#30661,.T.) ;
#46498=EDGE_CURVE('',#37957,#37958,#5028,.T.) ;
#46499=EDGE_CURVE('',#37958,#37956,#30662,.T.) ;
#46500=EDGE_CURVE('',#37957,#37959,#5029,.T.) ;
#46501=EDGE_CURVE('',#37959,#37960,#5030,.T.) ;
#46502=EDGE_CURVE('',#37960,#37958,#5031,.T.) ;
#46503=EDGE_CURVE('',#37959,#37961,#30663,.T.) ;
#46504=EDGE_CURVE('',#37961,#37962,#5032,.T.) ;
#46505=EDGE_CURVE('',#37962,#37960,#30664,.T.) ;
#46506=EDGE_CURVE('',#37961,#37963,#5033,.T.) ;
#46507=EDGE_CURVE('',#37963,#37964,#5034,.T.) ;
#46508=EDGE_CURVE('',#37964,#37962,#5035,.T.) ;
#46509=EDGE_CURVE('',#37963,#37965,#30665,.T.) ;
#46510=EDGE_CURVE('',#37965,#37966,#5036,.T.) ;
#46511=EDGE_CURVE('',#37966,#37964,#30666,.T.) ;
#46512=EDGE_CURVE('',#37965,#36351,#5037,.T.) ;
#46513=EDGE_CURVE('',#36351,#37967,#5038,.T.) ;
#46514=EDGE_CURVE('',#37967,#37966,#5039,.T.) ;
#46515=EDGE_CURVE('',#36352,#37968,#5040,.T.) ;
#46516=EDGE_CURVE('',#37968,#37967,#30667,.T.) ;
#46517=EDGE_CURVE('',#36352,#36361,#5041,.T.) ;
#46518=EDGE_CURVE('',#36315,#37968,#5042,.T.) ;
#46519=EDGE_CURVE('',#36362,#37969,#5043,.T.) ;
#46520=EDGE_CURVE('',#37969,#37970,#5044,.T.) ;
#46521=EDGE_CURVE('',#37970,#36316,#5045,.T.) ;
#46522=EDGE_CURVE('',#37969,#37971,#30668,.T.) ;
#46523=EDGE_CURVE('',#37971,#37972,#5046,.T.) ;
#46524=EDGE_CURVE('',#37972,#37970,#30669,.T.) ;
#46525=EDGE_CURVE('',#37971,#37973,#5047,.T.) ;
#46526=EDGE_CURVE('',#37973,#37974,#5048,.T.) ;
#46527=EDGE_CURVE('',#37974,#37972,#5049,.T.) ;
#46528=EDGE_CURVE('',#37973,#37975,#30670,.T.) ;
#46529=EDGE_CURVE('',#37975,#37976,#5050,.T.) ;
#46530=EDGE_CURVE('',#37976,#37974,#30671,.T.) ;
#46531=EDGE_CURVE('',#37975,#37977,#5051,.T.) ;
#46532=EDGE_CURVE('',#37977,#37978,#5052,.T.) ;
#46533=EDGE_CURVE('',#37978,#37976,#5053,.T.) ;
#46534=EDGE_CURVE('',#37977,#37979,#30672,.T.) ;
#46535=EDGE_CURVE('',#37979,#37980,#5054,.T.) ;
#46536=EDGE_CURVE('',#37980,#37978,#30673,.T.) ;
#46537=EDGE_CURVE('',#37979,#37981,#5055,.T.) ;
#46538=EDGE_CURVE('',#37981,#37982,#5056,.T.) ;
#46539=EDGE_CURVE('',#37982,#37980,#5057,.T.) ;
#46540=EDGE_CURVE('',#37981,#37983,#30674,.T.) ;
#46541=EDGE_CURVE('',#37983,#37984,#5058,.T.) ;
#46542=EDGE_CURVE('',#37984,#37982,#30675,.T.) ;
#46543=EDGE_CURVE('',#37983,#37985,#5059,.T.) ;
#46544=EDGE_CURVE('',#37985,#37986,#5060,.T.) ;
#46545=EDGE_CURVE('',#37986,#37984,#5061,.T.) ;
#46546=EDGE_CURVE('',#37985,#37987,#30676,.T.) ;
#46547=EDGE_CURVE('',#37987,#37988,#5062,.T.) ;
#46548=EDGE_CURVE('',#37988,#37986,#30677,.T.) ;
#46549=EDGE_CURVE('',#37987,#37989,#5063,.T.) ;
#46550=EDGE_CURVE('',#37989,#37990,#5064,.T.) ;
#46551=EDGE_CURVE('',#37990,#37988,#5065,.T.) ;
#46552=EDGE_CURVE('',#37989,#37991,#30678,.T.) ;
#46553=EDGE_CURVE('',#37991,#37992,#5066,.T.) ;
#46554=EDGE_CURVE('',#37992,#37990,#30679,.T.) ;
#46555=EDGE_CURVE('',#37991,#37993,#30680,.T.) ;
#46556=EDGE_CURVE('',#37993,#37994,#5067,.T.) ;
#46557=EDGE_CURVE('',#37994,#37992,#30681,.T.) ;
#46558=EDGE_CURVE('',#37993,#37995,#30682,.T.) ;
#46559=EDGE_CURVE('',#37995,#37996,#5068,.T.) ;
#46560=EDGE_CURVE('',#37996,#37994,#30683,.T.) ;
#46561=EDGE_CURVE('',#37995,#37997,#5069,.T.) ;
#46562=EDGE_CURVE('',#37997,#37998,#5070,.T.) ;
#46563=EDGE_CURVE('',#37998,#37996,#5071,.T.) ;
#46564=EDGE_CURVE('',#37997,#37999,#30684,.T.) ;
#46565=EDGE_CURVE('',#37999,#38000,#5072,.T.) ;
#46566=EDGE_CURVE('',#38000,#37998,#30685,.T.) ;
#46567=EDGE_CURVE('',#37999,#38001,#5073,.T.) ;
#46568=EDGE_CURVE('',#38001,#38002,#5074,.T.) ;
#46569=EDGE_CURVE('',#38002,#38000,#5075,.T.) ;
#46570=EDGE_CURVE('',#38001,#38003,#30686,.T.) ;
#46571=EDGE_CURVE('',#38003,#38004,#5076,.T.) ;
#46572=EDGE_CURVE('',#38004,#38002,#30687,.T.) ;
#46573=EDGE_CURVE('',#38003,#37955,#5077,.T.) ;
#46574=EDGE_CURVE('',#37956,#38004,#5078,.T.) ;
#46575=EDGE_CURVE('',#38005,#38006,#30688,.T.) ;
#46576=EDGE_CURVE('',#38006,#38007,#5079,.T.) ;
#46577=EDGE_CURVE('',#38007,#38008,#30689,.T.) ;
#46578=EDGE_CURVE('',#38008,#38009,#5080,.T.) ;
#46579=EDGE_CURVE('',#38009,#38010,#5081,.T.) ;
#46580=EDGE_CURVE('',#38010,#38011,#5082,.T.) ;
#46581=EDGE_CURVE('',#38011,#38012,#30690,.T.) ;
#46582=EDGE_CURVE('',#38012,#38013,#5083,.T.) ;
#46583=EDGE_CURVE('',#38013,#38014,#5084,.T.) ;
#46584=EDGE_CURVE('',#38014,#38015,#5085,.T.) ;
#46585=EDGE_CURVE('',#38015,#38016,#30691,.T.) ;
#46586=EDGE_CURVE('',#38016,#38017,#5086,.T.) ;
#46587=EDGE_CURVE('',#38017,#38018,#30692,.T.) ;
#46588=EDGE_CURVE('',#38018,#38019,#5087,.T.) ;
#46589=EDGE_CURVE('',#38019,#38020,#5088,.T.) ;
#46590=EDGE_CURVE('',#38020,#36353,#5089,.T.) ;
#46591=EDGE_CURVE('',#36353,#38021,#5090,.T.) ;
#46592=EDGE_CURVE('',#38021,#38005,#5091,.T.) ;
#46593=EDGE_CURVE('',#38022,#38023,#5092,.T.) ;
#46594=EDGE_CURVE('',#38022,#38024,#30693,.T.) ;
#46595=EDGE_CURVE('',#38024,#38025,#5093,.T.) ;
#46596=EDGE_CURVE('',#38025,#38026,#30694,.T.) ;
#46597=EDGE_CURVE('',#38026,#38027,#5094,.T.) ;
#46598=EDGE_CURVE('',#38027,#38028,#30695,.T.) ;
#46599=EDGE_CURVE('',#38028,#38029,#5095,.T.) ;
#46600=EDGE_CURVE('',#38029,#38023,#30696,.T.) ;
#46601=EDGE_CURVE('',#38030,#38031,#5096,.T.) ;
#46602=EDGE_CURVE('',#38030,#38032,#30697,.T.) ;
#46603=EDGE_CURVE('',#38032,#38033,#5097,.T.) ;
#46604=EDGE_CURVE('',#38033,#38034,#30698,.T.) ;
#46605=EDGE_CURVE('',#38034,#38035,#5098,.T.) ;
#46606=EDGE_CURVE('',#38035,#38036,#30699,.T.) ;
#46607=EDGE_CURVE('',#38036,#38037,#5099,.T.) ;
#46608=EDGE_CURVE('',#38037,#38031,#30700,.T.) ;
#46609=EDGE_CURVE('',#38038,#38039,#5100,.T.) ;
#46610=EDGE_CURVE('',#38038,#38040,#30701,.T.) ;
#46611=EDGE_CURVE('',#38040,#38041,#5101,.T.) ;
#46612=EDGE_CURVE('',#38041,#38042,#30702,.T.) ;
#46613=EDGE_CURVE('',#38042,#38043,#5102,.T.) ;
#46614=EDGE_CURVE('',#38043,#38044,#30703,.T.) ;
#46615=EDGE_CURVE('',#38044,#38045,#5103,.T.) ;
#46616=EDGE_CURVE('',#38045,#38039,#30704,.T.) ;
#46617=EDGE_CURVE('',#38046,#38047,#5104,.T.) ;
#46618=EDGE_CURVE('',#38046,#38048,#30705,.T.) ;
#46619=EDGE_CURVE('',#38048,#38049,#5105,.T.) ;
#46620=EDGE_CURVE('',#38049,#38050,#30706,.T.) ;
#46621=EDGE_CURVE('',#38050,#38051,#5106,.T.) ;
#46622=EDGE_CURVE('',#38051,#38052,#30707,.T.) ;
#46623=EDGE_CURVE('',#38052,#38053,#5107,.T.) ;
#46624=EDGE_CURVE('',#38053,#38047,#30708,.T.) ;
#46625=EDGE_CURVE('',#38054,#38055,#5108,.T.) ;
#46626=EDGE_CURVE('',#38054,#38056,#30709,.T.) ;
#46627=EDGE_CURVE('',#38056,#38057,#5109,.T.) ;
#46628=EDGE_CURVE('',#38057,#38058,#30710,.T.) ;
#46629=EDGE_CURVE('',#38058,#38059,#5110,.T.) ;
#46630=EDGE_CURVE('',#38059,#38060,#30711,.T.) ;
#46631=EDGE_CURVE('',#38060,#38061,#5111,.T.) ;
#46632=EDGE_CURVE('',#38061,#38055,#30712,.T.) ;
#46633=EDGE_CURVE('',#38062,#38063,#5112,.T.) ;
#46634=EDGE_CURVE('',#38062,#38064,#30713,.T.) ;
#46635=EDGE_CURVE('',#38064,#38065,#5113,.T.) ;
#46636=EDGE_CURVE('',#38065,#38066,#30714,.T.) ;
#46637=EDGE_CURVE('',#38066,#38067,#5114,.T.) ;
#46638=EDGE_CURVE('',#38067,#38068,#30715,.T.) ;
#46639=EDGE_CURVE('',#38068,#38069,#5115,.T.) ;
#46640=EDGE_CURVE('',#38069,#38063,#30716,.T.) ;
#46641=EDGE_CURVE('',#38070,#38071,#5116,.T.) ;
#46642=EDGE_CURVE('',#38070,#38072,#30717,.T.) ;
#46643=EDGE_CURVE('',#38072,#38073,#5117,.T.) ;
#46644=EDGE_CURVE('',#38073,#38074,#30718,.T.) ;
#46645=EDGE_CURVE('',#38074,#38075,#5118,.T.) ;
#46646=EDGE_CURVE('',#38075,#38076,#30719,.T.) ;
#46647=EDGE_CURVE('',#38076,#38077,#5119,.T.) ;
#46648=EDGE_CURVE('',#38077,#38071,#30720,.T.) ;
#46649=EDGE_CURVE('',#38078,#38079,#5120,.T.) ;
#46650=EDGE_CURVE('',#38078,#38080,#30721,.T.) ;
#46651=EDGE_CURVE('',#38080,#38081,#5121,.T.) ;
#46652=EDGE_CURVE('',#38081,#38082,#30722,.T.) ;
#46653=EDGE_CURVE('',#38082,#38083,#5122,.T.) ;
#46654=EDGE_CURVE('',#38083,#38084,#30723,.T.) ;
#46655=EDGE_CURVE('',#38084,#38085,#5123,.T.) ;
#46656=EDGE_CURVE('',#38085,#38079,#30724,.T.) ;
#46657=EDGE_CURVE('',#38086,#38087,#5124,.T.) ;
#46658=EDGE_CURVE('',#38086,#38088,#30725,.T.) ;
#46659=EDGE_CURVE('',#38088,#38089,#5125,.T.) ;
#46660=EDGE_CURVE('',#38089,#38090,#30726,.T.) ;
#46661=EDGE_CURVE('',#38090,#38091,#5126,.T.) ;
#46662=EDGE_CURVE('',#38091,#38092,#30727,.T.) ;
#46663=EDGE_CURVE('',#38092,#38093,#5127,.T.) ;
#46664=EDGE_CURVE('',#38093,#38087,#30728,.T.) ;
#46665=EDGE_CURVE('',#37269,#37256,#30729,.T.) ;
#46666=EDGE_CURVE('',#37247,#37268,#30730,.T.) ;
#46667=EDGE_CURVE('',#37270,#37263,#30731,.T.) ;
#46668=EDGE_CURVE('',#37264,#37269,#30732,.T.) ;
#46669=EDGE_CURVE('',#37270,#38094,#30733,.T.) ;
#46670=EDGE_CURVE('',#38094,#37263,#30734,.T.) ;
#46671=EDGE_CURVE('',#37247,#37273,#30735,.T.) ;
#46672=EDGE_CURVE('',#37273,#37268,#30736,.T.) ;
#46673=EDGE_CURVE('',#37264,#37255,#30737,.T.) ;
#46674=EDGE_CURVE('',#36354,#37266,#30738,.T.) ;
#46675=EDGE_CURVE('',#36355,#38095,#2170,.T.) ;
#46676=EDGE_CURVE('',#38094,#38095,#5128,.T.) ;
#46677=EDGE_CURVE('',#38096,#38094,#2171,.T.) ;
#46678=EDGE_CURVE('',#38096,#38097,#2172,.T.) ;
#46679=EDGE_CURVE('',#36481,#38097,#5129,.T.) ;
#46680=EDGE_CURVE('',#37267,#36480,#30739,.T.) ;
#46681=EDGE_CURVE('',#37274,#37267,#30740,.T.) ;
#46682=EDGE_CURVE('',#37248,#37272,#30741,.T.) ;
#46683=EDGE_CURVE('',#37265,#37254,#30742,.T.) ;
#46684=EDGE_CURVE('',#37266,#36356,#30743,.T.) ;
#46685=EDGE_CURVE('',#37261,#37265,#30744,.T.) ;
#46686=EDGE_CURVE('',#37274,#36489,#30745,.T.) ;
#46687=EDGE_CURVE('',#37248,#36576,#30746,.T.) ;
#46688=EDGE_CURVE('',#36575,#37272,#30747,.T.) ;
#46689=EDGE_CURVE('',#37261,#37253,#30748,.T.) ;
#46690=EDGE_CURVE('',#37271,#36488,#30749,.T.) ;
#46691=EDGE_CURVE('',#36577,#37271,#30750,.T.) ;
#46692=EDGE_CURVE('',#38098,#36576,#5130,.T.) ;
#46693=EDGE_CURVE('',#37249,#38098,#30751,.T.) ;
#46694=EDGE_CURVE('',#37262,#37252,#30752,.T.) ;
#46695=EDGE_CURVE('',#36357,#37257,#30753,.T.) ;
#46696=EDGE_CURVE('',#37258,#37262,#30754,.T.) ;
#46697=EDGE_CURVE('',#36484,#37257,#30755,.T.) ;
#46698=EDGE_CURVE('',#36577,#36488,#30756,.T.) ;
#46699=EDGE_CURVE('',#36582,#36579,#30757,.T.) ;
#46700=EDGE_CURVE('',#36579,#36580,#30758,.T.) ;
#46701=EDGE_CURVE('',#38098,#36721,#30759,.T.) ;
#46702=EDGE_CURVE('',#38099,#38098,#30760,.T.) ;
#46703=EDGE_CURVE('',#37249,#38099,#30761,.T.) ;
#46704=EDGE_CURVE('',#37258,#37252,#30762,.T.) ;
#46705=EDGE_CURVE('',#36485,#37260,#30763,.T.) ;
#46706=EDGE_CURVE('',#36578,#36487,#30764,.T.) ;
#46707=EDGE_CURVE('',#36652,#36578,#30765,.T.) ;
#46708=EDGE_CURVE('',#38099,#36720,#30766,.T.) ;
#46709=EDGE_CURVE('',#38100,#38099,#5131,.T.) ;
#46710=EDGE_CURVE('',#37250,#38100,#30767,.T.) ;
#46711=EDGE_CURVE('',#37259,#37251,#30768,.T.) ;
#46712=EDGE_CURVE('',#37260,#36574,#30769,.T.) ;
#46713=EDGE_CURVE('',#36571,#37259,#30770,.T.) ;
#46714=EDGE_CURVE('',#36485,#36574,#30771,.T.) ;
#46715=EDGE_CURVE('',#36653,#36487,#30772,.T.) ;
#46716=EDGE_CURVE('',#38100,#36719,#30773,.T.) ;
#46717=EDGE_CURVE('',#38101,#38100,#30774,.T.) ;
#46718=EDGE_CURVE('',#37250,#38101,#30775,.T.) ;
#46719=EDGE_CURVE('',#36570,#37251,#30776,.T.) ;
#46720=EDGE_CURVE('',#36486,#36573,#30777,.T.) ;
#46721=EDGE_CURVE('',#36654,#36486,#30778,.T.) ;
#46722=EDGE_CURVE('',#38101,#36718,#30779,.T.) ;
#46723=EDGE_CURVE('',#36570,#38101,#5132,.T.) ;
#46724=EDGE_CURVE('',#36655,#36573,#30780,.T.) ;
#46725=EDGE_CURVE('',#36572,#36585,#30781,.T.) ;
#46726=EDGE_CURVE('',#36587,#36572,#30782,.T.) ;
#46727=EDGE_CURVE('',#37981,#38014,#30783,.T.) ;
#46728=EDGE_CURVE('',#38015,#37979,#30784,.T.) ;
#46729=EDGE_CURVE('',#38016,#37977,#30785,.T.) ;
#46730=EDGE_CURVE('',#37983,#38014,#30786,.T.) ;
#46731=EDGE_CURVE('',#38017,#37975,#30787,.T.) ;
#46732=EDGE_CURVE('',#37985,#38013,#30788,.T.) ;
#46733=EDGE_CURVE('',#38018,#37973,#30789,.T.) ;
#46734=EDGE_CURVE('',#37987,#38013,#30790,.T.) ;
#46735=EDGE_CURVE('',#38019,#37971,#30791,.T.) ;
#46736=EDGE_CURVE('',#37989,#38012,#30792,.T.) ;
#46737=EDGE_CURVE('',#38019,#37969,#30793,.T.) ;
#46738=EDGE_CURVE('',#37991,#38012,#30794,.T.) ;
#46739=EDGE_CURVE('',#38020,#36362,#30795,.T.) ;
#46740=EDGE_CURVE('',#37993,#38011,#30796,.T.) ;
#46741=EDGE_CURVE('',#38020,#36361,#30797,.T.) ;
#46742=EDGE_CURVE('',#37995,#38011,#30798,.T.) ;
#46743=EDGE_CURVE('',#37997,#38010,#30799,.T.) ;
#46744=EDGE_CURVE('',#37999,#38010,#30800,.T.) ;
#46745=EDGE_CURVE('',#38021,#37965,#30801,.T.) ;
#46746=EDGE_CURVE('',#38001,#38009,#30802,.T.) ;
#46747=EDGE_CURVE('',#38021,#37963,#30803,.T.) ;
#46748=EDGE_CURVE('',#38003,#38009,#30804,.T.) ;
#46749=EDGE_CURVE('',#38005,#37961,#30805,.T.) ;
#46750=EDGE_CURVE('',#37955,#38008,#30806,.T.) ;
#46751=EDGE_CURVE('',#38006,#37959,#30807,.T.) ;
#46752=EDGE_CURVE('',#37957,#38007,#30808,.T.) ;
#46753=EDGE_CURVE('',#37440,#36762,#30809,.T.) ;
#46754=EDGE_CURVE('',#36763,#37442,#30810,.T.) ;
#46755=EDGE_CURVE('',#37438,#36762,#30811,.T.) ;
#46756=EDGE_CURVE('',#36763,#37444,#30812,.T.) ;
#46757=EDGE_CURVE('',#37436,#36761,#30813,.T.) ;
#46758=EDGE_CURVE('',#36764,#37446,#30814,.T.) ;
#46759=EDGE_CURVE('',#37434,#36760,#30815,.T.) ;
#46760=EDGE_CURVE('',#36765,#37448,#30816,.T.) ;
#46761=EDGE_CURVE('',#36766,#37450,#30817,.T.) ;
#46762=EDGE_CURVE('',#36767,#37452,#30818,.T.) ;
#46763=EDGE_CURVE('',#37432,#36759,#30819,.T.) ;
#46764=EDGE_CURVE('',#36768,#37454,#30820,.T.) ;
#46765=EDGE_CURVE('',#37431,#36758,#30821,.T.) ;
#46766=EDGE_CURVE('',#36769,#37456,#30822,.T.) ;
#46767=EDGE_CURVE('',#37430,#36757,#30823,.T.) ;
#46768=EDGE_CURVE('',#36770,#37458,#30824,.T.) ;
#46769=EDGE_CURVE('',#37428,#36756,#30825,.T.) ;
#46770=EDGE_CURVE('',#36771,#37460,#30826,.T.) ;
#46771=EDGE_CURVE('',#37426,#36755,#30827,.T.) ;
#46772=EDGE_CURVE('',#36772,#37462,#30828,.T.) ;
#46773=EDGE_CURVE('',#37424,#36755,#30829,.T.) ;
#46774=EDGE_CURVE('',#36773,#37464,#30830,.T.) ;
#46775=EDGE_CURVE('',#37422,#36754,#30831,.T.) ;
#46776=EDGE_CURVE('',#36752,#37466,#30832,.T.) ;
#46777=EDGE_CURVE('',#37420,#36754,#30833,.T.) ;
#46778=EDGE_CURVE('',#36753,#37468,#30834,.T.) ;
#46779=EDGE_CURVE('',#37507,#36784,#30835,.T.) ;
#46780=EDGE_CURVE('',#36785,#37509,#30836,.T.) ;
#46781=EDGE_CURVE('',#37505,#36784,#30837,.T.) ;
#46782=EDGE_CURVE('',#36785,#37511,#30838,.T.) ;
#46783=EDGE_CURVE('',#37503,#36783,#30839,.T.) ;
#46784=EDGE_CURVE('',#36786,#37513,#30840,.T.) ;
#46785=EDGE_CURVE('',#37501,#36782,#30841,.T.) ;
#46786=EDGE_CURVE('',#36787,#37515,#30842,.T.) ;
#46787=EDGE_CURVE('',#36788,#37517,#30843,.T.) ;
#46788=EDGE_CURVE('',#36789,#37519,#30844,.T.) ;
#46789=EDGE_CURVE('',#37499,#36781,#30845,.T.) ;
#46790=EDGE_CURVE('',#36790,#37521,#30846,.T.) ;
#46791=EDGE_CURVE('',#37498,#36780,#30847,.T.) ;
#46792=EDGE_CURVE('',#36791,#37523,#30848,.T.) ;
#46793=EDGE_CURVE('',#37497,#36779,#30849,.T.) ;
#46794=EDGE_CURVE('',#36792,#37525,#30850,.T.) ;
#46795=EDGE_CURVE('',#37495,#36778,#30851,.T.) ;
#46796=EDGE_CURVE('',#36793,#37527,#30852,.T.) ;
#46797=EDGE_CURVE('',#37493,#36777,#30853,.T.) ;
#46798=EDGE_CURVE('',#36794,#37529,#30854,.T.) ;
#46799=EDGE_CURVE('',#37491,#36777,#30855,.T.) ;
#46800=EDGE_CURVE('',#36795,#37531,#30856,.T.) ;
#46801=EDGE_CURVE('',#37489,#36776,#30857,.T.) ;
#46802=EDGE_CURVE('',#36774,#37533,#30858,.T.) ;
#46803=EDGE_CURVE('',#37487,#36776,#30859,.T.) ;
#46804=EDGE_CURVE('',#36775,#37535,#30860,.T.) ;
#46805=EDGE_CURVE('',#37574,#36806,#30861,.T.) ;
#46806=EDGE_CURVE('',#36807,#37576,#30862,.T.) ;
#46807=EDGE_CURVE('',#37572,#36806,#30863,.T.) ;
#46808=EDGE_CURVE('',#36807,#37578,#30864,.T.) ;
#46809=EDGE_CURVE('',#37570,#36805,#30865,.T.) ;
#46810=EDGE_CURVE('',#36808,#37580,#30866,.T.) ;
#46811=EDGE_CURVE('',#37568,#36804,#30867,.T.) ;
#46812=EDGE_CURVE('',#36809,#37582,#30868,.T.) ;
#46813=EDGE_CURVE('',#36810,#37584,#30869,.T.) ;
#46814=EDGE_CURVE('',#36811,#37586,#30870,.T.) ;
#46815=EDGE_CURVE('',#37566,#36803,#30871,.T.) ;
#46816=EDGE_CURVE('',#36812,#37588,#30872,.T.) ;
#46817=EDGE_CURVE('',#37565,#36802,#30873,.T.) ;
#46818=EDGE_CURVE('',#36813,#37590,#30874,.T.) ;
#46819=EDGE_CURVE('',#37564,#36801,#30875,.T.) ;
#46820=EDGE_CURVE('',#36814,#37592,#30876,.T.) ;
#46821=EDGE_CURVE('',#37562,#36800,#30877,.T.) ;
#46822=EDGE_CURVE('',#36815,#37594,#30878,.T.) ;
#46823=EDGE_CURVE('',#37560,#36799,#30879,.T.) ;
#46824=EDGE_CURVE('',#36816,#37596,#30880,.T.) ;
#46825=EDGE_CURVE('',#37558,#36799,#30881,.T.) ;
#46826=EDGE_CURVE('',#36817,#37598,#30882,.T.) ;
#46827=EDGE_CURVE('',#37556,#36798,#30883,.T.) ;
#46828=EDGE_CURVE('',#36796,#37600,#30884,.T.) ;
#46829=EDGE_CURVE('',#37554,#36798,#30885,.T.) ;
#46830=EDGE_CURVE('',#36797,#37602,#30886,.T.) ;
#46831=EDGE_CURVE('',#37641,#36828,#30887,.T.) ;
#46832=EDGE_CURVE('',#36829,#37643,#30888,.T.) ;
#46833=EDGE_CURVE('',#37639,#36828,#30889,.T.) ;
#46834=EDGE_CURVE('',#36829,#37645,#30890,.T.) ;
#46835=EDGE_CURVE('',#37637,#36827,#30891,.T.) ;
#46836=EDGE_CURVE('',#36830,#37647,#30892,.T.) ;
#46837=EDGE_CURVE('',#37635,#36826,#30893,.T.) ;
#46838=EDGE_CURVE('',#36831,#37649,#30894,.T.) ;
#46839=EDGE_CURVE('',#36832,#37651,#30895,.T.) ;
#46840=EDGE_CURVE('',#36833,#37653,#30896,.T.) ;
#46841=EDGE_CURVE('',#37633,#36825,#30897,.T.) ;
#46842=EDGE_CURVE('',#36834,#37655,#30898,.T.) ;
#46843=EDGE_CURVE('',#37632,#36824,#30899,.T.) ;
#46844=EDGE_CURVE('',#36835,#37657,#30900,.T.) ;
#46845=EDGE_CURVE('',#37631,#36823,#30901,.T.) ;
#46846=EDGE_CURVE('',#36836,#37659,#30902,.T.) ;
#46847=EDGE_CURVE('',#37629,#36822,#30903,.T.) ;
#46848=EDGE_CURVE('',#36837,#37661,#30904,.T.) ;
#46849=EDGE_CURVE('',#37627,#36821,#30905,.T.) ;
#46850=EDGE_CURVE('',#36838,#37663,#30906,.T.) ;
#46851=EDGE_CURVE('',#37625,#36821,#30907,.T.) ;
#46852=EDGE_CURVE('',#36839,#37665,#30908,.T.) ;
#46853=EDGE_CURVE('',#37623,#36820,#30909,.T.) ;
#46854=EDGE_CURVE('',#36818,#37667,#30910,.T.) ;
#46855=EDGE_CURVE('',#37621,#36820,#30911,.T.) ;
#46856=EDGE_CURVE('',#36819,#37669,#30912,.T.) ;
#46857=EDGE_CURVE('',#37708,#36850,#30913,.T.) ;
#46858=EDGE_CURVE('',#36851,#37710,#30914,.T.) ;
#46859=EDGE_CURVE('',#37706,#36850,#30915,.T.) ;
#46860=EDGE_CURVE('',#36851,#37712,#30916,.T.) ;
#46861=EDGE_CURVE('',#37704,#36849,#30917,.T.) ;
#46862=EDGE_CURVE('',#36852,#37714,#30918,.T.) ;
#46863=EDGE_CURVE('',#37702,#36848,#30919,.T.) ;
#46864=EDGE_CURVE('',#36853,#37716,#30920,.T.) ;
#46865=EDGE_CURVE('',#36854,#37718,#30921,.T.) ;
#46866=EDGE_CURVE('',#36855,#37720,#30922,.T.) ;
#46867=EDGE_CURVE('',#37700,#36847,#30923,.T.) ;
#46868=EDGE_CURVE('',#36856,#37722,#30924,.T.) ;
#46869=EDGE_CURVE('',#37699,#36846,#30925,.T.) ;
#46870=EDGE_CURVE('',#36857,#37724,#30926,.T.) ;
#46871=EDGE_CURVE('',#37698,#36845,#30927,.T.) ;
#46872=EDGE_CURVE('',#36858,#37726,#30928,.T.) ;
#46873=EDGE_CURVE('',#37696,#36844,#30929,.T.) ;
#46874=EDGE_CURVE('',#36859,#37728,#30930,.T.) ;
#46875=EDGE_CURVE('',#37694,#36843,#30931,.T.) ;
#46876=EDGE_CURVE('',#36860,#37730,#30932,.T.) ;
#46877=EDGE_CURVE('',#37692,#36843,#30933,.T.) ;
#46878=EDGE_CURVE('',#36861,#37732,#30934,.T.) ;
#46879=EDGE_CURVE('',#37690,#36842,#30935,.T.) ;
#46880=EDGE_CURVE('',#36840,#37734,#30936,.T.) ;
#46881=EDGE_CURVE('',#37688,#36842,#30937,.T.) ;
#46882=EDGE_CURVE('',#36841,#37736,#30938,.T.) ;
#46883=EDGE_CURVE('',#37775,#36872,#30939,.T.) ;
#46884=EDGE_CURVE('',#36873,#37777,#30940,.T.) ;
#46885=EDGE_CURVE('',#37773,#36872,#30941,.T.) ;
#46886=EDGE_CURVE('',#36873,#37779,#30942,.T.) ;
#46887=EDGE_CURVE('',#37771,#36871,#30943,.T.) ;
#46888=EDGE_CURVE('',#36874,#37781,#30944,.T.) ;
#46889=EDGE_CURVE('',#37769,#36870,#30945,.T.) ;
#46890=EDGE_CURVE('',#36875,#37783,#30946,.T.) ;
#46891=EDGE_CURVE('',#36876,#37785,#30947,.T.) ;
#46892=EDGE_CURVE('',#36877,#37787,#30948,.T.) ;
#46893=EDGE_CURVE('',#37767,#36869,#30949,.T.) ;
#46894=EDGE_CURVE('',#36878,#37789,#30950,.T.) ;
#46895=EDGE_CURVE('',#37766,#36868,#30951,.T.) ;
#46896=EDGE_CURVE('',#36879,#37791,#30952,.T.) ;
#46897=EDGE_CURVE('',#37765,#36867,#30953,.T.) ;
#46898=EDGE_CURVE('',#36880,#37793,#30954,.T.) ;
#46899=EDGE_CURVE('',#37763,#36866,#30955,.T.) ;
#46900=EDGE_CURVE('',#36881,#37795,#30956,.T.) ;
#46901=EDGE_CURVE('',#37761,#36865,#30957,.T.) ;
#46902=EDGE_CURVE('',#36882,#37797,#30958,.T.) ;
#46903=EDGE_CURVE('',#37759,#36865,#30959,.T.) ;
#46904=EDGE_CURVE('',#36883,#37799,#30960,.T.) ;
#46905=EDGE_CURVE('',#37757,#36864,#30961,.T.) ;
#46906=EDGE_CURVE('',#36862,#37801,#30962,.T.) ;
#46907=EDGE_CURVE('',#37755,#36864,#30963,.T.) ;
#46908=EDGE_CURVE('',#36863,#37803,#30964,.T.) ;
#46909=EDGE_CURVE('',#37842,#36894,#30965,.T.) ;
#46910=EDGE_CURVE('',#36895,#37844,#30966,.T.) ;
#46911=EDGE_CURVE('',#37840,#36894,#30967,.T.) ;
#46912=EDGE_CURVE('',#36895,#37846,#30968,.T.) ;
#46913=EDGE_CURVE('',#37838,#36893,#30969,.T.) ;
#46914=EDGE_CURVE('',#36896,#37848,#30970,.T.) ;
#46915=EDGE_CURVE('',#37836,#36892,#30971,.T.) ;
#46916=EDGE_CURVE('',#36897,#37850,#30972,.T.) ;
#46917=EDGE_CURVE('',#36898,#37852,#30973,.T.) ;
#46918=EDGE_CURVE('',#36899,#37854,#30974,.T.) ;
#46919=EDGE_CURVE('',#37834,#36891,#30975,.T.) ;
#46920=EDGE_CURVE('',#36900,#37856,#30976,.T.) ;
#46921=EDGE_CURVE('',#37833,#36890,#30977,.T.) ;
#46922=EDGE_CURVE('',#36901,#37858,#30978,.T.) ;
#46923=EDGE_CURVE('',#37832,#36889,#30979,.T.) ;
#46924=EDGE_CURVE('',#36902,#37860,#30980,.T.) ;
#46925=EDGE_CURVE('',#37830,#36888,#30981,.T.) ;
#46926=EDGE_CURVE('',#36903,#37862,#30982,.T.) ;
#46927=EDGE_CURVE('',#37828,#36887,#30983,.T.) ;
#46928=EDGE_CURVE('',#36904,#37864,#30984,.T.) ;
#46929=EDGE_CURVE('',#37826,#36887,#30985,.T.) ;
#46930=EDGE_CURVE('',#36905,#37866,#30986,.T.) ;
#46931=EDGE_CURVE('',#37824,#36886,#30987,.T.) ;
#46932=EDGE_CURVE('',#36884,#37868,#30988,.T.) ;
#46933=EDGE_CURVE('',#37822,#36886,#30989,.T.) ;
#46934=EDGE_CURVE('',#36885,#37870,#30990,.T.) ;
#46935=EDGE_CURVE('',#37909,#36916,#30991,.T.) ;
#46936=EDGE_CURVE('',#36917,#37911,#30992,.T.) ;
#46937=EDGE_CURVE('',#37907,#36916,#30993,.T.) ;
#46938=EDGE_CURVE('',#36917,#37913,#30994,.T.) ;
#46939=EDGE_CURVE('',#37905,#36915,#30995,.T.) ;
#46940=EDGE_CURVE('',#36918,#37915,#30996,.T.) ;
#46941=EDGE_CURVE('',#37903,#36914,#30997,.T.) ;
#46942=EDGE_CURVE('',#36919,#37917,#30998,.T.) ;
#46943=EDGE_CURVE('',#36920,#37919,#30999,.T.) ;
#46944=EDGE_CURVE('',#36921,#37921,#31000,.T.) ;
#46945=EDGE_CURVE('',#37901,#36913,#31001,.T.) ;
#46946=EDGE_CURVE('',#36922,#37923,#31002,.T.) ;
#46947=EDGE_CURVE('',#37900,#36912,#31003,.T.) ;
#46948=EDGE_CURVE('',#36923,#37925,#31004,.T.) ;
#46949=EDGE_CURVE('',#37899,#36911,#31005,.T.) ;
#46950=EDGE_CURVE('',#36924,#37927,#31006,.T.) ;
#46951=EDGE_CURVE('',#37897,#36910,#31007,.T.) ;
#46952=EDGE_CURVE('',#36925,#37929,#31008,.T.) ;
#46953=EDGE_CURVE('',#37895,#36909,#31009,.T.) ;
#46954=EDGE_CURVE('',#36926,#37931,#31010,.T.) ;
#46955=EDGE_CURVE('',#37893,#36909,#31011,.T.) ;
#46956=EDGE_CURVE('',#36927,#37933,#31012,.T.) ;
#46957=EDGE_CURVE('',#37891,#36908,#31013,.T.) ;
#46958=EDGE_CURVE('',#36906,#37935,#31014,.T.) ;
#46959=EDGE_CURVE('',#37889,#36908,#31015,.T.) ;
#46960=EDGE_CURVE('',#36907,#37937,#31016,.T.) ;
#46961=EDGE_CURVE('',#37976,#36938,#31017,.T.) ;
#46962=EDGE_CURVE('',#36939,#37978,#31018,.T.) ;
#46963=EDGE_CURVE('',#37974,#36938,#31019,.T.) ;
#46964=EDGE_CURVE('',#36939,#37980,#31020,.T.) ;
#46965=EDGE_CURVE('',#37972,#36937,#31021,.T.) ;
#46966=EDGE_CURVE('',#36940,#37982,#31022,.T.) ;
#46967=EDGE_CURVE('',#37970,#36936,#31023,.T.) ;
#46968=EDGE_CURVE('',#36941,#37984,#31024,.T.) ;
#46969=EDGE_CURVE('',#36942,#37986,#31025,.T.) ;
#46970=EDGE_CURVE('',#36943,#37988,#31026,.T.) ;
#46971=EDGE_CURVE('',#37968,#36935,#31027,.T.) ;
#46972=EDGE_CURVE('',#36944,#37990,#31028,.T.) ;
#46973=EDGE_CURVE('',#37967,#36934,#31029,.T.) ;
#46974=EDGE_CURVE('',#36945,#37992,#31030,.T.) ;
#46975=EDGE_CURVE('',#37966,#36933,#31031,.T.) ;
#46976=EDGE_CURVE('',#36946,#37994,#31032,.T.) ;
#46977=EDGE_CURVE('',#37964,#36932,#31033,.T.) ;
#46978=EDGE_CURVE('',#36947,#37996,#31034,.T.) ;
#46979=EDGE_CURVE('',#37962,#36931,#31035,.T.) ;
#46980=EDGE_CURVE('',#36948,#37998,#31036,.T.) ;
#46981=EDGE_CURVE('',#37960,#36931,#31037,.T.) ;
#46982=EDGE_CURVE('',#36949,#38000,#31038,.T.) ;
#46983=EDGE_CURVE('',#37958,#36930,#31039,.T.) ;
#46984=EDGE_CURVE('',#36928,#38002,#31040,.T.) ;
#46985=EDGE_CURVE('',#37956,#36930,#31041,.T.) ;
#46986=EDGE_CURVE('',#36929,#38004,#31042,.T.) ;
#46987=EDGE_CURVE('',#37287,#37246,#31043,.T.) ;
#46988=EDGE_CURVE('',#37237,#37286,#31044,.T.) ;
#46989=EDGE_CURVE('',#37288,#37281,#31045,.T.) ;
#46990=EDGE_CURVE('',#37282,#37287,#31046,.T.) ;
#46991=EDGE_CURVE('',#37288,#38102,#31047,.T.) ;
#46992=EDGE_CURVE('',#38102,#37281,#31048,.T.) ;
#46993=EDGE_CURVE('',#37237,#37291,#31049,.T.) ;
#46994=EDGE_CURVE('',#37291,#37286,#31050,.T.) ;
#46995=EDGE_CURVE('',#37282,#37245,#31051,.T.) ;
#46996=EDGE_CURVE('',#36303,#37284,#31052,.T.) ;
#46997=EDGE_CURVE('',#36304,#38103,#2173,.T.) ;
#46998=EDGE_CURVE('',#38102,#38103,#5133,.T.) ;
#46999=EDGE_CURVE('',#38104,#38102,#2174,.T.) ;
#47000=EDGE_CURVE('',#38104,#38105,#2175,.T.) ;
#47001=EDGE_CURVE('',#36471,#38105,#5134,.T.) ;
#47002=EDGE_CURVE('',#37285,#36470,#31053,.T.) ;
#47003=EDGE_CURVE('',#37292,#37285,#31054,.T.) ;
#47004=EDGE_CURVE('',#37238,#37290,#31055,.T.) ;
#47005=EDGE_CURVE('',#37283,#37244,#31056,.T.) ;
#47006=EDGE_CURVE('',#37284,#36305,#31057,.T.) ;
#47007=EDGE_CURVE('',#37279,#37283,#31058,.T.) ;
#47008=EDGE_CURVE('',#37292,#36479,#31059,.T.) ;
#47009=EDGE_CURVE('',#37238,#36566,#31060,.T.) ;
#47010=EDGE_CURVE('',#36565,#37290,#31061,.T.) ;
#47011=EDGE_CURVE('',#37279,#37243,#31062,.T.) ;
#47012=EDGE_CURVE('',#37289,#36478,#31063,.T.) ;
#47013=EDGE_CURVE('',#36567,#37289,#31064,.T.) ;
#47014=EDGE_CURVE('',#38106,#36566,#5135,.T.) ;
#47015=EDGE_CURVE('',#37239,#38106,#31065,.T.) ;
#47016=EDGE_CURVE('',#37280,#37242,#31066,.T.) ;
#47017=EDGE_CURVE('',#36306,#37275,#31067,.T.) ;
#47018=EDGE_CURVE('',#37276,#37280,#31068,.T.) ;
#47019=EDGE_CURVE('',#36474,#37275,#31069,.T.) ;
#47020=EDGE_CURVE('',#36567,#36478,#31070,.T.) ;
#47021=EDGE_CURVE('',#36586,#36569,#31071,.T.) ;
#47022=EDGE_CURVE('',#36569,#36584,#31072,.T.) ;
#47023=EDGE_CURVE('',#38106,#36717,#31073,.T.) ;
#47024=EDGE_CURVE('',#38107,#38106,#31074,.T.) ;
#47025=EDGE_CURVE('',#37239,#38107,#31075,.T.) ;
#47026=EDGE_CURVE('',#37276,#37242,#31076,.T.) ;
#47027=EDGE_CURVE('',#36475,#37278,#31077,.T.) ;
#47028=EDGE_CURVE('',#36568,#36477,#31078,.T.) ;
#47029=EDGE_CURVE('',#36656,#36568,#31079,.T.) ;
#47030=EDGE_CURVE('',#38107,#36716,#31080,.T.) ;
#47031=EDGE_CURVE('',#38108,#38107,#5136,.T.) ;
#47032=EDGE_CURVE('',#37240,#38108,#31081,.T.) ;
#47033=EDGE_CURVE('',#37277,#37241,#31082,.T.) ;
#47034=EDGE_CURVE('',#37278,#36564,#31083,.T.) ;
#47035=EDGE_CURVE('',#36561,#37277,#31084,.T.) ;
#47036=EDGE_CURVE('',#36475,#36564,#31085,.T.) ;
#47037=EDGE_CURVE('',#36657,#36477,#31086,.T.) ;
#47038=EDGE_CURVE('',#38108,#36715,#31087,.T.) ;
#47039=EDGE_CURVE('',#38109,#38108,#31088,.T.) ;
#47040=EDGE_CURVE('',#37240,#38109,#31089,.T.) ;
#47041=EDGE_CURVE('',#36560,#37241,#31090,.T.) ;
#47042=EDGE_CURVE('',#36476,#36563,#31091,.T.) ;
#47043=EDGE_CURVE('',#36658,#36476,#31092,.T.) ;
#47044=EDGE_CURVE('',#38109,#36714,#31093,.T.) ;
#47045=EDGE_CURVE('',#36560,#38109,#5137,.T.) ;
#47046=EDGE_CURVE('',#36659,#36563,#31094,.T.) ;
#47047=EDGE_CURVE('',#36562,#36589,#31095,.T.) ;
#47048=EDGE_CURVE('',#36591,#36562,#31096,.T.) ;
#47049=EDGE_CURVE('',#37914,#37947,#31097,.T.) ;
#47050=EDGE_CURVE('',#37948,#37912,#31098,.T.) ;
#47051=EDGE_CURVE('',#37949,#37910,#31099,.T.) ;
#47052=EDGE_CURVE('',#37916,#37947,#31100,.T.) ;
#47053=EDGE_CURVE('',#37950,#37908,#31101,.T.) ;
#47054=EDGE_CURVE('',#37918,#37946,#31102,.T.) ;
#47055=EDGE_CURVE('',#37951,#37906,#31103,.T.) ;
#47056=EDGE_CURVE('',#37920,#37946,#31104,.T.) ;
#47057=EDGE_CURVE('',#37952,#37904,#31105,.T.) ;
#47058=EDGE_CURVE('',#37922,#37945,#31106,.T.) ;
#47059=EDGE_CURVE('',#37952,#37902,#31107,.T.) ;
#47060=EDGE_CURVE('',#37924,#37945,#31108,.T.) ;
#47061=EDGE_CURVE('',#37953,#36364,#31109,.T.) ;
#47062=EDGE_CURVE('',#37926,#37944,#31110,.T.) ;
#47063=EDGE_CURVE('',#37953,#36363,#31111,.T.) ;
#47064=EDGE_CURVE('',#37928,#37944,#31112,.T.) ;
#47065=EDGE_CURVE('',#37930,#37943,#31113,.T.) ;
#47066=EDGE_CURVE('',#37932,#37943,#31114,.T.) ;
#47067=EDGE_CURVE('',#37954,#37898,#31115,.T.) ;
#47068=EDGE_CURVE('',#37934,#37942,#31116,.T.) ;
#47069=EDGE_CURVE('',#37954,#37896,#31117,.T.) ;
#47070=EDGE_CURVE('',#37936,#37942,#31118,.T.) ;
#47071=EDGE_CURVE('',#37938,#37894,#31119,.T.) ;
#47072=EDGE_CURVE('',#37888,#37941,#31120,.T.) ;
#47073=EDGE_CURVE('',#37939,#37892,#31121,.T.) ;
#47074=EDGE_CURVE('',#37890,#37940,#31122,.T.) ;
#47075=EDGE_CURVE('',#37305,#37236,#31123,.T.) ;
#47076=EDGE_CURVE('',#37227,#37304,#31124,.T.) ;
#47077=EDGE_CURVE('',#37306,#37299,#31125,.T.) ;
#47078=EDGE_CURVE('',#37300,#37305,#31126,.T.) ;
#47079=EDGE_CURVE('',#37306,#38110,#31127,.T.) ;
#47080=EDGE_CURVE('',#38110,#37299,#31128,.T.) ;
#47081=EDGE_CURVE('',#37227,#37309,#31129,.T.) ;
#47082=EDGE_CURVE('',#37309,#37304,#31130,.T.) ;
#47083=EDGE_CURVE('',#37300,#37235,#31131,.T.) ;
#47084=EDGE_CURVE('',#36288,#37302,#31132,.T.) ;
#47085=EDGE_CURVE('',#36289,#38111,#2176,.T.) ;
#47086=EDGE_CURVE('',#38110,#38111,#5138,.T.) ;
#47087=EDGE_CURVE('',#38112,#38110,#2177,.T.) ;
#47088=EDGE_CURVE('',#38112,#38113,#2178,.T.) ;
#47089=EDGE_CURVE('',#36461,#38113,#5139,.T.) ;
#47090=EDGE_CURVE('',#37303,#36460,#31133,.T.) ;
#47091=EDGE_CURVE('',#37310,#37303,#31134,.T.) ;
#47092=EDGE_CURVE('',#37228,#37308,#31135,.T.) ;
#47093=EDGE_CURVE('',#37301,#37234,#31136,.T.) ;
#47094=EDGE_CURVE('',#37302,#36290,#31137,.T.) ;
#47095=EDGE_CURVE('',#37297,#37301,#31138,.T.) ;
#47096=EDGE_CURVE('',#37310,#36469,#31139,.T.) ;
#47097=EDGE_CURVE('',#37228,#36556,#31140,.T.) ;
#47098=EDGE_CURVE('',#36555,#37308,#31141,.T.) ;
#47099=EDGE_CURVE('',#37297,#37233,#31142,.T.) ;
#47100=EDGE_CURVE('',#37307,#36468,#31143,.T.) ;
#47101=EDGE_CURVE('',#36557,#37307,#31144,.T.) ;
#47102=EDGE_CURVE('',#38114,#36556,#5140,.T.) ;
#47103=EDGE_CURVE('',#37229,#38114,#31145,.T.) ;
#47104=EDGE_CURVE('',#37298,#37232,#31146,.T.) ;
#47105=EDGE_CURVE('',#36291,#37293,#31147,.T.) ;
#47106=EDGE_CURVE('',#37294,#37298,#31148,.T.) ;
#47107=EDGE_CURVE('',#36464,#37293,#31149,.T.) ;
#47108=EDGE_CURVE('',#36557,#36468,#31150,.T.) ;
#47109=EDGE_CURVE('',#36590,#36559,#31151,.T.) ;
#47110=EDGE_CURVE('',#36559,#36588,#31152,.T.) ;
#47111=EDGE_CURVE('',#38114,#36713,#31153,.T.) ;
#47112=EDGE_CURVE('',#38115,#38114,#31154,.T.) ;
#47113=EDGE_CURVE('',#37229,#38115,#31155,.T.) ;
#47114=EDGE_CURVE('',#37294,#37232,#31156,.T.) ;
#47115=EDGE_CURVE('',#36465,#37296,#31157,.T.) ;
#47116=EDGE_CURVE('',#36558,#36467,#31158,.T.) ;
#47117=EDGE_CURVE('',#36660,#36558,#31159,.T.) ;
#47118=EDGE_CURVE('',#38115,#36712,#31160,.T.) ;
#47119=EDGE_CURVE('',#38116,#38115,#5141,.T.) ;
#47120=EDGE_CURVE('',#37230,#38116,#31161,.T.) ;
#47121=EDGE_CURVE('',#37295,#37231,#31162,.T.) ;
#47122=EDGE_CURVE('',#37296,#36554,#31163,.T.) ;
#47123=EDGE_CURVE('',#36551,#37295,#31164,.T.) ;
#47124=EDGE_CURVE('',#36465,#36554,#31165,.T.) ;
#47125=EDGE_CURVE('',#36661,#36467,#31166,.T.) ;
#47126=EDGE_CURVE('',#38116,#36711,#31167,.T.) ;
#47127=EDGE_CURVE('',#38117,#38116,#31168,.T.) ;
#47128=EDGE_CURVE('',#37230,#38117,#31169,.T.) ;
#47129=EDGE_CURVE('',#36550,#37231,#31170,.T.) ;
#47130=EDGE_CURVE('',#36466,#36553,#31171,.T.) ;
#47131=EDGE_CURVE('',#36662,#36466,#31172,.T.) ;
#47132=EDGE_CURVE('',#38117,#36710,#31173,.T.) ;
#47133=EDGE_CURVE('',#36550,#38117,#5142,.T.) ;
#47134=EDGE_CURVE('',#36663,#36553,#31174,.T.) ;
#47135=EDGE_CURVE('',#36552,#36593,#31175,.T.) ;
#47136=EDGE_CURVE('',#36595,#36552,#31176,.T.) ;
#47137=EDGE_CURVE('',#37847,#37880,#31177,.T.) ;
#47138=EDGE_CURVE('',#37881,#37845,#31178,.T.) ;
#47139=EDGE_CURVE('',#37882,#37843,#31179,.T.) ;
#47140=EDGE_CURVE('',#37849,#37880,#31180,.T.) ;
#47141=EDGE_CURVE('',#37883,#37841,#31181,.T.) ;
#47142=EDGE_CURVE('',#37851,#37879,#31182,.T.) ;
#47143=EDGE_CURVE('',#37884,#37839,#31183,.T.) ;
#47144=EDGE_CURVE('',#37853,#37879,#31184,.T.) ;
#47145=EDGE_CURVE('',#37885,#37837,#31185,.T.) ;
#47146=EDGE_CURVE('',#37855,#37878,#31186,.T.) ;
#47147=EDGE_CURVE('',#37885,#37835,#31187,.T.) ;
#47148=EDGE_CURVE('',#37857,#37878,#31188,.T.) ;
#47149=EDGE_CURVE('',#37886,#36366,#31189,.T.) ;
#47150=EDGE_CURVE('',#37859,#37877,#31190,.T.) ;
#47151=EDGE_CURVE('',#37886,#36365,#31191,.T.) ;
#47152=EDGE_CURVE('',#37861,#37877,#31192,.T.) ;
#47153=EDGE_CURVE('',#37863,#37876,#31193,.T.) ;
#47154=EDGE_CURVE('',#37865,#37876,#31194,.T.) ;
#47155=EDGE_CURVE('',#37887,#37831,#31195,.T.) ;
#47156=EDGE_CURVE('',#37867,#37875,#31196,.T.) ;
#47157=EDGE_CURVE('',#37887,#37829,#31197,.T.) ;
#47158=EDGE_CURVE('',#37869,#37875,#31198,.T.) ;
#47159=EDGE_CURVE('',#37871,#37827,#31199,.T.) ;
#47160=EDGE_CURVE('',#37821,#37874,#31200,.T.) ;
#47161=EDGE_CURVE('',#37872,#37825,#31201,.T.) ;
#47162=EDGE_CURVE('',#37823,#37873,#31202,.T.) ;
#47163=EDGE_CURVE('',#37323,#37226,#31203,.T.) ;
#47164=EDGE_CURVE('',#37217,#37322,#31204,.T.) ;
#47165=EDGE_CURVE('',#37324,#37317,#31205,.T.) ;
#47166=EDGE_CURVE('',#37318,#37323,#31206,.T.) ;
#47167=EDGE_CURVE('',#37324,#38118,#31207,.T.) ;
#47168=EDGE_CURVE('',#38118,#37317,#31208,.T.) ;
#47169=EDGE_CURVE('',#37217,#37327,#31209,.T.) ;
#47170=EDGE_CURVE('',#37327,#37322,#31210,.T.) ;
#47171=EDGE_CURVE('',#37318,#37225,#31211,.T.) ;
#47172=EDGE_CURVE('',#36273,#37320,#31212,.T.) ;
#47173=EDGE_CURVE('',#36274,#38119,#2179,.T.) ;
#47174=EDGE_CURVE('',#38118,#38119,#5143,.T.) ;
#47175=EDGE_CURVE('',#38120,#38118,#2180,.T.) ;
#47176=EDGE_CURVE('',#38120,#38121,#2181,.T.) ;
#47177=EDGE_CURVE('',#36451,#38121,#5144,.T.) ;
#47178=EDGE_CURVE('',#37321,#36450,#31213,.T.) ;
#47179=EDGE_CURVE('',#37328,#37321,#31214,.T.) ;
#47180=EDGE_CURVE('',#37218,#37326,#31215,.T.) ;
#47181=EDGE_CURVE('',#37319,#37224,#31216,.T.) ;
#47182=EDGE_CURVE('',#37320,#36275,#31217,.T.) ;
#47183=EDGE_CURVE('',#37315,#37319,#31218,.T.) ;
#47184=EDGE_CURVE('',#37328,#36459,#31219,.T.) ;
#47185=EDGE_CURVE('',#37218,#36546,#31220,.T.) ;
#47186=EDGE_CURVE('',#36545,#37326,#31221,.T.) ;
#47187=EDGE_CURVE('',#37315,#37223,#31222,.T.) ;
#47188=EDGE_CURVE('',#37325,#36458,#31223,.T.) ;
#47189=EDGE_CURVE('',#36547,#37325,#31224,.T.) ;
#47190=EDGE_CURVE('',#38122,#36546,#5145,.T.) ;
#47191=EDGE_CURVE('',#37219,#38122,#31225,.T.) ;
#47192=EDGE_CURVE('',#37316,#37222,#31226,.T.) ;
#47193=EDGE_CURVE('',#36276,#37311,#31227,.T.) ;
#47194=EDGE_CURVE('',#37312,#37316,#31228,.T.) ;
#47195=EDGE_CURVE('',#36454,#37311,#31229,.T.) ;
#47196=EDGE_CURVE('',#36547,#36458,#31230,.T.) ;
#47197=EDGE_CURVE('',#36594,#36549,#31231,.T.) ;
#47198=EDGE_CURVE('',#36549,#36592,#31232,.T.) ;
#47199=EDGE_CURVE('',#38122,#36709,#31233,.T.) ;
#47200=EDGE_CURVE('',#38123,#38122,#31234,.T.) ;
#47201=EDGE_CURVE('',#37219,#38123,#31235,.T.) ;
#47202=EDGE_CURVE('',#37312,#37222,#31236,.T.) ;
#47203=EDGE_CURVE('',#36455,#37314,#31237,.T.) ;
#47204=EDGE_CURVE('',#36548,#36457,#31238,.T.) ;
#47205=EDGE_CURVE('',#36664,#36548,#31239,.T.) ;
#47206=EDGE_CURVE('',#38123,#36708,#31240,.T.) ;
#47207=EDGE_CURVE('',#38124,#38123,#5146,.T.) ;
#47208=EDGE_CURVE('',#37220,#38124,#31241,.T.) ;
#47209=EDGE_CURVE('',#37313,#37221,#31242,.T.) ;
#47210=EDGE_CURVE('',#37314,#36544,#31243,.T.) ;
#47211=EDGE_CURVE('',#36541,#37313,#31244,.T.) ;
#47212=EDGE_CURVE('',#36455,#36544,#31245,.T.) ;
#47213=EDGE_CURVE('',#36665,#36457,#31246,.T.) ;
#47214=EDGE_CURVE('',#38124,#36707,#31247,.T.) ;
#47215=EDGE_CURVE('',#38125,#38124,#31248,.T.) ;
#47216=EDGE_CURVE('',#37220,#38125,#31249,.T.) ;
#47217=EDGE_CURVE('',#36540,#37221,#31250,.T.) ;
#47218=EDGE_CURVE('',#36456,#36543,#31251,.T.) ;
#47219=EDGE_CURVE('',#36666,#36456,#31252,.T.) ;
#47220=EDGE_CURVE('',#38125,#36706,#31253,.T.) ;
#47221=EDGE_CURVE('',#36540,#38125,#5147,.T.) ;
#47222=EDGE_CURVE('',#36667,#36543,#31254,.T.) ;
#47223=EDGE_CURVE('',#36542,#36597,#31255,.T.) ;
#47224=EDGE_CURVE('',#36599,#36542,#31256,.T.) ;
#47225=EDGE_CURVE('',#37780,#37813,#31257,.T.) ;
#47226=EDGE_CURVE('',#37814,#37778,#31258,.T.) ;
#47227=EDGE_CURVE('',#37815,#37776,#31259,.T.) ;
#47228=EDGE_CURVE('',#37782,#37813,#31260,.T.) ;
#47229=EDGE_CURVE('',#37816,#37774,#31261,.T.) ;
#47230=EDGE_CURVE('',#37784,#37812,#31262,.T.) ;
#47231=EDGE_CURVE('',#37817,#37772,#31263,.T.) ;
#47232=EDGE_CURVE('',#37786,#37812,#31264,.T.) ;
#47233=EDGE_CURVE('',#37818,#37770,#31265,.T.) ;
#47234=EDGE_CURVE('',#37788,#37811,#31266,.T.) ;
#47235=EDGE_CURVE('',#37818,#37768,#31267,.T.) ;
#47236=EDGE_CURVE('',#37790,#37811,#31268,.T.) ;
#47237=EDGE_CURVE('',#37819,#36368,#31269,.T.) ;
#47238=EDGE_CURVE('',#37792,#37810,#31270,.T.) ;
#47239=EDGE_CURVE('',#37819,#36367,#31271,.T.) ;
#47240=EDGE_CURVE('',#37794,#37810,#31272,.T.) ;
#47241=EDGE_CURVE('',#37796,#37809,#31273,.T.) ;
#47242=EDGE_CURVE('',#37798,#37809,#31274,.T.) ;
#47243=EDGE_CURVE('',#37820,#37764,#31275,.T.) ;
#47244=EDGE_CURVE('',#37800,#37808,#31276,.T.) ;
#47245=EDGE_CURVE('',#37820,#37762,#31277,.T.) ;
#47246=EDGE_CURVE('',#37802,#37808,#31278,.T.) ;
#47247=EDGE_CURVE('',#37804,#37760,#31279,.T.) ;
#47248=EDGE_CURVE('',#37754,#37807,#31280,.T.) ;
#47249=EDGE_CURVE('',#37805,#37758,#31281,.T.) ;
#47250=EDGE_CURVE('',#37756,#37806,#31282,.T.) ;
#47251=EDGE_CURVE('',#37341,#37216,#31283,.T.) ;
#47252=EDGE_CURVE('',#37207,#37340,#31284,.T.) ;
#47253=EDGE_CURVE('',#37342,#37335,#31285,.T.) ;
#47254=EDGE_CURVE('',#37336,#37341,#31286,.T.) ;
#47255=EDGE_CURVE('',#37342,#38126,#31287,.T.) ;
#47256=EDGE_CURVE('',#38126,#37335,#31288,.T.) ;
#47257=EDGE_CURVE('',#37207,#37345,#31289,.T.) ;
#47258=EDGE_CURVE('',#37345,#37340,#31290,.T.) ;
#47259=EDGE_CURVE('',#37336,#37215,#31291,.T.) ;
#47260=EDGE_CURVE('',#36258,#37338,#31292,.T.) ;
#47261=EDGE_CURVE('',#36259,#38127,#2182,.T.) ;
#47262=EDGE_CURVE('',#38126,#38127,#5148,.T.) ;
#47263=EDGE_CURVE('',#38128,#38126,#2183,.T.) ;
#47264=EDGE_CURVE('',#38128,#38129,#2184,.T.) ;
#47265=EDGE_CURVE('',#36441,#38129,#5149,.T.) ;
#47266=EDGE_CURVE('',#37339,#36440,#31293,.T.) ;
#47267=EDGE_CURVE('',#37346,#37339,#31294,.T.) ;
#47268=EDGE_CURVE('',#37208,#37344,#31295,.T.) ;
#47269=EDGE_CURVE('',#37337,#37214,#31296,.T.) ;
#47270=EDGE_CURVE('',#37338,#36260,#31297,.T.) ;
#47271=EDGE_CURVE('',#37333,#37337,#31298,.T.) ;
#47272=EDGE_CURVE('',#37346,#36449,#31299,.T.) ;
#47273=EDGE_CURVE('',#37208,#36536,#31300,.T.) ;
#47274=EDGE_CURVE('',#36535,#37344,#31301,.T.) ;
#47275=EDGE_CURVE('',#37333,#37213,#31302,.T.) ;
#47276=EDGE_CURVE('',#37343,#36448,#31303,.T.) ;
#47277=EDGE_CURVE('',#36537,#37343,#31304,.T.) ;
#47278=EDGE_CURVE('',#38130,#36536,#5150,.T.) ;
#47279=EDGE_CURVE('',#37209,#38130,#31305,.T.) ;
#47280=EDGE_CURVE('',#37334,#37212,#31306,.T.) ;
#47281=EDGE_CURVE('',#36261,#37329,#31307,.T.) ;
#47282=EDGE_CURVE('',#37330,#37334,#31308,.T.) ;
#47283=EDGE_CURVE('',#36444,#37329,#31309,.T.) ;
#47284=EDGE_CURVE('',#36537,#36448,#31310,.T.) ;
#47285=EDGE_CURVE('',#36598,#36539,#31311,.T.) ;
#47286=EDGE_CURVE('',#36539,#36596,#31312,.T.) ;
#47287=EDGE_CURVE('',#38130,#36705,#31313,.T.) ;
#47288=EDGE_CURVE('',#38131,#38130,#31314,.T.) ;
#47289=EDGE_CURVE('',#37209,#38131,#31315,.T.) ;
#47290=EDGE_CURVE('',#37330,#37212,#31316,.T.) ;
#47291=EDGE_CURVE('',#36445,#37332,#31317,.T.) ;
#47292=EDGE_CURVE('',#36538,#36447,#31318,.T.) ;
#47293=EDGE_CURVE('',#36668,#36538,#31319,.T.) ;
#47294=EDGE_CURVE('',#38131,#36704,#31320,.T.) ;
#47295=EDGE_CURVE('',#38132,#38131,#5151,.T.) ;
#47296=EDGE_CURVE('',#37210,#38132,#31321,.T.) ;
#47297=EDGE_CURVE('',#37331,#37211,#31322,.T.) ;
#47298=EDGE_CURVE('',#37332,#36534,#31323,.T.) ;
#47299=EDGE_CURVE('',#36531,#37331,#31324,.T.) ;
#47300=EDGE_CURVE('',#36445,#36534,#31325,.T.) ;
#47301=EDGE_CURVE('',#36669,#36447,#31326,.T.) ;
#47302=EDGE_CURVE('',#38132,#36703,#31327,.T.) ;
#47303=EDGE_CURVE('',#38133,#38132,#31328,.T.) ;
#47304=EDGE_CURVE('',#37210,#38133,#31329,.T.) ;
#47305=EDGE_CURVE('',#36530,#37211,#31330,.T.) ;
#47306=EDGE_CURVE('',#36446,#36533,#31331,.T.) ;
#47307=EDGE_CURVE('',#36670,#36446,#31332,.T.) ;
#47308=EDGE_CURVE('',#38133,#36702,#31333,.T.) ;
#47309=EDGE_CURVE('',#36530,#38133,#5152,.T.) ;
#47310=EDGE_CURVE('',#36671,#36533,#31334,.T.) ;
#47311=EDGE_CURVE('',#36532,#36601,#31335,.T.) ;
#47312=EDGE_CURVE('',#36603,#36532,#31336,.T.) ;
#47313=EDGE_CURVE('',#37713,#37746,#31337,.T.) ;
#47314=EDGE_CURVE('',#37747,#37711,#31338,.T.) ;
#47315=EDGE_CURVE('',#37748,#37709,#31339,.T.) ;
#47316=EDGE_CURVE('',#37715,#37746,#31340,.T.) ;
#47317=EDGE_CURVE('',#37749,#37707,#31341,.T.) ;
#47318=EDGE_CURVE('',#37717,#37745,#31342,.T.) ;
#47319=EDGE_CURVE('',#37750,#37705,#31343,.T.) ;
#47320=EDGE_CURVE('',#37719,#37745,#31344,.T.) ;
#47321=EDGE_CURVE('',#37751,#37703,#31345,.T.) ;
#47322=EDGE_CURVE('',#37721,#37744,#31346,.T.) ;
#47323=EDGE_CURVE('',#37751,#37701,#31347,.T.) ;
#47324=EDGE_CURVE('',#37723,#37744,#31348,.T.) ;
#47325=EDGE_CURVE('',#37752,#36370,#31349,.T.) ;
#47326=EDGE_CURVE('',#37725,#37743,#31350,.T.) ;
#47327=EDGE_CURVE('',#37752,#36369,#31351,.T.) ;
#47328=EDGE_CURVE('',#37727,#37743,#31352,.T.) ;
#47329=EDGE_CURVE('',#37729,#37742,#31353,.T.) ;
#47330=EDGE_CURVE('',#37731,#37742,#31354,.T.) ;
#47331=EDGE_CURVE('',#37753,#37697,#31355,.T.) ;
#47332=EDGE_CURVE('',#37733,#37741,#31356,.T.) ;
#47333=EDGE_CURVE('',#37753,#37695,#31357,.T.) ;
#47334=EDGE_CURVE('',#37735,#37741,#31358,.T.) ;
#47335=EDGE_CURVE('',#37737,#37693,#31359,.T.) ;
#47336=EDGE_CURVE('',#37687,#37740,#31360,.T.) ;
#47337=EDGE_CURVE('',#37738,#37691,#31361,.T.) ;
#47338=EDGE_CURVE('',#37689,#37739,#31362,.T.) ;
#47339=EDGE_CURVE('',#37359,#37206,#31363,.T.) ;
#47340=EDGE_CURVE('',#37197,#37358,#31364,.T.) ;
#47341=EDGE_CURVE('',#37360,#37353,#31365,.T.) ;
#47342=EDGE_CURVE('',#37354,#37359,#31366,.T.) ;
#47343=EDGE_CURVE('',#37360,#38134,#31367,.T.) ;
#47344=EDGE_CURVE('',#38134,#37353,#31368,.T.) ;
#47345=EDGE_CURVE('',#37197,#37363,#31369,.T.) ;
#47346=EDGE_CURVE('',#37363,#37358,#31370,.T.) ;
#47347=EDGE_CURVE('',#37354,#37205,#31371,.T.) ;
#47348=EDGE_CURVE('',#36243,#37356,#31372,.T.) ;
#47349=EDGE_CURVE('',#36244,#38135,#2185,.T.) ;
#47350=EDGE_CURVE('',#38134,#38135,#5153,.T.) ;
#47351=EDGE_CURVE('',#38136,#38134,#2186,.T.) ;
#47352=EDGE_CURVE('',#38136,#38137,#2187,.T.) ;
#47353=EDGE_CURVE('',#36431,#38137,#5154,.T.) ;
#47354=EDGE_CURVE('',#37357,#36430,#31373,.T.) ;
#47355=EDGE_CURVE('',#37364,#37357,#31374,.T.) ;
#47356=EDGE_CURVE('',#37198,#37362,#31375,.T.) ;
#47357=EDGE_CURVE('',#37355,#37204,#31376,.T.) ;
#47358=EDGE_CURVE('',#37356,#36245,#31377,.T.) ;
#47359=EDGE_CURVE('',#37351,#37355,#31378,.T.) ;
#47360=EDGE_CURVE('',#37364,#36439,#31379,.T.) ;
#47361=EDGE_CURVE('',#37198,#36526,#31380,.T.) ;
#47362=EDGE_CURVE('',#36525,#37362,#31381,.T.) ;
#47363=EDGE_CURVE('',#37351,#37203,#31382,.T.) ;
#47364=EDGE_CURVE('',#37361,#36438,#31383,.T.) ;
#47365=EDGE_CURVE('',#36527,#37361,#31384,.T.) ;
#47366=EDGE_CURVE('',#38138,#36526,#5155,.T.) ;
#47367=EDGE_CURVE('',#37199,#38138,#31385,.T.) ;
#47368=EDGE_CURVE('',#37352,#37202,#31386,.T.) ;
#47369=EDGE_CURVE('',#36246,#37347,#31387,.T.) ;
#47370=EDGE_CURVE('',#37348,#37352,#31388,.T.) ;
#47371=EDGE_CURVE('',#36434,#37347,#31389,.T.) ;
#47372=EDGE_CURVE('',#36527,#36438,#31390,.T.) ;
#47373=EDGE_CURVE('',#36602,#36529,#31391,.T.) ;
#47374=EDGE_CURVE('',#36529,#36600,#31392,.T.) ;
#47375=EDGE_CURVE('',#38138,#36701,#31393,.T.) ;
#47376=EDGE_CURVE('',#38139,#38138,#31394,.T.) ;
#47377=EDGE_CURVE('',#37199,#38139,#31395,.T.) ;
#47378=EDGE_CURVE('',#37348,#37202,#31396,.T.) ;
#47379=EDGE_CURVE('',#36435,#37350,#31397,.T.) ;
#47380=EDGE_CURVE('',#36528,#36437,#31398,.T.) ;
#47381=EDGE_CURVE('',#36672,#36528,#31399,.T.) ;
#47382=EDGE_CURVE('',#38139,#36700,#31400,.T.) ;
#47383=EDGE_CURVE('',#38140,#38139,#5156,.T.) ;
#47384=EDGE_CURVE('',#37200,#38140,#31401,.T.) ;
#47385=EDGE_CURVE('',#37349,#37201,#31402,.T.) ;
#47386=EDGE_CURVE('',#37350,#36524,#31403,.T.) ;
#47387=EDGE_CURVE('',#36521,#37349,#31404,.T.) ;
#47388=EDGE_CURVE('',#36435,#36524,#31405,.T.) ;
#47389=EDGE_CURVE('',#36673,#36437,#31406,.T.) ;
#47390=EDGE_CURVE('',#38140,#36699,#31407,.T.) ;
#47391=EDGE_CURVE('',#38141,#38140,#31408,.T.) ;
#47392=EDGE_CURVE('',#37200,#38141,#31409,.T.) ;
#47393=EDGE_CURVE('',#36520,#37201,#31410,.T.) ;
#47394=EDGE_CURVE('',#36436,#36523,#31411,.T.) ;
#47395=EDGE_CURVE('',#36674,#36436,#31412,.T.) ;
#47396=EDGE_CURVE('',#38141,#36698,#31413,.T.) ;
#47397=EDGE_CURVE('',#36520,#38141,#5157,.T.) ;
#47398=EDGE_CURVE('',#36675,#36523,#31414,.T.) ;
#47399=EDGE_CURVE('',#36522,#36605,#31415,.T.) ;
#47400=EDGE_CURVE('',#36607,#36522,#31416,.T.) ;
#47401=EDGE_CURVE('',#37646,#37679,#31417,.T.) ;
#47402=EDGE_CURVE('',#37680,#37644,#31418,.T.) ;
#47403=EDGE_CURVE('',#37681,#37642,#31419,.T.) ;
#47404=EDGE_CURVE('',#37648,#37679,#31420,.T.) ;
#47405=EDGE_CURVE('',#37682,#37640,#31421,.T.) ;
#47406=EDGE_CURVE('',#37650,#37678,#31422,.T.) ;
#47407=EDGE_CURVE('',#37683,#37638,#31423,.T.) ;
#47408=EDGE_CURVE('',#37652,#37678,#31424,.T.) ;
#47409=EDGE_CURVE('',#37684,#37636,#31425,.T.) ;
#47410=EDGE_CURVE('',#37654,#37677,#31426,.T.) ;
#47411=EDGE_CURVE('',#37684,#37634,#31427,.T.) ;
#47412=EDGE_CURVE('',#37656,#37677,#31428,.T.) ;
#47413=EDGE_CURVE('',#37685,#36372,#31429,.T.) ;
#47414=EDGE_CURVE('',#37658,#37676,#31430,.T.) ;
#47415=EDGE_CURVE('',#37685,#36371,#31431,.T.) ;
#47416=EDGE_CURVE('',#37660,#37676,#31432,.T.) ;
#47417=EDGE_CURVE('',#37662,#37675,#31433,.T.) ;
#47418=EDGE_CURVE('',#37664,#37675,#31434,.T.) ;
#47419=EDGE_CURVE('',#37686,#37630,#31435,.T.) ;
#47420=EDGE_CURVE('',#37666,#37674,#31436,.T.) ;
#47421=EDGE_CURVE('',#37686,#37628,#31437,.T.) ;
#47422=EDGE_CURVE('',#37668,#37674,#31438,.T.) ;
#47423=EDGE_CURVE('',#37670,#37626,#31439,.T.) ;
#47424=EDGE_CURVE('',#37620,#37673,#31440,.T.) ;
#47425=EDGE_CURVE('',#37671,#37624,#31441,.T.) ;
#47426=EDGE_CURVE('',#37622,#37672,#31442,.T.) ;
#47427=EDGE_CURVE('',#37377,#37196,#31443,.T.) ;
#47428=EDGE_CURVE('',#37187,#37376,#31444,.T.) ;
#47429=EDGE_CURVE('',#37378,#37371,#31445,.T.) ;
#47430=EDGE_CURVE('',#37372,#37377,#31446,.T.) ;
#47431=EDGE_CURVE('',#37378,#38142,#31447,.T.) ;
#47432=EDGE_CURVE('',#38142,#37371,#31448,.T.) ;
#47433=EDGE_CURVE('',#37187,#37381,#31449,.T.) ;
#47434=EDGE_CURVE('',#37381,#37376,#31450,.T.) ;
#47435=EDGE_CURVE('',#37372,#37195,#31451,.T.) ;
#47436=EDGE_CURVE('',#36228,#37374,#31452,.T.) ;
#47437=EDGE_CURVE('',#36229,#38143,#2188,.T.) ;
#47438=EDGE_CURVE('',#38142,#38143,#5158,.T.) ;
#47439=EDGE_CURVE('',#38144,#38142,#2189,.T.) ;
#47440=EDGE_CURVE('',#38144,#38145,#2190,.T.) ;
#47441=EDGE_CURVE('',#36421,#38145,#5159,.T.) ;
#47442=EDGE_CURVE('',#37375,#36420,#31453,.T.) ;
#47443=EDGE_CURVE('',#37382,#37375,#31454,.T.) ;
#47444=EDGE_CURVE('',#37188,#37380,#31455,.T.) ;
#47445=EDGE_CURVE('',#37373,#37194,#31456,.T.) ;
#47446=EDGE_CURVE('',#37374,#36230,#31457,.T.) ;
#47447=EDGE_CURVE('',#37369,#37373,#31458,.T.) ;
#47448=EDGE_CURVE('',#37382,#36429,#31459,.T.) ;
#47449=EDGE_CURVE('',#37188,#36516,#31460,.T.) ;
#47450=EDGE_CURVE('',#36515,#37380,#31461,.T.) ;
#47451=EDGE_CURVE('',#37369,#37193,#31462,.T.) ;
#47452=EDGE_CURVE('',#37379,#36428,#31463,.T.) ;
#47453=EDGE_CURVE('',#36517,#37379,#31464,.T.) ;
#47454=EDGE_CURVE('',#38146,#36516,#5160,.T.) ;
#47455=EDGE_CURVE('',#37189,#38146,#31465,.T.) ;
#47456=EDGE_CURVE('',#37370,#37192,#31466,.T.) ;
#47457=EDGE_CURVE('',#36231,#37365,#31467,.T.) ;
#47458=EDGE_CURVE('',#37366,#37370,#31468,.T.) ;
#47459=EDGE_CURVE('',#36424,#37365,#31469,.T.) ;
#47460=EDGE_CURVE('',#36517,#36428,#31470,.T.) ;
#47461=EDGE_CURVE('',#36606,#36519,#31471,.T.) ;
#47462=EDGE_CURVE('',#36519,#36604,#31472,.T.) ;
#47463=EDGE_CURVE('',#38146,#36697,#31473,.T.) ;
#47464=EDGE_CURVE('',#38147,#38146,#31474,.T.) ;
#47465=EDGE_CURVE('',#37189,#38147,#31475,.T.) ;
#47466=EDGE_CURVE('',#37366,#37192,#31476,.T.) ;
#47467=EDGE_CURVE('',#36425,#37368,#31477,.T.) ;
#47468=EDGE_CURVE('',#36518,#36427,#31478,.T.) ;
#47469=EDGE_CURVE('',#36676,#36518,#31479,.T.) ;
#47470=EDGE_CURVE('',#38147,#36696,#31480,.T.) ;
#47471=EDGE_CURVE('',#38148,#38147,#5161,.T.) ;
#47472=EDGE_CURVE('',#37190,#38148,#31481,.T.) ;
#47473=EDGE_CURVE('',#37367,#37191,#31482,.T.) ;
#47474=EDGE_CURVE('',#37368,#36514,#31483,.T.) ;
#47475=EDGE_CURVE('',#36511,#37367,#31484,.T.) ;
#47476=EDGE_CURVE('',#36425,#36514,#31485,.T.) ;
#47477=EDGE_CURVE('',#36677,#36427,#31486,.T.) ;
#47478=EDGE_CURVE('',#38148,#36695,#31487,.T.) ;
#47479=EDGE_CURVE('',#38149,#38148,#31488,.T.) ;
#47480=EDGE_CURVE('',#37190,#38149,#31489,.T.) ;
#47481=EDGE_CURVE('',#36510,#37191,#31490,.T.) ;
#47482=EDGE_CURVE('',#36426,#36513,#31491,.T.) ;
#47483=EDGE_CURVE('',#36678,#36426,#31492,.T.) ;
#47484=EDGE_CURVE('',#38149,#36694,#31493,.T.) ;
#47485=EDGE_CURVE('',#36510,#38149,#5162,.T.) ;
#47486=EDGE_CURVE('',#36679,#36513,#31494,.T.) ;
#47487=EDGE_CURVE('',#36512,#36609,#31495,.T.) ;
#47488=EDGE_CURVE('',#36611,#36512,#31496,.T.) ;
#47489=EDGE_CURVE('',#37579,#37612,#31497,.T.) ;
#47490=EDGE_CURVE('',#37613,#37577,#31498,.T.) ;
#47491=EDGE_CURVE('',#37614,#37575,#31499,.T.) ;
#47492=EDGE_CURVE('',#37581,#37612,#31500,.T.) ;
#47493=EDGE_CURVE('',#37615,#37573,#31501,.T.) ;
#47494=EDGE_CURVE('',#37583,#37611,#31502,.T.) ;
#47495=EDGE_CURVE('',#37616,#37571,#31503,.T.) ;
#47496=EDGE_CURVE('',#37585,#37611,#31504,.T.) ;
#47497=EDGE_CURVE('',#37617,#37569,#31505,.T.) ;
#47498=EDGE_CURVE('',#37587,#37610,#31506,.T.) ;
#47499=EDGE_CURVE('',#37617,#37567,#31507,.T.) ;
#47500=EDGE_CURVE('',#37589,#37610,#31508,.T.) ;
#47501=EDGE_CURVE('',#37618,#36374,#31509,.T.) ;
#47502=EDGE_CURVE('',#37591,#37609,#31510,.T.) ;
#47503=EDGE_CURVE('',#37618,#36373,#31511,.T.) ;
#47504=EDGE_CURVE('',#37593,#37609,#31512,.T.) ;
#47505=EDGE_CURVE('',#37595,#37608,#31513,.T.) ;
#47506=EDGE_CURVE('',#37597,#37608,#31514,.T.) ;
#47507=EDGE_CURVE('',#37619,#37563,#31515,.T.) ;
#47508=EDGE_CURVE('',#37599,#37607,#31516,.T.) ;
#47509=EDGE_CURVE('',#37619,#37561,#31517,.T.) ;
#47510=EDGE_CURVE('',#37601,#37607,#31518,.T.) ;
#47511=EDGE_CURVE('',#37603,#37559,#31519,.T.) ;
#47512=EDGE_CURVE('',#37553,#37606,#31520,.T.) ;
#47513=EDGE_CURVE('',#37604,#37557,#31521,.T.) ;
#47514=EDGE_CURVE('',#37555,#37605,#31522,.T.) ;
#47515=EDGE_CURVE('',#37395,#37186,#31523,.T.) ;
#47516=EDGE_CURVE('',#37177,#37394,#31524,.T.) ;
#47517=EDGE_CURVE('',#37396,#37389,#31525,.T.) ;
#47518=EDGE_CURVE('',#37390,#37395,#31526,.T.) ;
#47519=EDGE_CURVE('',#37396,#38150,#31527,.T.) ;
#47520=EDGE_CURVE('',#38150,#37389,#31528,.T.) ;
#47521=EDGE_CURVE('',#37177,#37399,#31529,.T.) ;
#47522=EDGE_CURVE('',#37399,#37394,#31530,.T.) ;
#47523=EDGE_CURVE('',#37390,#37185,#31531,.T.) ;
#47524=EDGE_CURVE('',#36213,#37392,#31532,.T.) ;
#47525=EDGE_CURVE('',#36214,#38151,#2191,.T.) ;
#47526=EDGE_CURVE('',#38150,#38151,#5163,.T.) ;
#47527=EDGE_CURVE('',#38152,#38150,#2192,.T.) ;
#47528=EDGE_CURVE('',#38152,#38153,#2193,.T.) ;
#47529=EDGE_CURVE('',#36411,#38153,#5164,.T.) ;
#47530=EDGE_CURVE('',#37393,#36410,#31533,.T.) ;
#47531=EDGE_CURVE('',#37400,#37393,#31534,.T.) ;
#47532=EDGE_CURVE('',#37178,#37398,#31535,.T.) ;
#47533=EDGE_CURVE('',#37391,#37184,#31536,.T.) ;
#47534=EDGE_CURVE('',#37392,#36215,#31537,.T.) ;
#47535=EDGE_CURVE('',#37387,#37391,#31538,.T.) ;
#47536=EDGE_CURVE('',#37400,#36419,#31539,.T.) ;
#47537=EDGE_CURVE('',#37178,#36506,#31540,.T.) ;
#47538=EDGE_CURVE('',#36505,#37398,#31541,.T.) ;
#47539=EDGE_CURVE('',#37387,#37183,#31542,.T.) ;
#47540=EDGE_CURVE('',#37397,#36418,#31543,.T.) ;
#47541=EDGE_CURVE('',#36507,#37397,#31544,.T.) ;
#47542=EDGE_CURVE('',#38154,#36506,#5165,.T.) ;
#47543=EDGE_CURVE('',#37179,#38154,#31545,.T.) ;
#47544=EDGE_CURVE('',#37388,#37182,#31546,.T.) ;
#47545=EDGE_CURVE('',#36216,#37383,#31547,.T.) ;
#47546=EDGE_CURVE('',#37384,#37388,#31548,.T.) ;
#47547=EDGE_CURVE('',#36414,#37383,#31549,.T.) ;
#47548=EDGE_CURVE('',#36507,#36418,#31550,.T.) ;
#47549=EDGE_CURVE('',#36610,#36509,#31551,.T.) ;
#47550=EDGE_CURVE('',#36509,#36608,#31552,.T.) ;
#47551=EDGE_CURVE('',#38154,#36693,#31553,.T.) ;
#47552=EDGE_CURVE('',#38155,#38154,#31554,.T.) ;
#47553=EDGE_CURVE('',#37179,#38155,#31555,.T.) ;
#47554=EDGE_CURVE('',#37384,#37182,#31556,.T.) ;
#47555=EDGE_CURVE('',#36415,#37386,#31557,.T.) ;
#47556=EDGE_CURVE('',#36508,#36417,#31558,.T.) ;
#47557=EDGE_CURVE('',#36680,#36508,#31559,.T.) ;
#47558=EDGE_CURVE('',#38155,#36692,#31560,.T.) ;
#47559=EDGE_CURVE('',#38156,#38155,#5166,.T.) ;
#47560=EDGE_CURVE('',#37180,#38156,#31561,.T.) ;
#47561=EDGE_CURVE('',#37385,#37181,#31562,.T.) ;
#47562=EDGE_CURVE('',#37386,#36504,#31563,.T.) ;
#47563=EDGE_CURVE('',#36501,#37385,#31564,.T.) ;
#47564=EDGE_CURVE('',#36415,#36504,#31565,.T.) ;
#47565=EDGE_CURVE('',#36681,#36417,#31566,.T.) ;
#47566=EDGE_CURVE('',#38156,#36691,#31567,.T.) ;
#47567=EDGE_CURVE('',#38157,#38156,#31568,.T.) ;
#47568=EDGE_CURVE('',#37180,#38157,#31569,.T.) ;
#47569=EDGE_CURVE('',#36500,#37181,#31570,.T.) ;
#47570=EDGE_CURVE('',#36416,#36503,#31571,.T.) ;
#47571=EDGE_CURVE('',#36682,#36416,#31572,.T.) ;
#47572=EDGE_CURVE('',#38157,#36690,#31573,.T.) ;
#47573=EDGE_CURVE('',#36500,#38157,#5167,.T.) ;
#47574=EDGE_CURVE('',#36683,#36503,#31574,.T.) ;
#47575=EDGE_CURVE('',#36502,#36613,#31575,.T.) ;
#47576=EDGE_CURVE('',#36615,#36502,#31576,.T.) ;
#47577=EDGE_CURVE('',#37512,#37545,#31577,.T.) ;
#47578=EDGE_CURVE('',#37546,#37510,#31578,.T.) ;
#47579=EDGE_CURVE('',#37547,#37508,#31579,.T.) ;
#47580=EDGE_CURVE('',#37514,#37545,#31580,.T.) ;
#47581=EDGE_CURVE('',#37548,#37506,#31581,.T.) ;
#47582=EDGE_CURVE('',#37516,#37544,#31582,.T.) ;
#47583=EDGE_CURVE('',#37549,#37504,#31583,.T.) ;
#47584=EDGE_CURVE('',#37518,#37544,#31584,.T.) ;
#47585=EDGE_CURVE('',#37550,#37502,#31585,.T.) ;
#47586=EDGE_CURVE('',#37520,#37543,#31586,.T.) ;
#47587=EDGE_CURVE('',#37550,#37500,#31587,.T.) ;
#47588=EDGE_CURVE('',#37522,#37543,#31588,.T.) ;
#47589=EDGE_CURVE('',#37551,#36376,#31589,.T.) ;
#47590=EDGE_CURVE('',#37524,#37542,#31590,.T.) ;
#47591=EDGE_CURVE('',#37551,#36375,#31591,.T.) ;
#47592=EDGE_CURVE('',#37526,#37542,#31592,.T.) ;
#47593=EDGE_CURVE('',#37528,#37541,#31593,.T.) ;
#47594=EDGE_CURVE('',#37530,#37541,#31594,.T.) ;
#47595=EDGE_CURVE('',#37552,#37496,#31595,.T.) ;
#47596=EDGE_CURVE('',#37532,#37540,#31596,.T.) ;
#47597=EDGE_CURVE('',#37552,#37494,#31597,.T.) ;
#47598=EDGE_CURVE('',#37534,#37540,#31598,.T.) ;
#47599=EDGE_CURVE('',#37536,#37492,#31599,.T.) ;
#47600=EDGE_CURVE('',#37486,#37539,#31600,.T.) ;
#47601=EDGE_CURVE('',#37537,#37490,#31601,.T.) ;
#47602=EDGE_CURVE('',#37488,#37538,#31602,.T.) ;
#47603=EDGE_CURVE('',#37413,#37176,#31603,.T.) ;
#47604=EDGE_CURVE('',#37167,#37412,#31604,.T.) ;
#47605=EDGE_CURVE('',#37414,#37407,#31605,.T.) ;
#47606=EDGE_CURVE('',#37408,#37413,#31606,.T.) ;
#47607=EDGE_CURVE('',#37414,#38158,#31607,.T.) ;
#47608=EDGE_CURVE('',#38158,#37407,#31608,.T.) ;
#47609=EDGE_CURVE('',#37167,#37417,#31609,.T.) ;
#47610=EDGE_CURVE('',#37417,#37412,#31610,.T.) ;
#47611=EDGE_CURVE('',#37408,#37175,#31611,.T.) ;
#47612=EDGE_CURVE('',#36198,#37410,#31612,.T.) ;
#47613=EDGE_CURVE('',#36199,#38159,#2194,.T.) ;
#47614=EDGE_CURVE('',#38158,#38159,#5168,.T.) ;
#47615=EDGE_CURVE('',#38160,#38158,#2195,.T.) ;
#47616=EDGE_CURVE('',#38160,#38161,#2196,.T.) ;
#47617=EDGE_CURVE('',#36401,#38161,#5169,.T.) ;
#47618=EDGE_CURVE('',#37411,#36400,#31613,.T.) ;
#47619=EDGE_CURVE('',#37418,#37411,#31614,.T.) ;
#47620=EDGE_CURVE('',#37168,#37416,#31615,.T.) ;
#47621=EDGE_CURVE('',#37409,#37174,#31616,.T.) ;
#47622=EDGE_CURVE('',#37410,#36200,#31617,.T.) ;
#47623=EDGE_CURVE('',#37405,#37409,#31618,.T.) ;
#47624=EDGE_CURVE('',#37418,#36409,#31619,.T.) ;
#47625=EDGE_CURVE('',#37168,#36496,#31620,.T.) ;
#47626=EDGE_CURVE('',#36495,#37416,#31621,.T.) ;
#47627=EDGE_CURVE('',#37405,#37173,#31622,.T.) ;
#47628=EDGE_CURVE('',#37415,#36408,#31623,.T.) ;
#47629=EDGE_CURVE('',#36497,#37415,#31624,.T.) ;
#47630=EDGE_CURVE('',#38162,#36496,#5170,.T.) ;
#47631=EDGE_CURVE('',#37169,#38162,#31625,.T.) ;
#47632=EDGE_CURVE('',#37406,#37172,#31626,.T.) ;
#47633=EDGE_CURVE('',#36201,#37401,#31627,.T.) ;
#47634=EDGE_CURVE('',#37402,#37406,#31628,.T.) ;
#47635=EDGE_CURVE('',#36404,#37401,#31629,.T.) ;
#47636=EDGE_CURVE('',#36497,#36408,#31630,.T.) ;
#47637=EDGE_CURVE('',#36614,#36499,#31631,.T.) ;
#47638=EDGE_CURVE('',#36499,#36612,#31632,.T.) ;
#47639=EDGE_CURVE('',#38162,#36688,#31633,.T.) ;
#47640=EDGE_CURVE('',#38163,#38162,#31634,.T.) ;
#47641=EDGE_CURVE('',#37169,#38163,#31635,.T.) ;
#47642=EDGE_CURVE('',#37402,#37172,#31636,.T.) ;
#47643=EDGE_CURVE('',#36405,#37404,#31637,.T.) ;
#47644=EDGE_CURVE('',#36498,#36407,#31638,.T.) ;
#47645=EDGE_CURVE('',#36684,#36498,#31639,.T.) ;
#47646=EDGE_CURVE('',#38163,#36689,#31640,.T.) ;
#47647=EDGE_CURVE('',#38164,#38163,#5171,.T.) ;
#47648=EDGE_CURVE('',#37170,#38164,#31641,.T.) ;
#47649=EDGE_CURVE('',#37403,#37171,#31642,.T.) ;
#47650=EDGE_CURVE('',#37404,#36494,#31643,.T.) ;
#47651=EDGE_CURVE('',#36491,#37403,#31644,.T.) ;
#47652=EDGE_CURVE('',#36405,#36494,#31645,.T.) ;
#47653=EDGE_CURVE('',#36685,#36407,#31646,.T.) ;
#47654=EDGE_CURVE('',#38164,#36729,#31647,.T.) ;
#47655=EDGE_CURVE('',#38165,#38164,#31648,.T.) ;
#47656=EDGE_CURVE('',#37170,#38165,#31649,.T.) ;
#47657=EDGE_CURVE('',#36490,#37171,#31650,.T.) ;
#47658=EDGE_CURVE('',#36406,#36493,#31651,.T.) ;
#47659=EDGE_CURVE('',#36645,#36406,#31652,.T.) ;
#47660=EDGE_CURVE('',#38165,#36728,#31653,.T.) ;
#47661=EDGE_CURVE('',#36490,#38165,#5172,.T.) ;
#47662=EDGE_CURVE('',#36644,#36493,#31654,.T.) ;
#47663=EDGE_CURVE('',#36492,#36686,#31655,.T.) ;
#47664=EDGE_CURVE('',#36646,#36492,#31656,.T.) ;
#47665=EDGE_CURVE('',#37445,#37478,#31657,.T.) ;
#47666=EDGE_CURVE('',#37479,#37443,#31658,.T.) ;
#47667=EDGE_CURVE('',#37480,#37441,#31659,.T.) ;
#47668=EDGE_CURVE('',#37447,#37478,#31660,.T.) ;
#47669=EDGE_CURVE('',#37481,#37439,#31661,.T.) ;
#47670=EDGE_CURVE('',#37449,#37477,#31662,.T.) ;
#47671=EDGE_CURVE('',#37482,#37437,#31663,.T.) ;
#47672=EDGE_CURVE('',#37451,#37477,#31664,.T.) ;
#47673=EDGE_CURVE('',#37483,#37435,#31665,.T.) ;
#47674=EDGE_CURVE('',#37453,#37476,#31666,.T.) ;
#47675=EDGE_CURVE('',#37483,#37433,#31667,.T.) ;
#47676=EDGE_CURVE('',#37455,#37476,#31668,.T.) ;
#47677=EDGE_CURVE('',#37484,#36378,#31669,.T.) ;
#47678=EDGE_CURVE('',#37457,#37475,#31670,.T.) ;
#47679=EDGE_CURVE('',#37484,#36377,#31671,.T.) ;
#47680=EDGE_CURVE('',#37459,#37475,#31672,.T.) ;
#47681=EDGE_CURVE('',#37461,#37474,#31673,.T.) ;
#47682=EDGE_CURVE('',#37463,#37474,#31674,.T.) ;
#47683=EDGE_CURVE('',#37485,#37429,#31675,.T.) ;
#47684=EDGE_CURVE('',#37465,#37473,#31676,.T.) ;
#47685=EDGE_CURVE('',#37485,#37427,#31677,.T.) ;
#47686=EDGE_CURVE('',#37467,#37473,#31678,.T.) ;
#47687=EDGE_CURVE('',#37469,#37425,#31679,.T.) ;
#47688=EDGE_CURVE('',#37419,#37472,#31680,.T.) ;
#47689=EDGE_CURVE('',#37470,#37423,#31681,.T.) ;
#47690=EDGE_CURVE('',#37421,#37471,#31682,.T.) ;
#47691=EDGE_CURVE('',#38166,#38167,#5173,.T.) ;
#47692=EDGE_CURVE('',#38167,#38168,#5174,.T.) ;
#47693=EDGE_CURVE('',#38168,#38169,#5175,.T.) ;
#47694=EDGE_CURVE('',#38169,#38166,#5176,.T.) ;
#47695=EDGE_CURVE('',#38170,#38171,#5177,.T.) ;
#47696=EDGE_CURVE('',#38171,#38172,#5178,.T.) ;
#47697=EDGE_CURVE('',#38172,#38173,#5179,.T.) ;
#47698=EDGE_CURVE('',#38173,#38170,#5180,.T.) ;
#47699=EDGE_CURVE('',#38174,#38175,#5181,.T.) ;
#47700=EDGE_CURVE('',#38175,#38176,#5182,.T.) ;
#47701=EDGE_CURVE('',#38176,#38177,#5183,.T.) ;
#47702=EDGE_CURVE('',#38177,#38174,#5184,.T.) ;
#47703=EDGE_CURVE('',#38178,#38179,#5185,.T.) ;
#47704=EDGE_CURVE('',#38179,#38180,#5186,.T.) ;
#47705=EDGE_CURVE('',#38180,#38181,#5187,.T.) ;
#47706=EDGE_CURVE('',#38181,#38178,#5188,.T.) ;
#47707=EDGE_CURVE('',#38182,#38183,#5189,.T.) ;
#47708=EDGE_CURVE('',#38183,#38184,#5190,.T.) ;
#47709=EDGE_CURVE('',#38185,#38184,#5191,.T.) ;
#47710=EDGE_CURVE('',#38185,#38182,#5192,.T.) ;
#47711=EDGE_CURVE('',#38186,#38187,#5193,.T.) ;
#47712=EDGE_CURVE('',#38187,#36481,#31683,.T.) ;
#47713=EDGE_CURVE('',#38097,#38188,#31684,.T.) ;
#47714=EDGE_CURVE('',#38188,#38189,#5194,.T.) ;
#47715=EDGE_CURVE('',#38189,#38186,#5195,.T.) ;
#47716=EDGE_CURVE('',#38190,#38191,#5196,.T.) ;
#47717=EDGE_CURVE('',#38191,#36360,#31685,.T.) ;
#47718=EDGE_CURVE('',#36359,#38192,#31686,.T.) ;
#47719=EDGE_CURVE('',#38192,#38193,#5197,.T.) ;
#47720=EDGE_CURVE('',#38193,#38190,#5198,.T.) ;
#47721=EDGE_CURVE('',#38095,#38167,#31687,.T.) ;
#47722=EDGE_CURVE('',#38166,#38096,#31688,.T.) ;
#47723=EDGE_CURVE('',#38184,#36483,#31689,.T.) ;
#47724=EDGE_CURVE('',#36482,#38185,#31690,.T.) ;
#47725=EDGE_CURVE('',#38194,#38195,#5199,.T.) ;
#47726=EDGE_CURVE('',#38195,#38196,#5200,.T.) ;
#47727=EDGE_CURVE('',#38196,#38197,#5201,.T.) ;
#47728=EDGE_CURVE('',#38197,#38194,#5202,.T.) ;
#47729=EDGE_CURVE('',#38198,#38199,#5203,.T.) ;
#47730=EDGE_CURVE('',#38199,#38025,#5204,.T.) ;
#47731=EDGE_CURVE('',#38024,#38198,#5205,.T.) ;
#47732=EDGE_CURVE('',#38028,#38200,#5206,.T.) ;
#47733=EDGE_CURVE('',#38200,#38201,#5207,.T.) ;
#47734=EDGE_CURVE('',#38201,#38029,#5208,.T.) ;
#47735=EDGE_CURVE('',#38202,#38203,#5209,.T.) ;
#47736=EDGE_CURVE('',#38203,#38204,#5210,.T.) ;
#47737=EDGE_CURVE('',#38204,#38205,#5211,.T.) ;
#47738=EDGE_CURVE('',#38205,#38202,#5212,.T.) ;
#47739=EDGE_CURVE('',#38206,#38207,#5213,.T.) ;
#47740=EDGE_CURVE('',#38207,#38208,#5214,.T.) ;
#47741=EDGE_CURVE('',#38208,#38209,#5215,.T.) ;
#47742=EDGE_CURVE('',#38209,#38206,#5216,.T.) ;
#47743=EDGE_CURVE('',#38210,#38211,#5217,.T.) ;
#47744=EDGE_CURVE('',#38211,#38022,#5218,.T.) ;
#47745=EDGE_CURVE('',#38023,#38210,#5219,.T.) ;
#47746=EDGE_CURVE('',#38026,#38212,#5220,.T.) ;
#47747=EDGE_CURVE('',#38212,#38213,#5221,.T.) ;
#47748=EDGE_CURVE('',#38213,#38027,#5222,.T.) ;
#47749=EDGE_CURVE('',#38214,#38215,#5223,.T.) ;
#47750=EDGE_CURVE('',#38215,#38216,#5224,.T.) ;
#47751=EDGE_CURVE('',#38216,#38217,#5225,.T.) ;
#47752=EDGE_CURVE('',#38217,#38214,#5226,.T.) ;
#47753=EDGE_CURVE('',#38218,#38219,#5227,.T.) ;
#47754=EDGE_CURVE('',#38219,#38220,#5228,.T.) ;
#47755=EDGE_CURVE('',#38220,#38221,#5229,.T.) ;
#47756=EDGE_CURVE('',#38221,#38218,#5230,.T.) ;
#47757=EDGE_CURVE('',#38222,#38223,#5231,.T.) ;
#47758=EDGE_CURVE('',#38223,#38224,#5232,.T.) ;
#47759=EDGE_CURVE('',#38224,#38225,#5233,.T.) ;
#47760=EDGE_CURVE('',#38225,#38222,#5234,.T.) ;
#47761=EDGE_CURVE('',#38226,#38227,#5235,.T.) ;
#47762=EDGE_CURVE('',#38227,#38228,#5236,.T.) ;
#47763=EDGE_CURVE('',#38228,#38229,#5237,.T.) ;
#47764=EDGE_CURVE('',#38229,#38226,#5238,.T.) ;
#47765=EDGE_CURVE('',#38230,#38231,#5239,.T.) ;
#47766=EDGE_CURVE('',#38231,#38232,#5240,.T.) ;
#47767=EDGE_CURVE('',#38233,#38232,#5241,.T.) ;
#47768=EDGE_CURVE('',#38233,#38230,#5242,.T.) ;
#47769=EDGE_CURVE('',#38234,#38235,#5243,.T.) ;
#47770=EDGE_CURVE('',#38235,#36471,#31691,.T.) ;
#47771=EDGE_CURVE('',#38105,#38236,#31692,.T.) ;
#47772=EDGE_CURVE('',#38236,#38237,#5244,.T.) ;
#47773=EDGE_CURVE('',#38237,#38234,#5245,.T.) ;
#47774=EDGE_CURVE('',#38238,#38239,#5246,.T.) ;
#47775=EDGE_CURVE('',#38239,#36309,#31693,.T.) ;
#47776=EDGE_CURVE('',#36308,#38240,#31694,.T.) ;
#47777=EDGE_CURVE('',#38240,#38241,#5247,.T.) ;
#47778=EDGE_CURVE('',#38241,#38238,#5248,.T.) ;
#47779=EDGE_CURVE('',#38103,#38215,#31695,.T.) ;
#47780=EDGE_CURVE('',#38214,#38104,#31696,.T.) ;
#47781=EDGE_CURVE('',#38232,#36473,#31697,.T.) ;
#47782=EDGE_CURVE('',#36472,#38233,#31698,.T.) ;
#47783=EDGE_CURVE('',#38242,#38243,#5249,.T.) ;
#47784=EDGE_CURVE('',#38243,#38244,#5250,.T.) ;
#47785=EDGE_CURVE('',#38244,#38245,#5251,.T.) ;
#47786=EDGE_CURVE('',#38245,#38242,#5252,.T.) ;
#47787=EDGE_CURVE('',#38246,#38247,#5253,.T.) ;
#47788=EDGE_CURVE('',#38247,#38033,#5254,.T.) ;
#47789=EDGE_CURVE('',#38032,#38246,#5255,.T.) ;
#47790=EDGE_CURVE('',#38036,#38248,#5256,.T.) ;
#47791=EDGE_CURVE('',#38248,#38249,#5257,.T.) ;
#47792=EDGE_CURVE('',#38249,#38037,#5258,.T.) ;
#47793=EDGE_CURVE('',#38250,#38251,#5259,.T.) ;
#47794=EDGE_CURVE('',#38251,#38252,#5260,.T.) ;
#47795=EDGE_CURVE('',#38252,#38253,#5261,.T.) ;
#47796=EDGE_CURVE('',#38253,#38250,#5262,.T.) ;
#47797=EDGE_CURVE('',#38254,#38255,#5263,.T.) ;
#47798=EDGE_CURVE('',#38255,#38256,#5264,.T.) ;
#47799=EDGE_CURVE('',#38256,#38257,#5265,.T.) ;
#47800=EDGE_CURVE('',#38257,#38254,#5266,.T.) ;
#47801=EDGE_CURVE('',#38258,#38259,#5267,.T.) ;
#47802=EDGE_CURVE('',#38259,#38030,#5268,.T.) ;
#47803=EDGE_CURVE('',#38031,#38258,#5269,.T.) ;
#47804=EDGE_CURVE('',#38034,#38260,#5270,.T.) ;
#47805=EDGE_CURVE('',#38260,#38261,#5271,.T.) ;
#47806=EDGE_CURVE('',#38261,#38035,#5272,.T.) ;
#47807=EDGE_CURVE('',#38262,#38263,#5273,.T.) ;
#47808=EDGE_CURVE('',#38263,#38264,#5274,.T.) ;
#47809=EDGE_CURVE('',#38264,#38265,#5275,.T.) ;
#47810=EDGE_CURVE('',#38265,#38262,#5276,.T.) ;
#47811=EDGE_CURVE('',#38266,#38267,#5277,.T.) ;
#47812=EDGE_CURVE('',#38267,#38268,#5278,.T.) ;
#47813=EDGE_CURVE('',#38268,#38269,#5279,.T.) ;
#47814=EDGE_CURVE('',#38269,#38266,#5280,.T.) ;
#47815=EDGE_CURVE('',#38270,#38271,#5281,.T.) ;
#47816=EDGE_CURVE('',#38271,#38272,#5282,.T.) ;
#47817=EDGE_CURVE('',#38272,#38273,#5283,.T.) ;
#47818=EDGE_CURVE('',#38273,#38270,#5284,.T.) ;
#47819=EDGE_CURVE('',#38274,#38275,#5285,.T.) ;
#47820=EDGE_CURVE('',#38275,#38276,#5286,.T.) ;
#47821=EDGE_CURVE('',#38276,#38277,#5287,.T.) ;
#47822=EDGE_CURVE('',#38277,#38274,#5288,.T.) ;
#47823=EDGE_CURVE('',#38278,#38279,#5289,.T.) ;
#47824=EDGE_CURVE('',#38279,#38280,#5290,.T.) ;
#47825=EDGE_CURVE('',#38281,#38280,#5291,.T.) ;
#47826=EDGE_CURVE('',#38281,#38278,#5292,.T.) ;
#47827=EDGE_CURVE('',#38282,#38283,#5293,.T.) ;
#47828=EDGE_CURVE('',#38283,#36461,#31699,.T.) ;
#47829=EDGE_CURVE('',#38113,#38284,#31700,.T.) ;
#47830=EDGE_CURVE('',#38284,#38285,#5294,.T.) ;
#47831=EDGE_CURVE('',#38285,#38282,#5295,.T.) ;
#47832=EDGE_CURVE('',#38286,#38287,#5296,.T.) ;
#47833=EDGE_CURVE('',#38287,#36294,#31701,.T.) ;
#47834=EDGE_CURVE('',#36293,#38288,#31702,.T.) ;
#47835=EDGE_CURVE('',#38288,#38289,#5297,.T.) ;
#47836=EDGE_CURVE('',#38289,#38286,#5298,.T.) ;
#47837=EDGE_CURVE('',#38111,#38263,#31703,.T.) ;
#47838=EDGE_CURVE('',#38262,#38112,#31704,.T.) ;
#47839=EDGE_CURVE('',#38280,#36463,#31705,.T.) ;
#47840=EDGE_CURVE('',#36462,#38281,#31706,.T.) ;
#47841=EDGE_CURVE('',#38290,#38291,#5299,.T.) ;
#47842=EDGE_CURVE('',#38291,#38292,#5300,.T.) ;
#47843=EDGE_CURVE('',#38292,#38293,#5301,.T.) ;
#47844=EDGE_CURVE('',#38293,#38290,#5302,.T.) ;
#47845=EDGE_CURVE('',#38294,#38295,#5303,.T.) ;
#47846=EDGE_CURVE('',#38295,#38041,#5304,.T.) ;
#47847=EDGE_CURVE('',#38040,#38294,#5305,.T.) ;
#47848=EDGE_CURVE('',#38044,#38296,#5306,.T.) ;
#47849=EDGE_CURVE('',#38296,#38297,#5307,.T.) ;
#47850=EDGE_CURVE('',#38297,#38045,#5308,.T.) ;
#47851=EDGE_CURVE('',#38298,#38299,#5309,.T.) ;
#47852=EDGE_CURVE('',#38299,#38300,#5310,.T.) ;
#47853=EDGE_CURVE('',#38300,#38301,#5311,.T.) ;
#47854=EDGE_CURVE('',#38301,#38298,#5312,.T.) ;
#47855=EDGE_CURVE('',#38302,#38303,#5313,.T.) ;
#47856=EDGE_CURVE('',#38303,#38304,#5314,.T.) ;
#47857=EDGE_CURVE('',#38304,#38305,#5315,.T.) ;
#47858=EDGE_CURVE('',#38305,#38302,#5316,.T.) ;
#47859=EDGE_CURVE('',#38306,#38307,#5317,.T.) ;
#47860=EDGE_CURVE('',#38307,#38038,#5318,.T.) ;
#47861=EDGE_CURVE('',#38039,#38306,#5319,.T.) ;
#47862=EDGE_CURVE('',#38042,#38308,#5320,.T.) ;
#47863=EDGE_CURVE('',#38308,#38309,#5321,.T.) ;
#47864=EDGE_CURVE('',#38309,#38043,#5322,.T.) ;
#47865=EDGE_CURVE('',#38310,#38311,#5323,.T.) ;
#47866=EDGE_CURVE('',#38311,#38312,#5324,.T.) ;
#47867=EDGE_CURVE('',#38312,#38313,#5325,.T.) ;
#47868=EDGE_CURVE('',#38313,#38310,#5326,.T.) ;
#47869=EDGE_CURVE('',#38314,#38315,#5327,.T.) ;
#47870=EDGE_CURVE('',#38315,#38316,#5328,.T.) ;
#47871=EDGE_CURVE('',#38316,#38317,#5329,.T.) ;
#47872=EDGE_CURVE('',#38317,#38314,#5330,.T.) ;
#47873=EDGE_CURVE('',#38318,#38319,#5331,.T.) ;
#47874=EDGE_CURVE('',#38319,#38320,#5332,.T.) ;
#47875=EDGE_CURVE('',#38320,#38321,#5333,.T.) ;
#47876=EDGE_CURVE('',#38321,#38318,#5334,.T.) ;
#47877=EDGE_CURVE('',#38322,#38323,#5335,.T.) ;
#47878=EDGE_CURVE('',#38323,#38324,#5336,.T.) ;
#47879=EDGE_CURVE('',#38324,#38325,#5337,.T.) ;
#47880=EDGE_CURVE('',#38325,#38322,#5338,.T.) ;
#47881=EDGE_CURVE('',#38326,#38327,#5339,.T.) ;
#47882=EDGE_CURVE('',#38327,#38328,#5340,.T.) ;
#47883=EDGE_CURVE('',#38329,#38328,#5341,.T.) ;
#47884=EDGE_CURVE('',#38329,#38326,#5342,.T.) ;
#47885=EDGE_CURVE('',#38330,#38331,#5343,.T.) ;
#47886=EDGE_CURVE('',#38331,#36451,#31707,.T.) ;
#47887=EDGE_CURVE('',#38121,#38332,#31708,.T.) ;
#47888=EDGE_CURVE('',#38332,#38333,#5344,.T.) ;
#47889=EDGE_CURVE('',#38333,#38330,#5345,.T.) ;
#47890=EDGE_CURVE('',#38334,#38335,#5346,.T.) ;
#47891=EDGE_CURVE('',#38335,#36279,#31709,.T.) ;
#47892=EDGE_CURVE('',#36278,#38336,#31710,.T.) ;
#47893=EDGE_CURVE('',#38336,#38337,#5347,.T.) ;
#47894=EDGE_CURVE('',#38337,#38334,#5348,.T.) ;
#47895=EDGE_CURVE('',#38119,#38311,#31711,.T.) ;
#47896=EDGE_CURVE('',#38310,#38120,#31712,.T.) ;
#47897=EDGE_CURVE('',#38328,#36453,#31713,.T.) ;
#47898=EDGE_CURVE('',#36452,#38329,#31714,.T.) ;
#47899=EDGE_CURVE('',#38338,#38339,#5349,.T.) ;
#47900=EDGE_CURVE('',#38339,#38340,#5350,.T.) ;
#47901=EDGE_CURVE('',#38340,#38341,#5351,.T.) ;
#47902=EDGE_CURVE('',#38341,#38338,#5352,.T.) ;
#47903=EDGE_CURVE('',#38342,#38343,#5353,.T.) ;
#47904=EDGE_CURVE('',#38343,#38049,#5354,.T.) ;
#47905=EDGE_CURVE('',#38048,#38342,#5355,.T.) ;
#47906=EDGE_CURVE('',#38052,#38344,#5356,.T.) ;
#47907=EDGE_CURVE('',#38344,#38345,#5357,.T.) ;
#47908=EDGE_CURVE('',#38345,#38053,#5358,.T.) ;
#47909=EDGE_CURVE('',#38346,#38347,#5359,.T.) ;
#47910=EDGE_CURVE('',#38347,#38348,#5360,.T.) ;
#47911=EDGE_CURVE('',#38348,#38349,#5361,.T.) ;
#47912=EDGE_CURVE('',#38349,#38346,#5362,.T.) ;
#47913=EDGE_CURVE('',#38350,#38351,#5363,.T.) ;
#47914=EDGE_CURVE('',#38351,#38352,#5364,.T.) ;
#47915=EDGE_CURVE('',#38352,#38353,#5365,.T.) ;
#47916=EDGE_CURVE('',#38353,#38350,#5366,.T.) ;
#47917=EDGE_CURVE('',#38354,#38355,#5367,.T.) ;
#47918=EDGE_CURVE('',#38355,#38046,#5368,.T.) ;
#47919=EDGE_CURVE('',#38047,#38354,#5369,.T.) ;
#47920=EDGE_CURVE('',#38050,#38356,#5370,.T.) ;
#47921=EDGE_CURVE('',#38356,#38357,#5371,.T.) ;
#47922=EDGE_CURVE('',#38357,#38051,#5372,.T.) ;
#47923=EDGE_CURVE('',#38358,#38359,#5373,.T.) ;
#47924=EDGE_CURVE('',#38359,#38360,#5374,.T.) ;
#47925=EDGE_CURVE('',#38360,#38361,#5375,.T.) ;
#47926=EDGE_CURVE('',#38361,#38358,#5376,.T.) ;
#47927=EDGE_CURVE('',#38362,#38363,#5377,.T.) ;
#47928=EDGE_CURVE('',#38363,#38364,#5378,.T.) ;
#47929=EDGE_CURVE('',#38364,#38365,#5379,.T.) ;
#47930=EDGE_CURVE('',#38365,#38362,#5380,.T.) ;
#47931=EDGE_CURVE('',#38366,#38367,#5381,.T.) ;
#47932=EDGE_CURVE('',#38367,#38368,#5382,.T.) ;
#47933=EDGE_CURVE('',#38368,#38369,#5383,.T.) ;
#47934=EDGE_CURVE('',#38369,#38366,#5384,.T.) ;
#47935=EDGE_CURVE('',#38370,#38371,#5385,.T.) ;
#47936=EDGE_CURVE('',#38371,#38372,#5386,.T.) ;
#47937=EDGE_CURVE('',#38372,#38373,#5387,.T.) ;
#47938=EDGE_CURVE('',#38373,#38370,#5388,.T.) ;
#47939=EDGE_CURVE('',#38374,#38375,#5389,.T.) ;
#47940=EDGE_CURVE('',#38375,#38376,#5390,.T.) ;
#47941=EDGE_CURVE('',#38377,#38376,#5391,.T.) ;
#47942=EDGE_CURVE('',#38377,#38374,#5392,.T.) ;
#47943=EDGE_CURVE('',#38378,#38379,#5393,.T.) ;
#47944=EDGE_CURVE('',#38379,#36441,#31715,.T.) ;
#47945=EDGE_CURVE('',#38129,#38380,#31716,.T.) ;
#47946=EDGE_CURVE('',#38380,#38381,#5394,.T.) ;
#47947=EDGE_CURVE('',#38381,#38378,#5395,.T.) ;
#47948=EDGE_CURVE('',#38382,#38383,#5396,.T.) ;
#47949=EDGE_CURVE('',#38383,#36264,#31717,.T.) ;
#47950=EDGE_CURVE('',#36263,#38384,#31718,.T.) ;
#47951=EDGE_CURVE('',#38384,#38385,#5397,.T.) ;
#47952=EDGE_CURVE('',#38385,#38382,#5398,.T.) ;
#47953=EDGE_CURVE('',#38127,#38359,#31719,.T.) ;
#47954=EDGE_CURVE('',#38358,#38128,#31720,.T.) ;
#47955=EDGE_CURVE('',#38376,#36443,#31721,.T.) ;
#47956=EDGE_CURVE('',#36442,#38377,#31722,.T.) ;
#47957=EDGE_CURVE('',#38386,#38387,#5399,.T.) ;
#47958=EDGE_CURVE('',#38387,#38388,#5400,.T.) ;
#47959=EDGE_CURVE('',#38388,#38389,#5401,.T.) ;
#47960=EDGE_CURVE('',#38389,#38386,#5402,.T.) ;
#47961=EDGE_CURVE('',#38390,#38391,#5403,.T.) ;
#47962=EDGE_CURVE('',#38391,#38057,#5404,.T.) ;
#47963=EDGE_CURVE('',#38056,#38390,#5405,.T.) ;
#47964=EDGE_CURVE('',#38060,#38392,#5406,.T.) ;
#47965=EDGE_CURVE('',#38392,#38393,#5407,.T.) ;
#47966=EDGE_CURVE('',#38393,#38061,#5408,.T.) ;
#47967=EDGE_CURVE('',#38394,#38395,#5409,.T.) ;
#47968=EDGE_CURVE('',#38395,#38396,#5410,.T.) ;
#47969=EDGE_CURVE('',#38396,#38397,#5411,.T.) ;
#47970=EDGE_CURVE('',#38397,#38394,#5412,.T.) ;
#47971=EDGE_CURVE('',#38398,#38399,#5413,.T.) ;
#47972=EDGE_CURVE('',#38399,#38400,#5414,.T.) ;
#47973=EDGE_CURVE('',#38400,#38401,#5415,.T.) ;
#47974=EDGE_CURVE('',#38401,#38398,#5416,.T.) ;
#47975=EDGE_CURVE('',#38402,#38403,#5417,.T.) ;
#47976=EDGE_CURVE('',#38403,#38054,#5418,.T.) ;
#47977=EDGE_CURVE('',#38055,#38402,#5419,.T.) ;
#47978=EDGE_CURVE('',#38058,#38404,#5420,.T.) ;
#47979=EDGE_CURVE('',#38404,#38405,#5421,.T.) ;
#47980=EDGE_CURVE('',#38405,#38059,#5422,.T.) ;
#47981=EDGE_CURVE('',#38406,#38407,#5423,.T.) ;
#47982=EDGE_CURVE('',#38407,#38408,#5424,.T.) ;
#47983=EDGE_CURVE('',#38408,#38409,#5425,.T.) ;
#47984=EDGE_CURVE('',#38409,#38406,#5426,.T.) ;
#47985=EDGE_CURVE('',#38410,#38411,#5427,.T.) ;
#47986=EDGE_CURVE('',#38411,#38412,#5428,.T.) ;
#47987=EDGE_CURVE('',#38412,#38413,#5429,.T.) ;
#47988=EDGE_CURVE('',#38413,#38410,#5430,.T.) ;
#47989=EDGE_CURVE('',#38414,#38415,#5431,.T.) ;
#47990=EDGE_CURVE('',#38415,#38416,#5432,.T.) ;
#47991=EDGE_CURVE('',#38416,#38417,#5433,.T.) ;
#47992=EDGE_CURVE('',#38417,#38414,#5434,.T.) ;
#47993=EDGE_CURVE('',#38418,#38419,#5435,.T.) ;
#47994=EDGE_CURVE('',#38419,#38420,#5436,.T.) ;
#47995=EDGE_CURVE('',#38420,#38421,#5437,.T.) ;
#47996=EDGE_CURVE('',#38421,#38418,#5438,.T.) ;
#47997=EDGE_CURVE('',#38422,#38423,#5439,.T.) ;
#47998=EDGE_CURVE('',#38423,#38424,#5440,.T.) ;
#47999=EDGE_CURVE('',#38425,#38424,#5441,.T.) ;
#48000=EDGE_CURVE('',#38425,#38422,#5442,.T.) ;
#48001=EDGE_CURVE('',#38426,#38427,#5443,.T.) ;
#48002=EDGE_CURVE('',#38427,#36431,#31723,.T.) ;
#48003=EDGE_CURVE('',#38137,#38428,#31724,.T.) ;
#48004=EDGE_CURVE('',#38428,#38429,#5444,.T.) ;
#48005=EDGE_CURVE('',#38429,#38426,#5445,.T.) ;
#48006=EDGE_CURVE('',#38430,#38431,#5446,.T.) ;
#48007=EDGE_CURVE('',#38431,#36249,#31725,.T.) ;
#48008=EDGE_CURVE('',#36248,#38432,#31726,.T.) ;
#48009=EDGE_CURVE('',#38432,#38433,#5447,.T.) ;
#48010=EDGE_CURVE('',#38433,#38430,#5448,.T.) ;
#48011=EDGE_CURVE('',#38135,#38407,#31727,.T.) ;
#48012=EDGE_CURVE('',#38406,#38136,#31728,.T.) ;
#48013=EDGE_CURVE('',#38424,#36433,#31729,.T.) ;
#48014=EDGE_CURVE('',#36432,#38425,#31730,.T.) ;
#48015=EDGE_CURVE('',#38434,#38435,#5449,.T.) ;
#48016=EDGE_CURVE('',#38435,#38436,#5450,.T.) ;
#48017=EDGE_CURVE('',#38436,#38437,#5451,.T.) ;
#48018=EDGE_CURVE('',#38437,#38434,#5452,.T.) ;
#48019=EDGE_CURVE('',#38438,#38439,#5453,.T.) ;
#48020=EDGE_CURVE('',#38439,#38065,#5454,.T.) ;
#48021=EDGE_CURVE('',#38064,#38438,#5455,.T.) ;
#48022=EDGE_CURVE('',#38068,#38440,#5456,.T.) ;
#48023=EDGE_CURVE('',#38440,#38441,#5457,.T.) ;
#48024=EDGE_CURVE('',#38441,#38069,#5458,.T.) ;
#48025=EDGE_CURVE('',#38442,#38443,#5459,.T.) ;
#48026=EDGE_CURVE('',#38443,#38444,#5460,.T.) ;
#48027=EDGE_CURVE('',#38444,#38445,#5461,.T.) ;
#48028=EDGE_CURVE('',#38445,#38442,#5462,.T.) ;
#48029=EDGE_CURVE('',#38446,#38447,#5463,.T.) ;
#48030=EDGE_CURVE('',#38447,#38448,#5464,.T.) ;
#48031=EDGE_CURVE('',#38448,#38449,#5465,.T.) ;
#48032=EDGE_CURVE('',#38449,#38446,#5466,.T.) ;
#48033=EDGE_CURVE('',#38450,#38451,#5467,.T.) ;
#48034=EDGE_CURVE('',#38451,#38062,#5468,.T.) ;
#48035=EDGE_CURVE('',#38063,#38450,#5469,.T.) ;
#48036=EDGE_CURVE('',#38066,#38452,#5470,.T.) ;
#48037=EDGE_CURVE('',#38452,#38453,#5471,.T.) ;
#48038=EDGE_CURVE('',#38453,#38067,#5472,.T.) ;
#48039=EDGE_CURVE('',#38454,#38455,#5473,.T.) ;
#48040=EDGE_CURVE('',#38455,#38456,#5474,.T.) ;
#48041=EDGE_CURVE('',#38456,#38457,#5475,.T.) ;
#48042=EDGE_CURVE('',#38457,#38454,#5476,.T.) ;
#48043=EDGE_CURVE('',#38458,#38459,#5477,.T.) ;
#48044=EDGE_CURVE('',#38459,#38460,#5478,.T.) ;
#48045=EDGE_CURVE('',#38460,#38461,#5479,.T.) ;
#48046=EDGE_CURVE('',#38461,#38458,#5480,.T.) ;
#48047=EDGE_CURVE('',#38462,#38463,#5481,.T.) ;
#48048=EDGE_CURVE('',#38463,#38464,#5482,.T.) ;
#48049=EDGE_CURVE('',#38464,#38465,#5483,.T.) ;
#48050=EDGE_CURVE('',#38465,#38462,#5484,.T.) ;
#48051=EDGE_CURVE('',#38466,#38467,#5485,.T.) ;
#48052=EDGE_CURVE('',#38467,#38468,#5486,.T.) ;
#48053=EDGE_CURVE('',#38468,#38469,#5487,.T.) ;
#48054=EDGE_CURVE('',#38469,#38466,#5488,.T.) ;
#48055=EDGE_CURVE('',#38470,#38471,#5489,.T.) ;
#48056=EDGE_CURVE('',#38471,#38472,#5490,.T.) ;
#48057=EDGE_CURVE('',#38473,#38472,#5491,.T.) ;
#48058=EDGE_CURVE('',#38473,#38470,#5492,.T.) ;
#48059=EDGE_CURVE('',#38474,#38475,#5493,.T.) ;
#48060=EDGE_CURVE('',#38475,#36421,#31731,.T.) ;
#48061=EDGE_CURVE('',#38145,#38476,#31732,.T.) ;
#48062=EDGE_CURVE('',#38476,#38477,#5494,.T.) ;
#48063=EDGE_CURVE('',#38477,#38474,#5495,.T.) ;
#48064=EDGE_CURVE('',#38478,#38479,#5496,.T.) ;
#48065=EDGE_CURVE('',#38479,#36234,#31733,.T.) ;
#48066=EDGE_CURVE('',#36233,#38480,#31734,.T.) ;
#48067=EDGE_CURVE('',#38480,#38481,#5497,.T.) ;
#48068=EDGE_CURVE('',#38481,#38478,#5498,.T.) ;
#48069=EDGE_CURVE('',#38143,#38455,#31735,.T.) ;
#48070=EDGE_CURVE('',#38454,#38144,#31736,.T.) ;
#48071=EDGE_CURVE('',#38472,#36423,#31737,.T.) ;
#48072=EDGE_CURVE('',#36422,#38473,#31738,.T.) ;
#48073=EDGE_CURVE('',#38482,#38483,#5499,.T.) ;
#48074=EDGE_CURVE('',#38483,#38484,#5500,.T.) ;
#48075=EDGE_CURVE('',#38484,#38485,#5501,.T.) ;
#48076=EDGE_CURVE('',#38485,#38482,#5502,.T.) ;
#48077=EDGE_CURVE('',#38486,#38487,#5503,.T.) ;
#48078=EDGE_CURVE('',#38487,#38073,#5504,.T.) ;
#48079=EDGE_CURVE('',#38072,#38486,#5505,.T.) ;
#48080=EDGE_CURVE('',#38076,#38488,#5506,.T.) ;
#48081=EDGE_CURVE('',#38488,#38489,#5507,.T.) ;
#48082=EDGE_CURVE('',#38489,#38077,#5508,.T.) ;
#48083=EDGE_CURVE('',#38490,#38491,#5509,.T.) ;
#48084=EDGE_CURVE('',#38491,#38492,#5510,.T.) ;
#48085=EDGE_CURVE('',#38492,#38493,#5511,.T.) ;
#48086=EDGE_CURVE('',#38493,#38490,#5512,.T.) ;
#48087=EDGE_CURVE('',#38494,#38495,#5513,.T.) ;
#48088=EDGE_CURVE('',#38495,#38496,#5514,.T.) ;
#48089=EDGE_CURVE('',#38496,#38497,#5515,.T.) ;
#48090=EDGE_CURVE('',#38497,#38494,#5516,.T.) ;
#48091=EDGE_CURVE('',#38498,#38499,#5517,.T.) ;
#48092=EDGE_CURVE('',#38499,#38070,#5518,.T.) ;
#48093=EDGE_CURVE('',#38071,#38498,#5519,.T.) ;
#48094=EDGE_CURVE('',#38074,#38500,#5520,.T.) ;
#48095=EDGE_CURVE('',#38500,#38501,#5521,.T.) ;
#48096=EDGE_CURVE('',#38501,#38075,#5522,.T.) ;
#48097=EDGE_CURVE('',#38502,#38503,#5523,.T.) ;
#48098=EDGE_CURVE('',#38503,#38504,#5524,.T.) ;
#48099=EDGE_CURVE('',#38504,#38505,#5525,.T.) ;
#48100=EDGE_CURVE('',#38505,#38502,#5526,.T.) ;
#48101=EDGE_CURVE('',#38506,#38507,#5527,.T.) ;
#48102=EDGE_CURVE('',#38507,#38508,#5528,.T.) ;
#48103=EDGE_CURVE('',#38508,#38509,#5529,.T.) ;
#48104=EDGE_CURVE('',#38509,#38506,#5530,.T.) ;
#48105=EDGE_CURVE('',#38510,#38511,#5531,.T.) ;
#48106=EDGE_CURVE('',#38511,#38512,#5532,.T.) ;
#48107=EDGE_CURVE('',#38512,#38513,#5533,.T.) ;
#48108=EDGE_CURVE('',#38513,#38510,#5534,.T.) ;
#48109=EDGE_CURVE('',#38514,#38515,#5535,.T.) ;
#48110=EDGE_CURVE('',#38515,#38516,#5536,.T.) ;
#48111=EDGE_CURVE('',#38516,#38517,#5537,.T.) ;
#48112=EDGE_CURVE('',#38517,#38514,#5538,.T.) ;
#48113=EDGE_CURVE('',#38518,#38519,#5539,.T.) ;
#48114=EDGE_CURVE('',#38519,#38520,#5540,.T.) ;
#48115=EDGE_CURVE('',#38521,#38520,#5541,.T.) ;
#48116=EDGE_CURVE('',#38521,#38518,#5542,.T.) ;
#48117=EDGE_CURVE('',#38522,#38523,#5543,.T.) ;
#48118=EDGE_CURVE('',#38523,#36411,#31739,.T.) ;
#48119=EDGE_CURVE('',#38153,#38524,#31740,.T.) ;
#48120=EDGE_CURVE('',#38524,#38525,#5544,.T.) ;
#48121=EDGE_CURVE('',#38525,#38522,#5545,.T.) ;
#48122=EDGE_CURVE('',#38526,#38527,#5546,.T.) ;
#48123=EDGE_CURVE('',#38527,#36219,#31741,.T.) ;
#48124=EDGE_CURVE('',#36218,#38528,#31742,.T.) ;
#48125=EDGE_CURVE('',#38528,#38529,#5547,.T.) ;
#48126=EDGE_CURVE('',#38529,#38526,#5548,.T.) ;
#48127=EDGE_CURVE('',#38151,#38503,#31743,.T.) ;
#48128=EDGE_CURVE('',#38502,#38152,#31744,.T.) ;
#48129=EDGE_CURVE('',#38520,#36413,#31745,.T.) ;
#48130=EDGE_CURVE('',#36412,#38521,#31746,.T.) ;
#48131=EDGE_CURVE('',#38530,#38531,#5549,.T.) ;
#48132=EDGE_CURVE('',#38531,#38532,#5550,.T.) ;
#48133=EDGE_CURVE('',#38532,#38533,#5551,.T.) ;
#48134=EDGE_CURVE('',#38533,#38530,#5552,.T.) ;
#48135=EDGE_CURVE('',#38534,#38535,#5553,.T.) ;
#48136=EDGE_CURVE('',#38535,#38081,#5554,.T.) ;
#48137=EDGE_CURVE('',#38080,#38534,#5555,.T.) ;
#48138=EDGE_CURVE('',#38084,#38536,#5556,.T.) ;
#48139=EDGE_CURVE('',#38536,#38537,#5557,.T.) ;
#48140=EDGE_CURVE('',#38537,#38085,#5558,.T.) ;
#48141=EDGE_CURVE('',#38538,#38539,#5559,.T.) ;
#48142=EDGE_CURVE('',#38539,#38540,#5560,.T.) ;
#48143=EDGE_CURVE('',#38540,#38541,#5561,.T.) ;
#48144=EDGE_CURVE('',#38541,#38538,#5562,.T.) ;
#48145=EDGE_CURVE('',#38542,#38543,#5563,.T.) ;
#48146=EDGE_CURVE('',#38543,#38544,#5564,.T.) ;
#48147=EDGE_CURVE('',#38544,#38545,#5565,.T.) ;
#48148=EDGE_CURVE('',#38545,#38542,#5566,.T.) ;
#48149=EDGE_CURVE('',#38546,#38547,#5567,.T.) ;
#48150=EDGE_CURVE('',#38547,#38078,#5568,.T.) ;
#48151=EDGE_CURVE('',#38079,#38546,#5569,.T.) ;
#48152=EDGE_CURVE('',#38082,#38548,#5570,.T.) ;
#48153=EDGE_CURVE('',#38548,#38549,#5571,.T.) ;
#48154=EDGE_CURVE('',#38549,#38083,#5572,.T.) ;
#48155=EDGE_CURVE('',#38550,#38551,#5573,.T.) ;
#48156=EDGE_CURVE('',#38551,#38552,#5574,.T.) ;
#48157=EDGE_CURVE('',#38552,#38553,#5575,.T.) ;
#48158=EDGE_CURVE('',#38553,#38550,#5576,.T.) ;
#48159=EDGE_CURVE('',#38554,#38555,#5577,.T.) ;
#48160=EDGE_CURVE('',#38555,#38556,#5578,.T.) ;
#48161=EDGE_CURVE('',#38556,#38557,#5579,.T.) ;
#48162=EDGE_CURVE('',#38557,#38554,#5580,.T.) ;
#48163=EDGE_CURVE('',#38558,#38559,#5581,.T.) ;
#48164=EDGE_CURVE('',#38559,#38560,#5582,.T.) ;
#48165=EDGE_CURVE('',#38560,#38561,#5583,.T.) ;
#48166=EDGE_CURVE('',#38561,#38558,#5584,.T.) ;
#48167=EDGE_CURVE('',#38562,#38563,#5585,.T.) ;
#48168=EDGE_CURVE('',#38563,#38564,#5586,.T.) ;
#48169=EDGE_CURVE('',#38564,#38565,#5587,.T.) ;
#48170=EDGE_CURVE('',#38565,#38562,#5588,.T.) ;
#48171=EDGE_CURVE('',#38566,#38567,#5589,.T.) ;
#48172=EDGE_CURVE('',#38567,#38568,#5590,.T.) ;
#48173=EDGE_CURVE('',#38569,#38568,#5591,.T.) ;
#48174=EDGE_CURVE('',#38569,#38566,#5592,.T.) ;
#48175=EDGE_CURVE('',#38570,#38571,#5593,.T.) ;
#48176=EDGE_CURVE('',#38571,#36401,#31747,.T.) ;
#48177=EDGE_CURVE('',#38161,#38572,#31748,.T.) ;
#48178=EDGE_CURVE('',#38572,#38573,#5594,.T.) ;
#48179=EDGE_CURVE('',#38573,#38570,#5595,.T.) ;
#48180=EDGE_CURVE('',#38574,#38575,#5596,.T.) ;
#48181=EDGE_CURVE('',#38575,#36204,#31749,.T.) ;
#48182=EDGE_CURVE('',#36203,#38576,#31750,.T.) ;
#48183=EDGE_CURVE('',#38576,#38577,#5597,.T.) ;
#48184=EDGE_CURVE('',#38577,#38574,#5598,.T.) ;
#48185=EDGE_CURVE('',#38159,#38551,#31751,.T.) ;
#48186=EDGE_CURVE('',#38550,#38160,#31752,.T.) ;
#48187=EDGE_CURVE('',#38568,#36403,#31753,.T.) ;
#48188=EDGE_CURVE('',#36402,#38569,#31754,.T.) ;
#48189=EDGE_CURVE('',#38578,#38579,#5599,.T.) ;
#48190=EDGE_CURVE('',#38579,#38580,#5600,.T.) ;
#48191=EDGE_CURVE('',#38580,#38581,#5601,.T.) ;
#48192=EDGE_CURVE('',#38581,#38578,#5602,.T.) ;
#48193=EDGE_CURVE('',#38582,#38583,#5603,.T.) ;
#48194=EDGE_CURVE('',#38583,#38089,#5604,.T.) ;
#48195=EDGE_CURVE('',#38088,#38582,#5605,.T.) ;
#48196=EDGE_CURVE('',#38092,#38584,#5606,.T.) ;
#48197=EDGE_CURVE('',#38584,#38585,#5607,.T.) ;
#48198=EDGE_CURVE('',#38585,#38093,#5608,.T.) ;
#48199=EDGE_CURVE('',#38586,#38587,#5609,.T.) ;
#48200=EDGE_CURVE('',#38587,#38588,#5610,.T.) ;
#48201=EDGE_CURVE('',#38588,#38589,#5611,.T.) ;
#48202=EDGE_CURVE('',#38589,#38586,#5612,.T.) ;
#48203=EDGE_CURVE('',#38590,#38591,#5613,.T.) ;
#48204=EDGE_CURVE('',#38591,#38592,#5614,.T.) ;
#48205=EDGE_CURVE('',#38592,#38593,#5615,.T.) ;
#48206=EDGE_CURVE('',#38593,#38590,#5616,.T.) ;
#48207=EDGE_CURVE('',#38594,#38595,#5617,.T.) ;
#48208=EDGE_CURVE('',#38595,#38086,#5618,.T.) ;
#48209=EDGE_CURVE('',#38087,#38594,#5619,.T.) ;
#48210=EDGE_CURVE('',#38090,#38596,#5620,.T.) ;
#48211=EDGE_CURVE('',#38596,#38597,#5621,.T.) ;
#48212=EDGE_CURVE('',#38597,#38091,#5622,.T.) ;
#48213=EDGE_CURVE('',#38598,#38599,#5623,.T.) ;
#48214=EDGE_CURVE('',#38599,#38600,#5624,.T.) ;
#48215=EDGE_CURVE('',#38600,#38601,#5625,.T.) ;
#48216=EDGE_CURVE('',#38601,#38598,#5626,.T.) ;
#48217=EDGE_CURVE('',#38602,#38603,#5627,.T.) ;
#48218=EDGE_CURVE('',#38603,#38604,#5628,.T.) ;
#48219=EDGE_CURVE('',#38604,#38605,#5629,.T.) ;
#48220=EDGE_CURVE('',#38605,#38602,#5630,.T.) ;
#48221=EDGE_CURVE('',#38606,#38607,#5631,.T.) ;
#48222=EDGE_CURVE('',#38607,#38608,#5632,.T.) ;
#48223=EDGE_CURVE('',#38608,#38609,#5633,.T.) ;
#48224=EDGE_CURVE('',#38609,#38606,#5634,.T.) ;
#48225=EDGE_CURVE('',#38610,#38611,#5635,.T.) ;
#48226=EDGE_CURVE('',#38611,#38612,#5636,.T.) ;
#48227=EDGE_CURVE('',#38612,#38613,#5637,.T.) ;
#48228=EDGE_CURVE('',#38613,#38610,#5638,.T.) ;
#48229=EDGE_CURVE('',#38614,#38615,#5639,.T.) ;
#48230=EDGE_CURVE('',#38615,#38616,#5640,.T.) ;
#48231=EDGE_CURVE('',#38616,#38617,#5641,.T.) ;
#48232=EDGE_CURVE('',#38617,#38614,#5642,.T.) ;
#48233=EDGE_CURVE('',#38618,#38619,#5643,.T.) ;
#48234=EDGE_CURVE('',#38619,#38620,#5644,.T.) ;
#48235=EDGE_CURVE('',#38620,#38621,#5645,.T.) ;
#48236=EDGE_CURVE('',#38621,#38618,#5646,.T.) ;
#48237=EDGE_CURVE('',#38622,#38623,#5647,.T.) ;
#48238=EDGE_CURVE('',#38623,#38624,#5648,.T.) ;
#48239=EDGE_CURVE('',#38624,#38625,#5649,.T.) ;
#48240=EDGE_CURVE('',#38625,#38622,#5650,.T.) ;
#48241=EDGE_CURVE('',#38626,#38627,#5651,.T.) ;
#48242=EDGE_CURVE('',#38627,#38628,#5652,.T.) ;
#48243=EDGE_CURVE('',#38628,#38629,#5653,.T.) ;
#48244=EDGE_CURVE('',#38629,#38626,#5654,.T.) ;
#48245=EDGE_CURVE('',#38630,#38631,#5655,.T.) ;
#48246=EDGE_CURVE('',#38631,#38632,#5656,.T.) ;
#48247=EDGE_CURVE('',#38632,#38633,#5657,.T.) ;
#48248=EDGE_CURVE('',#38633,#38630,#5658,.T.) ;
#48249=EDGE_CURVE('',#38634,#38635,#5659,.T.) ;
#48250=EDGE_CURVE('',#38635,#38636,#5660,.T.) ;
#48251=EDGE_CURVE('',#38636,#38637,#5661,.T.) ;
#48252=EDGE_CURVE('',#38637,#38634,#5662,.T.) ;
#48253=EDGE_CURVE('',#38638,#38639,#5663,.T.) ;
#48254=EDGE_CURVE('',#38639,#38640,#5664,.T.) ;
#48255=EDGE_CURVE('',#38640,#38641,#5665,.T.) ;
#48256=EDGE_CURVE('',#38641,#38638,#5666,.T.) ;
#48257=EDGE_CURVE('',#38642,#38643,#5667,.T.) ;
#48258=EDGE_CURVE('',#38643,#38644,#5668,.T.) ;
#48259=EDGE_CURVE('',#38644,#38645,#5669,.T.) ;
#48260=EDGE_CURVE('',#38645,#38642,#5670,.T.) ;
#48261=EDGE_CURVE('',#38646,#38647,#5671,.T.) ;
#48262=EDGE_CURVE('',#38647,#38648,#5672,.T.) ;
#48263=EDGE_CURVE('',#38648,#38649,#5673,.T.) ;
#48264=EDGE_CURVE('',#38649,#38646,#5674,.T.) ;
#48265=EDGE_CURVE('',#38650,#38651,#5675,.T.) ;
#48266=EDGE_CURVE('',#38651,#38652,#5676,.T.) ;
#48267=EDGE_CURVE('',#38652,#38653,#5677,.T.) ;
#48268=EDGE_CURVE('',#38653,#38650,#5678,.T.) ;
#48269=EDGE_CURVE('',#38654,#38655,#5679,.T.) ;
#48270=EDGE_CURVE('',#38655,#38656,#5680,.T.) ;
#48271=EDGE_CURVE('',#38656,#38657,#5681,.T.) ;
#48272=EDGE_CURVE('',#38657,#38654,#5682,.T.) ;
#48273=EDGE_CURVE('',#38658,#38659,#5683,.T.) ;
#48274=EDGE_CURVE('',#38659,#38660,#5684,.T.) ;
#48275=EDGE_CURVE('',#38660,#38661,#5685,.T.) ;
#48276=EDGE_CURVE('',#38661,#38658,#5686,.T.) ;
#48277=EDGE_CURVE('',#38662,#38663,#5687,.T.) ;
#48278=EDGE_CURVE('',#38663,#38664,#5688,.T.) ;
#48279=EDGE_CURVE('',#38664,#38665,#5689,.T.) ;
#48280=EDGE_CURVE('',#38665,#38662,#5690,.T.) ;
#48281=EDGE_CURVE('',#38666,#38667,#5691,.T.) ;
#48282=EDGE_CURVE('',#38667,#38668,#5692,.T.) ;
#48283=EDGE_CURVE('',#38668,#38669,#5693,.T.) ;
#48284=EDGE_CURVE('',#38669,#38666,#5694,.T.) ;
#48285=EDGE_CURVE('',#38670,#38671,#5695,.T.) ;
#48286=EDGE_CURVE('',#38671,#38672,#5696,.T.) ;
#48287=EDGE_CURVE('',#38672,#38673,#5697,.T.) ;
#48288=EDGE_CURVE('',#38673,#38670,#5698,.T.) ;
#48289=EDGE_CURVE('',#38674,#38675,#5699,.T.) ;
#48290=EDGE_CURVE('',#38675,#38676,#5700,.T.) ;
#48291=EDGE_CURVE('',#38676,#38677,#5701,.T.) ;
#48292=EDGE_CURVE('',#38677,#38674,#5702,.T.) ;
#48293=EDGE_CURVE('',#38678,#38679,#5703,.T.) ;
#48294=EDGE_CURVE('',#38679,#38680,#5704,.T.) ;
#48295=EDGE_CURVE('',#38680,#38681,#5705,.T.) ;
#48296=EDGE_CURVE('',#38681,#38678,#5706,.T.) ;
#48297=EDGE_CURVE('',#38682,#38683,#5707,.T.) ;
#48298=EDGE_CURVE('',#38683,#38684,#5708,.T.) ;
#48299=EDGE_CURVE('',#38684,#38685,#5709,.T.) ;
#48300=EDGE_CURVE('',#38685,#38682,#5710,.T.) ;
#48301=EDGE_CURVE('',#38686,#38687,#5711,.T.) ;
#48302=EDGE_CURVE('',#38687,#38688,#5712,.T.) ;
#48303=EDGE_CURVE('',#38688,#38689,#5713,.T.) ;
#48304=EDGE_CURVE('',#38689,#38686,#5714,.T.) ;
#48305=EDGE_CURVE('',#38690,#38691,#5715,.T.) ;
#48306=EDGE_CURVE('',#38691,#38692,#5716,.T.) ;
#48307=EDGE_CURVE('',#38692,#38693,#5717,.T.) ;
#48308=EDGE_CURVE('',#38693,#38690,#5718,.T.) ;
#48309=EDGE_CURVE('',#38694,#38695,#5719,.T.) ;
#48310=EDGE_CURVE('',#38695,#38696,#5720,.T.) ;
#48311=EDGE_CURVE('',#38696,#38697,#5721,.T.) ;
#48312=EDGE_CURVE('',#38697,#38694,#5722,.T.) ;
#48313=EDGE_CURVE('',#38698,#38699,#5723,.T.) ;
#48314=EDGE_CURVE('',#38699,#38700,#5724,.T.) ;
#48315=EDGE_CURVE('',#38700,#38701,#5725,.T.) ;
#48316=EDGE_CURVE('',#38701,#38698,#5726,.T.) ;
#48317=EDGE_CURVE('',#38702,#38703,#5727,.T.) ;
#48318=EDGE_CURVE('',#38703,#38704,#5728,.T.) ;
#48319=EDGE_CURVE('',#38704,#38705,#5729,.T.) ;
#48320=EDGE_CURVE('',#38705,#38702,#5730,.T.) ;
#48321=EDGE_CURVE('',#38706,#38707,#5731,.T.) ;
#48322=EDGE_CURVE('',#38707,#38708,#5732,.T.) ;
#48323=EDGE_CURVE('',#38708,#38709,#5733,.T.) ;
#48324=EDGE_CURVE('',#38709,#38706,#5734,.T.) ;
#48325=EDGE_CURVE('',#38710,#38711,#5735,.T.) ;
#48326=EDGE_CURVE('',#38711,#38712,#5736,.T.) ;
#48327=EDGE_CURVE('',#38712,#38713,#5737,.T.) ;
#48328=EDGE_CURVE('',#38713,#38710,#5738,.T.) ;
#48329=EDGE_CURVE('',#38714,#38715,#5739,.T.) ;
#48330=EDGE_CURVE('',#38715,#38716,#5740,.T.) ;
#48331=EDGE_CURVE('',#38716,#38717,#5741,.T.) ;
#48332=EDGE_CURVE('',#38717,#38714,#5742,.T.) ;
#48333=EDGE_CURVE('',#38718,#38719,#5743,.T.) ;
#48334=EDGE_CURVE('',#38719,#38720,#5744,.T.) ;
#48335=EDGE_CURVE('',#38720,#38721,#5745,.T.) ;
#48336=EDGE_CURVE('',#38721,#38718,#5746,.T.) ;
#48337=EDGE_CURVE('',#38722,#38723,#5747,.T.) ;
#48338=EDGE_CURVE('',#38723,#38724,#5748,.T.) ;
#48339=EDGE_CURVE('',#38724,#38725,#5749,.T.) ;
#48340=EDGE_CURVE('',#38725,#38722,#5750,.T.) ;
#48341=EDGE_CURVE('',#38726,#38727,#5751,.T.) ;
#48342=EDGE_CURVE('',#38727,#38728,#5752,.T.) ;
#48343=EDGE_CURVE('',#38728,#38729,#5753,.T.) ;
#48344=EDGE_CURVE('',#38729,#38726,#5754,.T.) ;
#48345=EDGE_CURVE('',#38730,#38731,#5755,.T.) ;
#48346=EDGE_CURVE('',#38731,#38732,#5756,.T.) ;
#48347=EDGE_CURVE('',#38732,#38733,#5757,.T.) ;
#48348=EDGE_CURVE('',#38733,#38730,#5758,.T.) ;
#48349=EDGE_CURVE('',#38734,#38735,#5759,.T.) ;
#48350=EDGE_CURVE('',#38735,#38736,#5760,.T.) ;
#48351=EDGE_CURVE('',#38736,#38737,#5761,.T.) ;
#48352=EDGE_CURVE('',#38737,#38734,#5762,.T.) ;
#48353=EDGE_CURVE('',#38738,#38739,#5763,.T.) ;
#48354=EDGE_CURVE('',#38739,#38740,#5764,.T.) ;
#48355=EDGE_CURVE('',#38740,#38741,#5765,.T.) ;
#48356=EDGE_CURVE('',#38741,#38738,#5766,.T.) ;
#48357=EDGE_CURVE('',#38664,#38178,#31755,.T.) ;
#48358=EDGE_CURVE('',#38665,#38181,#31756,.T.) ;
#48359=EDGE_CURVE('',#38178,#38183,#31757,.T.) ;
#48360=EDGE_CURVE('',#38182,#38179,#31758,.T.) ;
#48361=EDGE_CURVE('',#38665,#38174,#31759,.T.) ;
#48362=EDGE_CURVE('',#38174,#38181,#31760,.T.) ;
#48363=EDGE_CURVE('',#38179,#38667,#31761,.T.) ;
#48364=EDGE_CURVE('',#38180,#38666,#31762,.T.) ;
#48365=EDGE_CURVE('',#38175,#38180,#31763,.T.) ;
#48366=EDGE_CURVE('',#38662,#38177,#31764,.T.) ;
#48367=EDGE_CURVE('',#38175,#38666,#31765,.T.) ;
#48368=EDGE_CURVE('',#38662,#38170,#31766,.T.) ;
#48369=EDGE_CURVE('',#38170,#38177,#31767,.T.) ;
#48370=EDGE_CURVE('',#38176,#38669,#31768,.T.) ;
#48371=EDGE_CURVE('',#38171,#38176,#31769,.T.) ;
#48372=EDGE_CURVE('',#38173,#38663,#31770,.T.) ;
#48373=EDGE_CURVE('',#38171,#38669,#31771,.T.) ;
#48374=EDGE_CURVE('',#38168,#38173,#31772,.T.) ;
#48375=EDGE_CURVE('',#38172,#38169,#31773,.T.) ;
#48376=EDGE_CURVE('',#38668,#38172,#31774,.T.) ;
#48377=EDGE_CURVE('',#38736,#38194,#31775,.T.) ;
#48378=EDGE_CURVE('',#38737,#38197,#31776,.T.) ;
#48379=EDGE_CURVE('',#38194,#38199,#31777,.T.) ;
#48380=EDGE_CURVE('',#38198,#38195,#31778,.T.) ;
#48381=EDGE_CURVE('',#38737,#38208,#31779,.T.) ;
#48382=EDGE_CURVE('',#38208,#38197,#31780,.T.) ;
#48383=EDGE_CURVE('',#38195,#38739,#31781,.T.) ;
#48384=EDGE_CURVE('',#38196,#38738,#31782,.T.) ;
#48385=EDGE_CURVE('',#38209,#38196,#31783,.T.) ;
#48386=EDGE_CURVE('',#38734,#38207,#31784,.T.) ;
#48387=EDGE_CURVE('',#38209,#38738,#31785,.T.) ;
#48388=EDGE_CURVE('',#38734,#38202,#31786,.T.) ;
#48389=EDGE_CURVE('',#38202,#38207,#31787,.T.) ;
#48390=EDGE_CURVE('',#38206,#38741,#31788,.T.) ;
#48391=EDGE_CURVE('',#38203,#38206,#31789,.T.) ;
#48392=EDGE_CURVE('',#38205,#38735,#31790,.T.) ;
#48393=EDGE_CURVE('',#38203,#38741,#31791,.T.) ;
#48394=EDGE_CURVE('',#38200,#38205,#31792,.T.) ;
#48395=EDGE_CURVE('',#38204,#38201,#31793,.T.) ;
#48396=EDGE_CURVE('',#38740,#38204,#31794,.T.) ;
#48397=EDGE_CURVE('',#38656,#38226,#31795,.T.) ;
#48398=EDGE_CURVE('',#38657,#38229,#31796,.T.) ;
#48399=EDGE_CURVE('',#38226,#38231,#31797,.T.) ;
#48400=EDGE_CURVE('',#38230,#38227,#31798,.T.) ;
#48401=EDGE_CURVE('',#38657,#38222,#31799,.T.) ;
#48402=EDGE_CURVE('',#38222,#38229,#31800,.T.) ;
#48403=EDGE_CURVE('',#38227,#38659,#31801,.T.) ;
#48404=EDGE_CURVE('',#38228,#38658,#31802,.T.) ;
#48405=EDGE_CURVE('',#38223,#38228,#31803,.T.) ;
#48406=EDGE_CURVE('',#38654,#38225,#31804,.T.) ;
#48407=EDGE_CURVE('',#38223,#38658,#31805,.T.) ;
#48408=EDGE_CURVE('',#38654,#38218,#31806,.T.) ;
#48409=EDGE_CURVE('',#38218,#38225,#31807,.T.) ;
#48410=EDGE_CURVE('',#38224,#38661,#31808,.T.) ;
#48411=EDGE_CURVE('',#38219,#38224,#31809,.T.) ;
#48412=EDGE_CURVE('',#38221,#38655,#31810,.T.) ;
#48413=EDGE_CURVE('',#38219,#38661,#31811,.T.) ;
#48414=EDGE_CURVE('',#38216,#38221,#31812,.T.) ;
#48415=EDGE_CURVE('',#38220,#38217,#31813,.T.) ;
#48416=EDGE_CURVE('',#38660,#38220,#31814,.T.) ;
#48417=EDGE_CURVE('',#38728,#38242,#31815,.T.) ;
#48418=EDGE_CURVE('',#38729,#38245,#31816,.T.) ;
#48419=EDGE_CURVE('',#38242,#38247,#31817,.T.) ;
#48420=EDGE_CURVE('',#38246,#38243,#31818,.T.) ;
#48421=EDGE_CURVE('',#38729,#38256,#31819,.T.) ;
#48422=EDGE_CURVE('',#38256,#38245,#31820,.T.) ;
#48423=EDGE_CURVE('',#38243,#38731,#31821,.T.) ;
#48424=EDGE_CURVE('',#38244,#38730,#31822,.T.) ;
#48425=EDGE_CURVE('',#38257,#38244,#31823,.T.) ;
#48426=EDGE_CURVE('',#38726,#38255,#31824,.T.) ;
#48427=EDGE_CURVE('',#38257,#38730,#31825,.T.) ;
#48428=EDGE_CURVE('',#38726,#38250,#31826,.T.) ;
#48429=EDGE_CURVE('',#38250,#38255,#31827,.T.) ;
#48430=EDGE_CURVE('',#38254,#38733,#31828,.T.) ;
#48431=EDGE_CURVE('',#38251,#38254,#31829,.T.) ;
#48432=EDGE_CURVE('',#38253,#38727,#31830,.T.) ;
#48433=EDGE_CURVE('',#38251,#38733,#31831,.T.) ;
#48434=EDGE_CURVE('',#38248,#38253,#31832,.T.) ;
#48435=EDGE_CURVE('',#38252,#38249,#31833,.T.) ;
#48436=EDGE_CURVE('',#38732,#38252,#31834,.T.) ;
#48437=EDGE_CURVE('',#38648,#38274,#31835,.T.) ;
#48438=EDGE_CURVE('',#38649,#38277,#31836,.T.) ;
#48439=EDGE_CURVE('',#38274,#38279,#31837,.T.) ;
#48440=EDGE_CURVE('',#38278,#38275,#31838,.T.) ;
#48441=EDGE_CURVE('',#38649,#38270,#31839,.T.) ;
#48442=EDGE_CURVE('',#38270,#38277,#31840,.T.) ;
#48443=EDGE_CURVE('',#38275,#38651,#31841,.T.) ;
#48444=EDGE_CURVE('',#38276,#38650,#31842,.T.) ;
#48445=EDGE_CURVE('',#38271,#38276,#31843,.T.) ;
#48446=EDGE_CURVE('',#38646,#38273,#31844,.T.) ;
#48447=EDGE_CURVE('',#38271,#38650,#31845,.T.) ;
#48448=EDGE_CURVE('',#38646,#38266,#31846,.T.) ;
#48449=EDGE_CURVE('',#38266,#38273,#31847,.T.) ;
#48450=EDGE_CURVE('',#38272,#38653,#31848,.T.) ;
#48451=EDGE_CURVE('',#38267,#38272,#31849,.T.) ;
#48452=EDGE_CURVE('',#38269,#38647,#31850,.T.) ;
#48453=EDGE_CURVE('',#38267,#38653,#31851,.T.) ;
#48454=EDGE_CURVE('',#38264,#38269,#31852,.T.) ;
#48455=EDGE_CURVE('',#38268,#38265,#31853,.T.) ;
#48456=EDGE_CURVE('',#38652,#38268,#31854,.T.) ;
#48457=EDGE_CURVE('',#38720,#38290,#31855,.T.) ;
#48458=EDGE_CURVE('',#38721,#38293,#31856,.T.) ;
#48459=EDGE_CURVE('',#38290,#38295,#31857,.T.) ;
#48460=EDGE_CURVE('',#38294,#38291,#31858,.T.) ;
#48461=EDGE_CURVE('',#38721,#38304,#31859,.T.) ;
#48462=EDGE_CURVE('',#38304,#38293,#31860,.T.) ;
#48463=EDGE_CURVE('',#38291,#38723,#31861,.T.) ;
#48464=EDGE_CURVE('',#38292,#38722,#31862,.T.) ;
#48465=EDGE_CURVE('',#38305,#38292,#31863,.T.) ;
#48466=EDGE_CURVE('',#38718,#38303,#31864,.T.) ;
#48467=EDGE_CURVE('',#38305,#38722,#31865,.T.) ;
#48468=EDGE_CURVE('',#38718,#38298,#31866,.T.) ;
#48469=EDGE_CURVE('',#38298,#38303,#31867,.T.) ;
#48470=EDGE_CURVE('',#38302,#38725,#31868,.T.) ;
#48471=EDGE_CURVE('',#38299,#38302,#31869,.T.) ;
#48472=EDGE_CURVE('',#38301,#38719,#31870,.T.) ;
#48473=EDGE_CURVE('',#38299,#38725,#31871,.T.) ;
#48474=EDGE_CURVE('',#38296,#38301,#31872,.T.) ;
#48475=EDGE_CURVE('',#38300,#38297,#31873,.T.) ;
#48476=EDGE_CURVE('',#38724,#38300,#31874,.T.) ;
#48477=EDGE_CURVE('',#38640,#38322,#31875,.T.) ;
#48478=EDGE_CURVE('',#38641,#38325,#31876,.T.) ;
#48479=EDGE_CURVE('',#38322,#38327,#31877,.T.) ;
#48480=EDGE_CURVE('',#38326,#38323,#31878,.T.) ;
#48481=EDGE_CURVE('',#38641,#38318,#31879,.T.) ;
#48482=EDGE_CURVE('',#38318,#38325,#31880,.T.) ;
#48483=EDGE_CURVE('',#38323,#38643,#31881,.T.) ;
#48484=EDGE_CURVE('',#38324,#38642,#31882,.T.) ;
#48485=EDGE_CURVE('',#38319,#38324,#31883,.T.) ;
#48486=EDGE_CURVE('',#38638,#38321,#31884,.T.) ;
#48487=EDGE_CURVE('',#38319,#38642,#31885,.T.) ;
#48488=EDGE_CURVE('',#38638,#38314,#31886,.T.) ;
#48489=EDGE_CURVE('',#38314,#38321,#31887,.T.) ;
#48490=EDGE_CURVE('',#38320,#38645,#31888,.T.) ;
#48491=EDGE_CURVE('',#38315,#38320,#31889,.T.) ;
#48492=EDGE_CURVE('',#38317,#38639,#31890,.T.) ;
#48493=EDGE_CURVE('',#38315,#38645,#31891,.T.) ;
#48494=EDGE_CURVE('',#38312,#38317,#31892,.T.) ;
#48495=EDGE_CURVE('',#38316,#38313,#31893,.T.) ;
#48496=EDGE_CURVE('',#38644,#38316,#31894,.T.) ;
#48497=EDGE_CURVE('',#38712,#38338,#31895,.T.) ;
#48498=EDGE_CURVE('',#38713,#38341,#31896,.T.) ;
#48499=EDGE_CURVE('',#38338,#38343,#31897,.T.) ;
#48500=EDGE_CURVE('',#38342,#38339,#31898,.T.) ;
#48501=EDGE_CURVE('',#38713,#38352,#31899,.T.) ;
#48502=EDGE_CURVE('',#38352,#38341,#31900,.T.) ;
#48503=EDGE_CURVE('',#38339,#38715,#31901,.T.) ;
#48504=EDGE_CURVE('',#38340,#38714,#31902,.T.) ;
#48505=EDGE_CURVE('',#38353,#38340,#31903,.T.) ;
#48506=EDGE_CURVE('',#38710,#38351,#31904,.T.) ;
#48507=EDGE_CURVE('',#38353,#38714,#31905,.T.) ;
#48508=EDGE_CURVE('',#38710,#38346,#31906,.T.) ;
#48509=EDGE_CURVE('',#38346,#38351,#31907,.T.) ;
#48510=EDGE_CURVE('',#38350,#38717,#31908,.T.) ;
#48511=EDGE_CURVE('',#38347,#38350,#31909,.T.) ;
#48512=EDGE_CURVE('',#38349,#38711,#31910,.T.) ;
#48513=EDGE_CURVE('',#38347,#38717,#31911,.T.) ;
#48514=EDGE_CURVE('',#38344,#38349,#31912,.T.) ;
#48515=EDGE_CURVE('',#38348,#38345,#31913,.T.) ;
#48516=EDGE_CURVE('',#38716,#38348,#31914,.T.) ;
#48517=EDGE_CURVE('',#38632,#38370,#31915,.T.) ;
#48518=EDGE_CURVE('',#38633,#38373,#31916,.T.) ;
#48519=EDGE_CURVE('',#38370,#38375,#31917,.T.) ;
#48520=EDGE_CURVE('',#38374,#38371,#31918,.T.) ;
#48521=EDGE_CURVE('',#38633,#38366,#31919,.T.) ;
#48522=EDGE_CURVE('',#38366,#38373,#31920,.T.) ;
#48523=EDGE_CURVE('',#38371,#38635,#31921,.T.) ;
#48524=EDGE_CURVE('',#38372,#38634,#31922,.T.) ;
#48525=EDGE_CURVE('',#38367,#38372,#31923,.T.) ;
#48526=EDGE_CURVE('',#38630,#38369,#31924,.T.) ;
#48527=EDGE_CURVE('',#38367,#38634,#31925,.T.) ;
#48528=EDGE_CURVE('',#38630,#38362,#31926,.T.) ;
#48529=EDGE_CURVE('',#38362,#38369,#31927,.T.) ;
#48530=EDGE_CURVE('',#38368,#38637,#31928,.T.) ;
#48531=EDGE_CURVE('',#38363,#38368,#31929,.T.) ;
#48532=EDGE_CURVE('',#38365,#38631,#31930,.T.) ;
#48533=EDGE_CURVE('',#38363,#38637,#31931,.T.) ;
#48534=EDGE_CURVE('',#38360,#38365,#31932,.T.) ;
#48535=EDGE_CURVE('',#38364,#38361,#31933,.T.) ;
#48536=EDGE_CURVE('',#38636,#38364,#31934,.T.) ;
#48537=EDGE_CURVE('',#38704,#38386,#31935,.T.) ;
#48538=EDGE_CURVE('',#38705,#38389,#31936,.T.) ;
#48539=EDGE_CURVE('',#38386,#38391,#31937,.T.) ;
#48540=EDGE_CURVE('',#38390,#38387,#31938,.T.) ;
#48541=EDGE_CURVE('',#38705,#38400,#31939,.T.) ;
#48542=EDGE_CURVE('',#38400,#38389,#31940,.T.) ;
#48543=EDGE_CURVE('',#38387,#38707,#31941,.T.) ;
#48544=EDGE_CURVE('',#38388,#38706,#31942,.T.) ;
#48545=EDGE_CURVE('',#38401,#38388,#31943,.T.) ;
#48546=EDGE_CURVE('',#38702,#38399,#31944,.T.) ;
#48547=EDGE_CURVE('',#38401,#38706,#31945,.T.) ;
#48548=EDGE_CURVE('',#38702,#38394,#31946,.T.) ;
#48549=EDGE_CURVE('',#38394,#38399,#31947,.T.) ;
#48550=EDGE_CURVE('',#38398,#38709,#31948,.T.) ;
#48551=EDGE_CURVE('',#38395,#38398,#31949,.T.) ;
#48552=EDGE_CURVE('',#38397,#38703,#31950,.T.) ;
#48553=EDGE_CURVE('',#38395,#38709,#31951,.T.) ;
#48554=EDGE_CURVE('',#38392,#38397,#31952,.T.) ;
#48555=EDGE_CURVE('',#38396,#38393,#31953,.T.) ;
#48556=EDGE_CURVE('',#38708,#38396,#31954,.T.) ;
#48557=EDGE_CURVE('',#38624,#38418,#31955,.T.) ;
#48558=EDGE_CURVE('',#38625,#38421,#31956,.T.) ;
#48559=EDGE_CURVE('',#38418,#38423,#31957,.T.) ;
#48560=EDGE_CURVE('',#38422,#38419,#31958,.T.) ;
#48561=EDGE_CURVE('',#38625,#38414,#31959,.T.) ;
#48562=EDGE_CURVE('',#38414,#38421,#31960,.T.) ;
#48563=EDGE_CURVE('',#38419,#38627,#31961,.T.) ;
#48564=EDGE_CURVE('',#38420,#38626,#31962,.T.) ;
#48565=EDGE_CURVE('',#38415,#38420,#31963,.T.) ;
#48566=EDGE_CURVE('',#38622,#38417,#31964,.T.) ;
#48567=EDGE_CURVE('',#38415,#38626,#31965,.T.) ;
#48568=EDGE_CURVE('',#38622,#38410,#31966,.T.) ;
#48569=EDGE_CURVE('',#38410,#38417,#31967,.T.) ;
#48570=EDGE_CURVE('',#38416,#38629,#31968,.T.) ;
#48571=EDGE_CURVE('',#38411,#38416,#31969,.T.) ;
#48572=EDGE_CURVE('',#38413,#38623,#31970,.T.) ;
#48573=EDGE_CURVE('',#38411,#38629,#31971,.T.) ;
#48574=EDGE_CURVE('',#38408,#38413,#31972,.T.) ;
#48575=EDGE_CURVE('',#38412,#38409,#31973,.T.) ;
#48576=EDGE_CURVE('',#38628,#38412,#31974,.T.) ;
#48577=EDGE_CURVE('',#38696,#38434,#31975,.T.) ;
#48578=EDGE_CURVE('',#38697,#38437,#31976,.T.) ;
#48579=EDGE_CURVE('',#38434,#38439,#31977,.T.) ;
#48580=EDGE_CURVE('',#38438,#38435,#31978,.T.) ;
#48581=EDGE_CURVE('',#38697,#38448,#31979,.T.) ;
#48582=EDGE_CURVE('',#38448,#38437,#31980,.T.) ;
#48583=EDGE_CURVE('',#38435,#38699,#31981,.T.) ;
#48584=EDGE_CURVE('',#38436,#38698,#31982,.T.) ;
#48585=EDGE_CURVE('',#38449,#38436,#31983,.T.) ;
#48586=EDGE_CURVE('',#38694,#38447,#31984,.T.) ;
#48587=EDGE_CURVE('',#38449,#38698,#31985,.T.) ;
#48588=EDGE_CURVE('',#38694,#38442,#31986,.T.) ;
#48589=EDGE_CURVE('',#38442,#38447,#31987,.T.) ;
#48590=EDGE_CURVE('',#38446,#38701,#31988,.T.) ;
#48591=EDGE_CURVE('',#38443,#38446,#31989,.T.) ;
#48592=EDGE_CURVE('',#38445,#38695,#31990,.T.) ;
#48593=EDGE_CURVE('',#38443,#38701,#31991,.T.) ;
#48594=EDGE_CURVE('',#38440,#38445,#31992,.T.) ;
#48595=EDGE_CURVE('',#38444,#38441,#31993,.T.) ;
#48596=EDGE_CURVE('',#38700,#38444,#31994,.T.) ;
#48597=EDGE_CURVE('',#38616,#38466,#31995,.T.) ;
#48598=EDGE_CURVE('',#38617,#38469,#31996,.T.) ;
#48599=EDGE_CURVE('',#38466,#38471,#31997,.T.) ;
#48600=EDGE_CURVE('',#38470,#38467,#31998,.T.) ;
#48601=EDGE_CURVE('',#38617,#38462,#31999,.T.) ;
#48602=EDGE_CURVE('',#38462,#38469,#32000,.T.) ;
#48603=EDGE_CURVE('',#38467,#38619,#32001,.T.) ;
#48604=EDGE_CURVE('',#38468,#38618,#32002,.T.) ;
#48605=EDGE_CURVE('',#38463,#38468,#32003,.T.) ;
#48606=EDGE_CURVE('',#38614,#38465,#32004,.T.) ;
#48607=EDGE_CURVE('',#38463,#38618,#32005,.T.) ;
#48608=EDGE_CURVE('',#38614,#38458,#32006,.T.) ;
#48609=EDGE_CURVE('',#38458,#38465,#32007,.T.) ;
#48610=EDGE_CURVE('',#38464,#38621,#32008,.T.) ;
#48611=EDGE_CURVE('',#38459,#38464,#32009,.T.) ;
#48612=EDGE_CURVE('',#38461,#38615,#32010,.T.) ;
#48613=EDGE_CURVE('',#38459,#38621,#32011,.T.) ;
#48614=EDGE_CURVE('',#38456,#38461,#32012,.T.) ;
#48615=EDGE_CURVE('',#38460,#38457,#32013,.T.) ;
#48616=EDGE_CURVE('',#38620,#38460,#32014,.T.) ;
#48617=EDGE_CURVE('',#38688,#38482,#32015,.T.) ;
#48618=EDGE_CURVE('',#38689,#38485,#32016,.T.) ;
#48619=EDGE_CURVE('',#38482,#38487,#32017,.T.) ;
#48620=EDGE_CURVE('',#38486,#38483,#32018,.T.) ;
#48621=EDGE_CURVE('',#38689,#38496,#32019,.T.) ;
#48622=EDGE_CURVE('',#38496,#38485,#32020,.T.) ;
#48623=EDGE_CURVE('',#38483,#38691,#32021,.T.) ;
#48624=EDGE_CURVE('',#38484,#38690,#32022,.T.) ;
#48625=EDGE_CURVE('',#38497,#38484,#32023,.T.) ;
#48626=EDGE_CURVE('',#38686,#38495,#32024,.T.) ;
#48627=EDGE_CURVE('',#38497,#38690,#32025,.T.) ;
#48628=EDGE_CURVE('',#38686,#38490,#32026,.T.) ;
#48629=EDGE_CURVE('',#38490,#38495,#32027,.T.) ;
#48630=EDGE_CURVE('',#38494,#38693,#32028,.T.) ;
#48631=EDGE_CURVE('',#38491,#38494,#32029,.T.) ;
#48632=EDGE_CURVE('',#38493,#38687,#32030,.T.) ;
#48633=EDGE_CURVE('',#38491,#38693,#32031,.T.) ;
#48634=EDGE_CURVE('',#38488,#38493,#32032,.T.) ;
#48635=EDGE_CURVE('',#38492,#38489,#32033,.T.) ;
#48636=EDGE_CURVE('',#38692,#38492,#32034,.T.) ;
#48637=EDGE_CURVE('',#38608,#38514,#32035,.T.) ;
#48638=EDGE_CURVE('',#38609,#38517,#32036,.T.) ;
#48639=EDGE_CURVE('',#38514,#38519,#32037,.T.) ;
#48640=EDGE_CURVE('',#38518,#38515,#32038,.T.) ;
#48641=EDGE_CURVE('',#38609,#38510,#32039,.T.) ;
#48642=EDGE_CURVE('',#38510,#38517,#32040,.T.) ;
#48643=EDGE_CURVE('',#38515,#38611,#32041,.T.) ;
#48644=EDGE_CURVE('',#38516,#38610,#32042,.T.) ;
#48645=EDGE_CURVE('',#38511,#38516,#32043,.T.) ;
#48646=EDGE_CURVE('',#38606,#38513,#32044,.T.) ;
#48647=EDGE_CURVE('',#38511,#38610,#32045,.T.) ;
#48648=EDGE_CURVE('',#38606,#38506,#32046,.T.) ;
#48649=EDGE_CURVE('',#38506,#38513,#32047,.T.) ;
#48650=EDGE_CURVE('',#38512,#38613,#32048,.T.) ;
#48651=EDGE_CURVE('',#38507,#38512,#32049,.T.) ;
#48652=EDGE_CURVE('',#38509,#38607,#32050,.T.) ;
#48653=EDGE_CURVE('',#38507,#38613,#32051,.T.) ;
#48654=EDGE_CURVE('',#38504,#38509,#32052,.T.) ;
#48655=EDGE_CURVE('',#38508,#38505,#32053,.T.) ;
#48656=EDGE_CURVE('',#38612,#38508,#32054,.T.) ;
#48657=EDGE_CURVE('',#38680,#38530,#32055,.T.) ;
#48658=EDGE_CURVE('',#38681,#38533,#32056,.T.) ;
#48659=EDGE_CURVE('',#38530,#38535,#32057,.T.) ;
#48660=EDGE_CURVE('',#38534,#38531,#32058,.T.) ;
#48661=EDGE_CURVE('',#38681,#38544,#32059,.T.) ;
#48662=EDGE_CURVE('',#38544,#38533,#32060,.T.) ;
#48663=EDGE_CURVE('',#38531,#38683,#32061,.T.) ;
#48664=EDGE_CURVE('',#38532,#38682,#32062,.T.) ;
#48665=EDGE_CURVE('',#38545,#38532,#32063,.T.) ;
#48666=EDGE_CURVE('',#38678,#38543,#32064,.T.) ;
#48667=EDGE_CURVE('',#38545,#38682,#32065,.T.) ;
#48668=EDGE_CURVE('',#38678,#38538,#32066,.T.) ;
#48669=EDGE_CURVE('',#38538,#38543,#32067,.T.) ;
#48670=EDGE_CURVE('',#38542,#38685,#32068,.T.) ;
#48671=EDGE_CURVE('',#38539,#38542,#32069,.T.) ;
#48672=EDGE_CURVE('',#38541,#38679,#32070,.T.) ;
#48673=EDGE_CURVE('',#38539,#38685,#32071,.T.) ;
#48674=EDGE_CURVE('',#38536,#38541,#32072,.T.) ;
#48675=EDGE_CURVE('',#38540,#38537,#32073,.T.) ;
#48676=EDGE_CURVE('',#38684,#38540,#32074,.T.) ;
#48677=EDGE_CURVE('',#38600,#38562,#32075,.T.) ;
#48678=EDGE_CURVE('',#38601,#38565,#32076,.T.) ;
#48679=EDGE_CURVE('',#38562,#38567,#32077,.T.) ;
#48680=EDGE_CURVE('',#38566,#38563,#32078,.T.) ;
#48681=EDGE_CURVE('',#38601,#38558,#32079,.T.) ;
#48682=EDGE_CURVE('',#38558,#38565,#32080,.T.) ;
#48683=EDGE_CURVE('',#38563,#38603,#32081,.T.) ;
#48684=EDGE_CURVE('',#38564,#38602,#32082,.T.) ;
#48685=EDGE_CURVE('',#38559,#38564,#32083,.T.) ;
#48686=EDGE_CURVE('',#38598,#38561,#32084,.T.) ;
#48687=EDGE_CURVE('',#38559,#38602,#32085,.T.) ;
#48688=EDGE_CURVE('',#38598,#38554,#32086,.T.) ;
#48689=EDGE_CURVE('',#38554,#38561,#32087,.T.) ;
#48690=EDGE_CURVE('',#38560,#38605,#32088,.T.) ;
#48691=EDGE_CURVE('',#38555,#38560,#32089,.T.) ;
#48692=EDGE_CURVE('',#38557,#38599,#32090,.T.) ;
#48693=EDGE_CURVE('',#38555,#38605,#32091,.T.) ;
#48694=EDGE_CURVE('',#38552,#38557,#32092,.T.) ;
#48695=EDGE_CURVE('',#38556,#38553,#32093,.T.) ;
#48696=EDGE_CURVE('',#38604,#38556,#32094,.T.) ;
#48697=EDGE_CURVE('',#38672,#38578,#32095,.T.) ;
#48698=EDGE_CURVE('',#38673,#38581,#32096,.T.) ;
#48699=EDGE_CURVE('',#38578,#38583,#32097,.T.) ;
#48700=EDGE_CURVE('',#38582,#38579,#32098,.T.) ;
#48701=EDGE_CURVE('',#38673,#38592,#32099,.T.) ;
#48702=EDGE_CURVE('',#38592,#38581,#32100,.T.) ;
#48703=EDGE_CURVE('',#38579,#38675,#32101,.T.) ;
#48704=EDGE_CURVE('',#38580,#38674,#32102,.T.) ;
#48705=EDGE_CURVE('',#38593,#38580,#32103,.T.) ;
#48706=EDGE_CURVE('',#38670,#38591,#32104,.T.) ;
#48707=EDGE_CURVE('',#38593,#38674,#32105,.T.) ;
#48708=EDGE_CURVE('',#38670,#38586,#32106,.T.) ;
#48709=EDGE_CURVE('',#38586,#38591,#32107,.T.) ;
#48710=EDGE_CURVE('',#38590,#38677,#32108,.T.) ;
#48711=EDGE_CURVE('',#38587,#38590,#32109,.T.) ;
#48712=EDGE_CURVE('',#38589,#38671,#32110,.T.) ;
#48713=EDGE_CURVE('',#38587,#38677,#32111,.T.) ;
#48714=EDGE_CURVE('',#38584,#38589,#32112,.T.) ;
#48715=EDGE_CURVE('',#38588,#38585,#32113,.T.) ;
#48716=EDGE_CURVE('',#38676,#38588,#32114,.T.) ;
#48717=EDGE_CURVE('',#38192,#38184,#32115,.T.) ;
#48718=EDGE_CURVE('',#38193,#38183,#32116,.T.) ;
#48719=EDGE_CURVE('',#38193,#38664,#32117,.T.) ;
#48720=EDGE_CURVE('',#38190,#38663,#32118,.T.) ;
#48721=EDGE_CURVE('',#38190,#38168,#32119,.T.) ;
#48722=EDGE_CURVE('',#38191,#38167,#32120,.T.) ;
#48723=EDGE_CURVE('',#38188,#38166,#32121,.T.) ;
#48724=EDGE_CURVE('',#38189,#38169,#32122,.T.) ;
#48725=EDGE_CURVE('',#38189,#38668,#32123,.T.) ;
#48726=EDGE_CURVE('',#38186,#38667,#32124,.T.) ;
#48727=EDGE_CURVE('',#38186,#38182,#32125,.T.) ;
#48728=EDGE_CURVE('',#38187,#38185,#32126,.T.) ;
#48729=EDGE_CURVE('',#38212,#38199,#32127,.T.) ;
#48730=EDGE_CURVE('',#38212,#38736,#32128,.T.) ;
#48731=EDGE_CURVE('',#38213,#38735,#32129,.T.) ;
#48732=EDGE_CURVE('',#38213,#38200,#32130,.T.) ;
#48733=EDGE_CURVE('',#38198,#38211,#32131,.T.) ;
#48734=EDGE_CURVE('',#38739,#38211,#32132,.T.) ;
#48735=EDGE_CURVE('',#38740,#38210,#32133,.T.) ;
#48736=EDGE_CURVE('',#38210,#38201,#32134,.T.) ;
#48737=EDGE_CURVE('',#38240,#38232,#32135,.T.) ;
#48738=EDGE_CURVE('',#38241,#38231,#32136,.T.) ;
#48739=EDGE_CURVE('',#38241,#38656,#32137,.T.) ;
#48740=EDGE_CURVE('',#38238,#38655,#32138,.T.) ;
#48741=EDGE_CURVE('',#38238,#38216,#32139,.T.) ;
#48742=EDGE_CURVE('',#38239,#38215,#32140,.T.) ;
#48743=EDGE_CURVE('',#38236,#38214,#32141,.T.) ;
#48744=EDGE_CURVE('',#38237,#38217,#32142,.T.) ;
#48745=EDGE_CURVE('',#38237,#38660,#32143,.T.) ;
#48746=EDGE_CURVE('',#38234,#38659,#32144,.T.) ;
#48747=EDGE_CURVE('',#38234,#38230,#32145,.T.) ;
#48748=EDGE_CURVE('',#38235,#38233,#32146,.T.) ;
#48749=EDGE_CURVE('',#38260,#38247,#32147,.T.) ;
#48750=EDGE_CURVE('',#38260,#38728,#32148,.T.) ;
#48751=EDGE_CURVE('',#38261,#38727,#32149,.T.) ;
#48752=EDGE_CURVE('',#38261,#38248,#32150,.T.) ;
#48753=EDGE_CURVE('',#38246,#38259,#32151,.T.) ;
#48754=EDGE_CURVE('',#38731,#38259,#32152,.T.) ;
#48755=EDGE_CURVE('',#38732,#38258,#32153,.T.) ;
#48756=EDGE_CURVE('',#38258,#38249,#32154,.T.) ;
#48757=EDGE_CURVE('',#38288,#38280,#32155,.T.) ;
#48758=EDGE_CURVE('',#38289,#38279,#32156,.T.) ;
#48759=EDGE_CURVE('',#38289,#38648,#32157,.T.) ;
#48760=EDGE_CURVE('',#38286,#38647,#32158,.T.) ;
#48761=EDGE_CURVE('',#38286,#38264,#32159,.T.) ;
#48762=EDGE_CURVE('',#38287,#38263,#32160,.T.) ;
#48763=EDGE_CURVE('',#38284,#38262,#32161,.T.) ;
#48764=EDGE_CURVE('',#38285,#38265,#32162,.T.) ;
#48765=EDGE_CURVE('',#38285,#38652,#32163,.T.) ;
#48766=EDGE_CURVE('',#38282,#38651,#32164,.T.) ;
#48767=EDGE_CURVE('',#38282,#38278,#32165,.T.) ;
#48768=EDGE_CURVE('',#38283,#38281,#32166,.T.) ;
#48769=EDGE_CURVE('',#38308,#38295,#32167,.T.) ;
#48770=EDGE_CURVE('',#38308,#38720,#32168,.T.) ;
#48771=EDGE_CURVE('',#38309,#38719,#32169,.T.) ;
#48772=EDGE_CURVE('',#38309,#38296,#32170,.T.) ;
#48773=EDGE_CURVE('',#38294,#38307,#32171,.T.) ;
#48774=EDGE_CURVE('',#38723,#38307,#32172,.T.) ;
#48775=EDGE_CURVE('',#38724,#38306,#32173,.T.) ;
#48776=EDGE_CURVE('',#38306,#38297,#32174,.T.) ;
#48777=EDGE_CURVE('',#38336,#38328,#32175,.T.) ;
#48778=EDGE_CURVE('',#38337,#38327,#32176,.T.) ;
#48779=EDGE_CURVE('',#38337,#38640,#32177,.T.) ;
#48780=EDGE_CURVE('',#38334,#38639,#32178,.T.) ;
#48781=EDGE_CURVE('',#38334,#38312,#32179,.T.) ;
#48782=EDGE_CURVE('',#38335,#38311,#32180,.T.) ;
#48783=EDGE_CURVE('',#38332,#38310,#32181,.T.) ;
#48784=EDGE_CURVE('',#38333,#38313,#32182,.T.) ;
#48785=EDGE_CURVE('',#38333,#38644,#32183,.T.) ;
#48786=EDGE_CURVE('',#38330,#38643,#32184,.T.) ;
#48787=EDGE_CURVE('',#38330,#38326,#32185,.T.) ;
#48788=EDGE_CURVE('',#38331,#38329,#32186,.T.) ;
#48789=EDGE_CURVE('',#38356,#38343,#32187,.T.) ;
#48790=EDGE_CURVE('',#38356,#38712,#32188,.T.) ;
#48791=EDGE_CURVE('',#38357,#38711,#32189,.T.) ;
#48792=EDGE_CURVE('',#38357,#38344,#32190,.T.) ;
#48793=EDGE_CURVE('',#38342,#38355,#32191,.T.) ;
#48794=EDGE_CURVE('',#38715,#38355,#32192,.T.) ;
#48795=EDGE_CURVE('',#38716,#38354,#32193,.T.) ;
#48796=EDGE_CURVE('',#38354,#38345,#32194,.T.) ;
#48797=EDGE_CURVE('',#38384,#38376,#32195,.T.) ;
#48798=EDGE_CURVE('',#38385,#38375,#32196,.T.) ;
#48799=EDGE_CURVE('',#38385,#38632,#32197,.T.) ;
#48800=EDGE_CURVE('',#38382,#38631,#32198,.T.) ;
#48801=EDGE_CURVE('',#38382,#38360,#32199,.T.) ;
#48802=EDGE_CURVE('',#38383,#38359,#32200,.T.) ;
#48803=EDGE_CURVE('',#38380,#38358,#32201,.T.) ;
#48804=EDGE_CURVE('',#38381,#38361,#32202,.T.) ;
#48805=EDGE_CURVE('',#38381,#38636,#32203,.T.) ;
#48806=EDGE_CURVE('',#38378,#38635,#32204,.T.) ;
#48807=EDGE_CURVE('',#38378,#38374,#32205,.T.) ;
#48808=EDGE_CURVE('',#38379,#38377,#32206,.T.) ;
#48809=EDGE_CURVE('',#38404,#38391,#32207,.T.) ;
#48810=EDGE_CURVE('',#38404,#38704,#32208,.T.) ;
#48811=EDGE_CURVE('',#38405,#38703,#32209,.T.) ;
#48812=EDGE_CURVE('',#38405,#38392,#32210,.T.) ;
#48813=EDGE_CURVE('',#38390,#38403,#32211,.T.) ;
#48814=EDGE_CURVE('',#38707,#38403,#32212,.T.) ;
#48815=EDGE_CURVE('',#38708,#38402,#32213,.T.) ;
#48816=EDGE_CURVE('',#38402,#38393,#32214,.T.) ;
#48817=EDGE_CURVE('',#38432,#38424,#32215,.T.) ;
#48818=EDGE_CURVE('',#38433,#38423,#32216,.T.) ;
#48819=EDGE_CURVE('',#38433,#38624,#32217,.T.) ;
#48820=EDGE_CURVE('',#38430,#38623,#32218,.T.) ;
#48821=EDGE_CURVE('',#38430,#38408,#32219,.T.) ;
#48822=EDGE_CURVE('',#38431,#38407,#32220,.T.) ;
#48823=EDGE_CURVE('',#38428,#38406,#32221,.T.) ;
#48824=EDGE_CURVE('',#38429,#38409,#32222,.T.) ;
#48825=EDGE_CURVE('',#38429,#38628,#32223,.T.) ;
#48826=EDGE_CURVE('',#38426,#38627,#32224,.T.) ;
#48827=EDGE_CURVE('',#38426,#38422,#32225,.T.) ;
#48828=EDGE_CURVE('',#38427,#38425,#32226,.T.) ;
#48829=EDGE_CURVE('',#38452,#38439,#32227,.T.) ;
#48830=EDGE_CURVE('',#38452,#38696,#32228,.T.) ;
#48831=EDGE_CURVE('',#38453,#38695,#32229,.T.) ;
#48832=EDGE_CURVE('',#38453,#38440,#32230,.T.) ;
#48833=EDGE_CURVE('',#38438,#38451,#32231,.T.) ;
#48834=EDGE_CURVE('',#38699,#38451,#32232,.T.) ;
#48835=EDGE_CURVE('',#38700,#38450,#32233,.T.) ;
#48836=EDGE_CURVE('',#38450,#38441,#32234,.T.) ;
#48837=EDGE_CURVE('',#38480,#38472,#32235,.T.) ;
#48838=EDGE_CURVE('',#38481,#38471,#32236,.T.) ;
#48839=EDGE_CURVE('',#38481,#38616,#32237,.T.) ;
#48840=EDGE_CURVE('',#38478,#38615,#32238,.T.) ;
#48841=EDGE_CURVE('',#38478,#38456,#32239,.T.) ;
#48842=EDGE_CURVE('',#38479,#38455,#32240,.T.) ;
#48843=EDGE_CURVE('',#38476,#38454,#32241,.T.) ;
#48844=EDGE_CURVE('',#38477,#38457,#32242,.T.) ;
#48845=EDGE_CURVE('',#38477,#38620,#32243,.T.) ;
#48846=EDGE_CURVE('',#38474,#38619,#32244,.T.) ;
#48847=EDGE_CURVE('',#38474,#38470,#32245,.T.) ;
#48848=EDGE_CURVE('',#38475,#38473,#32246,.T.) ;
#48849=EDGE_CURVE('',#38500,#38487,#32247,.T.) ;
#48850=EDGE_CURVE('',#38500,#38688,#32248,.T.) ;
#48851=EDGE_CURVE('',#38501,#38687,#32249,.T.) ;
#48852=EDGE_CURVE('',#38501,#38488,#32250,.T.) ;
#48853=EDGE_CURVE('',#38486,#38499,#32251,.T.) ;
#48854=EDGE_CURVE('',#38691,#38499,#32252,.T.) ;
#48855=EDGE_CURVE('',#38692,#38498,#32253,.T.) ;
#48856=EDGE_CURVE('',#38498,#38489,#32254,.T.) ;
#48857=EDGE_CURVE('',#38528,#38520,#32255,.T.) ;
#48858=EDGE_CURVE('',#38529,#38519,#32256,.T.) ;
#48859=EDGE_CURVE('',#38529,#38608,#32257,.T.) ;
#48860=EDGE_CURVE('',#38526,#38607,#32258,.T.) ;
#48861=EDGE_CURVE('',#38526,#38504,#32259,.T.) ;
#48862=EDGE_CURVE('',#38527,#38503,#32260,.T.) ;
#48863=EDGE_CURVE('',#38524,#38502,#32261,.T.) ;
#48864=EDGE_CURVE('',#38525,#38505,#32262,.T.) ;
#48865=EDGE_CURVE('',#38525,#38612,#32263,.T.) ;
#48866=EDGE_CURVE('',#38522,#38611,#32264,.T.) ;
#48867=EDGE_CURVE('',#38522,#38518,#32265,.T.) ;
#48868=EDGE_CURVE('',#38523,#38521,#32266,.T.) ;
#48869=EDGE_CURVE('',#38548,#38535,#32267,.T.) ;
#48870=EDGE_CURVE('',#38548,#38680,#32268,.T.) ;
#48871=EDGE_CURVE('',#38549,#38679,#32269,.T.) ;
#48872=EDGE_CURVE('',#38549,#38536,#32270,.T.) ;
#48873=EDGE_CURVE('',#38534,#38547,#32271,.T.) ;
#48874=EDGE_CURVE('',#38683,#38547,#32272,.T.) ;
#48875=EDGE_CURVE('',#38684,#38546,#32273,.T.) ;
#48876=EDGE_CURVE('',#38546,#38537,#32274,.T.) ;
#48877=EDGE_CURVE('',#38576,#38568,#32275,.T.) ;
#48878=EDGE_CURVE('',#38577,#38567,#32276,.T.) ;
#48879=EDGE_CURVE('',#38577,#38600,#32277,.T.) ;
#48880=EDGE_CURVE('',#38574,#38599,#32278,.T.) ;
#48881=EDGE_CURVE('',#38574,#38552,#32279,.T.) ;
#48882=EDGE_CURVE('',#38575,#38551,#32280,.T.) ;
#48883=EDGE_CURVE('',#38572,#38550,#32281,.T.) ;
#48884=EDGE_CURVE('',#38573,#38553,#32282,.T.) ;
#48885=EDGE_CURVE('',#38573,#38604,#32283,.T.) ;
#48886=EDGE_CURVE('',#38570,#38603,#32284,.T.) ;
#48887=EDGE_CURVE('',#38570,#38566,#32285,.T.) ;
#48888=EDGE_CURVE('',#38571,#38569,#32286,.T.) ;
#48889=EDGE_CURVE('',#38596,#38583,#32287,.T.) ;
#48890=EDGE_CURVE('',#38596,#38672,#32288,.T.) ;
#48891=EDGE_CURVE('',#38597,#38671,#32289,.T.) ;
#48892=EDGE_CURVE('',#38597,#38584,#32290,.T.) ;
#48893=EDGE_CURVE('',#38582,#38595,#32291,.T.) ;
#48894=EDGE_CURVE('',#38675,#38595,#32292,.T.) ;
#48895=EDGE_CURVE('',#38676,#38594,#32293,.T.) ;
#48896=EDGE_CURVE('',#38594,#38585,#32294,.T.) ;
#59139=ORIENTED_EDGE('',*,*,#44147,.F.) ;
#59140=ORIENTED_EDGE('',*,*,#44148,.T.) ;
#59141=ORIENTED_EDGE('',*,*,#44149,.F.) ;
#59142=ORIENTED_EDGE('',*,*,#44150,.F.) ;
#59143=ORIENTED_EDGE('',*,*,#44148,.F.) ;
#59144=ORIENTED_EDGE('',*,*,#44151,.F.) ;
#59145=ORIENTED_EDGE('',*,*,#44152,.T.) ;
#59146=ORIENTED_EDGE('',*,*,#44153,.F.) ;
#59147=ORIENTED_EDGE('',*,*,#44152,.F.) ;
#59148=ORIENTED_EDGE('',*,*,#44154,.F.) ;
#59149=ORIENTED_EDGE('',*,*,#44155,.F.) ;
#59150=ORIENTED_EDGE('',*,*,#44156,.T.) ;
#59151=ORIENTED_EDGE('',*,*,#44157,.F.) ;
#59152=ORIENTED_EDGE('',*,*,#44158,.T.) ;
#59153=ORIENTED_EDGE('',*,*,#44159,.F.) ;
#59154=ORIENTED_EDGE('',*,*,#44160,.F.) ;
#59155=ORIENTED_EDGE('',*,*,#44161,.F.) ;
#59156=ORIENTED_EDGE('',*,*,#44162,.F.) ;
#59157=ORIENTED_EDGE('',*,*,#44163,.T.) ;
#59158=ORIENTED_EDGE('',*,*,#44164,.F.) ;
#59159=ORIENTED_EDGE('',*,*,#44165,.T.) ;
#59160=ORIENTED_EDGE('',*,*,#44166,.F.) ;
#59161=ORIENTED_EDGE('',*,*,#44167,.F.) ;
#59162=ORIENTED_EDGE('',*,*,#44165,.F.) ;
#59163=ORIENTED_EDGE('',*,*,#44168,.F.) ;
#59164=ORIENTED_EDGE('',*,*,#44169,.T.) ;
#59165=ORIENTED_EDGE('',*,*,#44170,.F.) ;
#59166=ORIENTED_EDGE('',*,*,#44169,.F.) ;
#59167=ORIENTED_EDGE('',*,*,#44171,.F.) ;
#59168=ORIENTED_EDGE('',*,*,#44172,.F.) ;
#59169=ORIENTED_EDGE('',*,*,#44173,.T.) ;
#59170=ORIENTED_EDGE('',*,*,#44174,.F.) ;
#59171=ORIENTED_EDGE('',*,*,#44175,.T.) ;
#59172=ORIENTED_EDGE('',*,*,#44176,.F.) ;
#59173=ORIENTED_EDGE('',*,*,#44177,.F.) ;
#59174=ORIENTED_EDGE('',*,*,#44178,.F.) ;
#59175=ORIENTED_EDGE('',*,*,#44179,.F.) ;
#59176=ORIENTED_EDGE('',*,*,#44180,.T.) ;
#59177=ORIENTED_EDGE('',*,*,#44181,.F.) ;
#59178=ORIENTED_EDGE('',*,*,#44182,.T.) ;
#59179=ORIENTED_EDGE('',*,*,#44183,.F.) ;
#59180=ORIENTED_EDGE('',*,*,#44184,.F.) ;
#59181=ORIENTED_EDGE('',*,*,#44182,.F.) ;
#59182=ORIENTED_EDGE('',*,*,#44185,.F.) ;
#59183=ORIENTED_EDGE('',*,*,#44186,.T.) ;
#59184=ORIENTED_EDGE('',*,*,#44187,.F.) ;
#59185=ORIENTED_EDGE('',*,*,#44186,.F.) ;
#59186=ORIENTED_EDGE('',*,*,#44188,.F.) ;
#59187=ORIENTED_EDGE('',*,*,#44189,.F.) ;
#59188=ORIENTED_EDGE('',*,*,#44190,.T.) ;
#59189=ORIENTED_EDGE('',*,*,#44191,.F.) ;
#59190=ORIENTED_EDGE('',*,*,#44192,.T.) ;
#59191=ORIENTED_EDGE('',*,*,#44193,.F.) ;
#59192=ORIENTED_EDGE('',*,*,#44194,.F.) ;
#59193=ORIENTED_EDGE('',*,*,#44195,.F.) ;
#59194=ORIENTED_EDGE('',*,*,#44196,.F.) ;
#59195=ORIENTED_EDGE('',*,*,#44197,.T.) ;
#59196=ORIENTED_EDGE('',*,*,#44198,.F.) ;
#59197=ORIENTED_EDGE('',*,*,#44199,.T.) ;
#59198=ORIENTED_EDGE('',*,*,#44200,.F.) ;
#59199=ORIENTED_EDGE('',*,*,#44201,.F.) ;
#59200=ORIENTED_EDGE('',*,*,#44199,.F.) ;
#59201=ORIENTED_EDGE('',*,*,#44202,.F.) ;
#59202=ORIENTED_EDGE('',*,*,#44203,.T.) ;
#59203=ORIENTED_EDGE('',*,*,#44204,.F.) ;
#59204=ORIENTED_EDGE('',*,*,#44203,.F.) ;
#59205=ORIENTED_EDGE('',*,*,#44205,.F.) ;
#59206=ORIENTED_EDGE('',*,*,#44206,.F.) ;
#59207=ORIENTED_EDGE('',*,*,#44207,.T.) ;
#59208=ORIENTED_EDGE('',*,*,#44208,.F.) ;
#59209=ORIENTED_EDGE('',*,*,#44209,.T.) ;
#59210=ORIENTED_EDGE('',*,*,#44210,.F.) ;
#59211=ORIENTED_EDGE('',*,*,#44211,.F.) ;
#59212=ORIENTED_EDGE('',*,*,#44212,.F.) ;
#59213=ORIENTED_EDGE('',*,*,#44213,.F.) ;
#59214=ORIENTED_EDGE('',*,*,#44214,.T.) ;
#59215=ORIENTED_EDGE('',*,*,#44215,.F.) ;
#59216=ORIENTED_EDGE('',*,*,#44216,.T.) ;
#59217=ORIENTED_EDGE('',*,*,#44217,.F.) ;
#59218=ORIENTED_EDGE('',*,*,#44218,.F.) ;
#59219=ORIENTED_EDGE('',*,*,#44216,.F.) ;
#59220=ORIENTED_EDGE('',*,*,#44219,.F.) ;
#59221=ORIENTED_EDGE('',*,*,#44220,.T.) ;
#59222=ORIENTED_EDGE('',*,*,#44221,.F.) ;
#59223=ORIENTED_EDGE('',*,*,#44220,.F.) ;
#59224=ORIENTED_EDGE('',*,*,#44222,.F.) ;
#59225=ORIENTED_EDGE('',*,*,#44223,.F.) ;
#59226=ORIENTED_EDGE('',*,*,#44224,.T.) ;
#59227=ORIENTED_EDGE('',*,*,#44225,.F.) ;
#59228=ORIENTED_EDGE('',*,*,#44226,.T.) ;
#59229=ORIENTED_EDGE('',*,*,#44227,.F.) ;
#59230=ORIENTED_EDGE('',*,*,#44228,.F.) ;
#59231=ORIENTED_EDGE('',*,*,#44229,.F.) ;
#59232=ORIENTED_EDGE('',*,*,#44230,.F.) ;
#59233=ORIENTED_EDGE('',*,*,#44231,.T.) ;
#59234=ORIENTED_EDGE('',*,*,#44232,.F.) ;
#59235=ORIENTED_EDGE('',*,*,#44233,.T.) ;
#59236=ORIENTED_EDGE('',*,*,#44234,.F.) ;
#59237=ORIENTED_EDGE('',*,*,#44235,.F.) ;
#59238=ORIENTED_EDGE('',*,*,#44233,.F.) ;
#59239=ORIENTED_EDGE('',*,*,#44236,.F.) ;
#59240=ORIENTED_EDGE('',*,*,#44237,.T.) ;
#59241=ORIENTED_EDGE('',*,*,#44238,.F.) ;
#59242=ORIENTED_EDGE('',*,*,#44237,.F.) ;
#59243=ORIENTED_EDGE('',*,*,#44239,.F.) ;
#59244=ORIENTED_EDGE('',*,*,#44240,.F.) ;
#59245=ORIENTED_EDGE('',*,*,#44241,.T.) ;
#59246=ORIENTED_EDGE('',*,*,#44242,.F.) ;
#59247=ORIENTED_EDGE('',*,*,#44243,.T.) ;
#59248=ORIENTED_EDGE('',*,*,#44244,.F.) ;
#59249=ORIENTED_EDGE('',*,*,#44245,.F.) ;
#59250=ORIENTED_EDGE('',*,*,#44246,.F.) ;
#59251=ORIENTED_EDGE('',*,*,#44247,.F.) ;
#59252=ORIENTED_EDGE('',*,*,#44248,.T.) ;
#59253=ORIENTED_EDGE('',*,*,#44249,.F.) ;
#59254=ORIENTED_EDGE('',*,*,#44250,.T.) ;
#59255=ORIENTED_EDGE('',*,*,#44251,.F.) ;
#59256=ORIENTED_EDGE('',*,*,#44252,.F.) ;
#59257=ORIENTED_EDGE('',*,*,#44250,.F.) ;
#59258=ORIENTED_EDGE('',*,*,#44253,.F.) ;
#59259=ORIENTED_EDGE('',*,*,#44254,.T.) ;
#59260=ORIENTED_EDGE('',*,*,#44255,.F.) ;
#59261=ORIENTED_EDGE('',*,*,#44254,.F.) ;
#59262=ORIENTED_EDGE('',*,*,#44256,.F.) ;
#59263=ORIENTED_EDGE('',*,*,#44257,.F.) ;
#59264=ORIENTED_EDGE('',*,*,#44258,.T.) ;
#59265=ORIENTED_EDGE('',*,*,#44259,.F.) ;
#59266=ORIENTED_EDGE('',*,*,#44260,.T.) ;
#59267=ORIENTED_EDGE('',*,*,#44261,.F.) ;
#59268=ORIENTED_EDGE('',*,*,#44262,.F.) ;
#59269=ORIENTED_EDGE('',*,*,#44263,.F.) ;
#59270=ORIENTED_EDGE('',*,*,#44264,.F.) ;
#59271=ORIENTED_EDGE('',*,*,#44265,.T.) ;
#59272=ORIENTED_EDGE('',*,*,#44266,.F.) ;
#59273=ORIENTED_EDGE('',*,*,#44267,.T.) ;
#59274=ORIENTED_EDGE('',*,*,#44268,.F.) ;
#59275=ORIENTED_EDGE('',*,*,#44269,.F.) ;
#59276=ORIENTED_EDGE('',*,*,#44267,.F.) ;
#59277=ORIENTED_EDGE('',*,*,#44270,.F.) ;
#59278=ORIENTED_EDGE('',*,*,#44271,.T.) ;
#59279=ORIENTED_EDGE('',*,*,#44272,.F.) ;
#59280=ORIENTED_EDGE('',*,*,#44271,.F.) ;
#59281=ORIENTED_EDGE('',*,*,#44273,.F.) ;
#59282=ORIENTED_EDGE('',*,*,#44274,.F.) ;
#59283=ORIENTED_EDGE('',*,*,#44275,.T.) ;
#59284=ORIENTED_EDGE('',*,*,#44276,.F.) ;
#59285=ORIENTED_EDGE('',*,*,#44277,.T.) ;
#59286=ORIENTED_EDGE('',*,*,#44278,.F.) ;
#59287=ORIENTED_EDGE('',*,*,#44279,.F.) ;
#59288=ORIENTED_EDGE('',*,*,#44280,.F.) ;
#59289=ORIENTED_EDGE('',*,*,#44281,.F.) ;
#59290=ORIENTED_EDGE('',*,*,#44282,.T.) ;
#59291=ORIENTED_EDGE('',*,*,#44283,.F.) ;
#59292=ORIENTED_EDGE('',*,*,#44284,.T.) ;
#59293=ORIENTED_EDGE('',*,*,#44285,.F.) ;
#59294=ORIENTED_EDGE('',*,*,#44286,.F.) ;
#59295=ORIENTED_EDGE('',*,*,#44284,.F.) ;
#59296=ORIENTED_EDGE('',*,*,#44287,.F.) ;
#59297=ORIENTED_EDGE('',*,*,#44288,.F.) ;
#59298=ORIENTED_EDGE('',*,*,#44289,.F.) ;
#59299=ORIENTED_EDGE('',*,*,#44290,.T.) ;
#59300=ORIENTED_EDGE('',*,*,#44291,.F.) ;
#59301=ORIENTED_EDGE('',*,*,#44292,.F.) ;
#59302=ORIENTED_EDGE('',*,*,#44293,.F.) ;
#59303=ORIENTED_EDGE('',*,*,#44294,.T.) ;
#59304=ORIENTED_EDGE('',*,*,#44295,.F.) ;
#59305=ORIENTED_EDGE('',*,*,#44296,.F.) ;
#59306=ORIENTED_EDGE('',*,*,#44297,.F.) ;
#59307=ORIENTED_EDGE('',*,*,#44298,.T.) ;
#59308=ORIENTED_EDGE('',*,*,#44299,.F.) ;
#59309=ORIENTED_EDGE('',*,*,#44300,.F.) ;
#59310=ORIENTED_EDGE('',*,*,#44301,.F.) ;
#59311=ORIENTED_EDGE('',*,*,#44302,.T.) ;
#59312=ORIENTED_EDGE('',*,*,#44303,.F.) ;
#59313=ORIENTED_EDGE('',*,*,#44304,.F.) ;
#59314=ORIENTED_EDGE('',*,*,#44305,.F.) ;
#59315=ORIENTED_EDGE('',*,*,#44306,.T.) ;
#59316=ORIENTED_EDGE('',*,*,#44307,.F.) ;
#59317=ORIENTED_EDGE('',*,*,#44308,.F.) ;
#59318=ORIENTED_EDGE('',*,*,#44309,.F.) ;
#59319=ORIENTED_EDGE('',*,*,#44310,.T.) ;
#59320=ORIENTED_EDGE('',*,*,#44311,.F.) ;
#59321=ORIENTED_EDGE('',*,*,#44312,.F.) ;
#59322=ORIENTED_EDGE('',*,*,#44313,.F.) ;
#59323=ORIENTED_EDGE('',*,*,#44314,.T.) ;
#59324=ORIENTED_EDGE('',*,*,#44315,.F.) ;
#59325=ORIENTED_EDGE('',*,*,#44316,.F.) ;
#59326=ORIENTED_EDGE('',*,*,#44317,.F.) ;
#59327=ORIENTED_EDGE('',*,*,#44318,.T.) ;
#59328=ORIENTED_EDGE('',*,*,#44319,.F.) ;
#59329=ORIENTED_EDGE('',*,*,#44320,.F.) ;
#59330=ORIENTED_EDGE('',*,*,#44321,.F.) ;
#59331=ORIENTED_EDGE('',*,*,#44322,.T.) ;
#59332=ORIENTED_EDGE('',*,*,#44323,.F.) ;
#59333=ORIENTED_EDGE('',*,*,#44324,.T.) ;
#59334=ORIENTED_EDGE('',*,*,#44325,.F.) ;
#59335=ORIENTED_EDGE('',*,*,#44324,.F.) ;
#59336=ORIENTED_EDGE('',*,*,#44326,.F.) ;
#59337=ORIENTED_EDGE('',*,*,#44327,.F.) ;
#59338=ORIENTED_EDGE('',*,*,#44328,.T.) ;
#59339=ORIENTED_EDGE('',*,*,#44329,.F.) ;
#59340=ORIENTED_EDGE('',*,*,#44330,.T.) ;
#59341=ORIENTED_EDGE('',*,*,#44331,.F.) ;
#59342=ORIENTED_EDGE('',*,*,#44332,.F.) ;
#59343=ORIENTED_EDGE('',*,*,#44333,.F.) ;
#59344=ORIENTED_EDGE('',*,*,#44334,.F.) ;
#59345=ORIENTED_EDGE('',*,*,#44335,.T.) ;
#59346=ORIENTED_EDGE('',*,*,#44153,.T.) ;
#59347=ORIENTED_EDGE('',*,*,#44336,.T.) ;
#59348=ORIENTED_EDGE('',*,*,#44149,.T.) ;
#59349=ORIENTED_EDGE('',*,*,#44150,.T.) ;
#59350=ORIENTED_EDGE('',*,*,#44336,.F.) ;
#59351=ORIENTED_EDGE('',*,*,#44170,.T.) ;
#59352=ORIENTED_EDGE('',*,*,#44337,.T.) ;
#59353=ORIENTED_EDGE('',*,*,#44166,.T.) ;
#59354=ORIENTED_EDGE('',*,*,#44167,.T.) ;
#59355=ORIENTED_EDGE('',*,*,#44337,.F.) ;
#59356=ORIENTED_EDGE('',*,*,#44187,.T.) ;
#59357=ORIENTED_EDGE('',*,*,#44338,.T.) ;
#59358=ORIENTED_EDGE('',*,*,#44183,.T.) ;
#59359=ORIENTED_EDGE('',*,*,#44184,.T.) ;
#59360=ORIENTED_EDGE('',*,*,#44338,.F.) ;
#59361=ORIENTED_EDGE('',*,*,#44204,.T.) ;
#59362=ORIENTED_EDGE('',*,*,#44339,.T.) ;
#59363=ORIENTED_EDGE('',*,*,#44200,.T.) ;
#59364=ORIENTED_EDGE('',*,*,#44201,.T.) ;
#59365=ORIENTED_EDGE('',*,*,#44339,.F.) ;
#59366=ORIENTED_EDGE('',*,*,#44221,.T.) ;
#59367=ORIENTED_EDGE('',*,*,#44340,.T.) ;
#59368=ORIENTED_EDGE('',*,*,#44217,.T.) ;
#59369=ORIENTED_EDGE('',*,*,#44218,.T.) ;
#59370=ORIENTED_EDGE('',*,*,#44340,.F.) ;
#59371=ORIENTED_EDGE('',*,*,#44238,.T.) ;
#59372=ORIENTED_EDGE('',*,*,#44341,.T.) ;
#59373=ORIENTED_EDGE('',*,*,#44234,.T.) ;
#59374=ORIENTED_EDGE('',*,*,#44235,.T.) ;
#59375=ORIENTED_EDGE('',*,*,#44341,.F.) ;
#59376=ORIENTED_EDGE('',*,*,#44255,.T.) ;
#59377=ORIENTED_EDGE('',*,*,#44342,.T.) ;
#59378=ORIENTED_EDGE('',*,*,#44251,.T.) ;
#59379=ORIENTED_EDGE('',*,*,#44252,.T.) ;
#59380=ORIENTED_EDGE('',*,*,#44342,.F.) ;
#59381=ORIENTED_EDGE('',*,*,#44272,.T.) ;
#59382=ORIENTED_EDGE('',*,*,#44343,.T.) ;
#59383=ORIENTED_EDGE('',*,*,#44268,.T.) ;
#59384=ORIENTED_EDGE('',*,*,#44269,.T.) ;
#59385=ORIENTED_EDGE('',*,*,#44343,.F.) ;
#59386=ORIENTED_EDGE('',*,*,#44325,.T.) ;
#59387=ORIENTED_EDGE('',*,*,#44344,.T.) ;
#59388=ORIENTED_EDGE('',*,*,#44285,.T.) ;
#59389=ORIENTED_EDGE('',*,*,#44286,.T.) ;
#59390=ORIENTED_EDGE('',*,*,#44344,.F.) ;
#59391=ORIENTED_EDGE('',*,*,#44345,.T.) ;
#59392=ORIENTED_EDGE('',*,*,#44346,.T.) ;
#59393=ORIENTED_EDGE('',*,*,#44289,.T.) ;
#59394=ORIENTED_EDGE('',*,*,#44347,.F.) ;
#59395=ORIENTED_EDGE('',*,*,#44348,.T.) ;
#59396=ORIENTED_EDGE('',*,*,#44349,.T.) ;
#59397=ORIENTED_EDGE('',*,*,#44293,.T.) ;
#59398=ORIENTED_EDGE('',*,*,#44350,.F.) ;
#59399=ORIENTED_EDGE('',*,*,#44351,.T.) ;
#59400=ORIENTED_EDGE('',*,*,#44352,.T.) ;
#59401=ORIENTED_EDGE('',*,*,#44297,.T.) ;
#59402=ORIENTED_EDGE('',*,*,#44353,.F.) ;
#59403=ORIENTED_EDGE('',*,*,#44354,.T.) ;
#59404=ORIENTED_EDGE('',*,*,#44355,.T.) ;
#59405=ORIENTED_EDGE('',*,*,#44301,.T.) ;
#59406=ORIENTED_EDGE('',*,*,#44356,.F.) ;
#59407=ORIENTED_EDGE('',*,*,#44357,.T.) ;
#59408=ORIENTED_EDGE('',*,*,#44358,.T.) ;
#59409=ORIENTED_EDGE('',*,*,#44305,.T.) ;
#59410=ORIENTED_EDGE('',*,*,#44359,.F.) ;
#59411=ORIENTED_EDGE('',*,*,#44360,.T.) ;
#59412=ORIENTED_EDGE('',*,*,#44361,.T.) ;
#59413=ORIENTED_EDGE('',*,*,#44309,.T.) ;
#59414=ORIENTED_EDGE('',*,*,#44362,.F.) ;
#59415=ORIENTED_EDGE('',*,*,#44363,.T.) ;
#59416=ORIENTED_EDGE('',*,*,#44364,.T.) ;
#59417=ORIENTED_EDGE('',*,*,#44313,.T.) ;
#59418=ORIENTED_EDGE('',*,*,#44365,.F.) ;
#59419=ORIENTED_EDGE('',*,*,#44366,.T.) ;
#59420=ORIENTED_EDGE('',*,*,#44367,.T.) ;
#59421=ORIENTED_EDGE('',*,*,#44317,.T.) ;
#59422=ORIENTED_EDGE('',*,*,#44368,.F.) ;
#59423=ORIENTED_EDGE('',*,*,#44369,.T.) ;
#59424=ORIENTED_EDGE('',*,*,#44370,.T.) ;
#59425=ORIENTED_EDGE('',*,*,#44321,.T.) ;
#59426=ORIENTED_EDGE('',*,*,#44371,.F.) ;
#59427=ORIENTED_EDGE('',*,*,#44372,.F.) ;
#59428=ORIENTED_EDGE('',*,*,#44373,.T.) ;
#59429=ORIENTED_EDGE('',*,*,#44374,.F.) ;
#59430=ORIENTED_EDGE('',*,*,#44375,.F.) ;
#59431=ORIENTED_EDGE('',*,*,#44373,.F.) ;
#59432=ORIENTED_EDGE('',*,*,#44376,.F.) ;
#59433=ORIENTED_EDGE('',*,*,#44377,.F.) ;
#59434=ORIENTED_EDGE('',*,*,#44378,.F.) ;
#59435=ORIENTED_EDGE('',*,*,#44379,.T.) ;
#59436=ORIENTED_EDGE('',*,*,#44380,.F.) ;
#59437=ORIENTED_EDGE('',*,*,#44381,.T.) ;
#59438=ORIENTED_EDGE('',*,*,#44382,.F.) ;
#59439=ORIENTED_EDGE('',*,*,#44381,.F.) ;
#59440=ORIENTED_EDGE('',*,*,#44383,.F.) ;
#59441=ORIENTED_EDGE('',*,*,#44384,.F.) ;
#59442=ORIENTED_EDGE('',*,*,#44385,.T.) ;
#59443=ORIENTED_EDGE('',*,*,#44386,.F.) ;
#59444=ORIENTED_EDGE('',*,*,#44387,.T.) ;
#59445=ORIENTED_EDGE('',*,*,#44388,.F.) ;
#59446=ORIENTED_EDGE('',*,*,#44389,.F.) ;
#59447=ORIENTED_EDGE('',*,*,#44390,.F.) ;
#59448=ORIENTED_EDGE('',*,*,#44391,.F.) ;
#59449=ORIENTED_EDGE('',*,*,#44392,.T.) ;
#59450=ORIENTED_EDGE('',*,*,#44382,.T.) ;
#59451=ORIENTED_EDGE('',*,*,#44393,.T.) ;
#59452=ORIENTED_EDGE('',*,*,#44374,.T.) ;
#59453=ORIENTED_EDGE('',*,*,#44375,.T.) ;
#59454=ORIENTED_EDGE('',*,*,#44393,.F.) ;
#59455=ORIENTED_EDGE('',*,*,#44394,.T.) ;
#59456=ORIENTED_EDGE('',*,*,#44395,.T.) ;
#59457=ORIENTED_EDGE('',*,*,#44378,.T.) ;
#59458=ORIENTED_EDGE('',*,*,#44396,.F.) ;
#59459=ORIENTED_EDGE('',*,*,#44397,.T.) ;
#59460=ORIENTED_EDGE('',*,*,#44398,.T.) ;
#59461=ORIENTED_EDGE('',*,*,#44399,.T.) ;
#59462=ORIENTED_EDGE('',*,*,#44400,.T.) ;
#59463=ORIENTED_EDGE('',*,*,#44161,.T.) ;
#59464=ORIENTED_EDGE('',*,*,#44401,.F.) ;
#59465=ORIENTED_EDGE('',*,*,#44402,.T.) ;
#59466=ORIENTED_EDGE('',*,*,#44403,.T.) ;
#59467=ORIENTED_EDGE('',*,*,#44404,.T.) ;
#59468=ORIENTED_EDGE('',*,*,#44405,.T.) ;
#59469=ORIENTED_EDGE('',*,*,#44406,.T.) ;
#59470=ORIENTED_EDGE('',*,*,#44407,.F.) ;
#59471=ORIENTED_EDGE('',*,*,#44408,.T.) ;
#59472=ORIENTED_EDGE('',*,*,#44409,.T.) ;
#59473=ORIENTED_EDGE('',*,*,#44410,.T.) ;
#59474=ORIENTED_EDGE('',*,*,#44411,.T.) ;
#59475=ORIENTED_EDGE('',*,*,#44178,.T.) ;
#59476=ORIENTED_EDGE('',*,*,#44412,.F.) ;
#59477=ORIENTED_EDGE('',*,*,#44413,.T.) ;
#59478=ORIENTED_EDGE('',*,*,#44414,.T.) ;
#59479=ORIENTED_EDGE('',*,*,#44415,.T.) ;
#59480=ORIENTED_EDGE('',*,*,#44416,.T.) ;
#59481=ORIENTED_EDGE('',*,*,#44417,.T.) ;
#59482=ORIENTED_EDGE('',*,*,#44418,.F.) ;
#59483=ORIENTED_EDGE('',*,*,#44419,.T.) ;
#59484=ORIENTED_EDGE('',*,*,#44420,.T.) ;
#59485=ORIENTED_EDGE('',*,*,#44421,.T.) ;
#59486=ORIENTED_EDGE('',*,*,#44422,.T.) ;
#59487=ORIENTED_EDGE('',*,*,#44195,.T.) ;
#59488=ORIENTED_EDGE('',*,*,#44423,.F.) ;
#59489=ORIENTED_EDGE('',*,*,#44424,.T.) ;
#59490=ORIENTED_EDGE('',*,*,#44425,.T.) ;
#59491=ORIENTED_EDGE('',*,*,#44426,.T.) ;
#59492=ORIENTED_EDGE('',*,*,#44427,.T.) ;
#59493=ORIENTED_EDGE('',*,*,#44428,.T.) ;
#59494=ORIENTED_EDGE('',*,*,#44429,.F.) ;
#59495=ORIENTED_EDGE('',*,*,#44430,.T.) ;
#59496=ORIENTED_EDGE('',*,*,#44431,.T.) ;
#59497=ORIENTED_EDGE('',*,*,#44432,.T.) ;
#59498=ORIENTED_EDGE('',*,*,#44433,.T.) ;
#59499=ORIENTED_EDGE('',*,*,#44212,.T.) ;
#59500=ORIENTED_EDGE('',*,*,#44434,.F.) ;
#59501=ORIENTED_EDGE('',*,*,#44435,.T.) ;
#59502=ORIENTED_EDGE('',*,*,#44436,.T.) ;
#59503=ORIENTED_EDGE('',*,*,#44437,.T.) ;
#59504=ORIENTED_EDGE('',*,*,#44438,.T.) ;
#59505=ORIENTED_EDGE('',*,*,#44439,.T.) ;
#59506=ORIENTED_EDGE('',*,*,#44440,.F.) ;
#59507=ORIENTED_EDGE('',*,*,#44441,.T.) ;
#59508=ORIENTED_EDGE('',*,*,#44442,.T.) ;
#59509=ORIENTED_EDGE('',*,*,#44443,.T.) ;
#59510=ORIENTED_EDGE('',*,*,#44444,.T.) ;
#59511=ORIENTED_EDGE('',*,*,#44229,.T.) ;
#59512=ORIENTED_EDGE('',*,*,#44445,.F.) ;
#59513=ORIENTED_EDGE('',*,*,#44446,.T.) ;
#59514=ORIENTED_EDGE('',*,*,#44447,.T.) ;
#59515=ORIENTED_EDGE('',*,*,#44448,.T.) ;
#59516=ORIENTED_EDGE('',*,*,#44449,.T.) ;
#59517=ORIENTED_EDGE('',*,*,#44450,.T.) ;
#59518=ORIENTED_EDGE('',*,*,#44451,.F.) ;
#59519=ORIENTED_EDGE('',*,*,#44452,.T.) ;
#59520=ORIENTED_EDGE('',*,*,#44453,.T.) ;
#59521=ORIENTED_EDGE('',*,*,#44454,.T.) ;
#59522=ORIENTED_EDGE('',*,*,#44455,.T.) ;
#59523=ORIENTED_EDGE('',*,*,#44246,.T.) ;
#59524=ORIENTED_EDGE('',*,*,#44456,.F.) ;
#59525=ORIENTED_EDGE('',*,*,#44457,.T.) ;
#59526=ORIENTED_EDGE('',*,*,#44458,.T.) ;
#59527=ORIENTED_EDGE('',*,*,#44459,.T.) ;
#59528=ORIENTED_EDGE('',*,*,#44460,.T.) ;
#59529=ORIENTED_EDGE('',*,*,#44461,.T.) ;
#59530=ORIENTED_EDGE('',*,*,#44462,.F.) ;
#59531=ORIENTED_EDGE('',*,*,#44463,.T.) ;
#59532=ORIENTED_EDGE('',*,*,#44464,.T.) ;
#59533=ORIENTED_EDGE('',*,*,#44465,.T.) ;
#59534=ORIENTED_EDGE('',*,*,#44466,.T.) ;
#59535=ORIENTED_EDGE('',*,*,#44263,.T.) ;
#59536=ORIENTED_EDGE('',*,*,#44467,.F.) ;
#59537=ORIENTED_EDGE('',*,*,#44468,.T.) ;
#59538=ORIENTED_EDGE('',*,*,#44469,.T.) ;
#59539=ORIENTED_EDGE('',*,*,#44470,.T.) ;
#59540=ORIENTED_EDGE('',*,*,#44471,.T.) ;
#59541=ORIENTED_EDGE('',*,*,#44472,.T.) ;
#59542=ORIENTED_EDGE('',*,*,#44473,.F.) ;
#59543=ORIENTED_EDGE('',*,*,#44474,.T.) ;
#59544=ORIENTED_EDGE('',*,*,#44475,.T.) ;
#59545=ORIENTED_EDGE('',*,*,#44476,.T.) ;
#59546=ORIENTED_EDGE('',*,*,#44477,.T.) ;
#59547=ORIENTED_EDGE('',*,*,#44280,.T.) ;
#59548=ORIENTED_EDGE('',*,*,#44478,.F.) ;
#59549=ORIENTED_EDGE('',*,*,#44479,.T.) ;
#59550=ORIENTED_EDGE('',*,*,#44480,.T.) ;
#59551=ORIENTED_EDGE('',*,*,#44481,.T.) ;
#59552=ORIENTED_EDGE('',*,*,#44482,.T.) ;
#59553=ORIENTED_EDGE('',*,*,#44483,.T.) ;
#59554=ORIENTED_EDGE('',*,*,#44484,.F.) ;
#59555=ORIENTED_EDGE('',*,*,#44485,.T.) ;
#59556=ORIENTED_EDGE('',*,*,#44486,.T.) ;
#59557=ORIENTED_EDGE('',*,*,#44487,.T.) ;
#59558=ORIENTED_EDGE('',*,*,#44488,.T.) ;
#59559=ORIENTED_EDGE('',*,*,#44333,.T.) ;
#59560=ORIENTED_EDGE('',*,*,#44489,.F.) ;
#59561=ORIENTED_EDGE('',*,*,#44490,.T.) ;
#59562=ORIENTED_EDGE('',*,*,#44491,.T.) ;
#59563=ORIENTED_EDGE('',*,*,#44492,.T.) ;
#59564=ORIENTED_EDGE('',*,*,#44493,.T.) ;
#59565=ORIENTED_EDGE('',*,*,#44494,.T.) ;
#59566=ORIENTED_EDGE('',*,*,#44495,.F.) ;
#59567=ORIENTED_EDGE('',*,*,#44496,.F.) ;
#59568=ORIENTED_EDGE('',*,*,#44497,.T.) ;
#59569=ORIENTED_EDGE('',*,*,#44498,.T.) ;
#59570=ORIENTED_EDGE('',*,*,#44499,.T.) ;
#59571=ORIENTED_EDGE('',*,*,#44500,.T.) ;
#59572=ORIENTED_EDGE('',*,*,#44501,.F.) ;
#59573=ORIENTED_EDGE('',*,*,#44502,.T.) ;
#59574=ORIENTED_EDGE('',*,*,#44503,.T.) ;
#59575=ORIENTED_EDGE('',*,*,#44504,.T.) ;
#59576=ORIENTED_EDGE('',*,*,#44505,.T.) ;
#59577=ORIENTED_EDGE('',*,*,#44506,.F.) ;
#59578=ORIENTED_EDGE('',*,*,#44507,.T.) ;
#59579=ORIENTED_EDGE('',*,*,#44508,.T.) ;
#59580=ORIENTED_EDGE('',*,*,#44509,.T.) ;
#59581=ORIENTED_EDGE('',*,*,#44510,.T.) ;
#59582=ORIENTED_EDGE('',*,*,#44511,.F.) ;
#59583=ORIENTED_EDGE('',*,*,#44512,.T.) ;
#59584=ORIENTED_EDGE('',*,*,#44513,.T.) ;
#59585=ORIENTED_EDGE('',*,*,#44514,.T.) ;
#59586=ORIENTED_EDGE('',*,*,#44515,.T.) ;
#59587=ORIENTED_EDGE('',*,*,#44516,.F.) ;
#59588=ORIENTED_EDGE('',*,*,#44517,.T.) ;
#59589=ORIENTED_EDGE('',*,*,#44518,.T.) ;
#59590=ORIENTED_EDGE('',*,*,#44519,.T.) ;
#59591=ORIENTED_EDGE('',*,*,#44520,.T.) ;
#59592=ORIENTED_EDGE('',*,*,#44521,.F.) ;
#59593=ORIENTED_EDGE('',*,*,#44522,.T.) ;
#59594=ORIENTED_EDGE('',*,*,#44523,.T.) ;
#59595=ORIENTED_EDGE('',*,*,#44524,.T.) ;
#59596=ORIENTED_EDGE('',*,*,#44525,.T.) ;
#59597=ORIENTED_EDGE('',*,*,#44526,.F.) ;
#59598=ORIENTED_EDGE('',*,*,#44527,.T.) ;
#59599=ORIENTED_EDGE('',*,*,#44528,.T.) ;
#59600=ORIENTED_EDGE('',*,*,#44529,.T.) ;
#59601=ORIENTED_EDGE('',*,*,#44530,.T.) ;
#59602=ORIENTED_EDGE('',*,*,#44531,.F.) ;
#59603=ORIENTED_EDGE('',*,*,#44532,.T.) ;
#59604=ORIENTED_EDGE('',*,*,#44533,.T.) ;
#59605=ORIENTED_EDGE('',*,*,#44534,.T.) ;
#59606=ORIENTED_EDGE('',*,*,#44535,.T.) ;
#59607=ORIENTED_EDGE('',*,*,#44536,.F.) ;
#59608=ORIENTED_EDGE('',*,*,#44537,.T.) ;
#59609=ORIENTED_EDGE('',*,*,#44538,.T.) ;
#59610=ORIENTED_EDGE('',*,*,#44539,.T.) ;
#59611=ORIENTED_EDGE('',*,*,#44540,.T.) ;
#59612=ORIENTED_EDGE('',*,*,#44541,.F.) ;
#59613=ORIENTED_EDGE('',*,*,#44542,.T.) ;
#59614=ORIENTED_EDGE('',*,*,#44543,.T.) ;
#59615=ORIENTED_EDGE('',*,*,#44544,.T.) ;
#59616=ORIENTED_EDGE('',*,*,#44545,.T.) ;
#59617=ORIENTED_EDGE('',*,*,#44546,.F.) ;
#59618=ORIENTED_EDGE('',*,*,#44547,.T.) ;
#59619=ORIENTED_EDGE('',*,*,#44548,.T.) ;
#59620=ORIENTED_EDGE('',*,*,#44549,.T.) ;
#59621=ORIENTED_EDGE('',*,*,#44550,.T.) ;
#59622=ORIENTED_EDGE('',*,*,#44551,.F.) ;
#59623=ORIENTED_EDGE('',*,*,#44552,.T.) ;
#59624=ORIENTED_EDGE('',*,*,#44553,.T.) ;
#59625=ORIENTED_EDGE('',*,*,#44554,.T.) ;
#59626=ORIENTED_EDGE('',*,*,#44555,.T.) ;
#59627=ORIENTED_EDGE('',*,*,#44556,.F.) ;
#59628=ORIENTED_EDGE('',*,*,#44557,.T.) ;
#59629=ORIENTED_EDGE('',*,*,#44558,.T.) ;
#59630=ORIENTED_EDGE('',*,*,#44559,.T.) ;
#59631=ORIENTED_EDGE('',*,*,#44560,.T.) ;
#59632=ORIENTED_EDGE('',*,*,#44561,.F.) ;
#59633=ORIENTED_EDGE('',*,*,#44562,.T.) ;
#59634=ORIENTED_EDGE('',*,*,#44563,.T.) ;
#59635=ORIENTED_EDGE('',*,*,#44564,.T.) ;
#59636=ORIENTED_EDGE('',*,*,#44565,.T.) ;
#59637=ORIENTED_EDGE('',*,*,#44566,.F.) ;
#59638=ORIENTED_EDGE('',*,*,#44567,.T.) ;
#59639=ORIENTED_EDGE('',*,*,#44568,.T.) ;
#59640=ORIENTED_EDGE('',*,*,#44569,.T.) ;
#59641=ORIENTED_EDGE('',*,*,#44570,.T.) ;
#59642=ORIENTED_EDGE('',*,*,#44571,.F.) ;
#59643=ORIENTED_EDGE('',*,*,#44572,.T.) ;
#59644=ORIENTED_EDGE('',*,*,#44573,.T.) ;
#59645=ORIENTED_EDGE('',*,*,#44574,.T.) ;
#59646=ORIENTED_EDGE('',*,*,#44575,.T.) ;
#59647=ORIENTED_EDGE('',*,*,#44576,.F.) ;
#59648=ORIENTED_EDGE('',*,*,#44577,.T.) ;
#59649=ORIENTED_EDGE('',*,*,#44578,.T.) ;
#59650=ORIENTED_EDGE('',*,*,#44579,.T.) ;
#59651=ORIENTED_EDGE('',*,*,#44580,.T.) ;
#59652=ORIENTED_EDGE('',*,*,#44581,.F.) ;
#59653=ORIENTED_EDGE('',*,*,#44582,.T.) ;
#59654=ORIENTED_EDGE('',*,*,#44583,.T.) ;
#59655=ORIENTED_EDGE('',*,*,#44584,.T.) ;
#59656=ORIENTED_EDGE('',*,*,#44585,.T.) ;
#59657=ORIENTED_EDGE('',*,*,#44586,.F.) ;
#59658=ORIENTED_EDGE('',*,*,#44587,.T.) ;
#59659=ORIENTED_EDGE('',*,*,#44588,.T.) ;
#59660=ORIENTED_EDGE('',*,*,#44589,.T.) ;
#59661=ORIENTED_EDGE('',*,*,#44590,.F.) ;
#59662=ORIENTED_EDGE('',*,*,#44591,.T.) ;
#59663=ORIENTED_EDGE('',*,*,#44592,.T.) ;
#59664=ORIENTED_EDGE('',*,*,#44593,.T.) ;
#59665=ORIENTED_EDGE('',*,*,#44594,.F.) ;
#59666=ORIENTED_EDGE('',*,*,#44595,.T.) ;
#59667=ORIENTED_EDGE('',*,*,#44596,.T.) ;
#59668=ORIENTED_EDGE('',*,*,#44597,.T.) ;
#59669=ORIENTED_EDGE('',*,*,#44598,.F.) ;
#59670=ORIENTED_EDGE('',*,*,#44599,.T.) ;
#59671=ORIENTED_EDGE('',*,*,#44600,.T.) ;
#59672=ORIENTED_EDGE('',*,*,#44601,.T.) ;
#59673=ORIENTED_EDGE('',*,*,#44602,.F.) ;
#59674=ORIENTED_EDGE('',*,*,#44603,.T.) ;
#59675=ORIENTED_EDGE('',*,*,#44604,.T.) ;
#59676=ORIENTED_EDGE('',*,*,#44605,.T.) ;
#59677=ORIENTED_EDGE('',*,*,#44606,.F.) ;
#59678=ORIENTED_EDGE('',*,*,#44607,.T.) ;
#59679=ORIENTED_EDGE('',*,*,#44608,.T.) ;
#59680=ORIENTED_EDGE('',*,*,#44609,.T.) ;
#59681=ORIENTED_EDGE('',*,*,#44610,.F.) ;
#59682=ORIENTED_EDGE('',*,*,#44611,.T.) ;
#59683=ORIENTED_EDGE('',*,*,#44612,.T.) ;
#59684=ORIENTED_EDGE('',*,*,#44613,.T.) ;
#59685=ORIENTED_EDGE('',*,*,#44614,.F.) ;
#59686=ORIENTED_EDGE('',*,*,#44615,.T.) ;
#59687=ORIENTED_EDGE('',*,*,#44616,.T.) ;
#59688=ORIENTED_EDGE('',*,*,#44617,.T.) ;
#59689=ORIENTED_EDGE('',*,*,#44618,.F.) ;
#59690=ORIENTED_EDGE('',*,*,#44619,.T.) ;
#59691=ORIENTED_EDGE('',*,*,#44620,.T.) ;
#59692=ORIENTED_EDGE('',*,*,#44621,.T.) ;
#59693=ORIENTED_EDGE('',*,*,#44622,.T.) ;
#59694=ORIENTED_EDGE('',*,*,#44623,.T.) ;
#59695=ORIENTED_EDGE('',*,*,#44624,.T.) ;
#59696=ORIENTED_EDGE('',*,*,#44625,.T.) ;
#59697=ORIENTED_EDGE('',*,*,#44390,.T.) ;
#59698=ORIENTED_EDGE('',*,*,#44626,.F.) ;
#59699=ORIENTED_EDGE('',*,*,#44627,.T.) ;
#59700=ORIENTED_EDGE('',*,*,#44628,.T.) ;
#59701=ORIENTED_EDGE('',*,*,#44629,.T.) ;
#59702=ORIENTED_EDGE('',*,*,#44630,.T.) ;
#59703=ORIENTED_EDGE('',*,*,#44631,.T.) ;
#59704=ORIENTED_EDGE('',*,*,#44632,.F.) ;
#59705=ORIENTED_EDGE('',*,*,#44633,.F.) ;
#59706=ORIENTED_EDGE('',*,*,#44634,.T.) ;
#59707=ORIENTED_EDGE('',*,*,#44635,.T.) ;
#59708=ORIENTED_EDGE('',*,*,#44636,.T.) ;
#59709=ORIENTED_EDGE('',*,*,#44637,.T.) ;
#59710=ORIENTED_EDGE('',*,*,#44638,.F.) ;
#59711=ORIENTED_EDGE('',*,*,#44639,.T.) ;
#59712=ORIENTED_EDGE('',*,*,#44640,.T.) ;
#59713=ORIENTED_EDGE('',*,*,#44641,.T.) ;
#59714=ORIENTED_EDGE('',*,*,#44642,.T.) ;
#59715=ORIENTED_EDGE('',*,*,#44643,.F.) ;
#59716=ORIENTED_EDGE('',*,*,#44644,.T.) ;
#59717=ORIENTED_EDGE('',*,*,#44645,.T.) ;
#59718=ORIENTED_EDGE('',*,*,#44646,.T.) ;
#59719=ORIENTED_EDGE('',*,*,#44647,.F.) ;
#59720=ORIENTED_EDGE('',*,*,#44648,.T.) ;
#59721=ORIENTED_EDGE('',*,*,#44649,.T.) ;
#59722=ORIENTED_EDGE('',*,*,#44650,.T.) ;
#59723=ORIENTED_EDGE('',*,*,#44651,.F.) ;
#59724=ORIENTED_EDGE('',*,*,#44652,.T.) ;
#59725=ORIENTED_EDGE('',*,*,#44653,.F.) ;
#59726=ORIENTED_EDGE('',*,*,#44654,.T.) ;
#59727=ORIENTED_EDGE('',*,*,#44647,.T.) ;
#59728=ORIENTED_EDGE('',*,*,#44655,.T.) ;
#59729=ORIENTED_EDGE('',*,*,#44645,.F.) ;
#59730=ORIENTED_EDGE('',*,*,#44656,.T.) ;
#59731=ORIENTED_EDGE('',*,*,#44657,.F.) ;
#59732=ORIENTED_EDGE('',*,*,#44658,.T.) ;
#59733=ORIENTED_EDGE('',*,*,#44659,.F.) ;
#59734=ORIENTED_EDGE('',*,*,#44660,.T.) ;
#59735=ORIENTED_EDGE('',*,*,#44588,.F.) ;
#59736=ORIENTED_EDGE('',*,*,#44661,.T.) ;
#59737=ORIENTED_EDGE('',*,*,#44662,.F.) ;
#59738=ORIENTED_EDGE('',*,*,#44663,.T.) ;
#59739=ORIENTED_EDGE('',*,*,#44664,.F.) ;
#59740=ORIENTED_EDGE('',*,*,#44665,.T.) ;
#59741=ORIENTED_EDGE('',*,*,#44592,.F.) ;
#59742=ORIENTED_EDGE('',*,*,#44666,.T.) ;
#59743=ORIENTED_EDGE('',*,*,#44667,.F.) ;
#59744=ORIENTED_EDGE('',*,*,#44668,.T.) ;
#59745=ORIENTED_EDGE('',*,*,#44669,.F.) ;
#59746=ORIENTED_EDGE('',*,*,#44670,.T.) ;
#59747=ORIENTED_EDGE('',*,*,#44596,.F.) ;
#59748=ORIENTED_EDGE('',*,*,#44671,.T.) ;
#59749=ORIENTED_EDGE('',*,*,#44672,.F.) ;
#59750=ORIENTED_EDGE('',*,*,#44673,.T.) ;
#59751=ORIENTED_EDGE('',*,*,#44674,.F.) ;
#59752=ORIENTED_EDGE('',*,*,#44675,.T.) ;
#59753=ORIENTED_EDGE('',*,*,#44600,.F.) ;
#59754=ORIENTED_EDGE('',*,*,#44676,.T.) ;
#59755=ORIENTED_EDGE('',*,*,#44677,.F.) ;
#59756=ORIENTED_EDGE('',*,*,#44678,.T.) ;
#59757=ORIENTED_EDGE('',*,*,#44679,.F.) ;
#59758=ORIENTED_EDGE('',*,*,#44680,.T.) ;
#59759=ORIENTED_EDGE('',*,*,#44604,.F.) ;
#59760=ORIENTED_EDGE('',*,*,#44681,.T.) ;
#59761=ORIENTED_EDGE('',*,*,#44682,.F.) ;
#59762=ORIENTED_EDGE('',*,*,#44683,.T.) ;
#59763=ORIENTED_EDGE('',*,*,#44684,.F.) ;
#59764=ORIENTED_EDGE('',*,*,#44685,.T.) ;
#59765=ORIENTED_EDGE('',*,*,#44608,.F.) ;
#59766=ORIENTED_EDGE('',*,*,#44686,.T.) ;
#59767=ORIENTED_EDGE('',*,*,#44687,.F.) ;
#59768=ORIENTED_EDGE('',*,*,#44688,.T.) ;
#59769=ORIENTED_EDGE('',*,*,#44689,.F.) ;
#59770=ORIENTED_EDGE('',*,*,#44690,.T.) ;
#59771=ORIENTED_EDGE('',*,*,#44612,.F.) ;
#59772=ORIENTED_EDGE('',*,*,#44691,.T.) ;
#59773=ORIENTED_EDGE('',*,*,#44692,.F.) ;
#59774=ORIENTED_EDGE('',*,*,#44693,.T.) ;
#59775=ORIENTED_EDGE('',*,*,#44694,.F.) ;
#59776=ORIENTED_EDGE('',*,*,#44695,.T.) ;
#59777=ORIENTED_EDGE('',*,*,#44616,.F.) ;
#59778=ORIENTED_EDGE('',*,*,#44696,.T.) ;
#59779=ORIENTED_EDGE('',*,*,#44697,.F.) ;
#59780=ORIENTED_EDGE('',*,*,#44698,.T.) ;
#59781=ORIENTED_EDGE('',*,*,#44699,.F.) ;
#59782=ORIENTED_EDGE('',*,*,#44700,.T.) ;
#59783=ORIENTED_EDGE('',*,*,#44620,.F.) ;
#59784=ORIENTED_EDGE('',*,*,#44701,.T.) ;
#59785=ORIENTED_EDGE('',*,*,#44702,.F.) ;
#59786=ORIENTED_EDGE('',*,*,#44703,.T.) ;
#59787=ORIENTED_EDGE('',*,*,#44653,.T.) ;
#59788=ORIENTED_EDGE('',*,*,#44704,.T.) ;
#59789=ORIENTED_EDGE('',*,*,#44705,.F.) ;
#59790=ORIENTED_EDGE('',*,*,#44706,.T.) ;
#59791=ORIENTED_EDGE('',*,*,#44707,.F.) ;
#59792=ORIENTED_EDGE('',*,*,#44708,.T.) ;
#59793=ORIENTED_EDGE('',*,*,#44618,.T.) ;
#59794=ORIENTED_EDGE('',*,*,#44709,.T.) ;
#59795=ORIENTED_EDGE('',*,*,#44710,.F.) ;
#59796=ORIENTED_EDGE('',*,*,#44711,.T.) ;
#59797=ORIENTED_EDGE('',*,*,#44712,.F.) ;
#59798=ORIENTED_EDGE('',*,*,#44713,.T.) ;
#59799=ORIENTED_EDGE('',*,*,#44614,.T.) ;
#59800=ORIENTED_EDGE('',*,*,#44714,.T.) ;
#59801=ORIENTED_EDGE('',*,*,#44715,.F.) ;
#59802=ORIENTED_EDGE('',*,*,#44716,.T.) ;
#59803=ORIENTED_EDGE('',*,*,#44717,.F.) ;
#59804=ORIENTED_EDGE('',*,*,#44718,.T.) ;
#59805=ORIENTED_EDGE('',*,*,#44610,.T.) ;
#59806=ORIENTED_EDGE('',*,*,#44719,.T.) ;
#59807=ORIENTED_EDGE('',*,*,#44720,.F.) ;
#59808=ORIENTED_EDGE('',*,*,#44721,.T.) ;
#59809=ORIENTED_EDGE('',*,*,#44722,.F.) ;
#59810=ORIENTED_EDGE('',*,*,#44723,.T.) ;
#59811=ORIENTED_EDGE('',*,*,#44606,.T.) ;
#59812=ORIENTED_EDGE('',*,*,#44724,.T.) ;
#59813=ORIENTED_EDGE('',*,*,#44725,.F.) ;
#59814=ORIENTED_EDGE('',*,*,#44726,.T.) ;
#59815=ORIENTED_EDGE('',*,*,#44727,.F.) ;
#59816=ORIENTED_EDGE('',*,*,#44728,.T.) ;
#59817=ORIENTED_EDGE('',*,*,#44602,.T.) ;
#59818=ORIENTED_EDGE('',*,*,#44729,.T.) ;
#59819=ORIENTED_EDGE('',*,*,#44730,.F.) ;
#59820=ORIENTED_EDGE('',*,*,#44731,.T.) ;
#59821=ORIENTED_EDGE('',*,*,#44732,.F.) ;
#59822=ORIENTED_EDGE('',*,*,#44733,.T.) ;
#59823=ORIENTED_EDGE('',*,*,#44598,.T.) ;
#59824=ORIENTED_EDGE('',*,*,#44734,.T.) ;
#59825=ORIENTED_EDGE('',*,*,#44735,.F.) ;
#59826=ORIENTED_EDGE('',*,*,#44736,.T.) ;
#59827=ORIENTED_EDGE('',*,*,#44737,.F.) ;
#59828=ORIENTED_EDGE('',*,*,#44738,.T.) ;
#59829=ORIENTED_EDGE('',*,*,#44594,.T.) ;
#59830=ORIENTED_EDGE('',*,*,#44739,.T.) ;
#59831=ORIENTED_EDGE('',*,*,#44740,.F.) ;
#59832=ORIENTED_EDGE('',*,*,#44741,.T.) ;
#59833=ORIENTED_EDGE('',*,*,#44742,.F.) ;
#59834=ORIENTED_EDGE('',*,*,#44743,.T.) ;
#59835=ORIENTED_EDGE('',*,*,#44590,.T.) ;
#59836=ORIENTED_EDGE('',*,*,#44744,.T.) ;
#59837=ORIENTED_EDGE('',*,*,#44745,.F.) ;
#59838=ORIENTED_EDGE('',*,*,#44746,.T.) ;
#59839=ORIENTED_EDGE('',*,*,#44747,.F.) ;
#59840=ORIENTED_EDGE('',*,*,#44748,.T.) ;
#59841=ORIENTED_EDGE('',*,*,#44586,.T.) ;
#59842=ORIENTED_EDGE('',*,*,#44749,.T.) ;
#59843=ORIENTED_EDGE('',*,*,#44750,.F.) ;
#59844=ORIENTED_EDGE('',*,*,#44751,.T.) ;
#59845=ORIENTED_EDGE('',*,*,#44752,.F.) ;
#59846=ORIENTED_EDGE('',*,*,#44753,.T.) ;
#59847=ORIENTED_EDGE('',*,*,#44643,.T.) ;
#59848=ORIENTED_EDGE('',*,*,#44754,.T.) ;
#59849=ORIENTED_EDGE('',*,*,#44755,.F.) ;
#59850=ORIENTED_EDGE('',*,*,#44756,.T.) ;
#59851=ORIENTED_EDGE('',*,*,#44705,.T.) ;
#59852=ORIENTED_EDGE('',*,*,#44757,.T.) ;
#59853=ORIENTED_EDGE('',*,*,#44758,.F.) ;
#59854=ORIENTED_EDGE('',*,*,#44759,.T.) ;
#59855=ORIENTED_EDGE('',*,*,#44760,.F.) ;
#59856=ORIENTED_EDGE('',*,*,#44761,.T.) ;
#59857=ORIENTED_EDGE('',*,*,#44755,.T.) ;
#59858=ORIENTED_EDGE('',*,*,#44762,.T.) ;
#59859=ORIENTED_EDGE('',*,*,#44763,.F.) ;
#59860=ORIENTED_EDGE('',*,*,#44764,.T.) ;
#59861=ORIENTED_EDGE('',*,*,#44760,.T.) ;
#59862=ORIENTED_EDGE('',*,*,#44765,.T.) ;
#59863=ORIENTED_EDGE('',*,*,#44766,.F.) ;
#59864=ORIENTED_EDGE('',*,*,#44767,.T.) ;
#59865=ORIENTED_EDGE('',*,*,#44763,.T.) ;
#59866=ORIENTED_EDGE('',*,*,#44768,.T.) ;
#59867=ORIENTED_EDGE('',*,*,#44769,.F.) ;
#59868=ORIENTED_EDGE('',*,*,#44770,.T.) ;
#59869=ORIENTED_EDGE('',*,*,#44766,.T.) ;
#59870=ORIENTED_EDGE('',*,*,#44771,.T.) ;
#59871=ORIENTED_EDGE('',*,*,#44772,.F.) ;
#59872=ORIENTED_EDGE('',*,*,#44773,.T.) ;
#59873=ORIENTED_EDGE('',*,*,#44769,.T.) ;
#59874=ORIENTED_EDGE('',*,*,#44774,.T.) ;
#59875=ORIENTED_EDGE('',*,*,#44775,.F.) ;
#59876=ORIENTED_EDGE('',*,*,#44776,.T.) ;
#59877=ORIENTED_EDGE('',*,*,#44772,.T.) ;
#59878=ORIENTED_EDGE('',*,*,#44777,.T.) ;
#59879=ORIENTED_EDGE('',*,*,#44778,.F.) ;
#59880=ORIENTED_EDGE('',*,*,#44779,.T.) ;
#59881=ORIENTED_EDGE('',*,*,#44775,.T.) ;
#59882=ORIENTED_EDGE('',*,*,#44780,.T.) ;
#59883=ORIENTED_EDGE('',*,*,#44781,.F.) ;
#59884=ORIENTED_EDGE('',*,*,#44782,.T.) ;
#59885=ORIENTED_EDGE('',*,*,#44778,.T.) ;
#59886=ORIENTED_EDGE('',*,*,#44783,.T.) ;
#59887=ORIENTED_EDGE('',*,*,#44784,.F.) ;
#59888=ORIENTED_EDGE('',*,*,#44785,.T.) ;
#59889=ORIENTED_EDGE('',*,*,#44781,.T.) ;
#59890=ORIENTED_EDGE('',*,*,#44786,.T.) ;
#59891=ORIENTED_EDGE('',*,*,#44787,.F.) ;
#59892=ORIENTED_EDGE('',*,*,#44788,.T.) ;
#59893=ORIENTED_EDGE('',*,*,#44784,.T.) ;
#59894=ORIENTED_EDGE('',*,*,#44789,.T.) ;
#59895=ORIENTED_EDGE('',*,*,#44790,.F.) ;
#59896=ORIENTED_EDGE('',*,*,#44791,.T.) ;
#59897=ORIENTED_EDGE('',*,*,#44787,.T.) ;
#59898=ORIENTED_EDGE('',*,*,#44792,.T.) ;
#59899=ORIENTED_EDGE('',*,*,#44649,.F.) ;
#59900=ORIENTED_EDGE('',*,*,#44793,.T.) ;
#59901=ORIENTED_EDGE('',*,*,#44790,.T.) ;
#59902=ORIENTED_EDGE('',*,*,#44794,.T.) ;
#59903=ORIENTED_EDGE('',*,*,#44795,.T.) ;
#59904=ORIENTED_EDGE('',*,*,#44796,.T.) ;
#59905=ORIENTED_EDGE('',*,*,#44797,.T.) ;
#59906=ORIENTED_EDGE('',*,*,#44798,.T.) ;
#59907=ORIENTED_EDGE('',*,*,#44799,.T.) ;
#59908=ORIENTED_EDGE('',*,*,#44800,.T.) ;
#59909=ORIENTED_EDGE('',*,*,#44801,.T.) ;
#59910=ORIENTED_EDGE('',*,*,#44802,.T.) ;
#59911=ORIENTED_EDGE('',*,*,#44319,.T.) ;
#59912=ORIENTED_EDGE('',*,*,#44803,.T.) ;
#59913=ORIENTED_EDGE('',*,*,#44804,.T.) ;
#59914=ORIENTED_EDGE('',*,*,#44805,.T.) ;
#59915=ORIENTED_EDGE('',*,*,#44806,.T.) ;
#59916=ORIENTED_EDGE('',*,*,#44807,.T.) ;
#59917=ORIENTED_EDGE('',*,*,#44808,.T.) ;
#59918=ORIENTED_EDGE('',*,*,#44809,.T.) ;
#59919=ORIENTED_EDGE('',*,*,#44810,.T.) ;
#59920=ORIENTED_EDGE('',*,*,#44811,.T.) ;
#59921=ORIENTED_EDGE('',*,*,#44812,.T.) ;
#59922=ORIENTED_EDGE('',*,*,#44813,.T.) ;
#59923=ORIENTED_EDGE('',*,*,#44814,.T.) ;
#59924=ORIENTED_EDGE('',*,*,#44815,.T.) ;
#59925=ORIENTED_EDGE('',*,*,#44816,.T.) ;
#59926=ORIENTED_EDGE('',*,*,#44817,.T.) ;
#59927=ORIENTED_EDGE('',*,*,#44818,.T.) ;
#59928=ORIENTED_EDGE('',*,*,#44819,.T.) ;
#59929=ORIENTED_EDGE('',*,*,#44820,.T.) ;
#59930=ORIENTED_EDGE('',*,*,#44821,.T.) ;
#59931=ORIENTED_EDGE('',*,*,#44822,.T.) ;
#59932=ORIENTED_EDGE('',*,*,#44823,.T.) ;
#59933=ORIENTED_EDGE('',*,*,#44824,.T.) ;
#59934=ORIENTED_EDGE('',*,*,#44825,.T.) ;
#59935=ORIENTED_EDGE('',*,*,#44315,.T.) ;
#59936=ORIENTED_EDGE('',*,*,#44826,.T.) ;
#59937=ORIENTED_EDGE('',*,*,#44827,.T.) ;
#59938=ORIENTED_EDGE('',*,*,#44828,.T.) ;
#59939=ORIENTED_EDGE('',*,*,#44829,.T.) ;
#59940=ORIENTED_EDGE('',*,*,#44830,.T.) ;
#59941=ORIENTED_EDGE('',*,*,#44831,.T.) ;
#59942=ORIENTED_EDGE('',*,*,#44832,.T.) ;
#59943=ORIENTED_EDGE('',*,*,#44833,.T.) ;
#59944=ORIENTED_EDGE('',*,*,#44834,.T.) ;
#59945=ORIENTED_EDGE('',*,*,#44835,.T.) ;
#59946=ORIENTED_EDGE('',*,*,#44836,.T.) ;
#59947=ORIENTED_EDGE('',*,*,#44837,.T.) ;
#59948=ORIENTED_EDGE('',*,*,#44838,.T.) ;
#59949=ORIENTED_EDGE('',*,*,#44839,.T.) ;
#59950=ORIENTED_EDGE('',*,*,#44840,.T.) ;
#59951=ORIENTED_EDGE('',*,*,#44841,.T.) ;
#59952=ORIENTED_EDGE('',*,*,#44842,.T.) ;
#59953=ORIENTED_EDGE('',*,*,#44843,.T.) ;
#59954=ORIENTED_EDGE('',*,*,#44844,.T.) ;
#59955=ORIENTED_EDGE('',*,*,#44845,.T.) ;
#59956=ORIENTED_EDGE('',*,*,#44846,.T.) ;
#59957=ORIENTED_EDGE('',*,*,#44847,.T.) ;
#59958=ORIENTED_EDGE('',*,*,#44848,.T.) ;
#59959=ORIENTED_EDGE('',*,*,#44311,.T.) ;
#59960=ORIENTED_EDGE('',*,*,#44849,.T.) ;
#59961=ORIENTED_EDGE('',*,*,#44850,.T.) ;
#59962=ORIENTED_EDGE('',*,*,#44851,.T.) ;
#59963=ORIENTED_EDGE('',*,*,#44852,.T.) ;
#59964=ORIENTED_EDGE('',*,*,#44853,.T.) ;
#59965=ORIENTED_EDGE('',*,*,#44854,.T.) ;
#59966=ORIENTED_EDGE('',*,*,#44855,.T.) ;
#59967=ORIENTED_EDGE('',*,*,#44856,.T.) ;
#59968=ORIENTED_EDGE('',*,*,#44857,.T.) ;
#59969=ORIENTED_EDGE('',*,*,#44858,.T.) ;
#59970=ORIENTED_EDGE('',*,*,#44859,.T.) ;
#59971=ORIENTED_EDGE('',*,*,#44860,.T.) ;
#59972=ORIENTED_EDGE('',*,*,#44861,.T.) ;
#59973=ORIENTED_EDGE('',*,*,#44862,.T.) ;
#59974=ORIENTED_EDGE('',*,*,#44863,.T.) ;
#59975=ORIENTED_EDGE('',*,*,#44864,.T.) ;
#59976=ORIENTED_EDGE('',*,*,#44865,.T.) ;
#59977=ORIENTED_EDGE('',*,*,#44866,.T.) ;
#59978=ORIENTED_EDGE('',*,*,#44867,.T.) ;
#59979=ORIENTED_EDGE('',*,*,#44868,.T.) ;
#59980=ORIENTED_EDGE('',*,*,#44869,.T.) ;
#59981=ORIENTED_EDGE('',*,*,#44870,.T.) ;
#59982=ORIENTED_EDGE('',*,*,#44871,.T.) ;
#59983=ORIENTED_EDGE('',*,*,#44307,.T.) ;
#59984=ORIENTED_EDGE('',*,*,#44872,.T.) ;
#59985=ORIENTED_EDGE('',*,*,#44873,.T.) ;
#59986=ORIENTED_EDGE('',*,*,#44874,.T.) ;
#59987=ORIENTED_EDGE('',*,*,#44875,.T.) ;
#59988=ORIENTED_EDGE('',*,*,#44876,.T.) ;
#59989=ORIENTED_EDGE('',*,*,#44877,.T.) ;
#59990=ORIENTED_EDGE('',*,*,#44878,.T.) ;
#59991=ORIENTED_EDGE('',*,*,#44879,.T.) ;
#59992=ORIENTED_EDGE('',*,*,#44880,.T.) ;
#59993=ORIENTED_EDGE('',*,*,#44881,.T.) ;
#59994=ORIENTED_EDGE('',*,*,#44882,.T.) ;
#59995=ORIENTED_EDGE('',*,*,#44883,.T.) ;
#59996=ORIENTED_EDGE('',*,*,#44884,.T.) ;
#59997=ORIENTED_EDGE('',*,*,#44885,.T.) ;
#59998=ORIENTED_EDGE('',*,*,#44886,.T.) ;
#59999=ORIENTED_EDGE('',*,*,#44887,.T.) ;
#60000=ORIENTED_EDGE('',*,*,#44888,.T.) ;
#60001=ORIENTED_EDGE('',*,*,#44889,.T.) ;
#60002=ORIENTED_EDGE('',*,*,#44890,.T.) ;
#60003=ORIENTED_EDGE('',*,*,#44891,.T.) ;
#60004=ORIENTED_EDGE('',*,*,#44892,.T.) ;
#60005=ORIENTED_EDGE('',*,*,#44893,.T.) ;
#60006=ORIENTED_EDGE('',*,*,#44894,.T.) ;
#60007=ORIENTED_EDGE('',*,*,#44303,.T.) ;
#60008=ORIENTED_EDGE('',*,*,#44895,.T.) ;
#60009=ORIENTED_EDGE('',*,*,#44896,.T.) ;
#60010=ORIENTED_EDGE('',*,*,#44897,.T.) ;
#60011=ORIENTED_EDGE('',*,*,#44898,.T.) ;
#60012=ORIENTED_EDGE('',*,*,#44899,.T.) ;
#60013=ORIENTED_EDGE('',*,*,#44900,.T.) ;
#60014=ORIENTED_EDGE('',*,*,#44901,.T.) ;
#60015=ORIENTED_EDGE('',*,*,#44902,.T.) ;
#60016=ORIENTED_EDGE('',*,*,#44903,.T.) ;
#60017=ORIENTED_EDGE('',*,*,#44904,.T.) ;
#60018=ORIENTED_EDGE('',*,*,#44905,.T.) ;
#60019=ORIENTED_EDGE('',*,*,#44906,.T.) ;
#60020=ORIENTED_EDGE('',*,*,#44907,.T.) ;
#60021=ORIENTED_EDGE('',*,*,#44908,.T.) ;
#60022=ORIENTED_EDGE('',*,*,#44909,.T.) ;
#60023=ORIENTED_EDGE('',*,*,#44910,.T.) ;
#60024=ORIENTED_EDGE('',*,*,#44911,.T.) ;
#60025=ORIENTED_EDGE('',*,*,#44912,.T.) ;
#60026=ORIENTED_EDGE('',*,*,#44913,.T.) ;
#60027=ORIENTED_EDGE('',*,*,#44914,.T.) ;
#60028=ORIENTED_EDGE('',*,*,#44915,.T.) ;
#60029=ORIENTED_EDGE('',*,*,#44916,.T.) ;
#60030=ORIENTED_EDGE('',*,*,#44917,.T.) ;
#60031=ORIENTED_EDGE('',*,*,#44299,.T.) ;
#60032=ORIENTED_EDGE('',*,*,#44918,.T.) ;
#60033=ORIENTED_EDGE('',*,*,#44919,.T.) ;
#60034=ORIENTED_EDGE('',*,*,#44920,.T.) ;
#60035=ORIENTED_EDGE('',*,*,#44921,.T.) ;
#60036=ORIENTED_EDGE('',*,*,#44922,.T.) ;
#60037=ORIENTED_EDGE('',*,*,#44923,.T.) ;
#60038=ORIENTED_EDGE('',*,*,#44924,.T.) ;
#60039=ORIENTED_EDGE('',*,*,#44925,.T.) ;
#60040=ORIENTED_EDGE('',*,*,#44926,.T.) ;
#60041=ORIENTED_EDGE('',*,*,#44927,.T.) ;
#60042=ORIENTED_EDGE('',*,*,#44928,.T.) ;
#60043=ORIENTED_EDGE('',*,*,#44929,.T.) ;
#60044=ORIENTED_EDGE('',*,*,#44930,.T.) ;
#60045=ORIENTED_EDGE('',*,*,#44931,.T.) ;
#60046=ORIENTED_EDGE('',*,*,#44932,.T.) ;
#60047=ORIENTED_EDGE('',*,*,#44933,.T.) ;
#60048=ORIENTED_EDGE('',*,*,#44934,.T.) ;
#60049=ORIENTED_EDGE('',*,*,#44935,.T.) ;
#60050=ORIENTED_EDGE('',*,*,#44936,.T.) ;
#60051=ORIENTED_EDGE('',*,*,#44937,.T.) ;
#60052=ORIENTED_EDGE('',*,*,#44938,.T.) ;
#60053=ORIENTED_EDGE('',*,*,#44939,.T.) ;
#60054=ORIENTED_EDGE('',*,*,#44940,.T.) ;
#60055=ORIENTED_EDGE('',*,*,#44295,.T.) ;
#60056=ORIENTED_EDGE('',*,*,#44941,.T.) ;
#60057=ORIENTED_EDGE('',*,*,#44942,.T.) ;
#60058=ORIENTED_EDGE('',*,*,#44943,.T.) ;
#60059=ORIENTED_EDGE('',*,*,#44944,.T.) ;
#60060=ORIENTED_EDGE('',*,*,#44945,.T.) ;
#60061=ORIENTED_EDGE('',*,*,#44946,.T.) ;
#60062=ORIENTED_EDGE('',*,*,#44947,.T.) ;
#60063=ORIENTED_EDGE('',*,*,#44948,.T.) ;
#60064=ORIENTED_EDGE('',*,*,#44949,.T.) ;
#60065=ORIENTED_EDGE('',*,*,#44950,.T.) ;
#60066=ORIENTED_EDGE('',*,*,#44951,.T.) ;
#60067=ORIENTED_EDGE('',*,*,#44952,.T.) ;
#60068=ORIENTED_EDGE('',*,*,#44953,.T.) ;
#60069=ORIENTED_EDGE('',*,*,#44954,.T.) ;
#60070=ORIENTED_EDGE('',*,*,#44955,.T.) ;
#60071=ORIENTED_EDGE('',*,*,#44956,.T.) ;
#60072=ORIENTED_EDGE('',*,*,#44957,.T.) ;
#60073=ORIENTED_EDGE('',*,*,#44958,.T.) ;
#60074=ORIENTED_EDGE('',*,*,#44959,.T.) ;
#60075=ORIENTED_EDGE('',*,*,#44960,.T.) ;
#60076=ORIENTED_EDGE('',*,*,#44961,.T.) ;
#60077=ORIENTED_EDGE('',*,*,#44962,.T.) ;
#60078=ORIENTED_EDGE('',*,*,#44963,.T.) ;
#60079=ORIENTED_EDGE('',*,*,#44291,.T.) ;
#60080=ORIENTED_EDGE('',*,*,#44964,.T.) ;
#60081=ORIENTED_EDGE('',*,*,#44965,.T.) ;
#60082=ORIENTED_EDGE('',*,*,#44966,.T.) ;
#60083=ORIENTED_EDGE('',*,*,#44967,.T.) ;
#60084=ORIENTED_EDGE('',*,*,#44968,.T.) ;
#60085=ORIENTED_EDGE('',*,*,#44969,.T.) ;
#60086=ORIENTED_EDGE('',*,*,#44970,.T.) ;
#60087=ORIENTED_EDGE('',*,*,#44971,.T.) ;
#60088=ORIENTED_EDGE('',*,*,#44972,.T.) ;
#60089=ORIENTED_EDGE('',*,*,#44973,.T.) ;
#60090=ORIENTED_EDGE('',*,*,#44974,.T.) ;
#60091=ORIENTED_EDGE('',*,*,#44975,.T.) ;
#60092=ORIENTED_EDGE('',*,*,#44976,.T.) ;
#60093=ORIENTED_EDGE('',*,*,#44977,.T.) ;
#60094=ORIENTED_EDGE('',*,*,#44978,.T.) ;
#60095=ORIENTED_EDGE('',*,*,#44979,.T.) ;
#60096=ORIENTED_EDGE('',*,*,#44980,.T.) ;
#60097=ORIENTED_EDGE('',*,*,#44981,.T.) ;
#60098=ORIENTED_EDGE('',*,*,#44982,.T.) ;
#60099=ORIENTED_EDGE('',*,*,#44983,.T.) ;
#60100=ORIENTED_EDGE('',*,*,#44984,.T.) ;
#60101=ORIENTED_EDGE('',*,*,#44985,.T.) ;
#60102=ORIENTED_EDGE('',*,*,#44986,.T.) ;
#60103=ORIENTED_EDGE('',*,*,#44287,.T.) ;
#60104=ORIENTED_EDGE('',*,*,#44987,.T.) ;
#60105=ORIENTED_EDGE('',*,*,#44988,.T.) ;
#60106=ORIENTED_EDGE('',*,*,#44989,.T.) ;
#60107=ORIENTED_EDGE('',*,*,#44990,.T.) ;
#60108=ORIENTED_EDGE('',*,*,#44991,.T.) ;
#60109=ORIENTED_EDGE('',*,*,#44992,.T.) ;
#60110=ORIENTED_EDGE('',*,*,#44993,.T.) ;
#60111=ORIENTED_EDGE('',*,*,#44994,.T.) ;
#60112=ORIENTED_EDGE('',*,*,#44995,.T.) ;
#60113=ORIENTED_EDGE('',*,*,#44996,.T.) ;
#60114=ORIENTED_EDGE('',*,*,#44997,.T.) ;
#60115=ORIENTED_EDGE('',*,*,#44998,.T.) ;
#60116=ORIENTED_EDGE('',*,*,#44999,.T.) ;
#60117=ORIENTED_EDGE('',*,*,#45000,.T.) ;
#60118=ORIENTED_EDGE('',*,*,#45001,.T.) ;
#60119=ORIENTED_EDGE('',*,*,#45002,.T.) ;
#60120=ORIENTED_EDGE('',*,*,#45003,.T.) ;
#60121=ORIENTED_EDGE('',*,*,#45004,.T.) ;
#60122=ORIENTED_EDGE('',*,*,#45005,.T.) ;
#60123=ORIENTED_EDGE('',*,*,#45006,.T.) ;
#60124=ORIENTED_EDGE('',*,*,#45007,.T.) ;
#60125=ORIENTED_EDGE('',*,*,#45008,.T.) ;
#60126=ORIENTED_EDGE('',*,*,#45009,.T.) ;
#60127=ORIENTED_EDGE('',*,*,#44376,.T.) ;
#60128=ORIENTED_EDGE('',*,*,#45010,.T.) ;
#60129=ORIENTED_EDGE('',*,*,#45011,.T.) ;
#60130=ORIENTED_EDGE('',*,*,#45012,.T.) ;
#60131=ORIENTED_EDGE('',*,*,#45013,.T.) ;
#60132=ORIENTED_EDGE('',*,*,#45014,.T.) ;
#60133=ORIENTED_EDGE('',*,*,#45015,.T.) ;
#60134=ORIENTED_EDGE('',*,*,#45016,.T.) ;
#60135=ORIENTED_EDGE('',*,*,#45017,.T.) ;
#60136=ORIENTED_EDGE('',*,*,#45018,.T.) ;
#60137=ORIENTED_EDGE('',*,*,#45019,.T.) ;
#60138=ORIENTED_EDGE('',*,*,#45020,.T.) ;
#60139=ORIENTED_EDGE('',*,*,#45021,.T.) ;
#60140=ORIENTED_EDGE('',*,*,#45022,.T.) ;
#60141=ORIENTED_EDGE('',*,*,#45023,.T.) ;
#60142=ORIENTED_EDGE('',*,*,#45024,.T.) ;
#60143=ORIENTED_EDGE('',*,*,#45025,.T.) ;
#60144=ORIENTED_EDGE('',*,*,#45026,.T.) ;
#60145=ORIENTED_EDGE('',*,*,#45027,.T.) ;
#60146=ORIENTED_EDGE('',*,*,#45028,.T.) ;
#60147=ORIENTED_EDGE('',*,*,#45029,.T.) ;
#60148=ORIENTED_EDGE('',*,*,#45030,.T.) ;
#60149=ORIENTED_EDGE('',*,*,#45031,.T.) ;
#60150=ORIENTED_EDGE('',*,*,#45032,.T.) ;
#60151=ORIENTED_EDGE('',*,*,#45033,.T.) ;
#60152=ORIENTED_EDGE('',*,*,#45034,.T.) ;
#60153=ORIENTED_EDGE('',*,*,#45035,.T.) ;
#60154=ORIENTED_EDGE('',*,*,#45036,.T.) ;
#60155=ORIENTED_EDGE('',*,*,#45037,.T.) ;
#60156=ORIENTED_EDGE('',*,*,#45038,.T.) ;
#60157=ORIENTED_EDGE('',*,*,#45039,.T.) ;
#60158=ORIENTED_EDGE('',*,*,#45040,.T.) ;
#60159=ORIENTED_EDGE('',*,*,#45041,.T.) ;
#60160=ORIENTED_EDGE('',*,*,#45042,.T.) ;
#60161=ORIENTED_EDGE('',*,*,#45043,.T.) ;
#60162=ORIENTED_EDGE('',*,*,#45044,.T.) ;
#60163=ORIENTED_EDGE('',*,*,#45045,.T.) ;
#60164=ORIENTED_EDGE('',*,*,#45046,.T.) ;
#60165=ORIENTED_EDGE('',*,*,#45047,.T.) ;
#60166=ORIENTED_EDGE('',*,*,#45048,.T.) ;
#60167=ORIENTED_EDGE('',*,*,#45049,.T.) ;
#60168=ORIENTED_EDGE('',*,*,#45050,.T.) ;
#60169=ORIENTED_EDGE('',*,*,#45051,.F.) ;
#60170=ORIENTED_EDGE('',*,*,#45052,.T.) ;
#60171=ORIENTED_EDGE('',*,*,#45053,.F.) ;
#60172=ORIENTED_EDGE('',*,*,#45054,.T.) ;
#60173=ORIENTED_EDGE('',*,*,#45055,.T.) ;
#60174=ORIENTED_EDGE('',*,*,#45056,.T.) ;
#60175=ORIENTED_EDGE('',*,*,#45057,.T.) ;
#60176=ORIENTED_EDGE('',*,*,#45058,.T.) ;
#60177=ORIENTED_EDGE('',*,*,#45059,.T.) ;
#60178=ORIENTED_EDGE('',*,*,#45060,.T.) ;
#60179=ORIENTED_EDGE('',*,*,#45061,.T.) ;
#60180=ORIENTED_EDGE('',*,*,#44388,.T.) ;
#60181=ORIENTED_EDGE('',*,*,#45062,.T.) ;
#60182=ORIENTED_EDGE('',*,*,#45063,.T.) ;
#60183=ORIENTED_EDGE('',*,*,#45064,.T.) ;
#60184=ORIENTED_EDGE('',*,*,#45065,.T.) ;
#60185=ORIENTED_EDGE('',*,*,#45066,.T.) ;
#60186=ORIENTED_EDGE('',*,*,#45067,.T.) ;
#60187=ORIENTED_EDGE('',*,*,#45068,.T.) ;
#60188=ORIENTED_EDGE('',*,*,#45069,.T.) ;
#60189=ORIENTED_EDGE('',*,*,#45070,.T.) ;
#60190=ORIENTED_EDGE('',*,*,#45071,.T.) ;
#60191=ORIENTED_EDGE('',*,*,#45072,.T.) ;
#60192=ORIENTED_EDGE('',*,*,#45073,.T.) ;
#60193=ORIENTED_EDGE('',*,*,#45074,.F.) ;
#60194=ORIENTED_EDGE('',*,*,#45075,.T.) ;
#60195=ORIENTED_EDGE('',*,*,#45076,.T.) ;
#60196=ORIENTED_EDGE('',*,*,#45077,.T.) ;
#60197=ORIENTED_EDGE('',*,*,#45076,.F.) ;
#60198=ORIENTED_EDGE('',*,*,#45078,.T.) ;
#60199=ORIENTED_EDGE('',*,*,#45079,.T.) ;
#60200=ORIENTED_EDGE('',*,*,#45080,.T.) ;
#60201=ORIENTED_EDGE('',*,*,#45079,.F.) ;
#60202=ORIENTED_EDGE('',*,*,#45081,.T.) ;
#60203=ORIENTED_EDGE('',*,*,#45082,.T.) ;
#60204=ORIENTED_EDGE('',*,*,#45083,.T.) ;
#60205=ORIENTED_EDGE('',*,*,#45082,.F.) ;
#60206=ORIENTED_EDGE('',*,*,#45084,.T.) ;
#60207=ORIENTED_EDGE('',*,*,#45085,.T.) ;
#60208=ORIENTED_EDGE('',*,*,#45086,.T.) ;
#60209=ORIENTED_EDGE('',*,*,#45085,.F.) ;
#60210=ORIENTED_EDGE('',*,*,#45087,.T.) ;
#60211=ORIENTED_EDGE('',*,*,#45088,.T.) ;
#60212=ORIENTED_EDGE('',*,*,#45089,.T.) ;
#60213=ORIENTED_EDGE('',*,*,#45088,.F.) ;
#60214=ORIENTED_EDGE('',*,*,#45090,.T.) ;
#60215=ORIENTED_EDGE('',*,*,#45091,.T.) ;
#60216=ORIENTED_EDGE('',*,*,#45092,.T.) ;
#60217=ORIENTED_EDGE('',*,*,#45091,.F.) ;
#60218=ORIENTED_EDGE('',*,*,#44383,.T.) ;
#60219=ORIENTED_EDGE('',*,*,#45093,.T.) ;
#60220=ORIENTED_EDGE('',*,*,#45094,.T.) ;
#60221=ORIENTED_EDGE('',*,*,#45093,.F.) ;
#60222=ORIENTED_EDGE('',*,*,#45095,.T.) ;
#60223=ORIENTED_EDGE('',*,*,#44396,.T.) ;
#60224=ORIENTED_EDGE('',*,*,#45096,.T.) ;
#60225=ORIENTED_EDGE('',*,*,#44395,.F.) ;
#60226=ORIENTED_EDGE('',*,*,#45097,.T.) ;
#60227=ORIENTED_EDGE('',*,*,#45098,.T.) ;
#60228=ORIENTED_EDGE('',*,*,#45099,.T.) ;
#60229=ORIENTED_EDGE('',*,*,#45098,.F.) ;
#60230=ORIENTED_EDGE('',*,*,#45100,.T.) ;
#60231=ORIENTED_EDGE('',*,*,#45101,.T.) ;
#60232=ORIENTED_EDGE('',*,*,#45102,.T.) ;
#60233=ORIENTED_EDGE('',*,*,#45101,.F.) ;
#60234=ORIENTED_EDGE('',*,*,#45103,.T.) ;
#60235=ORIENTED_EDGE('',*,*,#45104,.T.) ;
#60236=ORIENTED_EDGE('',*,*,#45105,.T.) ;
#60237=ORIENTED_EDGE('',*,*,#45104,.F.) ;
#60238=ORIENTED_EDGE('',*,*,#45106,.T.) ;
#60239=ORIENTED_EDGE('',*,*,#45107,.T.) ;
#60240=ORIENTED_EDGE('',*,*,#45108,.T.) ;
#60241=ORIENTED_EDGE('',*,*,#45107,.F.) ;
#60242=ORIENTED_EDGE('',*,*,#45109,.T.) ;
#60243=ORIENTED_EDGE('',*,*,#45110,.T.) ;
#60244=ORIENTED_EDGE('',*,*,#45111,.T.) ;
#60245=ORIENTED_EDGE('',*,*,#45110,.F.) ;
#60246=ORIENTED_EDGE('',*,*,#45112,.T.) ;
#60247=ORIENTED_EDGE('',*,*,#45113,.T.) ;
#60248=ORIENTED_EDGE('',*,*,#45114,.T.) ;
#60249=ORIENTED_EDGE('',*,*,#45113,.F.) ;
#60250=ORIENTED_EDGE('',*,*,#45115,.T.) ;
#60251=ORIENTED_EDGE('',*,*,#45116,.T.) ;
#60252=ORIENTED_EDGE('',*,*,#45117,.T.) ;
#60253=ORIENTED_EDGE('',*,*,#45116,.F.) ;
#60254=ORIENTED_EDGE('',*,*,#45118,.T.) ;
#60255=ORIENTED_EDGE('',*,*,#45119,.T.) ;
#60256=ORIENTED_EDGE('',*,*,#45120,.T.) ;
#60257=ORIENTED_EDGE('',*,*,#45119,.F.) ;
#60258=ORIENTED_EDGE('',*,*,#45121,.T.) ;
#60259=ORIENTED_EDGE('',*,*,#45122,.T.) ;
#60260=ORIENTED_EDGE('',*,*,#45123,.T.) ;
#60261=ORIENTED_EDGE('',*,*,#45122,.F.) ;
#60262=ORIENTED_EDGE('',*,*,#45124,.T.) ;
#60263=ORIENTED_EDGE('',*,*,#45125,.T.) ;
#60264=ORIENTED_EDGE('',*,*,#45126,.T.) ;
#60265=ORIENTED_EDGE('',*,*,#45125,.F.) ;
#60266=ORIENTED_EDGE('',*,*,#45127,.T.) ;
#60267=ORIENTED_EDGE('',*,*,#45128,.T.) ;
#60268=ORIENTED_EDGE('',*,*,#45129,.T.) ;
#60269=ORIENTED_EDGE('',*,*,#45128,.F.) ;
#60270=ORIENTED_EDGE('',*,*,#45130,.T.) ;
#60271=ORIENTED_EDGE('',*,*,#45131,.T.) ;
#60272=ORIENTED_EDGE('',*,*,#45132,.T.) ;
#60273=ORIENTED_EDGE('',*,*,#45131,.F.) ;
#60274=ORIENTED_EDGE('',*,*,#45133,.T.) ;
#60275=ORIENTED_EDGE('',*,*,#45134,.T.) ;
#60276=ORIENTED_EDGE('',*,*,#45135,.T.) ;
#60277=ORIENTED_EDGE('',*,*,#45134,.F.) ;
#60278=ORIENTED_EDGE('',*,*,#45136,.T.) ;
#60279=ORIENTED_EDGE('',*,*,#45137,.T.) ;
#60280=ORIENTED_EDGE('',*,*,#45138,.T.) ;
#60281=ORIENTED_EDGE('',*,*,#45137,.F.) ;
#60282=ORIENTED_EDGE('',*,*,#45139,.T.) ;
#60283=ORIENTED_EDGE('',*,*,#45140,.T.) ;
#60284=ORIENTED_EDGE('',*,*,#45141,.T.) ;
#60285=ORIENTED_EDGE('',*,*,#45140,.F.) ;
#60286=ORIENTED_EDGE('',*,*,#45142,.T.) ;
#60287=ORIENTED_EDGE('',*,*,#45143,.T.) ;
#60288=ORIENTED_EDGE('',*,*,#45144,.T.) ;
#60289=ORIENTED_EDGE('',*,*,#45143,.F.) ;
#60290=ORIENTED_EDGE('',*,*,#45145,.T.) ;
#60291=ORIENTED_EDGE('',*,*,#45146,.T.) ;
#60292=ORIENTED_EDGE('',*,*,#45147,.T.) ;
#60293=ORIENTED_EDGE('',*,*,#45146,.F.) ;
#60294=ORIENTED_EDGE('',*,*,#45148,.T.) ;
#60295=ORIENTED_EDGE('',*,*,#45149,.T.) ;
#60296=ORIENTED_EDGE('',*,*,#45150,.T.) ;
#60297=ORIENTED_EDGE('',*,*,#45149,.F.) ;
#60298=ORIENTED_EDGE('',*,*,#45151,.T.) ;
#60299=ORIENTED_EDGE('',*,*,#45074,.T.) ;
#60300=ORIENTED_EDGE('',*,*,#45152,.T.) ;
#60301=ORIENTED_EDGE('',*,*,#45153,.T.) ;
#60302=ORIENTED_EDGE('',*,*,#45154,.T.) ;
#60303=ORIENTED_EDGE('',*,*,#45155,.T.) ;
#60304=ORIENTED_EDGE('',*,*,#45156,.T.) ;
#60305=ORIENTED_EDGE('',*,*,#45157,.T.) ;
#60306=ORIENTED_EDGE('',*,*,#45158,.T.) ;
#60307=ORIENTED_EDGE('',*,*,#45159,.T.) ;
#60308=ORIENTED_EDGE('',*,*,#45160,.T.) ;
#60309=ORIENTED_EDGE('',*,*,#45161,.T.) ;
#60310=ORIENTED_EDGE('',*,*,#45162,.T.) ;
#60311=ORIENTED_EDGE('',*,*,#45163,.T.) ;
#60312=ORIENTED_EDGE('',*,*,#45164,.T.) ;
#60313=ORIENTED_EDGE('',*,*,#45165,.T.) ;
#60314=ORIENTED_EDGE('',*,*,#45166,.T.) ;
#60315=ORIENTED_EDGE('',*,*,#45167,.T.) ;
#60316=ORIENTED_EDGE('',*,*,#45168,.T.) ;
#60317=ORIENTED_EDGE('',*,*,#45169,.T.) ;
#60318=ORIENTED_EDGE('',*,*,#45170,.T.) ;
#60319=ORIENTED_EDGE('',*,*,#44380,.T.) ;
#60320=ORIENTED_EDGE('',*,*,#44372,.T.) ;
#60321=ORIENTED_EDGE('',*,*,#45171,.F.) ;
#60322=ORIENTED_EDGE('',*,*,#45172,.T.) ;
#60323=ORIENTED_EDGE('',*,*,#45173,.T.) ;
#60324=ORIENTED_EDGE('',*,*,#45174,.T.) ;
#60325=ORIENTED_EDGE('',*,*,#45175,.T.) ;
#60326=ORIENTED_EDGE('',*,*,#45176,.T.) ;
#60327=ORIENTED_EDGE('',*,*,#45177,.T.) ;
#60328=ORIENTED_EDGE('',*,*,#45178,.T.) ;
#60329=ORIENTED_EDGE('',*,*,#45179,.F.) ;
#60330=ORIENTED_EDGE('',*,*,#45067,.F.) ;
#60331=ORIENTED_EDGE('',*,*,#45180,.F.) ;
#60332=ORIENTED_EDGE('',*,*,#45054,.F.) ;
#60333=ORIENTED_EDGE('',*,*,#45181,.F.) ;
#60334=ORIENTED_EDGE('',*,*,#45068,.F.) ;
#60335=ORIENTED_EDGE('',*,*,#45182,.F.) ;
#60336=ORIENTED_EDGE('',*,*,#45062,.F.) ;
#60337=ORIENTED_EDGE('',*,*,#45183,.F.) ;
#60338=ORIENTED_EDGE('',*,*,#45181,.T.) ;
#60339=ORIENTED_EDGE('',*,*,#45184,.F.) ;
#60340=ORIENTED_EDGE('',*,*,#45185,.F.) ;
#60341=ORIENTED_EDGE('',*,*,#45180,.T.) ;
#60342=ORIENTED_EDGE('',*,*,#45186,.F.) ;
#60343=ORIENTED_EDGE('',*,*,#45179,.T.) ;
#60344=ORIENTED_EDGE('',*,*,#45053,.T.) ;
#60345=ORIENTED_EDGE('',*,*,#45187,.F.) ;
#60346=ORIENTED_EDGE('',*,*,#45182,.T.) ;
#60347=ORIENTED_EDGE('',*,*,#45184,.T.) ;
#60348=ORIENTED_EDGE('',*,*,#45065,.F.) ;
#60349=ORIENTED_EDGE('',*,*,#45188,.F.) ;
#60350=ORIENTED_EDGE('',*,*,#44386,.T.) ;
#60351=ORIENTED_EDGE('',*,*,#45189,.T.) ;
#60352=ORIENTED_EDGE('',*,*,#45190,.F.) ;
#60353=ORIENTED_EDGE('',*,*,#45183,.T.) ;
#60354=ORIENTED_EDGE('',*,*,#45191,.F.) ;
#60355=ORIENTED_EDGE('',*,*,#45192,.T.) ;
#60356=ORIENTED_EDGE('',*,*,#45193,.F.) ;
#60357=ORIENTED_EDGE('',*,*,#44622,.F.) ;
#60358=ORIENTED_EDGE('',*,*,#45194,.F.) ;
#60359=ORIENTED_EDGE('',*,*,#45069,.F.) ;
#60360=ORIENTED_EDGE('',*,*,#45186,.T.) ;
#60361=ORIENTED_EDGE('',*,*,#45066,.F.) ;
#60362=ORIENTED_EDGE('',*,*,#45195,.F.) ;
#60363=ORIENTED_EDGE('',*,*,#45072,.F.) ;
#60364=ORIENTED_EDGE('',*,*,#45185,.T.) ;
#60365=ORIENTED_EDGE('',*,*,#45071,.F.) ;
#60366=ORIENTED_EDGE('',*,*,#45196,.F.) ;
#60367=ORIENTED_EDGE('',*,*,#45045,.F.) ;
#60368=ORIENTED_EDGE('',*,*,#45187,.T.) ;
#60369=ORIENTED_EDGE('',*,*,#45052,.F.) ;
#60370=ORIENTED_EDGE('',*,*,#45197,.F.) ;
#60371=ORIENTED_EDGE('',*,*,#45063,.F.) ;
#60372=ORIENTED_EDGE('',*,*,#45198,.F.) ;
#60373=ORIENTED_EDGE('',*,*,#45064,.F.) ;
#60374=ORIENTED_EDGE('',*,*,#45199,.F.) ;
#60375=ORIENTED_EDGE('',*,*,#45059,.F.) ;
#60376=ORIENTED_EDGE('',*,*,#45188,.T.) ;
#60377=ORIENTED_EDGE('',*,*,#45198,.T.) ;
#60378=ORIENTED_EDGE('',*,*,#44387,.F.) ;
#60379=ORIENTED_EDGE('',*,*,#45194,.T.) ;
#60380=ORIENTED_EDGE('',*,*,#44632,.T.) ;
#60381=ORIENTED_EDGE('',*,*,#45200,.F.) ;
#60382=ORIENTED_EDGE('',*,*,#45195,.T.) ;
#60383=ORIENTED_EDGE('',*,*,#45201,.F.) ;
#60384=ORIENTED_EDGE('',*,*,#45196,.T.) ;
#60385=ORIENTED_EDGE('',*,*,#45202,.F.) ;
#60386=ORIENTED_EDGE('',*,*,#44638,.T.) ;
#60387=ORIENTED_EDGE('',*,*,#45197,.T.) ;
#60388=ORIENTED_EDGE('',*,*,#45051,.T.) ;
#60389=ORIENTED_EDGE('',*,*,#45203,.F.) ;
#60390=ORIENTED_EDGE('',*,*,#45199,.T.) ;
#60391=ORIENTED_EDGE('',*,*,#45200,.T.) ;
#60392=ORIENTED_EDGE('',*,*,#44631,.F.) ;
#60393=ORIENTED_EDGE('',*,*,#45204,.F.) ;
#60394=ORIENTED_EDGE('',*,*,#45073,.F.) ;
#60395=ORIENTED_EDGE('',*,*,#45202,.T.) ;
#60396=ORIENTED_EDGE('',*,*,#45070,.F.) ;
#60397=ORIENTED_EDGE('',*,*,#45205,.F.) ;
#60398=ORIENTED_EDGE('',*,*,#44639,.F.) ;
#60399=ORIENTED_EDGE('',*,*,#45046,.F.) ;
#60400=ORIENTED_EDGE('',*,*,#45201,.T.) ;
#60401=ORIENTED_EDGE('',*,*,#45206,.F.) ;
#60402=ORIENTED_EDGE('',*,*,#45207,.F.) ;
#60403=ORIENTED_EDGE('',*,*,#45203,.T.) ;
#60404=ORIENTED_EDGE('',*,*,#45050,.F.) ;
#60405=ORIENTED_EDGE('',*,*,#45208,.F.) ;
#60406=ORIENTED_EDGE('',*,*,#45060,.F.) ;
#60407=ORIENTED_EDGE('',*,*,#45209,.F.) ;
#60408=ORIENTED_EDGE('',*,*,#45061,.F.) ;
#60409=ORIENTED_EDGE('',*,*,#45210,.F.) ;
#60410=ORIENTED_EDGE('',*,*,#45055,.F.) ;
#60411=ORIENTED_EDGE('',*,*,#44389,.T.) ;
#60412=ORIENTED_EDGE('',*,*,#45209,.T.) ;
#60413=ORIENTED_EDGE('',*,*,#45211,.F.) ;
#60414=ORIENTED_EDGE('',*,*,#44626,.T.) ;
#60415=ORIENTED_EDGE('',*,*,#45205,.T.) ;
#60416=ORIENTED_EDGE('',*,*,#45204,.T.) ;
#60417=ORIENTED_EDGE('',*,*,#45212,.F.) ;
#60418=ORIENTED_EDGE('',*,*,#45213,.F.) ;
#60419=ORIENTED_EDGE('',*,*,#44644,.F.) ;
#60420=ORIENTED_EDGE('',*,*,#45214,.F.) ;
#60421=ORIENTED_EDGE('',*,*,#45215,.F.) ;
#60422=ORIENTED_EDGE('',*,*,#45206,.T.) ;
#60423=ORIENTED_EDGE('',*,*,#44642,.F.) ;
#60424=ORIENTED_EDGE('',*,*,#45214,.T.) ;
#60425=ORIENTED_EDGE('',*,*,#44753,.F.) ;
#60426=ORIENTED_EDGE('',*,*,#45207,.T.) ;
#60427=ORIENTED_EDGE('',*,*,#45216,.F.) ;
#60428=ORIENTED_EDGE('',*,*,#45217,.F.) ;
#60429=ORIENTED_EDGE('',*,*,#45210,.T.) ;
#60430=ORIENTED_EDGE('',*,*,#45208,.T.) ;
#60431=ORIENTED_EDGE('',*,*,#45218,.F.) ;
#60432=ORIENTED_EDGE('',*,*,#45211,.T.) ;
#60433=ORIENTED_EDGE('',*,*,#45058,.F.) ;
#60434=ORIENTED_EDGE('',*,*,#45219,.F.) ;
#60435=ORIENTED_EDGE('',*,*,#44627,.F.) ;
#60436=ORIENTED_EDGE('',*,*,#45212,.T.) ;
#60437=ORIENTED_EDGE('',*,*,#44630,.F.) ;
#60438=ORIENTED_EDGE('',*,*,#45220,.F.) ;
#60439=ORIENTED_EDGE('',*,*,#44640,.F.) ;
#60440=ORIENTED_EDGE('',*,*,#45213,.T.) ;
#60441=ORIENTED_EDGE('',*,*,#44641,.F.) ;
#60442=ORIENTED_EDGE('',*,*,#45221,.F.) ;
#60443=ORIENTED_EDGE('',*,*,#44656,.F.) ;
#60444=ORIENTED_EDGE('',*,*,#45215,.T.) ;
#60445=ORIENTED_EDGE('',*,*,#44752,.T.) ;
#60446=ORIENTED_EDGE('',*,*,#45222,.F.) ;
#60447=ORIENTED_EDGE('',*,*,#45216,.T.) ;
#60448=ORIENTED_EDGE('',*,*,#45047,.F.) ;
#60449=ORIENTED_EDGE('',*,*,#45217,.T.) ;
#60450=ORIENTED_EDGE('',*,*,#45223,.F.) ;
#60451=ORIENTED_EDGE('',*,*,#45224,.F.) ;
#60452=ORIENTED_EDGE('',*,*,#45218,.T.) ;
#60453=ORIENTED_EDGE('',*,*,#45049,.F.) ;
#60454=ORIENTED_EDGE('',*,*,#45225,.F.) ;
#60455=ORIENTED_EDGE('',*,*,#45056,.F.) ;
#60456=ORIENTED_EDGE('',*,*,#45226,.F.) ;
#60457=ORIENTED_EDGE('',*,*,#45057,.F.) ;
#60458=ORIENTED_EDGE('',*,*,#45227,.F.) ;
#60459=ORIENTED_EDGE('',*,*,#44637,.F.) ;
#60460=ORIENTED_EDGE('',*,*,#45219,.T.) ;
#60461=ORIENTED_EDGE('',*,*,#45226,.T.) ;
#60462=ORIENTED_EDGE('',*,*,#45228,.F.) ;
#60463=ORIENTED_EDGE('',*,*,#45221,.T.) ;
#60464=ORIENTED_EDGE('',*,*,#45220,.T.) ;
#60465=ORIENTED_EDGE('',*,*,#45229,.F.) ;
#60466=ORIENTED_EDGE('',*,*,#44657,.T.) ;
#60467=ORIENTED_EDGE('',*,*,#45230,.F.) ;
#60468=ORIENTED_EDGE('',*,*,#45223,.T.) ;
#60469=ORIENTED_EDGE('',*,*,#45222,.T.) ;
#60470=ORIENTED_EDGE('',*,*,#44751,.F.) ;
#60471=ORIENTED_EDGE('',*,*,#45224,.T.) ;
#60472=ORIENTED_EDGE('',*,*,#45231,.F.) ;
#60473=ORIENTED_EDGE('',*,*,#45232,.F.) ;
#60474=ORIENTED_EDGE('',*,*,#45227,.T.) ;
#60475=ORIENTED_EDGE('',*,*,#45225,.T.) ;
#60476=ORIENTED_EDGE('',*,*,#45233,.F.) ;
#60477=ORIENTED_EDGE('',*,*,#44633,.T.) ;
#60478=ORIENTED_EDGE('',*,*,#45228,.T.) ;
#60479=ORIENTED_EDGE('',*,*,#44636,.F.) ;
#60480=ORIENTED_EDGE('',*,*,#45234,.F.) ;
#60481=ORIENTED_EDGE('',*,*,#44628,.F.) ;
#60482=ORIENTED_EDGE('',*,*,#45229,.T.) ;
#60483=ORIENTED_EDGE('',*,*,#44629,.F.) ;
#60484=ORIENTED_EDGE('',*,*,#45235,.F.) ;
#60485=ORIENTED_EDGE('',*,*,#44658,.F.) ;
#60486=ORIENTED_EDGE('',*,*,#45230,.T.) ;
#60487=ORIENTED_EDGE('',*,*,#44750,.T.) ;
#60488=ORIENTED_EDGE('',*,*,#45236,.F.) ;
#60489=ORIENTED_EDGE('',*,*,#45231,.T.) ;
#60490=ORIENTED_EDGE('',*,*,#45048,.F.) ;
#60491=ORIENTED_EDGE('',*,*,#45232,.T.) ;
#60492=ORIENTED_EDGE('',*,*,#45237,.F.) ;
#60493=ORIENTED_EDGE('',*,*,#45233,.T.) ;
#60494=ORIENTED_EDGE('',*,*,#45235,.T.) ;
#60495=ORIENTED_EDGE('',*,*,#45234,.T.) ;
#60496=ORIENTED_EDGE('',*,*,#45238,.F.) ;
#60497=ORIENTED_EDGE('',*,*,#44659,.T.) ;
#60498=ORIENTED_EDGE('',*,*,#45236,.T.) ;
#60499=ORIENTED_EDGE('',*,*,#44749,.F.) ;
#60500=ORIENTED_EDGE('',*,*,#45239,.F.) ;
#60501=ORIENTED_EDGE('',*,*,#44634,.F.) ;
#60502=ORIENTED_EDGE('',*,*,#45237,.T.) ;
#60503=ORIENTED_EDGE('',*,*,#45238,.T.) ;
#60504=ORIENTED_EDGE('',*,*,#44635,.F.) ;
#60505=ORIENTED_EDGE('',*,*,#45240,.F.) ;
#60506=ORIENTED_EDGE('',*,*,#44660,.F.) ;
#60507=ORIENTED_EDGE('',*,*,#45239,.T.) ;
#60508=ORIENTED_EDGE('',*,*,#44589,.F.) ;
#60509=ORIENTED_EDGE('',*,*,#45240,.T.) ;
#60510=ORIENTED_EDGE('',*,*,#45241,.F.) ;
#60511=ORIENTED_EDGE('',*,*,#45242,.F.) ;
#60512=ORIENTED_EDGE('',*,*,#44773,.F.) ;
#60513=ORIENTED_EDGE('',*,*,#45242,.T.) ;
#60514=ORIENTED_EDGE('',*,*,#45030,.F.) ;
#60515=ORIENTED_EDGE('',*,*,#45243,.F.) ;
#60516=ORIENTED_EDGE('',*,*,#44770,.F.) ;
#60517=ORIENTED_EDGE('',*,*,#45241,.T.) ;
#60518=ORIENTED_EDGE('',*,*,#44776,.F.) ;
#60519=ORIENTED_EDGE('',*,*,#45244,.F.) ;
#60520=ORIENTED_EDGE('',*,*,#45031,.F.) ;
#60521=ORIENTED_EDGE('',*,*,#45243,.T.) ;
#60522=ORIENTED_EDGE('',*,*,#45029,.F.) ;
#60523=ORIENTED_EDGE('',*,*,#45245,.F.) ;
#60524=ORIENTED_EDGE('',*,*,#44767,.F.) ;
#60525=ORIENTED_EDGE('',*,*,#45244,.T.) ;
#60526=ORIENTED_EDGE('',*,*,#44779,.F.) ;
#60527=ORIENTED_EDGE('',*,*,#45246,.F.) ;
#60528=ORIENTED_EDGE('',*,*,#45245,.T.) ;
#60529=ORIENTED_EDGE('',*,*,#45028,.F.) ;
#60530=ORIENTED_EDGE('',*,*,#45247,.F.) ;
#60531=ORIENTED_EDGE('',*,*,#44764,.F.) ;
#60532=ORIENTED_EDGE('',*,*,#45246,.T.) ;
#60533=ORIENTED_EDGE('',*,*,#44782,.F.) ;
#60534=ORIENTED_EDGE('',*,*,#45248,.F.) ;
#60535=ORIENTED_EDGE('',*,*,#45032,.F.) ;
#60536=ORIENTED_EDGE('',*,*,#44761,.F.) ;
#60537=ORIENTED_EDGE('',*,*,#45247,.T.) ;
#60538=ORIENTED_EDGE('',*,*,#45249,.F.) ;
#60539=ORIENTED_EDGE('',*,*,#45248,.T.) ;
#60540=ORIENTED_EDGE('',*,*,#44785,.F.) ;
#60541=ORIENTED_EDGE('',*,*,#45250,.F.) ;
#60542=ORIENTED_EDGE('',*,*,#45033,.F.) ;
#60543=ORIENTED_EDGE('',*,*,#45249,.T.) ;
#60544=ORIENTED_EDGE('',*,*,#45027,.F.) ;
#60545=ORIENTED_EDGE('',*,*,#45251,.F.) ;
#60546=ORIENTED_EDGE('',*,*,#44756,.F.) ;
#60547=ORIENTED_EDGE('',*,*,#45250,.T.) ;
#60548=ORIENTED_EDGE('',*,*,#44788,.F.) ;
#60549=ORIENTED_EDGE('',*,*,#45252,.F.) ;
#60550=ORIENTED_EDGE('',*,*,#45034,.F.) ;
#60551=ORIENTED_EDGE('',*,*,#44706,.F.) ;
#60552=ORIENTED_EDGE('',*,*,#45251,.T.) ;
#60553=ORIENTED_EDGE('',*,*,#45253,.F.) ;
#60554=ORIENTED_EDGE('',*,*,#45252,.T.) ;
#60555=ORIENTED_EDGE('',*,*,#44791,.F.) ;
#60556=ORIENTED_EDGE('',*,*,#45254,.F.) ;
#60557=ORIENTED_EDGE('',*,*,#45253,.T.) ;
#60558=ORIENTED_EDGE('',*,*,#45026,.F.) ;
#60559=ORIENTED_EDGE('',*,*,#45255,.F.) ;
#60560=ORIENTED_EDGE('',*,*,#44654,.F.) ;
#60561=ORIENTED_EDGE('',*,*,#45254,.T.) ;
#60562=ORIENTED_EDGE('',*,*,#44793,.F.) ;
#60563=ORIENTED_EDGE('',*,*,#45256,.F.) ;
#60564=ORIENTED_EDGE('',*,*,#45025,.F.) ;
#60565=ORIENTED_EDGE('',*,*,#44648,.F.) ;
#60566=ORIENTED_EDGE('',*,*,#45255,.T.) ;
#60567=ORIENTED_EDGE('',*,*,#45256,.T.) ;
#60568=ORIENTED_EDGE('',*,*,#45257,.F.) ;
#60569=ORIENTED_EDGE('',*,*,#44774,.F.) ;
#60570=ORIENTED_EDGE('',*,*,#45258,.F.) ;
#60571=ORIENTED_EDGE('',*,*,#45258,.T.) ;
#60572=ORIENTED_EDGE('',*,*,#44771,.F.) ;
#60573=ORIENTED_EDGE('',*,*,#45259,.F.) ;
#60574=ORIENTED_EDGE('',*,*,#45042,.F.) ;
#60575=ORIENTED_EDGE('',*,*,#45257,.T.) ;
#60576=ORIENTED_EDGE('',*,*,#45041,.F.) ;
#60577=ORIENTED_EDGE('',*,*,#45260,.F.) ;
#60578=ORIENTED_EDGE('',*,*,#44777,.F.) ;
#60579=ORIENTED_EDGE('',*,*,#45259,.T.) ;
#60580=ORIENTED_EDGE('',*,*,#44768,.F.) ;
#60581=ORIENTED_EDGE('',*,*,#45261,.F.) ;
#60582=ORIENTED_EDGE('',*,*,#45043,.F.) ;
#60583=ORIENTED_EDGE('',*,*,#44780,.F.) ;
#60584=ORIENTED_EDGE('',*,*,#45260,.T.) ;
#60585=ORIENTED_EDGE('',*,*,#45262,.F.) ;
#60586=ORIENTED_EDGE('',*,*,#45261,.T.) ;
#60587=ORIENTED_EDGE('',*,*,#44765,.F.) ;
#60588=ORIENTED_EDGE('',*,*,#45263,.F.) ;
#60589=ORIENTED_EDGE('',*,*,#45044,.F.) ;
#60590=ORIENTED_EDGE('',*,*,#45262,.T.) ;
#60591=ORIENTED_EDGE('',*,*,#45040,.F.) ;
#60592=ORIENTED_EDGE('',*,*,#45264,.F.) ;
#60593=ORIENTED_EDGE('',*,*,#44783,.F.) ;
#60594=ORIENTED_EDGE('',*,*,#45263,.T.) ;
#60595=ORIENTED_EDGE('',*,*,#44762,.F.) ;
#60596=ORIENTED_EDGE('',*,*,#45265,.F.) ;
#60597=ORIENTED_EDGE('',*,*,#45264,.T.) ;
#60598=ORIENTED_EDGE('',*,*,#45039,.F.) ;
#60599=ORIENTED_EDGE('',*,*,#45266,.F.) ;
#60600=ORIENTED_EDGE('',*,*,#44786,.F.) ;
#60601=ORIENTED_EDGE('',*,*,#45265,.T.) ;
#60602=ORIENTED_EDGE('',*,*,#44754,.F.) ;
#60603=ORIENTED_EDGE('',*,*,#45267,.F.) ;
#60604=ORIENTED_EDGE('',*,*,#45035,.F.) ;
#60605=ORIENTED_EDGE('',*,*,#45266,.T.) ;
#60606=ORIENTED_EDGE('',*,*,#45038,.F.) ;
#60607=ORIENTED_EDGE('',*,*,#45268,.F.) ;
#60608=ORIENTED_EDGE('',*,*,#44789,.F.) ;
#60609=ORIENTED_EDGE('',*,*,#45267,.T.) ;
#60610=ORIENTED_EDGE('',*,*,#44646,.F.) ;
#60611=ORIENTED_EDGE('',*,*,#45269,.F.) ;
#60612=ORIENTED_EDGE('',*,*,#44792,.F.) ;
#60613=ORIENTED_EDGE('',*,*,#45268,.T.) ;
#60614=ORIENTED_EDGE('',*,*,#45270,.F.) ;
#60615=ORIENTED_EDGE('',*,*,#45269,.T.) ;
#60616=ORIENTED_EDGE('',*,*,#44655,.F.) ;
#60617=ORIENTED_EDGE('',*,*,#45271,.F.) ;
#60618=ORIENTED_EDGE('',*,*,#45036,.F.) ;
#60619=ORIENTED_EDGE('',*,*,#45270,.T.) ;
#60620=ORIENTED_EDGE('',*,*,#45037,.F.) ;
#60621=ORIENTED_EDGE('',*,*,#45272,.F.) ;
#60622=ORIENTED_EDGE('',*,*,#44794,.F.) ;
#60623=ORIENTED_EDGE('',*,*,#45271,.T.) ;
#60624=ORIENTED_EDGE('',*,*,#44650,.F.) ;
#60625=ORIENTED_EDGE('',*,*,#45272,.T.) ;
#60626=ORIENTED_EDGE('',*,*,#45273,.F.) ;
#60627=ORIENTED_EDGE('',*,*,#45115,.F.) ;
#60628=ORIENTED_EDGE('',*,*,#45274,.F.) ;
#60629=ORIENTED_EDGE('',*,*,#45162,.F.) ;
#60630=ORIENTED_EDGE('',*,*,#45274,.T.) ;
#60631=ORIENTED_EDGE('',*,*,#45112,.F.) ;
#60632=ORIENTED_EDGE('',*,*,#45275,.F.) ;
#60633=ORIENTED_EDGE('',*,*,#45163,.F.) ;
#60634=ORIENTED_EDGE('',*,*,#45118,.F.) ;
#60635=ORIENTED_EDGE('',*,*,#45273,.T.) ;
#60636=ORIENTED_EDGE('',*,*,#45276,.F.) ;
#60637=ORIENTED_EDGE('',*,*,#45275,.T.) ;
#60638=ORIENTED_EDGE('',*,*,#45109,.F.) ;
#60639=ORIENTED_EDGE('',*,*,#45277,.F.) ;
#60640=ORIENTED_EDGE('',*,*,#45164,.F.) ;
#60641=ORIENTED_EDGE('',*,*,#45276,.T.) ;
#60642=ORIENTED_EDGE('',*,*,#45161,.F.) ;
#60643=ORIENTED_EDGE('',*,*,#45278,.F.) ;
#60644=ORIENTED_EDGE('',*,*,#45121,.F.) ;
#60645=ORIENTED_EDGE('',*,*,#45277,.T.) ;
#60646=ORIENTED_EDGE('',*,*,#45106,.F.) ;
#60647=ORIENTED_EDGE('',*,*,#45279,.F.) ;
#60648=ORIENTED_EDGE('',*,*,#45165,.F.) ;
#60649=ORIENTED_EDGE('',*,*,#45124,.F.) ;
#60650=ORIENTED_EDGE('',*,*,#45278,.T.) ;
#60651=ORIENTED_EDGE('',*,*,#45280,.F.) ;
#60652=ORIENTED_EDGE('',*,*,#45279,.T.) ;
#60653=ORIENTED_EDGE('',*,*,#45103,.F.) ;
#60654=ORIENTED_EDGE('',*,*,#45281,.F.) ;
#60655=ORIENTED_EDGE('',*,*,#45166,.F.) ;
#60656=ORIENTED_EDGE('',*,*,#45280,.T.) ;
#60657=ORIENTED_EDGE('',*,*,#45160,.F.) ;
#60658=ORIENTED_EDGE('',*,*,#45282,.F.) ;
#60659=ORIENTED_EDGE('',*,*,#45127,.F.) ;
#60660=ORIENTED_EDGE('',*,*,#45281,.T.) ;
#60661=ORIENTED_EDGE('',*,*,#45100,.F.) ;
#60662=ORIENTED_EDGE('',*,*,#45283,.F.) ;
#60663=ORIENTED_EDGE('',*,*,#45130,.F.) ;
#60664=ORIENTED_EDGE('',*,*,#45282,.T.) ;
#60665=ORIENTED_EDGE('',*,*,#45284,.F.) ;
#60666=ORIENTED_EDGE('',*,*,#45283,.T.) ;
#60667=ORIENTED_EDGE('',*,*,#45097,.F.) ;
#60668=ORIENTED_EDGE('',*,*,#45285,.F.) ;
#60669=ORIENTED_EDGE('',*,*,#45167,.F.) ;
#60670=ORIENTED_EDGE('',*,*,#45284,.T.) ;
#60671=ORIENTED_EDGE('',*,*,#45159,.F.) ;
#60672=ORIENTED_EDGE('',*,*,#45286,.F.) ;
#60673=ORIENTED_EDGE('',*,*,#45133,.F.) ;
#60674=ORIENTED_EDGE('',*,*,#45285,.T.) ;
#60675=ORIENTED_EDGE('',*,*,#44394,.F.) ;
#60676=ORIENTED_EDGE('',*,*,#45287,.F.) ;
#60677=ORIENTED_EDGE('',*,*,#45136,.F.) ;
#60678=ORIENTED_EDGE('',*,*,#45286,.T.) ;
#60679=ORIENTED_EDGE('',*,*,#45288,.F.) ;
#60680=ORIENTED_EDGE('',*,*,#45287,.T.) ;
#60681=ORIENTED_EDGE('',*,*,#45095,.F.) ;
#60682=ORIENTED_EDGE('',*,*,#44385,.F.) ;
#60683=ORIENTED_EDGE('',*,*,#45168,.F.) ;
#60684=ORIENTED_EDGE('',*,*,#45288,.T.) ;
#60685=ORIENTED_EDGE('',*,*,#45158,.F.) ;
#60686=ORIENTED_EDGE('',*,*,#45289,.F.) ;
#60687=ORIENTED_EDGE('',*,*,#45139,.F.) ;
#60688=ORIENTED_EDGE('',*,*,#45142,.F.) ;
#60689=ORIENTED_EDGE('',*,*,#45289,.T.) ;
#60690=ORIENTED_EDGE('',*,*,#45290,.F.) ;
#60691=ORIENTED_EDGE('',*,*,#44384,.T.) ;
#60692=ORIENTED_EDGE('',*,*,#45090,.F.) ;
#60693=ORIENTED_EDGE('',*,*,#45291,.F.) ;
#60694=ORIENTED_EDGE('',*,*,#45169,.F.) ;
#60695=ORIENTED_EDGE('',*,*,#45290,.T.) ;
#60696=ORIENTED_EDGE('',*,*,#45157,.F.) ;
#60697=ORIENTED_EDGE('',*,*,#45292,.F.) ;
#60698=ORIENTED_EDGE('',*,*,#45145,.F.) ;
#60699=ORIENTED_EDGE('',*,*,#45291,.T.) ;
#60700=ORIENTED_EDGE('',*,*,#45087,.F.) ;
#60701=ORIENTED_EDGE('',*,*,#45293,.F.) ;
#60702=ORIENTED_EDGE('',*,*,#45148,.F.) ;
#60703=ORIENTED_EDGE('',*,*,#45292,.T.) ;
#60704=ORIENTED_EDGE('',*,*,#45294,.F.) ;
#60705=ORIENTED_EDGE('',*,*,#45293,.T.) ;
#60706=ORIENTED_EDGE('',*,*,#45084,.F.) ;
#60707=ORIENTED_EDGE('',*,*,#45295,.F.) ;
#60708=ORIENTED_EDGE('',*,*,#45170,.F.) ;
#60709=ORIENTED_EDGE('',*,*,#45294,.T.) ;
#60710=ORIENTED_EDGE('',*,*,#45156,.F.) ;
#60711=ORIENTED_EDGE('',*,*,#45296,.F.) ;
#60712=ORIENTED_EDGE('',*,*,#45151,.F.) ;
#60713=ORIENTED_EDGE('',*,*,#45295,.T.) ;
#60714=ORIENTED_EDGE('',*,*,#45081,.F.) ;
#60715=ORIENTED_EDGE('',*,*,#45297,.F.) ;
#60716=ORIENTED_EDGE('',*,*,#45153,.F.) ;
#60717=ORIENTED_EDGE('',*,*,#45296,.T.) ;
#60718=ORIENTED_EDGE('',*,*,#45155,.F.) ;
#60719=ORIENTED_EDGE('',*,*,#45298,.F.) ;
#60720=ORIENTED_EDGE('',*,*,#45075,.F.) ;
#60721=ORIENTED_EDGE('',*,*,#45297,.T.) ;
#60722=ORIENTED_EDGE('',*,*,#45078,.F.) ;
#60723=ORIENTED_EDGE('',*,*,#45298,.T.) ;
#60724=ORIENTED_EDGE('',*,*,#45154,.F.) ;
#60725=ORIENTED_EDGE('',*,*,#45299,.F.) ;
#60726=ORIENTED_EDGE('',*,*,#45111,.F.) ;
#60727=ORIENTED_EDGE('',*,*,#45300,.F.) ;
#60728=ORIENTED_EDGE('',*,*,#45013,.F.) ;
#60729=ORIENTED_EDGE('',*,*,#45108,.F.) ;
#60730=ORIENTED_EDGE('',*,*,#45299,.T.) ;
#60731=ORIENTED_EDGE('',*,*,#45301,.F.) ;
#60732=ORIENTED_EDGE('',*,*,#45300,.T.) ;
#60733=ORIENTED_EDGE('',*,*,#45114,.F.) ;
#60734=ORIENTED_EDGE('',*,*,#45302,.F.) ;
#60735=ORIENTED_EDGE('',*,*,#45301,.T.) ;
#60736=ORIENTED_EDGE('',*,*,#45012,.F.) ;
#60737=ORIENTED_EDGE('',*,*,#45303,.F.) ;
#60738=ORIENTED_EDGE('',*,*,#45105,.F.) ;
#60739=ORIENTED_EDGE('',*,*,#45302,.T.) ;
#60740=ORIENTED_EDGE('',*,*,#45117,.F.) ;
#60741=ORIENTED_EDGE('',*,*,#45304,.F.) ;
#60742=ORIENTED_EDGE('',*,*,#45014,.F.) ;
#60743=ORIENTED_EDGE('',*,*,#45303,.T.) ;
#60744=ORIENTED_EDGE('',*,*,#45011,.F.) ;
#60745=ORIENTED_EDGE('',*,*,#45305,.F.) ;
#60746=ORIENTED_EDGE('',*,*,#45102,.F.) ;
#60747=ORIENTED_EDGE('',*,*,#45304,.T.) ;
#60748=ORIENTED_EDGE('',*,*,#45120,.F.) ;
#60749=ORIENTED_EDGE('',*,*,#45306,.F.) ;
#60750=ORIENTED_EDGE('',*,*,#45015,.F.) ;
#60751=ORIENTED_EDGE('',*,*,#45305,.T.) ;
#60752=ORIENTED_EDGE('',*,*,#45010,.F.) ;
#60753=ORIENTED_EDGE('',*,*,#44379,.F.) ;
#60754=ORIENTED_EDGE('',*,*,#45099,.F.) ;
#60755=ORIENTED_EDGE('',*,*,#45306,.T.) ;
#60756=ORIENTED_EDGE('',*,*,#45123,.F.) ;
#60757=ORIENTED_EDGE('',*,*,#45307,.F.) ;
#60758=ORIENTED_EDGE('',*,*,#45016,.F.) ;
#60759=ORIENTED_EDGE('',*,*,#45307,.T.) ;
#60760=ORIENTED_EDGE('',*,*,#45126,.F.) ;
#60761=ORIENTED_EDGE('',*,*,#45308,.F.) ;
#60762=ORIENTED_EDGE('',*,*,#45017,.F.) ;
#60763=ORIENTED_EDGE('',*,*,#44377,.T.) ;
#60764=ORIENTED_EDGE('',*,*,#45009,.F.) ;
#60765=ORIENTED_EDGE('',*,*,#45309,.F.) ;
#60766=ORIENTED_EDGE('',*,*,#45096,.F.) ;
#60767=ORIENTED_EDGE('',*,*,#45308,.T.) ;
#60768=ORIENTED_EDGE('',*,*,#45129,.F.) ;
#60769=ORIENTED_EDGE('',*,*,#45310,.F.) ;
#60770=ORIENTED_EDGE('',*,*,#45018,.F.) ;
#60771=ORIENTED_EDGE('',*,*,#45309,.T.) ;
#60772=ORIENTED_EDGE('',*,*,#45008,.F.) ;
#60773=ORIENTED_EDGE('',*,*,#45311,.F.) ;
#60774=ORIENTED_EDGE('',*,*,#45094,.F.) ;
#60775=ORIENTED_EDGE('',*,*,#45310,.T.) ;
#60776=ORIENTED_EDGE('',*,*,#45132,.F.) ;
#60777=ORIENTED_EDGE('',*,*,#45312,.F.) ;
#60778=ORIENTED_EDGE('',*,*,#45019,.F.) ;
#60779=ORIENTED_EDGE('',*,*,#45311,.T.) ;
#60780=ORIENTED_EDGE('',*,*,#45007,.F.) ;
#60781=ORIENTED_EDGE('',*,*,#45313,.F.) ;
#60782=ORIENTED_EDGE('',*,*,#45092,.F.) ;
#60783=ORIENTED_EDGE('',*,*,#45312,.T.) ;
#60784=ORIENTED_EDGE('',*,*,#45135,.F.) ;
#60785=ORIENTED_EDGE('',*,*,#45314,.F.) ;
#60786=ORIENTED_EDGE('',*,*,#45020,.F.) ;
#60787=ORIENTED_EDGE('',*,*,#45313,.T.) ;
#60788=ORIENTED_EDGE('',*,*,#45006,.F.) ;
#60789=ORIENTED_EDGE('',*,*,#45315,.F.) ;
#60790=ORIENTED_EDGE('',*,*,#45089,.F.) ;
#60791=ORIENTED_EDGE('',*,*,#45314,.T.) ;
#60792=ORIENTED_EDGE('',*,*,#45138,.F.) ;
#60793=ORIENTED_EDGE('',*,*,#45316,.F.) ;
#60794=ORIENTED_EDGE('',*,*,#45021,.F.) ;
#60795=ORIENTED_EDGE('',*,*,#45315,.T.) ;
#60796=ORIENTED_EDGE('',*,*,#45005,.F.) ;
#60797=ORIENTED_EDGE('',*,*,#45317,.F.) ;
#60798=ORIENTED_EDGE('',*,*,#45086,.F.) ;
#60799=ORIENTED_EDGE('',*,*,#45316,.T.) ;
#60800=ORIENTED_EDGE('',*,*,#45141,.F.) ;
#60801=ORIENTED_EDGE('',*,*,#45318,.F.) ;
#60802=ORIENTED_EDGE('',*,*,#45022,.F.) ;
#60803=ORIENTED_EDGE('',*,*,#45083,.F.) ;
#60804=ORIENTED_EDGE('',*,*,#45317,.T.) ;
#60805=ORIENTED_EDGE('',*,*,#45319,.F.) ;
#60806=ORIENTED_EDGE('',*,*,#45318,.T.) ;
#60807=ORIENTED_EDGE('',*,*,#45144,.F.) ;
#60808=ORIENTED_EDGE('',*,*,#45320,.F.) ;
#60809=ORIENTED_EDGE('',*,*,#45023,.F.) ;
#60810=ORIENTED_EDGE('',*,*,#45319,.T.) ;
#60811=ORIENTED_EDGE('',*,*,#45004,.F.) ;
#60812=ORIENTED_EDGE('',*,*,#45321,.F.) ;
#60813=ORIENTED_EDGE('',*,*,#45080,.F.) ;
#60814=ORIENTED_EDGE('',*,*,#45320,.T.) ;
#60815=ORIENTED_EDGE('',*,*,#45147,.F.) ;
#60816=ORIENTED_EDGE('',*,*,#45322,.F.) ;
#60817=ORIENTED_EDGE('',*,*,#45024,.F.) ;
#60818=ORIENTED_EDGE('',*,*,#45077,.F.) ;
#60819=ORIENTED_EDGE('',*,*,#45321,.T.) ;
#60820=ORIENTED_EDGE('',*,*,#45323,.F.) ;
#60821=ORIENTED_EDGE('',*,*,#45322,.T.) ;
#60822=ORIENTED_EDGE('',*,*,#45150,.F.) ;
#60823=ORIENTED_EDGE('',*,*,#45324,.F.) ;
#60824=ORIENTED_EDGE('',*,*,#45002,.F.) ;
#60825=ORIENTED_EDGE('',*,*,#45323,.T.) ;
#60826=ORIENTED_EDGE('',*,*,#45003,.F.) ;
#60827=ORIENTED_EDGE('',*,*,#45324,.T.) ;
#60828=ORIENTED_EDGE('',*,*,#45152,.F.) ;
#60829=ORIENTED_EDGE('',*,*,#45325,.T.) ;
#60830=ORIENTED_EDGE('',*,*,#45326,.T.) ;
#60831=ORIENTED_EDGE('',*,*,#45327,.T.) ;
#60832=ORIENTED_EDGE('',*,*,#45328,.T.) ;
#60833=ORIENTED_EDGE('',*,*,#45329,.T.) ;
#60834=ORIENTED_EDGE('',*,*,#45330,.T.) ;
#60835=ORIENTED_EDGE('',*,*,#45331,.T.) ;
#60836=ORIENTED_EDGE('',*,*,#45332,.T.) ;
#60837=ORIENTED_EDGE('',*,*,#45333,.T.) ;
#60838=ORIENTED_EDGE('',*,*,#45334,.T.) ;
#60839=ORIENTED_EDGE('',*,*,#45335,.T.) ;
#60840=ORIENTED_EDGE('',*,*,#45336,.T.) ;
#60841=ORIENTED_EDGE('',*,*,#45337,.T.) ;
#60842=ORIENTED_EDGE('',*,*,#45338,.T.) ;
#60843=ORIENTED_EDGE('',*,*,#45339,.T.) ;
#60844=ORIENTED_EDGE('',*,*,#45340,.T.) ;
#60845=ORIENTED_EDGE('',*,*,#45341,.T.) ;
#60846=ORIENTED_EDGE('',*,*,#45342,.T.) ;
#60847=ORIENTED_EDGE('',*,*,#45343,.F.) ;
#60848=ORIENTED_EDGE('',*,*,#45344,.T.) ;
#60849=ORIENTED_EDGE('',*,*,#45345,.T.) ;
#60850=ORIENTED_EDGE('',*,*,#45346,.T.) ;
#60851=ORIENTED_EDGE('',*,*,#45193,.T.) ;
#60852=ORIENTED_EDGE('',*,*,#45347,.T.) ;
#60853=ORIENTED_EDGE('',*,*,#45348,.T.) ;
#60854=ORIENTED_EDGE('',*,*,#45349,.T.) ;
#60855=ORIENTED_EDGE('',*,*,#45350,.T.) ;
#60856=ORIENTED_EDGE('',*,*,#45351,.T.) ;
#60857=ORIENTED_EDGE('',*,*,#44391,.T.) ;
#60858=ORIENTED_EDGE('',*,*,#45352,.T.) ;
#60859=ORIENTED_EDGE('',*,*,#45353,.T.) ;
#60860=ORIENTED_EDGE('',*,*,#45354,.T.) ;
#60861=ORIENTED_EDGE('',*,*,#45190,.T.) ;
#60862=ORIENTED_EDGE('',*,*,#45355,.T.) ;
#60863=ORIENTED_EDGE('',*,*,#45325,.F.) ;
#60864=ORIENTED_EDGE('',*,*,#45356,.T.) ;
#60865=ORIENTED_EDGE('',*,*,#45191,.T.) ;
#60866=ORIENTED_EDGE('',*,*,#45343,.T.) ;
#60867=ORIENTED_EDGE('',*,*,#45357,.T.) ;
#60868=ORIENTED_EDGE('',*,*,#44624,.F.) ;
#60869=ORIENTED_EDGE('',*,*,#45358,.T.) ;
#60870=ORIENTED_EDGE('',*,*,#45359,.T.) ;
#60871=ORIENTED_EDGE('',*,*,#45360,.T.) ;
#60872=ORIENTED_EDGE('',*,*,#45361,.T.) ;
#60873=ORIENTED_EDGE('',*,*,#45362,.T.) ;
#60874=ORIENTED_EDGE('',*,*,#45363,.T.) ;
#60875=ORIENTED_EDGE('',*,*,#45364,.T.) ;
#60876=ORIENTED_EDGE('',*,*,#45173,.F.) ;
#60877=ORIENTED_EDGE('',*,*,#45365,.T.) ;
#60878=ORIENTED_EDGE('',*,*,#45177,.F.) ;
#60879=ORIENTED_EDGE('',*,*,#45366,.T.) ;
#60880=ORIENTED_EDGE('',*,*,#45367,.T.) ;
#60881=ORIENTED_EDGE('',*,*,#45368,.T.) ;
#60882=ORIENTED_EDGE('',*,*,#45369,.T.) ;
#60883=ORIENTED_EDGE('',*,*,#45370,.T.) ;
#60884=ORIENTED_EDGE('',*,*,#45371,.T.) ;
#60885=ORIENTED_EDGE('',*,*,#45372,.T.) ;
#60886=ORIENTED_EDGE('',*,*,#45373,.T.) ;
#60887=ORIENTED_EDGE('',*,*,#45374,.T.) ;
#60888=ORIENTED_EDGE('',*,*,#45375,.T.) ;
#60889=ORIENTED_EDGE('',*,*,#45376,.T.) ;
#60890=ORIENTED_EDGE('',*,*,#45377,.T.) ;
#60891=ORIENTED_EDGE('',*,*,#45378,.T.) ;
#60892=ORIENTED_EDGE('',*,*,#45171,.T.) ;
#60893=ORIENTED_EDGE('',*,*,#45379,.T.) ;
#60894=ORIENTED_EDGE('',*,*,#45175,.F.) ;
#60895=ORIENTED_EDGE('',*,*,#45380,.T.) ;
#60896=ORIENTED_EDGE('',*,*,#45381,.T.) ;
#60897=ORIENTED_EDGE('',*,*,#45382,.T.) ;
#60898=ORIENTED_EDGE('',*,*,#45383,.T.) ;
#60899=ORIENTED_EDGE('',*,*,#45384,.T.) ;
#60900=ORIENTED_EDGE('',*,*,#45385,.T.) ;
#60901=ORIENTED_EDGE('',*,*,#45386,.T.) ;
#60902=ORIENTED_EDGE('',*,*,#45387,.T.) ;
#60903=ORIENTED_EDGE('',*,*,#45388,.T.) ;
#60904=ORIENTED_EDGE('',*,*,#45389,.T.) ;
#60905=ORIENTED_EDGE('',*,*,#45390,.T.) ;
#60906=ORIENTED_EDGE('',*,*,#45391,.T.) ;
#60907=ORIENTED_EDGE('',*,*,#45392,.T.) ;
#60908=ORIENTED_EDGE('',*,*,#45393,.T.) ;
#60909=ORIENTED_EDGE('',*,*,#45394,.T.) ;
#60910=ORIENTED_EDGE('',*,*,#45395,.T.) ;
#60911=ORIENTED_EDGE('',*,*,#45396,.T.) ;
#60912=ORIENTED_EDGE('',*,*,#45397,.T.) ;
#60913=ORIENTED_EDGE('',*,*,#45398,.T.) ;
#60914=ORIENTED_EDGE('',*,*,#45385,.F.) ;
#60915=ORIENTED_EDGE('',*,*,#45399,.T.) ;
#60916=ORIENTED_EDGE('',*,*,#45340,.F.) ;
#60917=ORIENTED_EDGE('',*,*,#45400,.F.) ;
#60918=ORIENTED_EDGE('',*,*,#45337,.F.) ;
#60919=ORIENTED_EDGE('',*,*,#45401,.T.) ;
#60920=ORIENTED_EDGE('',*,*,#45341,.F.) ;
#60921=ORIENTED_EDGE('',*,*,#45402,.T.) ;
#60922=ORIENTED_EDGE('',*,*,#45403,.F.) ;
#60923=ORIENTED_EDGE('',*,*,#45400,.T.) ;
#60924=ORIENTED_EDGE('',*,*,#45404,.F.) ;
#60925=ORIENTED_EDGE('',*,*,#45338,.F.) ;
#60926=ORIENTED_EDGE('',*,*,#45405,.T.) ;
#60927=ORIENTED_EDGE('',*,*,#45387,.F.) ;
#60928=ORIENTED_EDGE('',*,*,#45406,.F.) ;
#60929=ORIENTED_EDGE('',*,*,#45404,.T.) ;
#60930=ORIENTED_EDGE('',*,*,#45339,.F.) ;
#60931=ORIENTED_EDGE('',*,*,#45407,.F.) ;
#60932=ORIENTED_EDGE('',*,*,#45333,.F.) ;
#60933=ORIENTED_EDGE('',*,*,#45403,.T.) ;
#60934=ORIENTED_EDGE('',*,*,#45336,.F.) ;
#60935=ORIENTED_EDGE('',*,*,#45408,.F.) ;
#60936=ORIENTED_EDGE('',*,*,#45386,.F.) ;
#60937=ORIENTED_EDGE('',*,*,#45407,.T.) ;
#60938=ORIENTED_EDGE('',*,*,#45406,.T.) ;
#60939=ORIENTED_EDGE('',*,*,#45409,.F.) ;
#60940=ORIENTED_EDGE('',*,*,#45410,.F.) ;
#60941=ORIENTED_EDGE('',*,*,#45408,.T.) ;
#60942=ORIENTED_EDGE('',*,*,#45411,.F.) ;
#60943=ORIENTED_EDGE('',*,*,#45409,.T.) ;
#60944=ORIENTED_EDGE('',*,*,#45390,.F.) ;
#60945=ORIENTED_EDGE('',*,*,#45412,.F.) ;
#60946=ORIENTED_EDGE('',*,*,#45334,.F.) ;
#60947=ORIENTED_EDGE('',*,*,#45411,.T.) ;
#60948=ORIENTED_EDGE('',*,*,#45335,.F.) ;
#60949=ORIENTED_EDGE('',*,*,#45413,.F.) ;
#60950=ORIENTED_EDGE('',*,*,#45329,.F.) ;
#60951=ORIENTED_EDGE('',*,*,#45332,.F.) ;
#60952=ORIENTED_EDGE('',*,*,#45414,.T.) ;
#60953=ORIENTED_EDGE('',*,*,#45383,.F.) ;
#60954=ORIENTED_EDGE('',*,*,#45410,.T.) ;
#60955=ORIENTED_EDGE('',*,*,#45413,.T.) ;
#60956=ORIENTED_EDGE('',*,*,#45412,.T.) ;
#60957=ORIENTED_EDGE('',*,*,#45415,.F.) ;
#60958=ORIENTED_EDGE('',*,*,#45327,.F.) ;
#60959=ORIENTED_EDGE('',*,*,#45416,.T.) ;
#60960=ORIENTED_EDGE('',*,*,#45331,.F.) ;
#60961=ORIENTED_EDGE('',*,*,#45417,.T.) ;
#60962=ORIENTED_EDGE('',*,*,#45389,.F.) ;
#60963=ORIENTED_EDGE('',*,*,#45418,.T.) ;
#60964=ORIENTED_EDGE('',*,*,#45330,.F.) ;
#60965=ORIENTED_EDGE('',*,*,#45415,.T.) ;
#60966=ORIENTED_EDGE('',*,*,#45393,.F.) ;
#60967=ORIENTED_EDGE('',*,*,#45419,.T.) ;
#60968=ORIENTED_EDGE('',*,*,#45362,.F.) ;
#60969=ORIENTED_EDGE('',*,*,#45420,.F.) ;
#60970=ORIENTED_EDGE('',*,*,#45359,.F.) ;
#60971=ORIENTED_EDGE('',*,*,#45421,.T.) ;
#60972=ORIENTED_EDGE('',*,*,#45363,.F.) ;
#60973=ORIENTED_EDGE('',*,*,#45422,.T.) ;
#60974=ORIENTED_EDGE('',*,*,#45423,.F.) ;
#60975=ORIENTED_EDGE('',*,*,#45420,.T.) ;
#60976=ORIENTED_EDGE('',*,*,#45424,.F.) ;
#60977=ORIENTED_EDGE('',*,*,#45360,.F.) ;
#60978=ORIENTED_EDGE('',*,*,#45425,.T.) ;
#60979=ORIENTED_EDGE('',*,*,#45395,.F.) ;
#60980=ORIENTED_EDGE('',*,*,#45426,.F.) ;
#60981=ORIENTED_EDGE('',*,*,#45424,.T.) ;
#60982=ORIENTED_EDGE('',*,*,#45361,.F.) ;
#60983=ORIENTED_EDGE('',*,*,#45427,.F.) ;
#60984=ORIENTED_EDGE('',*,*,#45375,.F.) ;
#60985=ORIENTED_EDGE('',*,*,#45423,.T.) ;
#60986=ORIENTED_EDGE('',*,*,#45374,.F.) ;
#60987=ORIENTED_EDGE('',*,*,#45428,.F.) ;
#60988=ORIENTED_EDGE('',*,*,#45394,.F.) ;
#60989=ORIENTED_EDGE('',*,*,#45427,.T.) ;
#60990=ORIENTED_EDGE('',*,*,#45426,.T.) ;
#60991=ORIENTED_EDGE('',*,*,#45429,.F.) ;
#60992=ORIENTED_EDGE('',*,*,#45430,.F.) ;
#60993=ORIENTED_EDGE('',*,*,#45428,.T.) ;
#60994=ORIENTED_EDGE('',*,*,#45431,.F.) ;
#60995=ORIENTED_EDGE('',*,*,#45429,.T.) ;
#60996=ORIENTED_EDGE('',*,*,#45398,.F.) ;
#60997=ORIENTED_EDGE('',*,*,#45432,.F.) ;
#60998=ORIENTED_EDGE('',*,*,#45376,.F.) ;
#60999=ORIENTED_EDGE('',*,*,#45431,.T.) ;
#61000=ORIENTED_EDGE('',*,*,#45373,.F.) ;
#61001=ORIENTED_EDGE('',*,*,#45433,.F.) ;
#61002=ORIENTED_EDGE('',*,*,#45369,.F.) ;
#61003=ORIENTED_EDGE('',*,*,#45372,.F.) ;
#61004=ORIENTED_EDGE('',*,*,#45434,.T.) ;
#61005=ORIENTED_EDGE('',*,*,#45391,.F.) ;
#61006=ORIENTED_EDGE('',*,*,#45430,.T.) ;
#61007=ORIENTED_EDGE('',*,*,#45433,.T.) ;
#61008=ORIENTED_EDGE('',*,*,#45432,.T.) ;
#61009=ORIENTED_EDGE('',*,*,#45435,.F.) ;
#61010=ORIENTED_EDGE('',*,*,#45367,.F.) ;
#61011=ORIENTED_EDGE('',*,*,#45436,.T.) ;
#61012=ORIENTED_EDGE('',*,*,#45371,.F.) ;
#61013=ORIENTED_EDGE('',*,*,#45437,.T.) ;
#61014=ORIENTED_EDGE('',*,*,#45397,.F.) ;
#61015=ORIENTED_EDGE('',*,*,#45438,.T.) ;
#61016=ORIENTED_EDGE('',*,*,#45370,.F.) ;
#61017=ORIENTED_EDGE('',*,*,#45435,.T.) ;
#61018=ORIENTED_EDGE('',*,*,#44625,.F.) ;
#61019=ORIENTED_EDGE('',*,*,#45357,.F.) ;
#61020=ORIENTED_EDGE('',*,*,#45439,.F.) ;
#61021=ORIENTED_EDGE('',*,*,#45352,.F.) ;
#61022=ORIENTED_EDGE('',*,*,#45439,.T.) ;
#61023=ORIENTED_EDGE('',*,*,#45342,.F.) ;
#61024=ORIENTED_EDGE('',*,*,#45440,.F.) ;
#61025=ORIENTED_EDGE('',*,*,#45353,.F.) ;
#61026=ORIENTED_EDGE('',*,*,#45440,.T.) ;
#61027=ORIENTED_EDGE('',*,*,#45401,.F.) ;
#61028=ORIENTED_EDGE('',*,*,#45399,.F.) ;
#61029=ORIENTED_EDGE('',*,*,#45441,.F.) ;
#61030=ORIENTED_EDGE('',*,*,#45441,.T.) ;
#61031=ORIENTED_EDGE('',*,*,#45384,.F.) ;
#61032=ORIENTED_EDGE('',*,*,#45442,.F.) ;
#61033=ORIENTED_EDGE('',*,*,#45354,.F.) ;
#61034=ORIENTED_EDGE('',*,*,#45442,.T.) ;
#61035=ORIENTED_EDGE('',*,*,#45414,.F.) ;
#61036=ORIENTED_EDGE('',*,*,#45416,.F.) ;
#61037=ORIENTED_EDGE('',*,*,#45443,.F.) ;
#61038=ORIENTED_EDGE('',*,*,#45443,.T.) ;
#61039=ORIENTED_EDGE('',*,*,#45326,.F.) ;
#61040=ORIENTED_EDGE('',*,*,#45444,.F.) ;
#61041=ORIENTED_EDGE('',*,*,#45350,.F.) ;
#61042=ORIENTED_EDGE('',*,*,#44392,.F.) ;
#61043=ORIENTED_EDGE('',*,*,#45351,.F.) ;
#61044=ORIENTED_EDGE('',*,*,#45444,.T.) ;
#61045=ORIENTED_EDGE('',*,*,#45355,.F.) ;
#61046=ORIENTED_EDGE('',*,*,#45189,.F.) ;
#61047=ORIENTED_EDGE('',*,*,#45192,.F.) ;
#61048=ORIENTED_EDGE('',*,*,#45356,.F.) ;
#61049=ORIENTED_EDGE('',*,*,#45445,.F.) ;
#61050=ORIENTED_EDGE('',*,*,#45347,.F.) ;
#61051=ORIENTED_EDGE('',*,*,#45445,.T.) ;
#61052=ORIENTED_EDGE('',*,*,#45328,.F.) ;
#61053=ORIENTED_EDGE('',*,*,#45446,.F.) ;
#61054=ORIENTED_EDGE('',*,*,#45348,.F.) ;
#61055=ORIENTED_EDGE('',*,*,#45446,.T.) ;
#61056=ORIENTED_EDGE('',*,*,#45417,.F.) ;
#61057=ORIENTED_EDGE('',*,*,#45418,.F.) ;
#61058=ORIENTED_EDGE('',*,*,#45447,.F.) ;
#61059=ORIENTED_EDGE('',*,*,#45447,.T.) ;
#61060=ORIENTED_EDGE('',*,*,#45388,.F.) ;
#61061=ORIENTED_EDGE('',*,*,#45448,.F.) ;
#61062=ORIENTED_EDGE('',*,*,#45349,.F.) ;
#61063=ORIENTED_EDGE('',*,*,#45448,.T.) ;
#61064=ORIENTED_EDGE('',*,*,#45405,.F.) ;
#61065=ORIENTED_EDGE('',*,*,#45402,.F.) ;
#61066=ORIENTED_EDGE('',*,*,#45449,.F.) ;
#61067=ORIENTED_EDGE('',*,*,#45449,.T.) ;
#61068=ORIENTED_EDGE('',*,*,#45344,.F.) ;
#61069=ORIENTED_EDGE('',*,*,#45450,.F.) ;
#61070=ORIENTED_EDGE('',*,*,#45345,.F.) ;
#61071=ORIENTED_EDGE('',*,*,#45450,.T.) ;
#61072=ORIENTED_EDGE('',*,*,#45358,.F.) ;
#61073=ORIENTED_EDGE('',*,*,#44623,.F.) ;
#61074=ORIENTED_EDGE('',*,*,#45346,.F.) ;
#61075=ORIENTED_EDGE('',*,*,#45174,.F.) ;
#61076=ORIENTED_EDGE('',*,*,#45364,.F.) ;
#61077=ORIENTED_EDGE('',*,*,#45451,.F.) ;
#61078=ORIENTED_EDGE('',*,*,#45380,.F.) ;
#61079=ORIENTED_EDGE('',*,*,#45451,.T.) ;
#61080=ORIENTED_EDGE('',*,*,#45421,.F.) ;
#61081=ORIENTED_EDGE('',*,*,#45419,.F.) ;
#61082=ORIENTED_EDGE('',*,*,#45452,.F.) ;
#61083=ORIENTED_EDGE('',*,*,#45452,.T.) ;
#61084=ORIENTED_EDGE('',*,*,#45392,.F.) ;
#61085=ORIENTED_EDGE('',*,*,#45453,.F.) ;
#61086=ORIENTED_EDGE('',*,*,#45381,.F.) ;
#61087=ORIENTED_EDGE('',*,*,#45453,.T.) ;
#61088=ORIENTED_EDGE('',*,*,#45434,.F.) ;
#61089=ORIENTED_EDGE('',*,*,#45436,.F.) ;
#61090=ORIENTED_EDGE('',*,*,#45454,.F.) ;
#61091=ORIENTED_EDGE('',*,*,#45176,.F.) ;
#61092=ORIENTED_EDGE('',*,*,#45382,.F.) ;
#61093=ORIENTED_EDGE('',*,*,#45454,.T.) ;
#61094=ORIENTED_EDGE('',*,*,#45366,.F.) ;
#61095=ORIENTED_EDGE('',*,*,#45455,.F.) ;
#61096=ORIENTED_EDGE('',*,*,#45365,.F.) ;
#61097=ORIENTED_EDGE('',*,*,#45172,.F.) ;
#61098=ORIENTED_EDGE('',*,*,#45378,.F.) ;
#61099=ORIENTED_EDGE('',*,*,#45422,.F.) ;
#61100=ORIENTED_EDGE('',*,*,#45455,.T.) ;
#61101=ORIENTED_EDGE('',*,*,#45456,.F.) ;
#61102=ORIENTED_EDGE('',*,*,#45425,.F.) ;
#61103=ORIENTED_EDGE('',*,*,#45456,.T.) ;
#61104=ORIENTED_EDGE('',*,*,#45377,.F.) ;
#61105=ORIENTED_EDGE('',*,*,#45457,.F.) ;
#61106=ORIENTED_EDGE('',*,*,#45396,.F.) ;
#61107=ORIENTED_EDGE('',*,*,#45178,.F.) ;
#61108=ORIENTED_EDGE('',*,*,#45368,.F.) ;
#61109=ORIENTED_EDGE('',*,*,#45458,.F.) ;
#61110=ORIENTED_EDGE('',*,*,#45379,.F.) ;
#61111=ORIENTED_EDGE('',*,*,#45438,.F.) ;
#61112=ORIENTED_EDGE('',*,*,#45457,.T.) ;
#61113=ORIENTED_EDGE('',*,*,#45458,.T.) ;
#61114=ORIENTED_EDGE('',*,*,#45437,.F.) ;
#61115=ORIENTED_EDGE('',*,*,#45459,.T.) ;
#61116=ORIENTED_EDGE('',*,*,#45460,.T.) ;
#61117=ORIENTED_EDGE('',*,*,#45461,.T.) ;
#61118=ORIENTED_EDGE('',*,*,#45462,.T.) ;
#61119=ORIENTED_EDGE('',*,*,#45463,.T.) ;
#61120=ORIENTED_EDGE('',*,*,#45464,.T.) ;
#61121=ORIENTED_EDGE('',*,*,#45465,.F.) ;
#61122=ORIENTED_EDGE('',*,*,#45466,.T.) ;
#61123=ORIENTED_EDGE('',*,*,#45467,.F.) ;
#61124=ORIENTED_EDGE('',*,*,#45468,.T.) ;
#61125=ORIENTED_EDGE('',*,*,#45469,.T.) ;
#61126=ORIENTED_EDGE('',*,*,#45470,.T.) ;
#61127=ORIENTED_EDGE('',*,*,#45471,.T.) ;
#61128=ORIENTED_EDGE('',*,*,#45472,.T.) ;
#61129=ORIENTED_EDGE('',*,*,#45473,.T.) ;
#61130=ORIENTED_EDGE('',*,*,#45474,.T.) ;
#61131=ORIENTED_EDGE('',*,*,#45475,.F.) ;
#61132=ORIENTED_EDGE('',*,*,#45476,.T.) ;
#61133=ORIENTED_EDGE('',*,*,#45477,.F.) ;
#61134=ORIENTED_EDGE('',*,*,#45478,.T.) ;
#61135=ORIENTED_EDGE('',*,*,#45479,.T.) ;
#61136=ORIENTED_EDGE('',*,*,#45480,.T.) ;
#61137=ORIENTED_EDGE('',*,*,#45481,.T.) ;
#61138=ORIENTED_EDGE('',*,*,#45482,.T.) ;
#61139=ORIENTED_EDGE('',*,*,#45483,.T.) ;
#61140=ORIENTED_EDGE('',*,*,#45484,.T.) ;
#61141=ORIENTED_EDGE('',*,*,#45485,.F.) ;
#61142=ORIENTED_EDGE('',*,*,#45486,.T.) ;
#61143=ORIENTED_EDGE('',*,*,#45487,.F.) ;
#61144=ORIENTED_EDGE('',*,*,#45488,.T.) ;
#61145=ORIENTED_EDGE('',*,*,#45489,.T.) ;
#61146=ORIENTED_EDGE('',*,*,#45490,.T.) ;
#61147=ORIENTED_EDGE('',*,*,#45491,.T.) ;
#61148=ORIENTED_EDGE('',*,*,#45492,.T.) ;
#61149=ORIENTED_EDGE('',*,*,#45493,.T.) ;
#61150=ORIENTED_EDGE('',*,*,#45494,.T.) ;
#61151=ORIENTED_EDGE('',*,*,#45495,.F.) ;
#61152=ORIENTED_EDGE('',*,*,#45496,.T.) ;
#61153=ORIENTED_EDGE('',*,*,#45497,.F.) ;
#61154=ORIENTED_EDGE('',*,*,#45498,.T.) ;
#61155=ORIENTED_EDGE('',*,*,#45499,.T.) ;
#61156=ORIENTED_EDGE('',*,*,#45500,.T.) ;
#61157=ORIENTED_EDGE('',*,*,#45501,.T.) ;
#61158=ORIENTED_EDGE('',*,*,#45502,.T.) ;
#61159=ORIENTED_EDGE('',*,*,#45503,.T.) ;
#61160=ORIENTED_EDGE('',*,*,#45504,.T.) ;
#61161=ORIENTED_EDGE('',*,*,#45505,.F.) ;
#61162=ORIENTED_EDGE('',*,*,#45506,.T.) ;
#61163=ORIENTED_EDGE('',*,*,#45507,.F.) ;
#61164=ORIENTED_EDGE('',*,*,#45508,.T.) ;
#61165=ORIENTED_EDGE('',*,*,#45509,.T.) ;
#61166=ORIENTED_EDGE('',*,*,#45510,.T.) ;
#61167=ORIENTED_EDGE('',*,*,#45511,.T.) ;
#61168=ORIENTED_EDGE('',*,*,#45512,.T.) ;
#61169=ORIENTED_EDGE('',*,*,#45513,.T.) ;
#61170=ORIENTED_EDGE('',*,*,#45514,.T.) ;
#61171=ORIENTED_EDGE('',*,*,#45515,.F.) ;
#61172=ORIENTED_EDGE('',*,*,#45516,.T.) ;
#61173=ORIENTED_EDGE('',*,*,#45517,.F.) ;
#61174=ORIENTED_EDGE('',*,*,#45518,.T.) ;
#61175=ORIENTED_EDGE('',*,*,#45519,.T.) ;
#61176=ORIENTED_EDGE('',*,*,#45520,.T.) ;
#61177=ORIENTED_EDGE('',*,*,#45521,.T.) ;
#61178=ORIENTED_EDGE('',*,*,#45522,.T.) ;
#61179=ORIENTED_EDGE('',*,*,#45523,.T.) ;
#61180=ORIENTED_EDGE('',*,*,#45524,.T.) ;
#61181=ORIENTED_EDGE('',*,*,#45525,.F.) ;
#61182=ORIENTED_EDGE('',*,*,#45526,.T.) ;
#61183=ORIENTED_EDGE('',*,*,#45527,.F.) ;
#61184=ORIENTED_EDGE('',*,*,#45528,.T.) ;
#61185=ORIENTED_EDGE('',*,*,#45529,.T.) ;
#61186=ORIENTED_EDGE('',*,*,#45530,.T.) ;
#61187=ORIENTED_EDGE('',*,*,#45531,.T.) ;
#61188=ORIENTED_EDGE('',*,*,#45532,.T.) ;
#61189=ORIENTED_EDGE('',*,*,#45533,.T.) ;
#61190=ORIENTED_EDGE('',*,*,#45534,.T.) ;
#61191=ORIENTED_EDGE('',*,*,#45535,.F.) ;
#61192=ORIENTED_EDGE('',*,*,#45536,.T.) ;
#61193=ORIENTED_EDGE('',*,*,#45537,.F.) ;
#61194=ORIENTED_EDGE('',*,*,#45538,.T.) ;
#61195=ORIENTED_EDGE('',*,*,#45539,.T.) ;
#61196=ORIENTED_EDGE('',*,*,#45540,.T.) ;
#61197=ORIENTED_EDGE('',*,*,#45541,.T.) ;
#61198=ORIENTED_EDGE('',*,*,#45542,.T.) ;
#61199=ORIENTED_EDGE('',*,*,#45543,.T.) ;
#61200=ORIENTED_EDGE('',*,*,#45544,.T.) ;
#61201=ORIENTED_EDGE('',*,*,#45545,.F.) ;
#61202=ORIENTED_EDGE('',*,*,#45546,.T.) ;
#61203=ORIENTED_EDGE('',*,*,#45547,.F.) ;
#61204=ORIENTED_EDGE('',*,*,#45548,.T.) ;
#61205=ORIENTED_EDGE('',*,*,#45549,.T.) ;
#61206=ORIENTED_EDGE('',*,*,#45550,.T.) ;
#61207=ORIENTED_EDGE('',*,*,#45551,.T.) ;
#61208=ORIENTED_EDGE('',*,*,#45552,.T.) ;
#61209=ORIENTED_EDGE('',*,*,#45553,.T.) ;
#61210=ORIENTED_EDGE('',*,*,#45554,.T.) ;
#61211=ORIENTED_EDGE('',*,*,#45555,.T.) ;
#61212=ORIENTED_EDGE('',*,*,#44331,.T.) ;
#61213=ORIENTED_EDGE('',*,*,#45556,.T.) ;
#61214=ORIENTED_EDGE('',*,*,#45557,.T.) ;
#61215=ORIENTED_EDGE('',*,*,#45558,.T.) ;
#61216=ORIENTED_EDGE('',*,*,#45559,.T.) ;
#61217=ORIENTED_EDGE('',*,*,#45560,.T.) ;
#61218=ORIENTED_EDGE('',*,*,#45561,.T.) ;
#61219=ORIENTED_EDGE('',*,*,#45562,.T.) ;
#61220=ORIENTED_EDGE('',*,*,#45563,.T.) ;
#61221=ORIENTED_EDGE('',*,*,#45564,.T.) ;
#61222=ORIENTED_EDGE('',*,*,#45565,.T.) ;
#61223=ORIENTED_EDGE('',*,*,#45566,.T.) ;
#61224=ORIENTED_EDGE('',*,*,#45567,.T.) ;
#61225=ORIENTED_EDGE('',*,*,#45568,.T.) ;
#61226=ORIENTED_EDGE('',*,*,#45569,.T.) ;
#61227=ORIENTED_EDGE('',*,*,#45570,.T.) ;
#61228=ORIENTED_EDGE('',*,*,#45571,.T.) ;
#61229=ORIENTED_EDGE('',*,*,#45572,.T.) ;
#61230=ORIENTED_EDGE('',*,*,#45573,.T.) ;
#61231=ORIENTED_EDGE('',*,*,#45574,.T.) ;
#61232=ORIENTED_EDGE('',*,*,#44278,.T.) ;
#61233=ORIENTED_EDGE('',*,*,#45575,.T.) ;
#61234=ORIENTED_EDGE('',*,*,#45576,.T.) ;
#61235=ORIENTED_EDGE('',*,*,#45577,.T.) ;
#61236=ORIENTED_EDGE('',*,*,#45578,.T.) ;
#61237=ORIENTED_EDGE('',*,*,#45579,.T.) ;
#61238=ORIENTED_EDGE('',*,*,#45580,.T.) ;
#61239=ORIENTED_EDGE('',*,*,#45581,.T.) ;
#61240=ORIENTED_EDGE('',*,*,#45582,.T.) ;
#61241=ORIENTED_EDGE('',*,*,#45583,.T.) ;
#61242=ORIENTED_EDGE('',*,*,#45584,.T.) ;
#61243=ORIENTED_EDGE('',*,*,#45585,.T.) ;
#61244=ORIENTED_EDGE('',*,*,#45586,.T.) ;
#61245=ORIENTED_EDGE('',*,*,#45587,.T.) ;
#61246=ORIENTED_EDGE('',*,*,#45588,.T.) ;
#61247=ORIENTED_EDGE('',*,*,#45589,.T.) ;
#61248=ORIENTED_EDGE('',*,*,#45590,.T.) ;
#61249=ORIENTED_EDGE('',*,*,#45591,.T.) ;
#61250=ORIENTED_EDGE('',*,*,#45592,.T.) ;
#61251=ORIENTED_EDGE('',*,*,#45593,.T.) ;
#61252=ORIENTED_EDGE('',*,*,#44261,.T.) ;
#61253=ORIENTED_EDGE('',*,*,#45594,.T.) ;
#61254=ORIENTED_EDGE('',*,*,#45595,.T.) ;
#61255=ORIENTED_EDGE('',*,*,#45596,.T.) ;
#61256=ORIENTED_EDGE('',*,*,#45597,.T.) ;
#61257=ORIENTED_EDGE('',*,*,#45598,.T.) ;
#61258=ORIENTED_EDGE('',*,*,#45599,.T.) ;
#61259=ORIENTED_EDGE('',*,*,#45600,.T.) ;
#61260=ORIENTED_EDGE('',*,*,#45601,.T.) ;
#61261=ORIENTED_EDGE('',*,*,#45602,.T.) ;
#61262=ORIENTED_EDGE('',*,*,#45603,.T.) ;
#61263=ORIENTED_EDGE('',*,*,#45604,.T.) ;
#61264=ORIENTED_EDGE('',*,*,#45605,.T.) ;
#61265=ORIENTED_EDGE('',*,*,#45606,.T.) ;
#61266=ORIENTED_EDGE('',*,*,#45607,.T.) ;
#61267=ORIENTED_EDGE('',*,*,#45608,.T.) ;
#61268=ORIENTED_EDGE('',*,*,#45609,.T.) ;
#61269=ORIENTED_EDGE('',*,*,#45610,.T.) ;
#61270=ORIENTED_EDGE('',*,*,#45611,.T.) ;
#61271=ORIENTED_EDGE('',*,*,#45612,.T.) ;
#61272=ORIENTED_EDGE('',*,*,#44244,.T.) ;
#61273=ORIENTED_EDGE('',*,*,#45613,.T.) ;
#61274=ORIENTED_EDGE('',*,*,#45614,.T.) ;
#61275=ORIENTED_EDGE('',*,*,#45615,.T.) ;
#61276=ORIENTED_EDGE('',*,*,#45616,.T.) ;
#61277=ORIENTED_EDGE('',*,*,#45617,.T.) ;
#61278=ORIENTED_EDGE('',*,*,#45618,.T.) ;
#61279=ORIENTED_EDGE('',*,*,#45619,.T.) ;
#61280=ORIENTED_EDGE('',*,*,#45620,.T.) ;
#61281=ORIENTED_EDGE('',*,*,#45621,.T.) ;
#61282=ORIENTED_EDGE('',*,*,#45622,.T.) ;
#61283=ORIENTED_EDGE('',*,*,#45623,.T.) ;
#61284=ORIENTED_EDGE('',*,*,#45624,.T.) ;
#61285=ORIENTED_EDGE('',*,*,#45625,.T.) ;
#61286=ORIENTED_EDGE('',*,*,#45626,.T.) ;
#61287=ORIENTED_EDGE('',*,*,#45627,.T.) ;
#61288=ORIENTED_EDGE('',*,*,#45628,.T.) ;
#61289=ORIENTED_EDGE('',*,*,#45629,.T.) ;
#61290=ORIENTED_EDGE('',*,*,#45630,.T.) ;
#61291=ORIENTED_EDGE('',*,*,#45631,.T.) ;
#61292=ORIENTED_EDGE('',*,*,#44227,.T.) ;
#61293=ORIENTED_EDGE('',*,*,#45632,.T.) ;
#61294=ORIENTED_EDGE('',*,*,#45633,.T.) ;
#61295=ORIENTED_EDGE('',*,*,#45634,.T.) ;
#61296=ORIENTED_EDGE('',*,*,#45635,.T.) ;
#61297=ORIENTED_EDGE('',*,*,#45636,.T.) ;
#61298=ORIENTED_EDGE('',*,*,#45637,.T.) ;
#61299=ORIENTED_EDGE('',*,*,#45638,.T.) ;
#61300=ORIENTED_EDGE('',*,*,#45639,.T.) ;
#61301=ORIENTED_EDGE('',*,*,#45640,.T.) ;
#61302=ORIENTED_EDGE('',*,*,#45641,.T.) ;
#61303=ORIENTED_EDGE('',*,*,#45642,.T.) ;
#61304=ORIENTED_EDGE('',*,*,#45643,.T.) ;
#61305=ORIENTED_EDGE('',*,*,#45644,.T.) ;
#61306=ORIENTED_EDGE('',*,*,#45645,.T.) ;
#61307=ORIENTED_EDGE('',*,*,#45646,.T.) ;
#61308=ORIENTED_EDGE('',*,*,#45647,.T.) ;
#61309=ORIENTED_EDGE('',*,*,#45648,.T.) ;
#61310=ORIENTED_EDGE('',*,*,#45649,.T.) ;
#61311=ORIENTED_EDGE('',*,*,#45650,.T.) ;
#61312=ORIENTED_EDGE('',*,*,#44210,.T.) ;
#61313=ORIENTED_EDGE('',*,*,#45651,.T.) ;
#61314=ORIENTED_EDGE('',*,*,#45652,.T.) ;
#61315=ORIENTED_EDGE('',*,*,#45653,.T.) ;
#61316=ORIENTED_EDGE('',*,*,#45654,.T.) ;
#61317=ORIENTED_EDGE('',*,*,#45655,.T.) ;
#61318=ORIENTED_EDGE('',*,*,#45656,.T.) ;
#61319=ORIENTED_EDGE('',*,*,#45657,.T.) ;
#61320=ORIENTED_EDGE('',*,*,#45658,.T.) ;
#61321=ORIENTED_EDGE('',*,*,#45659,.T.) ;
#61322=ORIENTED_EDGE('',*,*,#45660,.T.) ;
#61323=ORIENTED_EDGE('',*,*,#45661,.T.) ;
#61324=ORIENTED_EDGE('',*,*,#45662,.T.) ;
#61325=ORIENTED_EDGE('',*,*,#45663,.T.) ;
#61326=ORIENTED_EDGE('',*,*,#45664,.T.) ;
#61327=ORIENTED_EDGE('',*,*,#45665,.T.) ;
#61328=ORIENTED_EDGE('',*,*,#45666,.T.) ;
#61329=ORIENTED_EDGE('',*,*,#45667,.T.) ;
#61330=ORIENTED_EDGE('',*,*,#45668,.T.) ;
#61331=ORIENTED_EDGE('',*,*,#45669,.T.) ;
#61332=ORIENTED_EDGE('',*,*,#44193,.T.) ;
#61333=ORIENTED_EDGE('',*,*,#45670,.T.) ;
#61334=ORIENTED_EDGE('',*,*,#45671,.T.) ;
#61335=ORIENTED_EDGE('',*,*,#45672,.T.) ;
#61336=ORIENTED_EDGE('',*,*,#45673,.T.) ;
#61337=ORIENTED_EDGE('',*,*,#45674,.T.) ;
#61338=ORIENTED_EDGE('',*,*,#45675,.T.) ;
#61339=ORIENTED_EDGE('',*,*,#45676,.T.) ;
#61340=ORIENTED_EDGE('',*,*,#45677,.T.) ;
#61341=ORIENTED_EDGE('',*,*,#45678,.T.) ;
#61342=ORIENTED_EDGE('',*,*,#45679,.T.) ;
#61343=ORIENTED_EDGE('',*,*,#45680,.T.) ;
#61344=ORIENTED_EDGE('',*,*,#45681,.T.) ;
#61345=ORIENTED_EDGE('',*,*,#45682,.T.) ;
#61346=ORIENTED_EDGE('',*,*,#45683,.T.) ;
#61347=ORIENTED_EDGE('',*,*,#45684,.T.) ;
#61348=ORIENTED_EDGE('',*,*,#45685,.T.) ;
#61349=ORIENTED_EDGE('',*,*,#45686,.T.) ;
#61350=ORIENTED_EDGE('',*,*,#45687,.T.) ;
#61351=ORIENTED_EDGE('',*,*,#45688,.T.) ;
#61352=ORIENTED_EDGE('',*,*,#44176,.T.) ;
#61353=ORIENTED_EDGE('',*,*,#45689,.T.) ;
#61354=ORIENTED_EDGE('',*,*,#45690,.T.) ;
#61355=ORIENTED_EDGE('',*,*,#45691,.T.) ;
#61356=ORIENTED_EDGE('',*,*,#45692,.T.) ;
#61357=ORIENTED_EDGE('',*,*,#45693,.T.) ;
#61358=ORIENTED_EDGE('',*,*,#45694,.T.) ;
#61359=ORIENTED_EDGE('',*,*,#45695,.T.) ;
#61360=ORIENTED_EDGE('',*,*,#45696,.T.) ;
#61361=ORIENTED_EDGE('',*,*,#45697,.T.) ;
#61362=ORIENTED_EDGE('',*,*,#45698,.T.) ;
#61363=ORIENTED_EDGE('',*,*,#45699,.T.) ;
#61364=ORIENTED_EDGE('',*,*,#45700,.T.) ;
#61365=ORIENTED_EDGE('',*,*,#45701,.T.) ;
#61366=ORIENTED_EDGE('',*,*,#45702,.T.) ;
#61367=ORIENTED_EDGE('',*,*,#45703,.T.) ;
#61368=ORIENTED_EDGE('',*,*,#45704,.T.) ;
#61369=ORIENTED_EDGE('',*,*,#45705,.T.) ;
#61370=ORIENTED_EDGE('',*,*,#45706,.T.) ;
#61371=ORIENTED_EDGE('',*,*,#45707,.T.) ;
#61372=ORIENTED_EDGE('',*,*,#44159,.T.) ;
#61373=ORIENTED_EDGE('',*,*,#45708,.T.) ;
#61374=ORIENTED_EDGE('',*,*,#45709,.T.) ;
#61375=ORIENTED_EDGE('',*,*,#45710,.T.) ;
#61376=ORIENTED_EDGE('',*,*,#45711,.T.) ;
#61377=ORIENTED_EDGE('',*,*,#45712,.T.) ;
#61378=ORIENTED_EDGE('',*,*,#45713,.T.) ;
#61379=ORIENTED_EDGE('',*,*,#45714,.T.) ;
#61380=ORIENTED_EDGE('',*,*,#45715,.T.) ;
#61381=ORIENTED_EDGE('',*,*,#45716,.T.) ;
#61382=ORIENTED_EDGE('',*,*,#45717,.T.) ;
#61383=ORIENTED_EDGE('',*,*,#45718,.T.) ;
#61384=ORIENTED_EDGE('',*,*,#45719,.T.) ;
#61385=ORIENTED_EDGE('',*,*,#45720,.F.) ;
#61386=ORIENTED_EDGE('',*,*,#45721,.T.) ;
#61387=ORIENTED_EDGE('',*,*,#45722,.T.) ;
#61388=ORIENTED_EDGE('',*,*,#45723,.T.) ;
#61389=ORIENTED_EDGE('',*,*,#45722,.F.) ;
#61390=ORIENTED_EDGE('',*,*,#45724,.T.) ;
#61391=ORIENTED_EDGE('',*,*,#45725,.T.) ;
#61392=ORIENTED_EDGE('',*,*,#45726,.T.) ;
#61393=ORIENTED_EDGE('',*,*,#45725,.F.) ;
#61394=ORIENTED_EDGE('',*,*,#45727,.T.) ;
#61395=ORIENTED_EDGE('',*,*,#45728,.T.) ;
#61396=ORIENTED_EDGE('',*,*,#45729,.T.) ;
#61397=ORIENTED_EDGE('',*,*,#45728,.F.) ;
#61398=ORIENTED_EDGE('',*,*,#45730,.T.) ;
#61399=ORIENTED_EDGE('',*,*,#45731,.T.) ;
#61400=ORIENTED_EDGE('',*,*,#45732,.T.) ;
#61401=ORIENTED_EDGE('',*,*,#45731,.F.) ;
#61402=ORIENTED_EDGE('',*,*,#45733,.T.) ;
#61403=ORIENTED_EDGE('',*,*,#45734,.T.) ;
#61404=ORIENTED_EDGE('',*,*,#45735,.T.) ;
#61405=ORIENTED_EDGE('',*,*,#45734,.F.) ;
#61406=ORIENTED_EDGE('',*,*,#45736,.T.) ;
#61407=ORIENTED_EDGE('',*,*,#45737,.T.) ;
#61408=ORIENTED_EDGE('',*,*,#45738,.T.) ;
#61409=ORIENTED_EDGE('',*,*,#45737,.F.) ;
#61410=ORIENTED_EDGE('',*,*,#44154,.T.) ;
#61411=ORIENTED_EDGE('',*,*,#45739,.T.) ;
#61412=ORIENTED_EDGE('',*,*,#45740,.T.) ;
#61413=ORIENTED_EDGE('',*,*,#45739,.F.) ;
#61414=ORIENTED_EDGE('',*,*,#45741,.T.) ;
#61415=ORIENTED_EDGE('',*,*,#44371,.T.) ;
#61416=ORIENTED_EDGE('',*,*,#45742,.T.) ;
#61417=ORIENTED_EDGE('',*,*,#44370,.F.) ;
#61418=ORIENTED_EDGE('',*,*,#45743,.T.) ;
#61419=ORIENTED_EDGE('',*,*,#45744,.T.) ;
#61420=ORIENTED_EDGE('',*,*,#45745,.T.) ;
#61421=ORIENTED_EDGE('',*,*,#45744,.F.) ;
#61422=ORIENTED_EDGE('',*,*,#45746,.T.) ;
#61423=ORIENTED_EDGE('',*,*,#45747,.T.) ;
#61424=ORIENTED_EDGE('',*,*,#45748,.T.) ;
#61425=ORIENTED_EDGE('',*,*,#45747,.F.) ;
#61426=ORIENTED_EDGE('',*,*,#45749,.T.) ;
#61427=ORIENTED_EDGE('',*,*,#45750,.T.) ;
#61428=ORIENTED_EDGE('',*,*,#45751,.T.) ;
#61429=ORIENTED_EDGE('',*,*,#45750,.F.) ;
#61430=ORIENTED_EDGE('',*,*,#45752,.T.) ;
#61431=ORIENTED_EDGE('',*,*,#45753,.T.) ;
#61432=ORIENTED_EDGE('',*,*,#45754,.T.) ;
#61433=ORIENTED_EDGE('',*,*,#45753,.F.) ;
#61434=ORIENTED_EDGE('',*,*,#45755,.T.) ;
#61435=ORIENTED_EDGE('',*,*,#45756,.T.) ;
#61436=ORIENTED_EDGE('',*,*,#45757,.T.) ;
#61437=ORIENTED_EDGE('',*,*,#45756,.F.) ;
#61438=ORIENTED_EDGE('',*,*,#45758,.T.) ;
#61439=ORIENTED_EDGE('',*,*,#45759,.T.) ;
#61440=ORIENTED_EDGE('',*,*,#45760,.T.) ;
#61441=ORIENTED_EDGE('',*,*,#45759,.F.) ;
#61442=ORIENTED_EDGE('',*,*,#45761,.T.) ;
#61443=ORIENTED_EDGE('',*,*,#45762,.T.) ;
#61444=ORIENTED_EDGE('',*,*,#45763,.T.) ;
#61445=ORIENTED_EDGE('',*,*,#45762,.F.) ;
#61446=ORIENTED_EDGE('',*,*,#45764,.T.) ;
#61447=ORIENTED_EDGE('',*,*,#45765,.T.) ;
#61448=ORIENTED_EDGE('',*,*,#45766,.T.) ;
#61449=ORIENTED_EDGE('',*,*,#45765,.F.) ;
#61450=ORIENTED_EDGE('',*,*,#45767,.T.) ;
#61451=ORIENTED_EDGE('',*,*,#45768,.T.) ;
#61452=ORIENTED_EDGE('',*,*,#45769,.T.) ;
#61453=ORIENTED_EDGE('',*,*,#45768,.F.) ;
#61454=ORIENTED_EDGE('',*,*,#45770,.T.) ;
#61455=ORIENTED_EDGE('',*,*,#45771,.T.) ;
#61456=ORIENTED_EDGE('',*,*,#45772,.T.) ;
#61457=ORIENTED_EDGE('',*,*,#45771,.F.) ;
#61458=ORIENTED_EDGE('',*,*,#45773,.T.) ;
#61459=ORIENTED_EDGE('',*,*,#45774,.T.) ;
#61460=ORIENTED_EDGE('',*,*,#45775,.T.) ;
#61461=ORIENTED_EDGE('',*,*,#45774,.F.) ;
#61462=ORIENTED_EDGE('',*,*,#45776,.T.) ;
#61463=ORIENTED_EDGE('',*,*,#45777,.T.) ;
#61464=ORIENTED_EDGE('',*,*,#45778,.T.) ;
#61465=ORIENTED_EDGE('',*,*,#45777,.F.) ;
#61466=ORIENTED_EDGE('',*,*,#45779,.T.) ;
#61467=ORIENTED_EDGE('',*,*,#45780,.T.) ;
#61468=ORIENTED_EDGE('',*,*,#45781,.T.) ;
#61469=ORIENTED_EDGE('',*,*,#45780,.F.) ;
#61470=ORIENTED_EDGE('',*,*,#45782,.T.) ;
#61471=ORIENTED_EDGE('',*,*,#45783,.T.) ;
#61472=ORIENTED_EDGE('',*,*,#45784,.T.) ;
#61473=ORIENTED_EDGE('',*,*,#45783,.F.) ;
#61474=ORIENTED_EDGE('',*,*,#45785,.T.) ;
#61475=ORIENTED_EDGE('',*,*,#45786,.T.) ;
#61476=ORIENTED_EDGE('',*,*,#45787,.T.) ;
#61477=ORIENTED_EDGE('',*,*,#45786,.F.) ;
#61478=ORIENTED_EDGE('',*,*,#45788,.T.) ;
#61479=ORIENTED_EDGE('',*,*,#45789,.T.) ;
#61480=ORIENTED_EDGE('',*,*,#45790,.T.) ;
#61481=ORIENTED_EDGE('',*,*,#45789,.F.) ;
#61482=ORIENTED_EDGE('',*,*,#45791,.T.) ;
#61483=ORIENTED_EDGE('',*,*,#45792,.T.) ;
#61484=ORIENTED_EDGE('',*,*,#45793,.T.) ;
#61485=ORIENTED_EDGE('',*,*,#45792,.F.) ;
#61486=ORIENTED_EDGE('',*,*,#45794,.T.) ;
#61487=ORIENTED_EDGE('',*,*,#45795,.T.) ;
#61488=ORIENTED_EDGE('',*,*,#45796,.T.) ;
#61489=ORIENTED_EDGE('',*,*,#45795,.F.) ;
#61490=ORIENTED_EDGE('',*,*,#45797,.T.) ;
#61491=ORIENTED_EDGE('',*,*,#45720,.T.) ;
#61492=ORIENTED_EDGE('',*,*,#45798,.T.) ;
#61493=ORIENTED_EDGE('',*,*,#45799,.T.) ;
#61494=ORIENTED_EDGE('',*,*,#45800,.T.) ;
#61495=ORIENTED_EDGE('',*,*,#45801,.T.) ;
#61496=ORIENTED_EDGE('',*,*,#45802,.T.) ;
#61497=ORIENTED_EDGE('',*,*,#45803,.T.) ;
#61498=ORIENTED_EDGE('',*,*,#45804,.T.) ;
#61499=ORIENTED_EDGE('',*,*,#45805,.T.) ;
#61500=ORIENTED_EDGE('',*,*,#45806,.T.) ;
#61501=ORIENTED_EDGE('',*,*,#45807,.T.) ;
#61502=ORIENTED_EDGE('',*,*,#45808,.T.) ;
#61503=ORIENTED_EDGE('',*,*,#45809,.T.) ;
#61504=ORIENTED_EDGE('',*,*,#45810,.T.) ;
#61505=ORIENTED_EDGE('',*,*,#45811,.T.) ;
#61506=ORIENTED_EDGE('',*,*,#45812,.T.) ;
#61507=ORIENTED_EDGE('',*,*,#45813,.T.) ;
#61508=ORIENTED_EDGE('',*,*,#45814,.T.) ;
#61509=ORIENTED_EDGE('',*,*,#45815,.T.) ;
#61510=ORIENTED_EDGE('',*,*,#45816,.T.) ;
#61511=ORIENTED_EDGE('',*,*,#44151,.T.) ;
#61512=ORIENTED_EDGE('',*,*,#45817,.F.) ;
#61513=ORIENTED_EDGE('',*,*,#45818,.T.) ;
#61514=ORIENTED_EDGE('',*,*,#45819,.T.) ;
#61515=ORIENTED_EDGE('',*,*,#45820,.T.) ;
#61516=ORIENTED_EDGE('',*,*,#45819,.F.) ;
#61517=ORIENTED_EDGE('',*,*,#45821,.T.) ;
#61518=ORIENTED_EDGE('',*,*,#45822,.T.) ;
#61519=ORIENTED_EDGE('',*,*,#45823,.T.) ;
#61520=ORIENTED_EDGE('',*,*,#45822,.F.) ;
#61521=ORIENTED_EDGE('',*,*,#45824,.T.) ;
#61522=ORIENTED_EDGE('',*,*,#45825,.T.) ;
#61523=ORIENTED_EDGE('',*,*,#45826,.T.) ;
#61524=ORIENTED_EDGE('',*,*,#45825,.F.) ;
#61525=ORIENTED_EDGE('',*,*,#45827,.T.) ;
#61526=ORIENTED_EDGE('',*,*,#45828,.T.) ;
#61527=ORIENTED_EDGE('',*,*,#45829,.T.) ;
#61528=ORIENTED_EDGE('',*,*,#45828,.F.) ;
#61529=ORIENTED_EDGE('',*,*,#45830,.T.) ;
#61530=ORIENTED_EDGE('',*,*,#45831,.T.) ;
#61531=ORIENTED_EDGE('',*,*,#45832,.T.) ;
#61532=ORIENTED_EDGE('',*,*,#45831,.F.) ;
#61533=ORIENTED_EDGE('',*,*,#45833,.T.) ;
#61534=ORIENTED_EDGE('',*,*,#45834,.T.) ;
#61535=ORIENTED_EDGE('',*,*,#45835,.T.) ;
#61536=ORIENTED_EDGE('',*,*,#45834,.F.) ;
#61537=ORIENTED_EDGE('',*,*,#44171,.T.) ;
#61538=ORIENTED_EDGE('',*,*,#45836,.T.) ;
#61539=ORIENTED_EDGE('',*,*,#45837,.T.) ;
#61540=ORIENTED_EDGE('',*,*,#45836,.F.) ;
#61541=ORIENTED_EDGE('',*,*,#45838,.T.) ;
#61542=ORIENTED_EDGE('',*,*,#44368,.T.) ;
#61543=ORIENTED_EDGE('',*,*,#45839,.T.) ;
#61544=ORIENTED_EDGE('',*,*,#44367,.F.) ;
#61545=ORIENTED_EDGE('',*,*,#45840,.T.) ;
#61546=ORIENTED_EDGE('',*,*,#45841,.T.) ;
#61547=ORIENTED_EDGE('',*,*,#45842,.T.) ;
#61548=ORIENTED_EDGE('',*,*,#45841,.F.) ;
#61549=ORIENTED_EDGE('',*,*,#45843,.T.) ;
#61550=ORIENTED_EDGE('',*,*,#45844,.T.) ;
#61551=ORIENTED_EDGE('',*,*,#45845,.T.) ;
#61552=ORIENTED_EDGE('',*,*,#45844,.F.) ;
#61553=ORIENTED_EDGE('',*,*,#45846,.T.) ;
#61554=ORIENTED_EDGE('',*,*,#45847,.T.) ;
#61555=ORIENTED_EDGE('',*,*,#45848,.T.) ;
#61556=ORIENTED_EDGE('',*,*,#45847,.F.) ;
#61557=ORIENTED_EDGE('',*,*,#45849,.T.) ;
#61558=ORIENTED_EDGE('',*,*,#45850,.T.) ;
#61559=ORIENTED_EDGE('',*,*,#45851,.T.) ;
#61560=ORIENTED_EDGE('',*,*,#45850,.F.) ;
#61561=ORIENTED_EDGE('',*,*,#45852,.T.) ;
#61562=ORIENTED_EDGE('',*,*,#45853,.T.) ;
#61563=ORIENTED_EDGE('',*,*,#45854,.T.) ;
#61564=ORIENTED_EDGE('',*,*,#45853,.F.) ;
#61565=ORIENTED_EDGE('',*,*,#45855,.T.) ;
#61566=ORIENTED_EDGE('',*,*,#45856,.T.) ;
#61567=ORIENTED_EDGE('',*,*,#45857,.T.) ;
#61568=ORIENTED_EDGE('',*,*,#45856,.F.) ;
#61569=ORIENTED_EDGE('',*,*,#45858,.T.) ;
#61570=ORIENTED_EDGE('',*,*,#45859,.T.) ;
#61571=ORIENTED_EDGE('',*,*,#45860,.T.) ;
#61572=ORIENTED_EDGE('',*,*,#45859,.F.) ;
#61573=ORIENTED_EDGE('',*,*,#45861,.T.) ;
#61574=ORIENTED_EDGE('',*,*,#45862,.T.) ;
#61575=ORIENTED_EDGE('',*,*,#45863,.T.) ;
#61576=ORIENTED_EDGE('',*,*,#45862,.F.) ;
#61577=ORIENTED_EDGE('',*,*,#45864,.T.) ;
#61578=ORIENTED_EDGE('',*,*,#45865,.T.) ;
#61579=ORIENTED_EDGE('',*,*,#45866,.T.) ;
#61580=ORIENTED_EDGE('',*,*,#45865,.F.) ;
#61581=ORIENTED_EDGE('',*,*,#45867,.T.) ;
#61582=ORIENTED_EDGE('',*,*,#45868,.T.) ;
#61583=ORIENTED_EDGE('',*,*,#45869,.T.) ;
#61584=ORIENTED_EDGE('',*,*,#45868,.F.) ;
#61585=ORIENTED_EDGE('',*,*,#45870,.T.) ;
#61586=ORIENTED_EDGE('',*,*,#45871,.T.) ;
#61587=ORIENTED_EDGE('',*,*,#45872,.T.) ;
#61588=ORIENTED_EDGE('',*,*,#45871,.F.) ;
#61589=ORIENTED_EDGE('',*,*,#45873,.T.) ;
#61590=ORIENTED_EDGE('',*,*,#45874,.T.) ;
#61591=ORIENTED_EDGE('',*,*,#45875,.T.) ;
#61592=ORIENTED_EDGE('',*,*,#45874,.F.) ;
#61593=ORIENTED_EDGE('',*,*,#45876,.T.) ;
#61594=ORIENTED_EDGE('',*,*,#45877,.T.) ;
#61595=ORIENTED_EDGE('',*,*,#45878,.T.) ;
#61596=ORIENTED_EDGE('',*,*,#45877,.F.) ;
#61597=ORIENTED_EDGE('',*,*,#45879,.T.) ;
#61598=ORIENTED_EDGE('',*,*,#45880,.T.) ;
#61599=ORIENTED_EDGE('',*,*,#45881,.T.) ;
#61600=ORIENTED_EDGE('',*,*,#45880,.F.) ;
#61601=ORIENTED_EDGE('',*,*,#45882,.T.) ;
#61602=ORIENTED_EDGE('',*,*,#45883,.T.) ;
#61603=ORIENTED_EDGE('',*,*,#45884,.T.) ;
#61604=ORIENTED_EDGE('',*,*,#45883,.F.) ;
#61605=ORIENTED_EDGE('',*,*,#45885,.T.) ;
#61606=ORIENTED_EDGE('',*,*,#45886,.T.) ;
#61607=ORIENTED_EDGE('',*,*,#45887,.T.) ;
#61608=ORIENTED_EDGE('',*,*,#45886,.F.) ;
#61609=ORIENTED_EDGE('',*,*,#45888,.T.) ;
#61610=ORIENTED_EDGE('',*,*,#45889,.T.) ;
#61611=ORIENTED_EDGE('',*,*,#45890,.T.) ;
#61612=ORIENTED_EDGE('',*,*,#45889,.F.) ;
#61613=ORIENTED_EDGE('',*,*,#45891,.T.) ;
#61614=ORIENTED_EDGE('',*,*,#45892,.T.) ;
#61615=ORIENTED_EDGE('',*,*,#45893,.T.) ;
#61616=ORIENTED_EDGE('',*,*,#45892,.F.) ;
#61617=ORIENTED_EDGE('',*,*,#45894,.T.) ;
#61618=ORIENTED_EDGE('',*,*,#45817,.T.) ;
#61619=ORIENTED_EDGE('',*,*,#45895,.T.) ;
#61620=ORIENTED_EDGE('',*,*,#45896,.T.) ;
#61621=ORIENTED_EDGE('',*,*,#45897,.T.) ;
#61622=ORIENTED_EDGE('',*,*,#45898,.T.) ;
#61623=ORIENTED_EDGE('',*,*,#45899,.T.) ;
#61624=ORIENTED_EDGE('',*,*,#45900,.T.) ;
#61625=ORIENTED_EDGE('',*,*,#45901,.T.) ;
#61626=ORIENTED_EDGE('',*,*,#45902,.T.) ;
#61627=ORIENTED_EDGE('',*,*,#45903,.T.) ;
#61628=ORIENTED_EDGE('',*,*,#45904,.T.) ;
#61629=ORIENTED_EDGE('',*,*,#45905,.T.) ;
#61630=ORIENTED_EDGE('',*,*,#45906,.T.) ;
#61631=ORIENTED_EDGE('',*,*,#45907,.T.) ;
#61632=ORIENTED_EDGE('',*,*,#45908,.T.) ;
#61633=ORIENTED_EDGE('',*,*,#45909,.T.) ;
#61634=ORIENTED_EDGE('',*,*,#45910,.T.) ;
#61635=ORIENTED_EDGE('',*,*,#45911,.T.) ;
#61636=ORIENTED_EDGE('',*,*,#45912,.T.) ;
#61637=ORIENTED_EDGE('',*,*,#45913,.T.) ;
#61638=ORIENTED_EDGE('',*,*,#44168,.T.) ;
#61639=ORIENTED_EDGE('',*,*,#45914,.F.) ;
#61640=ORIENTED_EDGE('',*,*,#45915,.T.) ;
#61641=ORIENTED_EDGE('',*,*,#45916,.T.) ;
#61642=ORIENTED_EDGE('',*,*,#45917,.T.) ;
#61643=ORIENTED_EDGE('',*,*,#45916,.F.) ;
#61644=ORIENTED_EDGE('',*,*,#45918,.T.) ;
#61645=ORIENTED_EDGE('',*,*,#45919,.T.) ;
#61646=ORIENTED_EDGE('',*,*,#45920,.T.) ;
#61647=ORIENTED_EDGE('',*,*,#45919,.F.) ;
#61648=ORIENTED_EDGE('',*,*,#45921,.T.) ;
#61649=ORIENTED_EDGE('',*,*,#45922,.T.) ;
#61650=ORIENTED_EDGE('',*,*,#45923,.T.) ;
#61651=ORIENTED_EDGE('',*,*,#45922,.F.) ;
#61652=ORIENTED_EDGE('',*,*,#45924,.T.) ;
#61653=ORIENTED_EDGE('',*,*,#45925,.T.) ;
#61654=ORIENTED_EDGE('',*,*,#45926,.T.) ;
#61655=ORIENTED_EDGE('',*,*,#45925,.F.) ;
#61656=ORIENTED_EDGE('',*,*,#45927,.T.) ;
#61657=ORIENTED_EDGE('',*,*,#45928,.T.) ;
#61658=ORIENTED_EDGE('',*,*,#45929,.T.) ;
#61659=ORIENTED_EDGE('',*,*,#45928,.F.) ;
#61660=ORIENTED_EDGE('',*,*,#45930,.T.) ;
#61661=ORIENTED_EDGE('',*,*,#45931,.T.) ;
#61662=ORIENTED_EDGE('',*,*,#45932,.T.) ;
#61663=ORIENTED_EDGE('',*,*,#45931,.F.) ;
#61664=ORIENTED_EDGE('',*,*,#44188,.T.) ;
#61665=ORIENTED_EDGE('',*,*,#45933,.T.) ;
#61666=ORIENTED_EDGE('',*,*,#45934,.T.) ;
#61667=ORIENTED_EDGE('',*,*,#45933,.F.) ;
#61668=ORIENTED_EDGE('',*,*,#45935,.T.) ;
#61669=ORIENTED_EDGE('',*,*,#44365,.T.) ;
#61670=ORIENTED_EDGE('',*,*,#45936,.T.) ;
#61671=ORIENTED_EDGE('',*,*,#44364,.F.) ;
#61672=ORIENTED_EDGE('',*,*,#45937,.T.) ;
#61673=ORIENTED_EDGE('',*,*,#45938,.T.) ;
#61674=ORIENTED_EDGE('',*,*,#45939,.T.) ;
#61675=ORIENTED_EDGE('',*,*,#45938,.F.) ;
#61676=ORIENTED_EDGE('',*,*,#45940,.T.) ;
#61677=ORIENTED_EDGE('',*,*,#45941,.T.) ;
#61678=ORIENTED_EDGE('',*,*,#45942,.T.) ;
#61679=ORIENTED_EDGE('',*,*,#45941,.F.) ;
#61680=ORIENTED_EDGE('',*,*,#45943,.T.) ;
#61681=ORIENTED_EDGE('',*,*,#45944,.T.) ;
#61682=ORIENTED_EDGE('',*,*,#45945,.T.) ;
#61683=ORIENTED_EDGE('',*,*,#45944,.F.) ;
#61684=ORIENTED_EDGE('',*,*,#45946,.T.) ;
#61685=ORIENTED_EDGE('',*,*,#45947,.T.) ;
#61686=ORIENTED_EDGE('',*,*,#45948,.T.) ;
#61687=ORIENTED_EDGE('',*,*,#45947,.F.) ;
#61688=ORIENTED_EDGE('',*,*,#45949,.T.) ;
#61689=ORIENTED_EDGE('',*,*,#45950,.T.) ;
#61690=ORIENTED_EDGE('',*,*,#45951,.T.) ;
#61691=ORIENTED_EDGE('',*,*,#45950,.F.) ;
#61692=ORIENTED_EDGE('',*,*,#45952,.T.) ;
#61693=ORIENTED_EDGE('',*,*,#45953,.T.) ;
#61694=ORIENTED_EDGE('',*,*,#45954,.T.) ;
#61695=ORIENTED_EDGE('',*,*,#45953,.F.) ;
#61696=ORIENTED_EDGE('',*,*,#45955,.T.) ;
#61697=ORIENTED_EDGE('',*,*,#45956,.T.) ;
#61698=ORIENTED_EDGE('',*,*,#45957,.T.) ;
#61699=ORIENTED_EDGE('',*,*,#45956,.F.) ;
#61700=ORIENTED_EDGE('',*,*,#45958,.T.) ;
#61701=ORIENTED_EDGE('',*,*,#45959,.T.) ;
#61702=ORIENTED_EDGE('',*,*,#45960,.T.) ;
#61703=ORIENTED_EDGE('',*,*,#45959,.F.) ;
#61704=ORIENTED_EDGE('',*,*,#45961,.T.) ;
#61705=ORIENTED_EDGE('',*,*,#45962,.T.) ;
#61706=ORIENTED_EDGE('',*,*,#45963,.T.) ;
#61707=ORIENTED_EDGE('',*,*,#45962,.F.) ;
#61708=ORIENTED_EDGE('',*,*,#45964,.T.) ;
#61709=ORIENTED_EDGE('',*,*,#45965,.T.) ;
#61710=ORIENTED_EDGE('',*,*,#45966,.T.) ;
#61711=ORIENTED_EDGE('',*,*,#45965,.F.) ;
#61712=ORIENTED_EDGE('',*,*,#45967,.T.) ;
#61713=ORIENTED_EDGE('',*,*,#45968,.T.) ;
#61714=ORIENTED_EDGE('',*,*,#45969,.T.) ;
#61715=ORIENTED_EDGE('',*,*,#45968,.F.) ;
#61716=ORIENTED_EDGE('',*,*,#45970,.T.) ;
#61717=ORIENTED_EDGE('',*,*,#45971,.T.) ;
#61718=ORIENTED_EDGE('',*,*,#45972,.T.) ;
#61719=ORIENTED_EDGE('',*,*,#45971,.F.) ;
#61720=ORIENTED_EDGE('',*,*,#45973,.T.) ;
#61721=ORIENTED_EDGE('',*,*,#45974,.T.) ;
#61722=ORIENTED_EDGE('',*,*,#45975,.T.) ;
#61723=ORIENTED_EDGE('',*,*,#45974,.F.) ;
#61724=ORIENTED_EDGE('',*,*,#45976,.T.) ;
#61725=ORIENTED_EDGE('',*,*,#45977,.T.) ;
#61726=ORIENTED_EDGE('',*,*,#45978,.T.) ;
#61727=ORIENTED_EDGE('',*,*,#45977,.F.) ;
#61728=ORIENTED_EDGE('',*,*,#45979,.T.) ;
#61729=ORIENTED_EDGE('',*,*,#45980,.T.) ;
#61730=ORIENTED_EDGE('',*,*,#45981,.T.) ;
#61731=ORIENTED_EDGE('',*,*,#45980,.F.) ;
#61732=ORIENTED_EDGE('',*,*,#45982,.T.) ;
#61733=ORIENTED_EDGE('',*,*,#45983,.T.) ;
#61734=ORIENTED_EDGE('',*,*,#45984,.T.) ;
#61735=ORIENTED_EDGE('',*,*,#45983,.F.) ;
#61736=ORIENTED_EDGE('',*,*,#45985,.T.) ;
#61737=ORIENTED_EDGE('',*,*,#45986,.T.) ;
#61738=ORIENTED_EDGE('',*,*,#45987,.T.) ;
#61739=ORIENTED_EDGE('',*,*,#45986,.F.) ;
#61740=ORIENTED_EDGE('',*,*,#45988,.T.) ;
#61741=ORIENTED_EDGE('',*,*,#45989,.T.) ;
#61742=ORIENTED_EDGE('',*,*,#45990,.T.) ;
#61743=ORIENTED_EDGE('',*,*,#45989,.F.) ;
#61744=ORIENTED_EDGE('',*,*,#45991,.T.) ;
#61745=ORIENTED_EDGE('',*,*,#45914,.T.) ;
#61746=ORIENTED_EDGE('',*,*,#45992,.T.) ;
#61747=ORIENTED_EDGE('',*,*,#45993,.T.) ;
#61748=ORIENTED_EDGE('',*,*,#45994,.T.) ;
#61749=ORIENTED_EDGE('',*,*,#45995,.T.) ;
#61750=ORIENTED_EDGE('',*,*,#45996,.T.) ;
#61751=ORIENTED_EDGE('',*,*,#45997,.T.) ;
#61752=ORIENTED_EDGE('',*,*,#45998,.T.) ;
#61753=ORIENTED_EDGE('',*,*,#45999,.T.) ;
#61754=ORIENTED_EDGE('',*,*,#46000,.T.) ;
#61755=ORIENTED_EDGE('',*,*,#46001,.T.) ;
#61756=ORIENTED_EDGE('',*,*,#46002,.T.) ;
#61757=ORIENTED_EDGE('',*,*,#46003,.T.) ;
#61758=ORIENTED_EDGE('',*,*,#46004,.T.) ;
#61759=ORIENTED_EDGE('',*,*,#46005,.T.) ;
#61760=ORIENTED_EDGE('',*,*,#46006,.T.) ;
#61761=ORIENTED_EDGE('',*,*,#46007,.T.) ;
#61762=ORIENTED_EDGE('',*,*,#46008,.T.) ;
#61763=ORIENTED_EDGE('',*,*,#46009,.T.) ;
#61764=ORIENTED_EDGE('',*,*,#46010,.T.) ;
#61765=ORIENTED_EDGE('',*,*,#44185,.T.) ;
#61766=ORIENTED_EDGE('',*,*,#46011,.F.) ;
#61767=ORIENTED_EDGE('',*,*,#46012,.T.) ;
#61768=ORIENTED_EDGE('',*,*,#46013,.T.) ;
#61769=ORIENTED_EDGE('',*,*,#46014,.T.) ;
#61770=ORIENTED_EDGE('',*,*,#46013,.F.) ;
#61771=ORIENTED_EDGE('',*,*,#46015,.T.) ;
#61772=ORIENTED_EDGE('',*,*,#46016,.T.) ;
#61773=ORIENTED_EDGE('',*,*,#46017,.T.) ;
#61774=ORIENTED_EDGE('',*,*,#46016,.F.) ;
#61775=ORIENTED_EDGE('',*,*,#46018,.T.) ;
#61776=ORIENTED_EDGE('',*,*,#46019,.T.) ;
#61777=ORIENTED_EDGE('',*,*,#46020,.T.) ;
#61778=ORIENTED_EDGE('',*,*,#46019,.F.) ;
#61779=ORIENTED_EDGE('',*,*,#46021,.T.) ;
#61780=ORIENTED_EDGE('',*,*,#46022,.T.) ;
#61781=ORIENTED_EDGE('',*,*,#46023,.T.) ;
#61782=ORIENTED_EDGE('',*,*,#46022,.F.) ;
#61783=ORIENTED_EDGE('',*,*,#46024,.T.) ;
#61784=ORIENTED_EDGE('',*,*,#46025,.T.) ;
#61785=ORIENTED_EDGE('',*,*,#46026,.T.) ;
#61786=ORIENTED_EDGE('',*,*,#46025,.F.) ;
#61787=ORIENTED_EDGE('',*,*,#46027,.T.) ;
#61788=ORIENTED_EDGE('',*,*,#46028,.T.) ;
#61789=ORIENTED_EDGE('',*,*,#46029,.T.) ;
#61790=ORIENTED_EDGE('',*,*,#46028,.F.) ;
#61791=ORIENTED_EDGE('',*,*,#44205,.T.) ;
#61792=ORIENTED_EDGE('',*,*,#46030,.T.) ;
#61793=ORIENTED_EDGE('',*,*,#46031,.T.) ;
#61794=ORIENTED_EDGE('',*,*,#46030,.F.) ;
#61795=ORIENTED_EDGE('',*,*,#46032,.T.) ;
#61796=ORIENTED_EDGE('',*,*,#44362,.T.) ;
#61797=ORIENTED_EDGE('',*,*,#46033,.T.) ;
#61798=ORIENTED_EDGE('',*,*,#44361,.F.) ;
#61799=ORIENTED_EDGE('',*,*,#46034,.T.) ;
#61800=ORIENTED_EDGE('',*,*,#46035,.T.) ;
#61801=ORIENTED_EDGE('',*,*,#46036,.T.) ;
#61802=ORIENTED_EDGE('',*,*,#46035,.F.) ;
#61803=ORIENTED_EDGE('',*,*,#46037,.T.) ;
#61804=ORIENTED_EDGE('',*,*,#46038,.T.) ;
#61805=ORIENTED_EDGE('',*,*,#46039,.T.) ;
#61806=ORIENTED_EDGE('',*,*,#46038,.F.) ;
#61807=ORIENTED_EDGE('',*,*,#46040,.T.) ;
#61808=ORIENTED_EDGE('',*,*,#46041,.T.) ;
#61809=ORIENTED_EDGE('',*,*,#46042,.T.) ;
#61810=ORIENTED_EDGE('',*,*,#46041,.F.) ;
#61811=ORIENTED_EDGE('',*,*,#46043,.T.) ;
#61812=ORIENTED_EDGE('',*,*,#46044,.T.) ;
#61813=ORIENTED_EDGE('',*,*,#46045,.T.) ;
#61814=ORIENTED_EDGE('',*,*,#46044,.F.) ;
#61815=ORIENTED_EDGE('',*,*,#46046,.T.) ;
#61816=ORIENTED_EDGE('',*,*,#46047,.T.) ;
#61817=ORIENTED_EDGE('',*,*,#46048,.T.) ;
#61818=ORIENTED_EDGE('',*,*,#46047,.F.) ;
#61819=ORIENTED_EDGE('',*,*,#46049,.T.) ;
#61820=ORIENTED_EDGE('',*,*,#46050,.T.) ;
#61821=ORIENTED_EDGE('',*,*,#46051,.T.) ;
#61822=ORIENTED_EDGE('',*,*,#46050,.F.) ;
#61823=ORIENTED_EDGE('',*,*,#46052,.T.) ;
#61824=ORIENTED_EDGE('',*,*,#46053,.T.) ;
#61825=ORIENTED_EDGE('',*,*,#46054,.T.) ;
#61826=ORIENTED_EDGE('',*,*,#46053,.F.) ;
#61827=ORIENTED_EDGE('',*,*,#46055,.T.) ;
#61828=ORIENTED_EDGE('',*,*,#46056,.T.) ;
#61829=ORIENTED_EDGE('',*,*,#46057,.T.) ;
#61830=ORIENTED_EDGE('',*,*,#46056,.F.) ;
#61831=ORIENTED_EDGE('',*,*,#46058,.T.) ;
#61832=ORIENTED_EDGE('',*,*,#46059,.T.) ;
#61833=ORIENTED_EDGE('',*,*,#46060,.T.) ;
#61834=ORIENTED_EDGE('',*,*,#46059,.F.) ;
#61835=ORIENTED_EDGE('',*,*,#46061,.T.) ;
#61836=ORIENTED_EDGE('',*,*,#46062,.T.) ;
#61837=ORIENTED_EDGE('',*,*,#46063,.T.) ;
#61838=ORIENTED_EDGE('',*,*,#46062,.F.) ;
#61839=ORIENTED_EDGE('',*,*,#46064,.T.) ;
#61840=ORIENTED_EDGE('',*,*,#46065,.T.) ;
#61841=ORIENTED_EDGE('',*,*,#46066,.T.) ;
#61842=ORIENTED_EDGE('',*,*,#46065,.F.) ;
#61843=ORIENTED_EDGE('',*,*,#46067,.T.) ;
#61844=ORIENTED_EDGE('',*,*,#46068,.T.) ;
#61845=ORIENTED_EDGE('',*,*,#46069,.T.) ;
#61846=ORIENTED_EDGE('',*,*,#46068,.F.) ;
#61847=ORIENTED_EDGE('',*,*,#46070,.T.) ;
#61848=ORIENTED_EDGE('',*,*,#46071,.T.) ;
#61849=ORIENTED_EDGE('',*,*,#46072,.T.) ;
#61850=ORIENTED_EDGE('',*,*,#46071,.F.) ;
#61851=ORIENTED_EDGE('',*,*,#46073,.T.) ;
#61852=ORIENTED_EDGE('',*,*,#46074,.T.) ;
#61853=ORIENTED_EDGE('',*,*,#46075,.T.) ;
#61854=ORIENTED_EDGE('',*,*,#46074,.F.) ;
#61855=ORIENTED_EDGE('',*,*,#46076,.T.) ;
#61856=ORIENTED_EDGE('',*,*,#46077,.T.) ;
#61857=ORIENTED_EDGE('',*,*,#46078,.T.) ;
#61858=ORIENTED_EDGE('',*,*,#46077,.F.) ;
#61859=ORIENTED_EDGE('',*,*,#46079,.T.) ;
#61860=ORIENTED_EDGE('',*,*,#46080,.T.) ;
#61861=ORIENTED_EDGE('',*,*,#46081,.T.) ;
#61862=ORIENTED_EDGE('',*,*,#46080,.F.) ;
#61863=ORIENTED_EDGE('',*,*,#46082,.T.) ;
#61864=ORIENTED_EDGE('',*,*,#46083,.T.) ;
#61865=ORIENTED_EDGE('',*,*,#46084,.T.) ;
#61866=ORIENTED_EDGE('',*,*,#46083,.F.) ;
#61867=ORIENTED_EDGE('',*,*,#46085,.T.) ;
#61868=ORIENTED_EDGE('',*,*,#46086,.T.) ;
#61869=ORIENTED_EDGE('',*,*,#46087,.T.) ;
#61870=ORIENTED_EDGE('',*,*,#46086,.F.) ;
#61871=ORIENTED_EDGE('',*,*,#46088,.T.) ;
#61872=ORIENTED_EDGE('',*,*,#46011,.T.) ;
#61873=ORIENTED_EDGE('',*,*,#46089,.T.) ;
#61874=ORIENTED_EDGE('',*,*,#46090,.T.) ;
#61875=ORIENTED_EDGE('',*,*,#46091,.T.) ;
#61876=ORIENTED_EDGE('',*,*,#46092,.T.) ;
#61877=ORIENTED_EDGE('',*,*,#46093,.T.) ;
#61878=ORIENTED_EDGE('',*,*,#46094,.T.) ;
#61879=ORIENTED_EDGE('',*,*,#46095,.T.) ;
#61880=ORIENTED_EDGE('',*,*,#46096,.T.) ;
#61881=ORIENTED_EDGE('',*,*,#46097,.T.) ;
#61882=ORIENTED_EDGE('',*,*,#46098,.T.) ;
#61883=ORIENTED_EDGE('',*,*,#46099,.T.) ;
#61884=ORIENTED_EDGE('',*,*,#46100,.T.) ;
#61885=ORIENTED_EDGE('',*,*,#46101,.T.) ;
#61886=ORIENTED_EDGE('',*,*,#46102,.T.) ;
#61887=ORIENTED_EDGE('',*,*,#46103,.T.) ;
#61888=ORIENTED_EDGE('',*,*,#46104,.T.) ;
#61889=ORIENTED_EDGE('',*,*,#46105,.T.) ;
#61890=ORIENTED_EDGE('',*,*,#46106,.T.) ;
#61891=ORIENTED_EDGE('',*,*,#46107,.T.) ;
#61892=ORIENTED_EDGE('',*,*,#44202,.T.) ;
#61893=ORIENTED_EDGE('',*,*,#46108,.F.) ;
#61894=ORIENTED_EDGE('',*,*,#46109,.T.) ;
#61895=ORIENTED_EDGE('',*,*,#46110,.T.) ;
#61896=ORIENTED_EDGE('',*,*,#46111,.T.) ;
#61897=ORIENTED_EDGE('',*,*,#46110,.F.) ;
#61898=ORIENTED_EDGE('',*,*,#46112,.T.) ;
#61899=ORIENTED_EDGE('',*,*,#46113,.T.) ;
#61900=ORIENTED_EDGE('',*,*,#46114,.T.) ;
#61901=ORIENTED_EDGE('',*,*,#46113,.F.) ;
#61902=ORIENTED_EDGE('',*,*,#46115,.T.) ;
#61903=ORIENTED_EDGE('',*,*,#46116,.T.) ;
#61904=ORIENTED_EDGE('',*,*,#46117,.T.) ;
#61905=ORIENTED_EDGE('',*,*,#46116,.F.) ;
#61906=ORIENTED_EDGE('',*,*,#46118,.T.) ;
#61907=ORIENTED_EDGE('',*,*,#46119,.T.) ;
#61908=ORIENTED_EDGE('',*,*,#46120,.T.) ;
#61909=ORIENTED_EDGE('',*,*,#46119,.F.) ;
#61910=ORIENTED_EDGE('',*,*,#46121,.T.) ;
#61911=ORIENTED_EDGE('',*,*,#46122,.T.) ;
#61912=ORIENTED_EDGE('',*,*,#46123,.T.) ;
#61913=ORIENTED_EDGE('',*,*,#46122,.F.) ;
#61914=ORIENTED_EDGE('',*,*,#46124,.T.) ;
#61915=ORIENTED_EDGE('',*,*,#46125,.T.) ;
#61916=ORIENTED_EDGE('',*,*,#46126,.T.) ;
#61917=ORIENTED_EDGE('',*,*,#46125,.F.) ;
#61918=ORIENTED_EDGE('',*,*,#44222,.T.) ;
#61919=ORIENTED_EDGE('',*,*,#46127,.T.) ;
#61920=ORIENTED_EDGE('',*,*,#46128,.T.) ;
#61921=ORIENTED_EDGE('',*,*,#46127,.F.) ;
#61922=ORIENTED_EDGE('',*,*,#46129,.T.) ;
#61923=ORIENTED_EDGE('',*,*,#44359,.T.) ;
#61924=ORIENTED_EDGE('',*,*,#46130,.T.) ;
#61925=ORIENTED_EDGE('',*,*,#44358,.F.) ;
#61926=ORIENTED_EDGE('',*,*,#46131,.T.) ;
#61927=ORIENTED_EDGE('',*,*,#46132,.T.) ;
#61928=ORIENTED_EDGE('',*,*,#46133,.T.) ;
#61929=ORIENTED_EDGE('',*,*,#46132,.F.) ;
#61930=ORIENTED_EDGE('',*,*,#46134,.T.) ;
#61931=ORIENTED_EDGE('',*,*,#46135,.T.) ;
#61932=ORIENTED_EDGE('',*,*,#46136,.T.) ;
#61933=ORIENTED_EDGE('',*,*,#46135,.F.) ;
#61934=ORIENTED_EDGE('',*,*,#46137,.T.) ;
#61935=ORIENTED_EDGE('',*,*,#46138,.T.) ;
#61936=ORIENTED_EDGE('',*,*,#46139,.T.) ;
#61937=ORIENTED_EDGE('',*,*,#46138,.F.) ;
#61938=ORIENTED_EDGE('',*,*,#46140,.T.) ;
#61939=ORIENTED_EDGE('',*,*,#46141,.T.) ;
#61940=ORIENTED_EDGE('',*,*,#46142,.T.) ;
#61941=ORIENTED_EDGE('',*,*,#46141,.F.) ;
#61942=ORIENTED_EDGE('',*,*,#46143,.T.) ;
#61943=ORIENTED_EDGE('',*,*,#46144,.T.) ;
#61944=ORIENTED_EDGE('',*,*,#46145,.T.) ;
#61945=ORIENTED_EDGE('',*,*,#46144,.F.) ;
#61946=ORIENTED_EDGE('',*,*,#46146,.T.) ;
#61947=ORIENTED_EDGE('',*,*,#46147,.T.) ;
#61948=ORIENTED_EDGE('',*,*,#46148,.T.) ;
#61949=ORIENTED_EDGE('',*,*,#46147,.F.) ;
#61950=ORIENTED_EDGE('',*,*,#46149,.T.) ;
#61951=ORIENTED_EDGE('',*,*,#46150,.T.) ;
#61952=ORIENTED_EDGE('',*,*,#46151,.T.) ;
#61953=ORIENTED_EDGE('',*,*,#46150,.F.) ;
#61954=ORIENTED_EDGE('',*,*,#46152,.T.) ;
#61955=ORIENTED_EDGE('',*,*,#46153,.T.) ;
#61956=ORIENTED_EDGE('',*,*,#46154,.T.) ;
#61957=ORIENTED_EDGE('',*,*,#46153,.F.) ;
#61958=ORIENTED_EDGE('',*,*,#46155,.T.) ;
#61959=ORIENTED_EDGE('',*,*,#46156,.T.) ;
#61960=ORIENTED_EDGE('',*,*,#46157,.T.) ;
#61961=ORIENTED_EDGE('',*,*,#46156,.F.) ;
#61962=ORIENTED_EDGE('',*,*,#46158,.T.) ;
#61963=ORIENTED_EDGE('',*,*,#46159,.T.) ;
#61964=ORIENTED_EDGE('',*,*,#46160,.T.) ;
#61965=ORIENTED_EDGE('',*,*,#46159,.F.) ;
#61966=ORIENTED_EDGE('',*,*,#46161,.T.) ;
#61967=ORIENTED_EDGE('',*,*,#46162,.T.) ;
#61968=ORIENTED_EDGE('',*,*,#46163,.T.) ;
#61969=ORIENTED_EDGE('',*,*,#46162,.F.) ;
#61970=ORIENTED_EDGE('',*,*,#46164,.T.) ;
#61971=ORIENTED_EDGE('',*,*,#46165,.T.) ;
#61972=ORIENTED_EDGE('',*,*,#46166,.T.) ;
#61973=ORIENTED_EDGE('',*,*,#46165,.F.) ;
#61974=ORIENTED_EDGE('',*,*,#46167,.T.) ;
#61975=ORIENTED_EDGE('',*,*,#46168,.T.) ;
#61976=ORIENTED_EDGE('',*,*,#46169,.T.) ;
#61977=ORIENTED_EDGE('',*,*,#46168,.F.) ;
#61978=ORIENTED_EDGE('',*,*,#46170,.T.) ;
#61979=ORIENTED_EDGE('',*,*,#46171,.T.) ;
#61980=ORIENTED_EDGE('',*,*,#46172,.T.) ;
#61981=ORIENTED_EDGE('',*,*,#46171,.F.) ;
#61982=ORIENTED_EDGE('',*,*,#46173,.T.) ;
#61983=ORIENTED_EDGE('',*,*,#46174,.T.) ;
#61984=ORIENTED_EDGE('',*,*,#46175,.T.) ;
#61985=ORIENTED_EDGE('',*,*,#46174,.F.) ;
#61986=ORIENTED_EDGE('',*,*,#46176,.T.) ;
#61987=ORIENTED_EDGE('',*,*,#46177,.T.) ;
#61988=ORIENTED_EDGE('',*,*,#46178,.T.) ;
#61989=ORIENTED_EDGE('',*,*,#46177,.F.) ;
#61990=ORIENTED_EDGE('',*,*,#46179,.T.) ;
#61991=ORIENTED_EDGE('',*,*,#46180,.T.) ;
#61992=ORIENTED_EDGE('',*,*,#46181,.T.) ;
#61993=ORIENTED_EDGE('',*,*,#46180,.F.) ;
#61994=ORIENTED_EDGE('',*,*,#46182,.T.) ;
#61995=ORIENTED_EDGE('',*,*,#46183,.T.) ;
#61996=ORIENTED_EDGE('',*,*,#46184,.T.) ;
#61997=ORIENTED_EDGE('',*,*,#46183,.F.) ;
#61998=ORIENTED_EDGE('',*,*,#46185,.T.) ;
#61999=ORIENTED_EDGE('',*,*,#46108,.T.) ;
#62000=ORIENTED_EDGE('',*,*,#46186,.T.) ;
#62001=ORIENTED_EDGE('',*,*,#46187,.T.) ;
#62002=ORIENTED_EDGE('',*,*,#46188,.T.) ;
#62003=ORIENTED_EDGE('',*,*,#46189,.T.) ;
#62004=ORIENTED_EDGE('',*,*,#46190,.T.) ;
#62005=ORIENTED_EDGE('',*,*,#46191,.T.) ;
#62006=ORIENTED_EDGE('',*,*,#46192,.T.) ;
#62007=ORIENTED_EDGE('',*,*,#46193,.T.) ;
#62008=ORIENTED_EDGE('',*,*,#46194,.T.) ;
#62009=ORIENTED_EDGE('',*,*,#46195,.T.) ;
#62010=ORIENTED_EDGE('',*,*,#46196,.T.) ;
#62011=ORIENTED_EDGE('',*,*,#46197,.T.) ;
#62012=ORIENTED_EDGE('',*,*,#46198,.T.) ;
#62013=ORIENTED_EDGE('',*,*,#46199,.T.) ;
#62014=ORIENTED_EDGE('',*,*,#46200,.T.) ;
#62015=ORIENTED_EDGE('',*,*,#46201,.T.) ;
#62016=ORIENTED_EDGE('',*,*,#46202,.T.) ;
#62017=ORIENTED_EDGE('',*,*,#46203,.T.) ;
#62018=ORIENTED_EDGE('',*,*,#46204,.T.) ;
#62019=ORIENTED_EDGE('',*,*,#44219,.T.) ;
#62020=ORIENTED_EDGE('',*,*,#46205,.F.) ;
#62021=ORIENTED_EDGE('',*,*,#46206,.T.) ;
#62022=ORIENTED_EDGE('',*,*,#46207,.T.) ;
#62023=ORIENTED_EDGE('',*,*,#46208,.T.) ;
#62024=ORIENTED_EDGE('',*,*,#46207,.F.) ;
#62025=ORIENTED_EDGE('',*,*,#46209,.T.) ;
#62026=ORIENTED_EDGE('',*,*,#46210,.T.) ;
#62027=ORIENTED_EDGE('',*,*,#46211,.T.) ;
#62028=ORIENTED_EDGE('',*,*,#46210,.F.) ;
#62029=ORIENTED_EDGE('',*,*,#46212,.T.) ;
#62030=ORIENTED_EDGE('',*,*,#46213,.T.) ;
#62031=ORIENTED_EDGE('',*,*,#46214,.T.) ;
#62032=ORIENTED_EDGE('',*,*,#46213,.F.) ;
#62033=ORIENTED_EDGE('',*,*,#46215,.T.) ;
#62034=ORIENTED_EDGE('',*,*,#46216,.T.) ;
#62035=ORIENTED_EDGE('',*,*,#46217,.T.) ;
#62036=ORIENTED_EDGE('',*,*,#46216,.F.) ;
#62037=ORIENTED_EDGE('',*,*,#46218,.T.) ;
#62038=ORIENTED_EDGE('',*,*,#46219,.T.) ;
#62039=ORIENTED_EDGE('',*,*,#46220,.T.) ;
#62040=ORIENTED_EDGE('',*,*,#46219,.F.) ;
#62041=ORIENTED_EDGE('',*,*,#46221,.T.) ;
#62042=ORIENTED_EDGE('',*,*,#46222,.T.) ;
#62043=ORIENTED_EDGE('',*,*,#46223,.T.) ;
#62044=ORIENTED_EDGE('',*,*,#46222,.F.) ;
#62045=ORIENTED_EDGE('',*,*,#44239,.T.) ;
#62046=ORIENTED_EDGE('',*,*,#46224,.T.) ;
#62047=ORIENTED_EDGE('',*,*,#46225,.T.) ;
#62048=ORIENTED_EDGE('',*,*,#46224,.F.) ;
#62049=ORIENTED_EDGE('',*,*,#46226,.T.) ;
#62050=ORIENTED_EDGE('',*,*,#44356,.T.) ;
#62051=ORIENTED_EDGE('',*,*,#46227,.T.) ;
#62052=ORIENTED_EDGE('',*,*,#44355,.F.) ;
#62053=ORIENTED_EDGE('',*,*,#46228,.T.) ;
#62054=ORIENTED_EDGE('',*,*,#46229,.T.) ;
#62055=ORIENTED_EDGE('',*,*,#46230,.T.) ;
#62056=ORIENTED_EDGE('',*,*,#46229,.F.) ;
#62057=ORIENTED_EDGE('',*,*,#46231,.T.) ;
#62058=ORIENTED_EDGE('',*,*,#46232,.T.) ;
#62059=ORIENTED_EDGE('',*,*,#46233,.T.) ;
#62060=ORIENTED_EDGE('',*,*,#46232,.F.) ;
#62061=ORIENTED_EDGE('',*,*,#46234,.T.) ;
#62062=ORIENTED_EDGE('',*,*,#46235,.T.) ;
#62063=ORIENTED_EDGE('',*,*,#46236,.T.) ;
#62064=ORIENTED_EDGE('',*,*,#46235,.F.) ;
#62065=ORIENTED_EDGE('',*,*,#46237,.T.) ;
#62066=ORIENTED_EDGE('',*,*,#46238,.T.) ;
#62067=ORIENTED_EDGE('',*,*,#46239,.T.) ;
#62068=ORIENTED_EDGE('',*,*,#46238,.F.) ;
#62069=ORIENTED_EDGE('',*,*,#46240,.T.) ;
#62070=ORIENTED_EDGE('',*,*,#46241,.T.) ;
#62071=ORIENTED_EDGE('',*,*,#46242,.T.) ;
#62072=ORIENTED_EDGE('',*,*,#46241,.F.) ;
#62073=ORIENTED_EDGE('',*,*,#46243,.T.) ;
#62074=ORIENTED_EDGE('',*,*,#46244,.T.) ;
#62075=ORIENTED_EDGE('',*,*,#46245,.T.) ;
#62076=ORIENTED_EDGE('',*,*,#46244,.F.) ;
#62077=ORIENTED_EDGE('',*,*,#46246,.T.) ;
#62078=ORIENTED_EDGE('',*,*,#46247,.T.) ;
#62079=ORIENTED_EDGE('',*,*,#46248,.T.) ;
#62080=ORIENTED_EDGE('',*,*,#46247,.F.) ;
#62081=ORIENTED_EDGE('',*,*,#46249,.T.) ;
#62082=ORIENTED_EDGE('',*,*,#46250,.T.) ;
#62083=ORIENTED_EDGE('',*,*,#46251,.T.) ;
#62084=ORIENTED_EDGE('',*,*,#46250,.F.) ;
#62085=ORIENTED_EDGE('',*,*,#46252,.T.) ;
#62086=ORIENTED_EDGE('',*,*,#46253,.T.) ;
#62087=ORIENTED_EDGE('',*,*,#46254,.T.) ;
#62088=ORIENTED_EDGE('',*,*,#46253,.F.) ;
#62089=ORIENTED_EDGE('',*,*,#46255,.T.) ;
#62090=ORIENTED_EDGE('',*,*,#46256,.T.) ;
#62091=ORIENTED_EDGE('',*,*,#46257,.T.) ;
#62092=ORIENTED_EDGE('',*,*,#46256,.F.) ;
#62093=ORIENTED_EDGE('',*,*,#46258,.T.) ;
#62094=ORIENTED_EDGE('',*,*,#46259,.T.) ;
#62095=ORIENTED_EDGE('',*,*,#46260,.T.) ;
#62096=ORIENTED_EDGE('',*,*,#46259,.F.) ;
#62097=ORIENTED_EDGE('',*,*,#46261,.T.) ;
#62098=ORIENTED_EDGE('',*,*,#46262,.T.) ;
#62099=ORIENTED_EDGE('',*,*,#46263,.T.) ;
#62100=ORIENTED_EDGE('',*,*,#46262,.F.) ;
#62101=ORIENTED_EDGE('',*,*,#46264,.T.) ;
#62102=ORIENTED_EDGE('',*,*,#46265,.T.) ;
#62103=ORIENTED_EDGE('',*,*,#46266,.T.) ;
#62104=ORIENTED_EDGE('',*,*,#46265,.F.) ;
#62105=ORIENTED_EDGE('',*,*,#46267,.T.) ;
#62106=ORIENTED_EDGE('',*,*,#46268,.T.) ;
#62107=ORIENTED_EDGE('',*,*,#46269,.T.) ;
#62108=ORIENTED_EDGE('',*,*,#46268,.F.) ;
#62109=ORIENTED_EDGE('',*,*,#46270,.T.) ;
#62110=ORIENTED_EDGE('',*,*,#46271,.T.) ;
#62111=ORIENTED_EDGE('',*,*,#46272,.T.) ;
#62112=ORIENTED_EDGE('',*,*,#46271,.F.) ;
#62113=ORIENTED_EDGE('',*,*,#46273,.T.) ;
#62114=ORIENTED_EDGE('',*,*,#46274,.T.) ;
#62115=ORIENTED_EDGE('',*,*,#46275,.T.) ;
#62116=ORIENTED_EDGE('',*,*,#46274,.F.) ;
#62117=ORIENTED_EDGE('',*,*,#46276,.T.) ;
#62118=ORIENTED_EDGE('',*,*,#46277,.T.) ;
#62119=ORIENTED_EDGE('',*,*,#46278,.T.) ;
#62120=ORIENTED_EDGE('',*,*,#46277,.F.) ;
#62121=ORIENTED_EDGE('',*,*,#46279,.T.) ;
#62122=ORIENTED_EDGE('',*,*,#46280,.T.) ;
#62123=ORIENTED_EDGE('',*,*,#46281,.T.) ;
#62124=ORIENTED_EDGE('',*,*,#46280,.F.) ;
#62125=ORIENTED_EDGE('',*,*,#46282,.T.) ;
#62126=ORIENTED_EDGE('',*,*,#46205,.T.) ;
#62127=ORIENTED_EDGE('',*,*,#46283,.T.) ;
#62128=ORIENTED_EDGE('',*,*,#46284,.T.) ;
#62129=ORIENTED_EDGE('',*,*,#46285,.T.) ;
#62130=ORIENTED_EDGE('',*,*,#46286,.T.) ;
#62131=ORIENTED_EDGE('',*,*,#46287,.T.) ;
#62132=ORIENTED_EDGE('',*,*,#46288,.T.) ;
#62133=ORIENTED_EDGE('',*,*,#46289,.T.) ;
#62134=ORIENTED_EDGE('',*,*,#46290,.T.) ;
#62135=ORIENTED_EDGE('',*,*,#46291,.T.) ;
#62136=ORIENTED_EDGE('',*,*,#46292,.T.) ;
#62137=ORIENTED_EDGE('',*,*,#46293,.T.) ;
#62138=ORIENTED_EDGE('',*,*,#46294,.T.) ;
#62139=ORIENTED_EDGE('',*,*,#46295,.T.) ;
#62140=ORIENTED_EDGE('',*,*,#46296,.T.) ;
#62141=ORIENTED_EDGE('',*,*,#46297,.T.) ;
#62142=ORIENTED_EDGE('',*,*,#46298,.T.) ;
#62143=ORIENTED_EDGE('',*,*,#46299,.T.) ;
#62144=ORIENTED_EDGE('',*,*,#46300,.T.) ;
#62145=ORIENTED_EDGE('',*,*,#46301,.T.) ;
#62146=ORIENTED_EDGE('',*,*,#44236,.T.) ;
#62147=ORIENTED_EDGE('',*,*,#46302,.F.) ;
#62148=ORIENTED_EDGE('',*,*,#46303,.T.) ;
#62149=ORIENTED_EDGE('',*,*,#46304,.T.) ;
#62150=ORIENTED_EDGE('',*,*,#46305,.T.) ;
#62151=ORIENTED_EDGE('',*,*,#46304,.F.) ;
#62152=ORIENTED_EDGE('',*,*,#46306,.T.) ;
#62153=ORIENTED_EDGE('',*,*,#46307,.T.) ;
#62154=ORIENTED_EDGE('',*,*,#46308,.T.) ;
#62155=ORIENTED_EDGE('',*,*,#46307,.F.) ;
#62156=ORIENTED_EDGE('',*,*,#46309,.T.) ;
#62157=ORIENTED_EDGE('',*,*,#46310,.T.) ;
#62158=ORIENTED_EDGE('',*,*,#46311,.T.) ;
#62159=ORIENTED_EDGE('',*,*,#46310,.F.) ;
#62160=ORIENTED_EDGE('',*,*,#46312,.T.) ;
#62161=ORIENTED_EDGE('',*,*,#46313,.T.) ;
#62162=ORIENTED_EDGE('',*,*,#46314,.T.) ;
#62163=ORIENTED_EDGE('',*,*,#46313,.F.) ;
#62164=ORIENTED_EDGE('',*,*,#46315,.T.) ;
#62165=ORIENTED_EDGE('',*,*,#46316,.T.) ;
#62166=ORIENTED_EDGE('',*,*,#46317,.T.) ;
#62167=ORIENTED_EDGE('',*,*,#46316,.F.) ;
#62168=ORIENTED_EDGE('',*,*,#46318,.T.) ;
#62169=ORIENTED_EDGE('',*,*,#46319,.T.) ;
#62170=ORIENTED_EDGE('',*,*,#46320,.T.) ;
#62171=ORIENTED_EDGE('',*,*,#46319,.F.) ;
#62172=ORIENTED_EDGE('',*,*,#44256,.T.) ;
#62173=ORIENTED_EDGE('',*,*,#46321,.T.) ;
#62174=ORIENTED_EDGE('',*,*,#46322,.T.) ;
#62175=ORIENTED_EDGE('',*,*,#46321,.F.) ;
#62176=ORIENTED_EDGE('',*,*,#46323,.T.) ;
#62177=ORIENTED_EDGE('',*,*,#44353,.T.) ;
#62178=ORIENTED_EDGE('',*,*,#46324,.T.) ;
#62179=ORIENTED_EDGE('',*,*,#44352,.F.) ;
#62180=ORIENTED_EDGE('',*,*,#46325,.T.) ;
#62181=ORIENTED_EDGE('',*,*,#46326,.T.) ;
#62182=ORIENTED_EDGE('',*,*,#46327,.T.) ;
#62183=ORIENTED_EDGE('',*,*,#46326,.F.) ;
#62184=ORIENTED_EDGE('',*,*,#46328,.T.) ;
#62185=ORIENTED_EDGE('',*,*,#46329,.T.) ;
#62186=ORIENTED_EDGE('',*,*,#46330,.T.) ;
#62187=ORIENTED_EDGE('',*,*,#46329,.F.) ;
#62188=ORIENTED_EDGE('',*,*,#46331,.T.) ;
#62189=ORIENTED_EDGE('',*,*,#46332,.T.) ;
#62190=ORIENTED_EDGE('',*,*,#46333,.T.) ;
#62191=ORIENTED_EDGE('',*,*,#46332,.F.) ;
#62192=ORIENTED_EDGE('',*,*,#46334,.T.) ;
#62193=ORIENTED_EDGE('',*,*,#46335,.T.) ;
#62194=ORIENTED_EDGE('',*,*,#46336,.T.) ;
#62195=ORIENTED_EDGE('',*,*,#46335,.F.) ;
#62196=ORIENTED_EDGE('',*,*,#46337,.T.) ;
#62197=ORIENTED_EDGE('',*,*,#46338,.T.) ;
#62198=ORIENTED_EDGE('',*,*,#46339,.T.) ;
#62199=ORIENTED_EDGE('',*,*,#46338,.F.) ;
#62200=ORIENTED_EDGE('',*,*,#46340,.T.) ;
#62201=ORIENTED_EDGE('',*,*,#46341,.T.) ;
#62202=ORIENTED_EDGE('',*,*,#46342,.T.) ;
#62203=ORIENTED_EDGE('',*,*,#46341,.F.) ;
#62204=ORIENTED_EDGE('',*,*,#46343,.T.) ;
#62205=ORIENTED_EDGE('',*,*,#46344,.T.) ;
#62206=ORIENTED_EDGE('',*,*,#46345,.T.) ;
#62207=ORIENTED_EDGE('',*,*,#46344,.F.) ;
#62208=ORIENTED_EDGE('',*,*,#46346,.T.) ;
#62209=ORIENTED_EDGE('',*,*,#46347,.T.) ;
#62210=ORIENTED_EDGE('',*,*,#46348,.T.) ;
#62211=ORIENTED_EDGE('',*,*,#46347,.F.) ;
#62212=ORIENTED_EDGE('',*,*,#46349,.T.) ;
#62213=ORIENTED_EDGE('',*,*,#46350,.T.) ;
#62214=ORIENTED_EDGE('',*,*,#46351,.T.) ;
#62215=ORIENTED_EDGE('',*,*,#46350,.F.) ;
#62216=ORIENTED_EDGE('',*,*,#46352,.T.) ;
#62217=ORIENTED_EDGE('',*,*,#46353,.T.) ;
#62218=ORIENTED_EDGE('',*,*,#46354,.T.) ;
#62219=ORIENTED_EDGE('',*,*,#46353,.F.) ;
#62220=ORIENTED_EDGE('',*,*,#46355,.T.) ;
#62221=ORIENTED_EDGE('',*,*,#46356,.T.) ;
#62222=ORIENTED_EDGE('',*,*,#46357,.T.) ;
#62223=ORIENTED_EDGE('',*,*,#46356,.F.) ;
#62224=ORIENTED_EDGE('',*,*,#46358,.T.) ;
#62225=ORIENTED_EDGE('',*,*,#46359,.T.) ;
#62226=ORIENTED_EDGE('',*,*,#46360,.T.) ;
#62227=ORIENTED_EDGE('',*,*,#46359,.F.) ;
#62228=ORIENTED_EDGE('',*,*,#46361,.T.) ;
#62229=ORIENTED_EDGE('',*,*,#46362,.T.) ;
#62230=ORIENTED_EDGE('',*,*,#46363,.T.) ;
#62231=ORIENTED_EDGE('',*,*,#46362,.F.) ;
#62232=ORIENTED_EDGE('',*,*,#46364,.T.) ;
#62233=ORIENTED_EDGE('',*,*,#46365,.T.) ;
#62234=ORIENTED_EDGE('',*,*,#46366,.T.) ;
#62235=ORIENTED_EDGE('',*,*,#46365,.F.) ;
#62236=ORIENTED_EDGE('',*,*,#46367,.T.) ;
#62237=ORIENTED_EDGE('',*,*,#46368,.T.) ;
#62238=ORIENTED_EDGE('',*,*,#46369,.T.) ;
#62239=ORIENTED_EDGE('',*,*,#46368,.F.) ;
#62240=ORIENTED_EDGE('',*,*,#46370,.T.) ;
#62241=ORIENTED_EDGE('',*,*,#46371,.T.) ;
#62242=ORIENTED_EDGE('',*,*,#46372,.T.) ;
#62243=ORIENTED_EDGE('',*,*,#46371,.F.) ;
#62244=ORIENTED_EDGE('',*,*,#46373,.T.) ;
#62245=ORIENTED_EDGE('',*,*,#46374,.T.) ;
#62246=ORIENTED_EDGE('',*,*,#46375,.T.) ;
#62247=ORIENTED_EDGE('',*,*,#46374,.F.) ;
#62248=ORIENTED_EDGE('',*,*,#46376,.T.) ;
#62249=ORIENTED_EDGE('',*,*,#46377,.T.) ;
#62250=ORIENTED_EDGE('',*,*,#46378,.T.) ;
#62251=ORIENTED_EDGE('',*,*,#46377,.F.) ;
#62252=ORIENTED_EDGE('',*,*,#46379,.T.) ;
#62253=ORIENTED_EDGE('',*,*,#46302,.T.) ;
#62254=ORIENTED_EDGE('',*,*,#46380,.T.) ;
#62255=ORIENTED_EDGE('',*,*,#46381,.T.) ;
#62256=ORIENTED_EDGE('',*,*,#46382,.T.) ;
#62257=ORIENTED_EDGE('',*,*,#46383,.T.) ;
#62258=ORIENTED_EDGE('',*,*,#46384,.T.) ;
#62259=ORIENTED_EDGE('',*,*,#46385,.T.) ;
#62260=ORIENTED_EDGE('',*,*,#46386,.T.) ;
#62261=ORIENTED_EDGE('',*,*,#46387,.T.) ;
#62262=ORIENTED_EDGE('',*,*,#46388,.T.) ;
#62263=ORIENTED_EDGE('',*,*,#46389,.T.) ;
#62264=ORIENTED_EDGE('',*,*,#46390,.T.) ;
#62265=ORIENTED_EDGE('',*,*,#46391,.T.) ;
#62266=ORIENTED_EDGE('',*,*,#46392,.T.) ;
#62267=ORIENTED_EDGE('',*,*,#46393,.T.) ;
#62268=ORIENTED_EDGE('',*,*,#46394,.T.) ;
#62269=ORIENTED_EDGE('',*,*,#46395,.T.) ;
#62270=ORIENTED_EDGE('',*,*,#46396,.T.) ;
#62271=ORIENTED_EDGE('',*,*,#46397,.T.) ;
#62272=ORIENTED_EDGE('',*,*,#46398,.T.) ;
#62273=ORIENTED_EDGE('',*,*,#44253,.T.) ;
#62274=ORIENTED_EDGE('',*,*,#46399,.F.) ;
#62275=ORIENTED_EDGE('',*,*,#46400,.T.) ;
#62276=ORIENTED_EDGE('',*,*,#46401,.T.) ;
#62277=ORIENTED_EDGE('',*,*,#46402,.T.) ;
#62278=ORIENTED_EDGE('',*,*,#46401,.F.) ;
#62279=ORIENTED_EDGE('',*,*,#46403,.T.) ;
#62280=ORIENTED_EDGE('',*,*,#46404,.T.) ;
#62281=ORIENTED_EDGE('',*,*,#46405,.T.) ;
#62282=ORIENTED_EDGE('',*,*,#46404,.F.) ;
#62283=ORIENTED_EDGE('',*,*,#46406,.T.) ;
#62284=ORIENTED_EDGE('',*,*,#46407,.T.) ;
#62285=ORIENTED_EDGE('',*,*,#46408,.T.) ;
#62286=ORIENTED_EDGE('',*,*,#46407,.F.) ;
#62287=ORIENTED_EDGE('',*,*,#46409,.T.) ;
#62288=ORIENTED_EDGE('',*,*,#46410,.T.) ;
#62289=ORIENTED_EDGE('',*,*,#46411,.T.) ;
#62290=ORIENTED_EDGE('',*,*,#46410,.F.) ;
#62291=ORIENTED_EDGE('',*,*,#46412,.T.) ;
#62292=ORIENTED_EDGE('',*,*,#46413,.T.) ;
#62293=ORIENTED_EDGE('',*,*,#46414,.T.) ;
#62294=ORIENTED_EDGE('',*,*,#46413,.F.) ;
#62295=ORIENTED_EDGE('',*,*,#46415,.T.) ;
#62296=ORIENTED_EDGE('',*,*,#46416,.T.) ;
#62297=ORIENTED_EDGE('',*,*,#46417,.T.) ;
#62298=ORIENTED_EDGE('',*,*,#46416,.F.) ;
#62299=ORIENTED_EDGE('',*,*,#44273,.T.) ;
#62300=ORIENTED_EDGE('',*,*,#46418,.T.) ;
#62301=ORIENTED_EDGE('',*,*,#46419,.T.) ;
#62302=ORIENTED_EDGE('',*,*,#46418,.F.) ;
#62303=ORIENTED_EDGE('',*,*,#46420,.T.) ;
#62304=ORIENTED_EDGE('',*,*,#44350,.T.) ;
#62305=ORIENTED_EDGE('',*,*,#46421,.T.) ;
#62306=ORIENTED_EDGE('',*,*,#44349,.F.) ;
#62307=ORIENTED_EDGE('',*,*,#46422,.T.) ;
#62308=ORIENTED_EDGE('',*,*,#46423,.T.) ;
#62309=ORIENTED_EDGE('',*,*,#46424,.T.) ;
#62310=ORIENTED_EDGE('',*,*,#46423,.F.) ;
#62311=ORIENTED_EDGE('',*,*,#46425,.T.) ;
#62312=ORIENTED_EDGE('',*,*,#46426,.T.) ;
#62313=ORIENTED_EDGE('',*,*,#46427,.T.) ;
#62314=ORIENTED_EDGE('',*,*,#46426,.F.) ;
#62315=ORIENTED_EDGE('',*,*,#46428,.T.) ;
#62316=ORIENTED_EDGE('',*,*,#46429,.T.) ;
#62317=ORIENTED_EDGE('',*,*,#46430,.T.) ;
#62318=ORIENTED_EDGE('',*,*,#46429,.F.) ;
#62319=ORIENTED_EDGE('',*,*,#46431,.T.) ;
#62320=ORIENTED_EDGE('',*,*,#46432,.T.) ;
#62321=ORIENTED_EDGE('',*,*,#46433,.T.) ;
#62322=ORIENTED_EDGE('',*,*,#46432,.F.) ;
#62323=ORIENTED_EDGE('',*,*,#46434,.T.) ;
#62324=ORIENTED_EDGE('',*,*,#46435,.T.) ;
#62325=ORIENTED_EDGE('',*,*,#46436,.T.) ;
#62326=ORIENTED_EDGE('',*,*,#46435,.F.) ;
#62327=ORIENTED_EDGE('',*,*,#46437,.T.) ;
#62328=ORIENTED_EDGE('',*,*,#46438,.T.) ;
#62329=ORIENTED_EDGE('',*,*,#46439,.T.) ;
#62330=ORIENTED_EDGE('',*,*,#46438,.F.) ;
#62331=ORIENTED_EDGE('',*,*,#46440,.T.) ;
#62332=ORIENTED_EDGE('',*,*,#46441,.T.) ;
#62333=ORIENTED_EDGE('',*,*,#46442,.T.) ;
#62334=ORIENTED_EDGE('',*,*,#46441,.F.) ;
#62335=ORIENTED_EDGE('',*,*,#46443,.T.) ;
#62336=ORIENTED_EDGE('',*,*,#46444,.T.) ;
#62337=ORIENTED_EDGE('',*,*,#46445,.T.) ;
#62338=ORIENTED_EDGE('',*,*,#46444,.F.) ;
#62339=ORIENTED_EDGE('',*,*,#46446,.T.) ;
#62340=ORIENTED_EDGE('',*,*,#46447,.T.) ;
#62341=ORIENTED_EDGE('',*,*,#46448,.T.) ;
#62342=ORIENTED_EDGE('',*,*,#46447,.F.) ;
#62343=ORIENTED_EDGE('',*,*,#46449,.T.) ;
#62344=ORIENTED_EDGE('',*,*,#46450,.T.) ;
#62345=ORIENTED_EDGE('',*,*,#46451,.T.) ;
#62346=ORIENTED_EDGE('',*,*,#46450,.F.) ;
#62347=ORIENTED_EDGE('',*,*,#46452,.T.) ;
#62348=ORIENTED_EDGE('',*,*,#46453,.T.) ;
#62349=ORIENTED_EDGE('',*,*,#46454,.T.) ;
#62350=ORIENTED_EDGE('',*,*,#46453,.F.) ;
#62351=ORIENTED_EDGE('',*,*,#46455,.T.) ;
#62352=ORIENTED_EDGE('',*,*,#46456,.T.) ;
#62353=ORIENTED_EDGE('',*,*,#46457,.T.) ;
#62354=ORIENTED_EDGE('',*,*,#46456,.F.) ;
#62355=ORIENTED_EDGE('',*,*,#46458,.T.) ;
#62356=ORIENTED_EDGE('',*,*,#46459,.T.) ;
#62357=ORIENTED_EDGE('',*,*,#46460,.T.) ;
#62358=ORIENTED_EDGE('',*,*,#46459,.F.) ;
#62359=ORIENTED_EDGE('',*,*,#46461,.T.) ;
#62360=ORIENTED_EDGE('',*,*,#46462,.T.) ;
#62361=ORIENTED_EDGE('',*,*,#46463,.T.) ;
#62362=ORIENTED_EDGE('',*,*,#46462,.F.) ;
#62363=ORIENTED_EDGE('',*,*,#46464,.T.) ;
#62364=ORIENTED_EDGE('',*,*,#46465,.T.) ;
#62365=ORIENTED_EDGE('',*,*,#46466,.T.) ;
#62366=ORIENTED_EDGE('',*,*,#46465,.F.) ;
#62367=ORIENTED_EDGE('',*,*,#46467,.T.) ;
#62368=ORIENTED_EDGE('',*,*,#46468,.T.) ;
#62369=ORIENTED_EDGE('',*,*,#46469,.T.) ;
#62370=ORIENTED_EDGE('',*,*,#46468,.F.) ;
#62371=ORIENTED_EDGE('',*,*,#46470,.T.) ;
#62372=ORIENTED_EDGE('',*,*,#46471,.T.) ;
#62373=ORIENTED_EDGE('',*,*,#46472,.T.) ;
#62374=ORIENTED_EDGE('',*,*,#46471,.F.) ;
#62375=ORIENTED_EDGE('',*,*,#46473,.T.) ;
#62376=ORIENTED_EDGE('',*,*,#46474,.T.) ;
#62377=ORIENTED_EDGE('',*,*,#46475,.T.) ;
#62378=ORIENTED_EDGE('',*,*,#46474,.F.) ;
#62379=ORIENTED_EDGE('',*,*,#46476,.T.) ;
#62380=ORIENTED_EDGE('',*,*,#46399,.T.) ;
#62381=ORIENTED_EDGE('',*,*,#46477,.T.) ;
#62382=ORIENTED_EDGE('',*,*,#46478,.T.) ;
#62383=ORIENTED_EDGE('',*,*,#46479,.T.) ;
#62384=ORIENTED_EDGE('',*,*,#46480,.T.) ;
#62385=ORIENTED_EDGE('',*,*,#46481,.T.) ;
#62386=ORIENTED_EDGE('',*,*,#46482,.T.) ;
#62387=ORIENTED_EDGE('',*,*,#46483,.T.) ;
#62388=ORIENTED_EDGE('',*,*,#46484,.T.) ;
#62389=ORIENTED_EDGE('',*,*,#46485,.T.) ;
#62390=ORIENTED_EDGE('',*,*,#46486,.T.) ;
#62391=ORIENTED_EDGE('',*,*,#46487,.T.) ;
#62392=ORIENTED_EDGE('',*,*,#46488,.T.) ;
#62393=ORIENTED_EDGE('',*,*,#46489,.T.) ;
#62394=ORIENTED_EDGE('',*,*,#46490,.T.) ;
#62395=ORIENTED_EDGE('',*,*,#46491,.T.) ;
#62396=ORIENTED_EDGE('',*,*,#46492,.T.) ;
#62397=ORIENTED_EDGE('',*,*,#46493,.T.) ;
#62398=ORIENTED_EDGE('',*,*,#46494,.T.) ;
#62399=ORIENTED_EDGE('',*,*,#46495,.T.) ;
#62400=ORIENTED_EDGE('',*,*,#44270,.T.) ;
#62401=ORIENTED_EDGE('',*,*,#46496,.F.) ;
#62402=ORIENTED_EDGE('',*,*,#46497,.T.) ;
#62403=ORIENTED_EDGE('',*,*,#46498,.T.) ;
#62404=ORIENTED_EDGE('',*,*,#46499,.T.) ;
#62405=ORIENTED_EDGE('',*,*,#46498,.F.) ;
#62406=ORIENTED_EDGE('',*,*,#46500,.T.) ;
#62407=ORIENTED_EDGE('',*,*,#46501,.T.) ;
#62408=ORIENTED_EDGE('',*,*,#46502,.T.) ;
#62409=ORIENTED_EDGE('',*,*,#46501,.F.) ;
#62410=ORIENTED_EDGE('',*,*,#46503,.T.) ;
#62411=ORIENTED_EDGE('',*,*,#46504,.T.) ;
#62412=ORIENTED_EDGE('',*,*,#46505,.T.) ;
#62413=ORIENTED_EDGE('',*,*,#46504,.F.) ;
#62414=ORIENTED_EDGE('',*,*,#46506,.T.) ;
#62415=ORIENTED_EDGE('',*,*,#46507,.T.) ;
#62416=ORIENTED_EDGE('',*,*,#46508,.T.) ;
#62417=ORIENTED_EDGE('',*,*,#46507,.F.) ;
#62418=ORIENTED_EDGE('',*,*,#46509,.T.) ;
#62419=ORIENTED_EDGE('',*,*,#46510,.T.) ;
#62420=ORIENTED_EDGE('',*,*,#46511,.T.) ;
#62421=ORIENTED_EDGE('',*,*,#46510,.F.) ;
#62422=ORIENTED_EDGE('',*,*,#46512,.T.) ;
#62423=ORIENTED_EDGE('',*,*,#46513,.T.) ;
#62424=ORIENTED_EDGE('',*,*,#46514,.T.) ;
#62425=ORIENTED_EDGE('',*,*,#46513,.F.) ;
#62426=ORIENTED_EDGE('',*,*,#44326,.T.) ;
#62427=ORIENTED_EDGE('',*,*,#46515,.T.) ;
#62428=ORIENTED_EDGE('',*,*,#46516,.T.) ;
#62429=ORIENTED_EDGE('',*,*,#46515,.F.) ;
#62430=ORIENTED_EDGE('',*,*,#46517,.T.) ;
#62431=ORIENTED_EDGE('',*,*,#44347,.T.) ;
#62432=ORIENTED_EDGE('',*,*,#46518,.T.) ;
#62433=ORIENTED_EDGE('',*,*,#44346,.F.) ;
#62434=ORIENTED_EDGE('',*,*,#46519,.T.) ;
#62435=ORIENTED_EDGE('',*,*,#46520,.T.) ;
#62436=ORIENTED_EDGE('',*,*,#46521,.T.) ;
#62437=ORIENTED_EDGE('',*,*,#46520,.F.) ;
#62438=ORIENTED_EDGE('',*,*,#46522,.T.) ;
#62439=ORIENTED_EDGE('',*,*,#46523,.T.) ;
#62440=ORIENTED_EDGE('',*,*,#46524,.T.) ;
#62441=ORIENTED_EDGE('',*,*,#46523,.F.) ;
#62442=ORIENTED_EDGE('',*,*,#46525,.T.) ;
#62443=ORIENTED_EDGE('',*,*,#46526,.T.) ;
#62444=ORIENTED_EDGE('',*,*,#46527,.T.) ;
#62445=ORIENTED_EDGE('',*,*,#46526,.F.) ;
#62446=ORIENTED_EDGE('',*,*,#46528,.T.) ;
#62447=ORIENTED_EDGE('',*,*,#46529,.T.) ;
#62448=ORIENTED_EDGE('',*,*,#46530,.T.) ;
#62449=ORIENTED_EDGE('',*,*,#46529,.F.) ;
#62450=ORIENTED_EDGE('',*,*,#46531,.T.) ;
#62451=ORIENTED_EDGE('',*,*,#46532,.T.) ;
#62452=ORIENTED_EDGE('',*,*,#46533,.T.) ;
#62453=ORIENTED_EDGE('',*,*,#46532,.F.) ;
#62454=ORIENTED_EDGE('',*,*,#46534,.T.) ;
#62455=ORIENTED_EDGE('',*,*,#46535,.T.) ;
#62456=ORIENTED_EDGE('',*,*,#46536,.T.) ;
#62457=ORIENTED_EDGE('',*,*,#46535,.F.) ;
#62458=ORIENTED_EDGE('',*,*,#46537,.T.) ;
#62459=ORIENTED_EDGE('',*,*,#46538,.T.) ;
#62460=ORIENTED_EDGE('',*,*,#46539,.T.) ;
#62461=ORIENTED_EDGE('',*,*,#46538,.F.) ;
#62462=ORIENTED_EDGE('',*,*,#46540,.T.) ;
#62463=ORIENTED_EDGE('',*,*,#46541,.T.) ;
#62464=ORIENTED_EDGE('',*,*,#46542,.T.) ;
#62465=ORIENTED_EDGE('',*,*,#46541,.F.) ;
#62466=ORIENTED_EDGE('',*,*,#46543,.T.) ;
#62467=ORIENTED_EDGE('',*,*,#46544,.T.) ;
#62468=ORIENTED_EDGE('',*,*,#46545,.T.) ;
#62469=ORIENTED_EDGE('',*,*,#46544,.F.) ;
#62470=ORIENTED_EDGE('',*,*,#46546,.T.) ;
#62471=ORIENTED_EDGE('',*,*,#46547,.T.) ;
#62472=ORIENTED_EDGE('',*,*,#46548,.T.) ;
#62473=ORIENTED_EDGE('',*,*,#46547,.F.) ;
#62474=ORIENTED_EDGE('',*,*,#46549,.T.) ;
#62475=ORIENTED_EDGE('',*,*,#46550,.T.) ;
#62476=ORIENTED_EDGE('',*,*,#46551,.T.) ;
#62477=ORIENTED_EDGE('',*,*,#46550,.F.) ;
#62478=ORIENTED_EDGE('',*,*,#46552,.T.) ;
#62479=ORIENTED_EDGE('',*,*,#46553,.T.) ;
#62480=ORIENTED_EDGE('',*,*,#46554,.T.) ;
#62481=ORIENTED_EDGE('',*,*,#46553,.F.) ;
#62482=ORIENTED_EDGE('',*,*,#46555,.T.) ;
#62483=ORIENTED_EDGE('',*,*,#46556,.T.) ;
#62484=ORIENTED_EDGE('',*,*,#46557,.T.) ;
#62485=ORIENTED_EDGE('',*,*,#46556,.F.) ;
#62486=ORIENTED_EDGE('',*,*,#46558,.T.) ;
#62487=ORIENTED_EDGE('',*,*,#46559,.T.) ;
#62488=ORIENTED_EDGE('',*,*,#46560,.T.) ;
#62489=ORIENTED_EDGE('',*,*,#46559,.F.) ;
#62490=ORIENTED_EDGE('',*,*,#46561,.T.) ;
#62491=ORIENTED_EDGE('',*,*,#46562,.T.) ;
#62492=ORIENTED_EDGE('',*,*,#46563,.T.) ;
#62493=ORIENTED_EDGE('',*,*,#46562,.F.) ;
#62494=ORIENTED_EDGE('',*,*,#46564,.T.) ;
#62495=ORIENTED_EDGE('',*,*,#46565,.T.) ;
#62496=ORIENTED_EDGE('',*,*,#46566,.T.) ;
#62497=ORIENTED_EDGE('',*,*,#46565,.F.) ;
#62498=ORIENTED_EDGE('',*,*,#46567,.T.) ;
#62499=ORIENTED_EDGE('',*,*,#46568,.T.) ;
#62500=ORIENTED_EDGE('',*,*,#46569,.T.) ;
#62501=ORIENTED_EDGE('',*,*,#46568,.F.) ;
#62502=ORIENTED_EDGE('',*,*,#46570,.T.) ;
#62503=ORIENTED_EDGE('',*,*,#46571,.T.) ;
#62504=ORIENTED_EDGE('',*,*,#46572,.T.) ;
#62505=ORIENTED_EDGE('',*,*,#46571,.F.) ;
#62506=ORIENTED_EDGE('',*,*,#46573,.T.) ;
#62507=ORIENTED_EDGE('',*,*,#46496,.T.) ;
#62508=ORIENTED_EDGE('',*,*,#46574,.T.) ;
#62509=ORIENTED_EDGE('',*,*,#46575,.T.) ;
#62510=ORIENTED_EDGE('',*,*,#46576,.T.) ;
#62511=ORIENTED_EDGE('',*,*,#46577,.T.) ;
#62512=ORIENTED_EDGE('',*,*,#46578,.T.) ;
#62513=ORIENTED_EDGE('',*,*,#46579,.T.) ;
#62514=ORIENTED_EDGE('',*,*,#46580,.T.) ;
#62515=ORIENTED_EDGE('',*,*,#46581,.T.) ;
#62516=ORIENTED_EDGE('',*,*,#46582,.T.) ;
#62517=ORIENTED_EDGE('',*,*,#46583,.T.) ;
#62518=ORIENTED_EDGE('',*,*,#46584,.T.) ;
#62519=ORIENTED_EDGE('',*,*,#46585,.T.) ;
#62520=ORIENTED_EDGE('',*,*,#46586,.T.) ;
#62521=ORIENTED_EDGE('',*,*,#46587,.T.) ;
#62522=ORIENTED_EDGE('',*,*,#46588,.T.) ;
#62523=ORIENTED_EDGE('',*,*,#46589,.T.) ;
#62524=ORIENTED_EDGE('',*,*,#46590,.T.) ;
#62525=ORIENTED_EDGE('',*,*,#46591,.T.) ;
#62526=ORIENTED_EDGE('',*,*,#46592,.T.) ;
#62527=ORIENTED_EDGE('',*,*,#44323,.T.) ;
#62528=ORIENTED_EDGE('',*,*,#44283,.T.) ;
#62529=ORIENTED_EDGE('',*,*,#46593,.F.) ;
#62530=ORIENTED_EDGE('',*,*,#46594,.T.) ;
#62531=ORIENTED_EDGE('',*,*,#46595,.T.) ;
#62532=ORIENTED_EDGE('',*,*,#46596,.T.) ;
#62533=ORIENTED_EDGE('',*,*,#46597,.T.) ;
#62534=ORIENTED_EDGE('',*,*,#46598,.T.) ;
#62535=ORIENTED_EDGE('',*,*,#46599,.T.) ;
#62536=ORIENTED_EDGE('',*,*,#46600,.T.) ;
#62537=ORIENTED_EDGE('',*,*,#44266,.T.) ;
#62538=ORIENTED_EDGE('',*,*,#46601,.F.) ;
#62539=ORIENTED_EDGE('',*,*,#46602,.T.) ;
#62540=ORIENTED_EDGE('',*,*,#46603,.T.) ;
#62541=ORIENTED_EDGE('',*,*,#46604,.T.) ;
#62542=ORIENTED_EDGE('',*,*,#46605,.T.) ;
#62543=ORIENTED_EDGE('',*,*,#46606,.T.) ;
#62544=ORIENTED_EDGE('',*,*,#46607,.T.) ;
#62545=ORIENTED_EDGE('',*,*,#46608,.T.) ;
#62546=ORIENTED_EDGE('',*,*,#44249,.T.) ;
#62547=ORIENTED_EDGE('',*,*,#46609,.F.) ;
#62548=ORIENTED_EDGE('',*,*,#46610,.T.) ;
#62549=ORIENTED_EDGE('',*,*,#46611,.T.) ;
#62550=ORIENTED_EDGE('',*,*,#46612,.T.) ;
#62551=ORIENTED_EDGE('',*,*,#46613,.T.) ;
#62552=ORIENTED_EDGE('',*,*,#46614,.T.) ;
#62553=ORIENTED_EDGE('',*,*,#46615,.T.) ;
#62554=ORIENTED_EDGE('',*,*,#46616,.T.) ;
#62555=ORIENTED_EDGE('',*,*,#44232,.T.) ;
#62556=ORIENTED_EDGE('',*,*,#46617,.F.) ;
#62557=ORIENTED_EDGE('',*,*,#46618,.T.) ;
#62558=ORIENTED_EDGE('',*,*,#46619,.T.) ;
#62559=ORIENTED_EDGE('',*,*,#46620,.T.) ;
#62560=ORIENTED_EDGE('',*,*,#46621,.T.) ;
#62561=ORIENTED_EDGE('',*,*,#46622,.T.) ;
#62562=ORIENTED_EDGE('',*,*,#46623,.T.) ;
#62563=ORIENTED_EDGE('',*,*,#46624,.T.) ;
#62564=ORIENTED_EDGE('',*,*,#44215,.T.) ;
#62565=ORIENTED_EDGE('',*,*,#46625,.F.) ;
#62566=ORIENTED_EDGE('',*,*,#46626,.T.) ;
#62567=ORIENTED_EDGE('',*,*,#46627,.T.) ;
#62568=ORIENTED_EDGE('',*,*,#46628,.T.) ;
#62569=ORIENTED_EDGE('',*,*,#46629,.T.) ;
#62570=ORIENTED_EDGE('',*,*,#46630,.T.) ;
#62571=ORIENTED_EDGE('',*,*,#46631,.T.) ;
#62572=ORIENTED_EDGE('',*,*,#46632,.T.) ;
#62573=ORIENTED_EDGE('',*,*,#44198,.T.) ;
#62574=ORIENTED_EDGE('',*,*,#46633,.F.) ;
#62575=ORIENTED_EDGE('',*,*,#46634,.T.) ;
#62576=ORIENTED_EDGE('',*,*,#46635,.T.) ;
#62577=ORIENTED_EDGE('',*,*,#46636,.T.) ;
#62578=ORIENTED_EDGE('',*,*,#46637,.T.) ;
#62579=ORIENTED_EDGE('',*,*,#46638,.T.) ;
#62580=ORIENTED_EDGE('',*,*,#46639,.T.) ;
#62581=ORIENTED_EDGE('',*,*,#46640,.T.) ;
#62582=ORIENTED_EDGE('',*,*,#44181,.T.) ;
#62583=ORIENTED_EDGE('',*,*,#46641,.F.) ;
#62584=ORIENTED_EDGE('',*,*,#46642,.T.) ;
#62585=ORIENTED_EDGE('',*,*,#46643,.T.) ;
#62586=ORIENTED_EDGE('',*,*,#46644,.T.) ;
#62587=ORIENTED_EDGE('',*,*,#46645,.T.) ;
#62588=ORIENTED_EDGE('',*,*,#46646,.T.) ;
#62589=ORIENTED_EDGE('',*,*,#46647,.T.) ;
#62590=ORIENTED_EDGE('',*,*,#46648,.T.) ;
#62591=ORIENTED_EDGE('',*,*,#44164,.T.) ;
#62592=ORIENTED_EDGE('',*,*,#46649,.F.) ;
#62593=ORIENTED_EDGE('',*,*,#46650,.T.) ;
#62594=ORIENTED_EDGE('',*,*,#46651,.T.) ;
#62595=ORIENTED_EDGE('',*,*,#46652,.T.) ;
#62596=ORIENTED_EDGE('',*,*,#46653,.T.) ;
#62597=ORIENTED_EDGE('',*,*,#46654,.T.) ;
#62598=ORIENTED_EDGE('',*,*,#46655,.T.) ;
#62599=ORIENTED_EDGE('',*,*,#46656,.T.) ;
#62600=ORIENTED_EDGE('',*,*,#44147,.T.) ;
#62601=ORIENTED_EDGE('',*,*,#46657,.F.) ;
#62602=ORIENTED_EDGE('',*,*,#46658,.T.) ;
#62603=ORIENTED_EDGE('',*,*,#46659,.T.) ;
#62604=ORIENTED_EDGE('',*,*,#46660,.T.) ;
#62605=ORIENTED_EDGE('',*,*,#46661,.T.) ;
#62606=ORIENTED_EDGE('',*,*,#46662,.T.) ;
#62607=ORIENTED_EDGE('',*,*,#46663,.T.) ;
#62608=ORIENTED_EDGE('',*,*,#46664,.T.) ;
#62609=ORIENTED_EDGE('',*,*,#46665,.F.) ;
#62610=ORIENTED_EDGE('',*,*,#45561,.F.) ;
#62611=ORIENTED_EDGE('',*,*,#46666,.F.) ;
#62612=ORIENTED_EDGE('',*,*,#45548,.F.) ;
#62613=ORIENTED_EDGE('',*,*,#46667,.F.) ;
#62614=ORIENTED_EDGE('',*,*,#45562,.F.) ;
#62615=ORIENTED_EDGE('',*,*,#46668,.F.) ;
#62616=ORIENTED_EDGE('',*,*,#45556,.F.) ;
#62617=ORIENTED_EDGE('',*,*,#46669,.F.) ;
#62618=ORIENTED_EDGE('',*,*,#46667,.T.) ;
#62619=ORIENTED_EDGE('',*,*,#46670,.F.) ;
#62620=ORIENTED_EDGE('',*,*,#46671,.F.) ;
#62621=ORIENTED_EDGE('',*,*,#46666,.T.) ;
#62622=ORIENTED_EDGE('',*,*,#46672,.F.) ;
#62623=ORIENTED_EDGE('',*,*,#46665,.T.) ;
#62624=ORIENTED_EDGE('',*,*,#45547,.T.) ;
#62625=ORIENTED_EDGE('',*,*,#46673,.F.) ;
#62626=ORIENTED_EDGE('',*,*,#46668,.T.) ;
#62627=ORIENTED_EDGE('',*,*,#46670,.T.) ;
#62628=ORIENTED_EDGE('',*,*,#45559,.F.) ;
#62629=ORIENTED_EDGE('',*,*,#46674,.F.) ;
#62630=ORIENTED_EDGE('',*,*,#44329,.T.) ;
#62631=ORIENTED_EDGE('',*,*,#46675,.T.) ;
#62632=ORIENTED_EDGE('',*,*,#46676,.F.) ;
#62633=ORIENTED_EDGE('',*,*,#46669,.T.) ;
#62634=ORIENTED_EDGE('',*,*,#46677,.F.) ;
#62635=ORIENTED_EDGE('',*,*,#46678,.T.) ;
#62636=ORIENTED_EDGE('',*,*,#46679,.F.) ;
#62637=ORIENTED_EDGE('',*,*,#44485,.F.) ;
#62638=ORIENTED_EDGE('',*,*,#46680,.F.) ;
#62639=ORIENTED_EDGE('',*,*,#45563,.F.) ;
#62640=ORIENTED_EDGE('',*,*,#46672,.T.) ;
#62641=ORIENTED_EDGE('',*,*,#45560,.F.) ;
#62642=ORIENTED_EDGE('',*,*,#46681,.F.) ;
#62643=ORIENTED_EDGE('',*,*,#45566,.F.) ;
#62644=ORIENTED_EDGE('',*,*,#46671,.T.) ;
#62645=ORIENTED_EDGE('',*,*,#45565,.F.) ;
#62646=ORIENTED_EDGE('',*,*,#46682,.F.) ;
#62647=ORIENTED_EDGE('',*,*,#45539,.F.) ;
#62648=ORIENTED_EDGE('',*,*,#46673,.T.) ;
#62649=ORIENTED_EDGE('',*,*,#45546,.F.) ;
#62650=ORIENTED_EDGE('',*,*,#46683,.F.) ;
#62651=ORIENTED_EDGE('',*,*,#45557,.F.) ;
#62652=ORIENTED_EDGE('',*,*,#46684,.F.) ;
#62653=ORIENTED_EDGE('',*,*,#45558,.F.) ;
#62654=ORIENTED_EDGE('',*,*,#46685,.F.) ;
#62655=ORIENTED_EDGE('',*,*,#45553,.F.) ;
#62656=ORIENTED_EDGE('',*,*,#46674,.T.) ;
#62657=ORIENTED_EDGE('',*,*,#46684,.T.) ;
#62658=ORIENTED_EDGE('',*,*,#44330,.F.) ;
#62659=ORIENTED_EDGE('',*,*,#46680,.T.) ;
#62660=ORIENTED_EDGE('',*,*,#44495,.T.) ;
#62661=ORIENTED_EDGE('',*,*,#46686,.F.) ;
#62662=ORIENTED_EDGE('',*,*,#46681,.T.) ;
#62663=ORIENTED_EDGE('',*,*,#46687,.F.) ;
#62664=ORIENTED_EDGE('',*,*,#46682,.T.) ;
#62665=ORIENTED_EDGE('',*,*,#46688,.F.) ;
#62666=ORIENTED_EDGE('',*,*,#44581,.T.) ;
#62667=ORIENTED_EDGE('',*,*,#46683,.T.) ;
#62668=ORIENTED_EDGE('',*,*,#45545,.T.) ;
#62669=ORIENTED_EDGE('',*,*,#46689,.F.) ;
#62670=ORIENTED_EDGE('',*,*,#46685,.T.) ;
#62671=ORIENTED_EDGE('',*,*,#46686,.T.) ;
#62672=ORIENTED_EDGE('',*,*,#44494,.F.) ;
#62673=ORIENTED_EDGE('',*,*,#46690,.F.) ;
#62674=ORIENTED_EDGE('',*,*,#45567,.F.) ;
#62675=ORIENTED_EDGE('',*,*,#46688,.T.) ;
#62676=ORIENTED_EDGE('',*,*,#45564,.F.) ;
#62677=ORIENTED_EDGE('',*,*,#46691,.F.) ;
#62678=ORIENTED_EDGE('',*,*,#44582,.F.) ;
#62679=ORIENTED_EDGE('',*,*,#45540,.F.) ;
#62680=ORIENTED_EDGE('',*,*,#46687,.T.) ;
#62681=ORIENTED_EDGE('',*,*,#46692,.F.) ;
#62682=ORIENTED_EDGE('',*,*,#46693,.F.) ;
#62683=ORIENTED_EDGE('',*,*,#46689,.T.) ;
#62684=ORIENTED_EDGE('',*,*,#45544,.F.) ;
#62685=ORIENTED_EDGE('',*,*,#46694,.F.) ;
#62686=ORIENTED_EDGE('',*,*,#45554,.F.) ;
#62687=ORIENTED_EDGE('',*,*,#46695,.F.) ;
#62688=ORIENTED_EDGE('',*,*,#45555,.F.) ;
#62689=ORIENTED_EDGE('',*,*,#46696,.F.) ;
#62690=ORIENTED_EDGE('',*,*,#45549,.F.) ;
#62691=ORIENTED_EDGE('',*,*,#44332,.T.) ;
#62692=ORIENTED_EDGE('',*,*,#46695,.T.) ;
#62693=ORIENTED_EDGE('',*,*,#46697,.F.) ;
#62694=ORIENTED_EDGE('',*,*,#44489,.T.) ;
#62695=ORIENTED_EDGE('',*,*,#46691,.T.) ;
#62696=ORIENTED_EDGE('',*,*,#46690,.T.) ;
#62697=ORIENTED_EDGE('',*,*,#46698,.F.) ;
#62698=ORIENTED_EDGE('',*,*,#46699,.F.) ;
#62699=ORIENTED_EDGE('',*,*,#44587,.F.) ;
#62700=ORIENTED_EDGE('',*,*,#46700,.F.) ;
#62701=ORIENTED_EDGE('',*,*,#46701,.F.) ;
#62702=ORIENTED_EDGE('',*,*,#46692,.T.) ;
#62703=ORIENTED_EDGE('',*,*,#44585,.F.) ;
#62704=ORIENTED_EDGE('',*,*,#46700,.T.) ;
#62705=ORIENTED_EDGE('',*,*,#44748,.F.) ;
#62706=ORIENTED_EDGE('',*,*,#46693,.T.) ;
#62707=ORIENTED_EDGE('',*,*,#46702,.F.) ;
#62708=ORIENTED_EDGE('',*,*,#46703,.F.) ;
#62709=ORIENTED_EDGE('',*,*,#46696,.T.) ;
#62710=ORIENTED_EDGE('',*,*,#46694,.T.) ;
#62711=ORIENTED_EDGE('',*,*,#46704,.F.) ;
#62712=ORIENTED_EDGE('',*,*,#46697,.T.) ;
#62713=ORIENTED_EDGE('',*,*,#45552,.F.) ;
#62714=ORIENTED_EDGE('',*,*,#46705,.F.) ;
#62715=ORIENTED_EDGE('',*,*,#44490,.F.) ;
#62716=ORIENTED_EDGE('',*,*,#46698,.T.) ;
#62717=ORIENTED_EDGE('',*,*,#44493,.F.) ;
#62718=ORIENTED_EDGE('',*,*,#46706,.F.) ;
#62719=ORIENTED_EDGE('',*,*,#44583,.F.) ;
#62720=ORIENTED_EDGE('',*,*,#46699,.T.) ;
#62721=ORIENTED_EDGE('',*,*,#44584,.F.) ;
#62722=ORIENTED_EDGE('',*,*,#46707,.F.) ;
#62723=ORIENTED_EDGE('',*,*,#44661,.F.) ;
#62724=ORIENTED_EDGE('',*,*,#46701,.T.) ;
#62725=ORIENTED_EDGE('',*,*,#44747,.T.) ;
#62726=ORIENTED_EDGE('',*,*,#46708,.F.) ;
#62727=ORIENTED_EDGE('',*,*,#46702,.T.) ;
#62728=ORIENTED_EDGE('',*,*,#45541,.F.) ;
#62729=ORIENTED_EDGE('',*,*,#46703,.T.) ;
#62730=ORIENTED_EDGE('',*,*,#46709,.F.) ;
#62731=ORIENTED_EDGE('',*,*,#46710,.F.) ;
#62732=ORIENTED_EDGE('',*,*,#46704,.T.) ;
#62733=ORIENTED_EDGE('',*,*,#45543,.F.) ;
#62734=ORIENTED_EDGE('',*,*,#46711,.F.) ;
#62735=ORIENTED_EDGE('',*,*,#45550,.F.) ;
#62736=ORIENTED_EDGE('',*,*,#46712,.F.) ;
#62737=ORIENTED_EDGE('',*,*,#45551,.F.) ;
#62738=ORIENTED_EDGE('',*,*,#46713,.F.) ;
#62739=ORIENTED_EDGE('',*,*,#44580,.F.) ;
#62740=ORIENTED_EDGE('',*,*,#46705,.T.) ;
#62741=ORIENTED_EDGE('',*,*,#46712,.T.) ;
#62742=ORIENTED_EDGE('',*,*,#46714,.F.) ;
#62743=ORIENTED_EDGE('',*,*,#46707,.T.) ;
#62744=ORIENTED_EDGE('',*,*,#46706,.T.) ;
#62745=ORIENTED_EDGE('',*,*,#46715,.F.) ;
#62746=ORIENTED_EDGE('',*,*,#44662,.T.) ;
#62747=ORIENTED_EDGE('',*,*,#46716,.F.) ;
#62748=ORIENTED_EDGE('',*,*,#46709,.T.) ;
#62749=ORIENTED_EDGE('',*,*,#46708,.T.) ;
#62750=ORIENTED_EDGE('',*,*,#44746,.F.) ;
#62751=ORIENTED_EDGE('',*,*,#46710,.T.) ;
#62752=ORIENTED_EDGE('',*,*,#46717,.F.) ;
#62753=ORIENTED_EDGE('',*,*,#46718,.F.) ;
#62754=ORIENTED_EDGE('',*,*,#46713,.T.) ;
#62755=ORIENTED_EDGE('',*,*,#46711,.T.) ;
#62756=ORIENTED_EDGE('',*,*,#46719,.F.) ;
#62757=ORIENTED_EDGE('',*,*,#44576,.T.) ;
#62758=ORIENTED_EDGE('',*,*,#46714,.T.) ;
#62759=ORIENTED_EDGE('',*,*,#44579,.F.) ;
#62760=ORIENTED_EDGE('',*,*,#46720,.F.) ;
#62761=ORIENTED_EDGE('',*,*,#44491,.F.) ;
#62762=ORIENTED_EDGE('',*,*,#46715,.T.) ;
#62763=ORIENTED_EDGE('',*,*,#44492,.F.) ;
#62764=ORIENTED_EDGE('',*,*,#46721,.F.) ;
#62765=ORIENTED_EDGE('',*,*,#44663,.F.) ;
#62766=ORIENTED_EDGE('',*,*,#46716,.T.) ;
#62767=ORIENTED_EDGE('',*,*,#44745,.T.) ;
#62768=ORIENTED_EDGE('',*,*,#46722,.F.) ;
#62769=ORIENTED_EDGE('',*,*,#46717,.T.) ;
#62770=ORIENTED_EDGE('',*,*,#45542,.F.) ;
#62771=ORIENTED_EDGE('',*,*,#46718,.T.) ;
#62772=ORIENTED_EDGE('',*,*,#46723,.F.) ;
#62773=ORIENTED_EDGE('',*,*,#46719,.T.) ;
#62774=ORIENTED_EDGE('',*,*,#46721,.T.) ;
#62775=ORIENTED_EDGE('',*,*,#46720,.T.) ;
#62776=ORIENTED_EDGE('',*,*,#46724,.F.) ;
#62777=ORIENTED_EDGE('',*,*,#44664,.T.) ;
#62778=ORIENTED_EDGE('',*,*,#46722,.T.) ;
#62779=ORIENTED_EDGE('',*,*,#44744,.F.) ;
#62780=ORIENTED_EDGE('',*,*,#46725,.F.) ;
#62781=ORIENTED_EDGE('',*,*,#44577,.F.) ;
#62782=ORIENTED_EDGE('',*,*,#46723,.T.) ;
#62783=ORIENTED_EDGE('',*,*,#46724,.T.) ;
#62784=ORIENTED_EDGE('',*,*,#44578,.F.) ;
#62785=ORIENTED_EDGE('',*,*,#46726,.F.) ;
#62786=ORIENTED_EDGE('',*,*,#44665,.F.) ;
#62787=ORIENTED_EDGE('',*,*,#46725,.T.) ;
#62788=ORIENTED_EDGE('',*,*,#44593,.F.) ;
#62789=ORIENTED_EDGE('',*,*,#46726,.T.) ;
#62790=ORIENTED_EDGE('',*,*,#46727,.F.) ;
#62791=ORIENTED_EDGE('',*,*,#46537,.F.) ;
#62792=ORIENTED_EDGE('',*,*,#46728,.F.) ;
#62793=ORIENTED_EDGE('',*,*,#46584,.F.) ;
#62794=ORIENTED_EDGE('',*,*,#46728,.T.) ;
#62795=ORIENTED_EDGE('',*,*,#46534,.F.) ;
#62796=ORIENTED_EDGE('',*,*,#46729,.F.) ;
#62797=ORIENTED_EDGE('',*,*,#46585,.F.) ;
#62798=ORIENTED_EDGE('',*,*,#46540,.F.) ;
#62799=ORIENTED_EDGE('',*,*,#46727,.T.) ;
#62800=ORIENTED_EDGE('',*,*,#46730,.F.) ;
#62801=ORIENTED_EDGE('',*,*,#46729,.T.) ;
#62802=ORIENTED_EDGE('',*,*,#46531,.F.) ;
#62803=ORIENTED_EDGE('',*,*,#46731,.F.) ;
#62804=ORIENTED_EDGE('',*,*,#46586,.F.) ;
#62805=ORIENTED_EDGE('',*,*,#46730,.T.) ;
#62806=ORIENTED_EDGE('',*,*,#46583,.F.) ;
#62807=ORIENTED_EDGE('',*,*,#46732,.F.) ;
#62808=ORIENTED_EDGE('',*,*,#46543,.F.) ;
#62809=ORIENTED_EDGE('',*,*,#46731,.T.) ;
#62810=ORIENTED_EDGE('',*,*,#46528,.F.) ;
#62811=ORIENTED_EDGE('',*,*,#46733,.F.) ;
#62812=ORIENTED_EDGE('',*,*,#46587,.F.) ;
#62813=ORIENTED_EDGE('',*,*,#46546,.F.) ;
#62814=ORIENTED_EDGE('',*,*,#46732,.T.) ;
#62815=ORIENTED_EDGE('',*,*,#46734,.F.) ;
#62816=ORIENTED_EDGE('',*,*,#46733,.T.) ;
#62817=ORIENTED_EDGE('',*,*,#46525,.F.) ;
#62818=ORIENTED_EDGE('',*,*,#46735,.F.) ;
#62819=ORIENTED_EDGE('',*,*,#46588,.F.) ;
#62820=ORIENTED_EDGE('',*,*,#46734,.T.) ;
#62821=ORIENTED_EDGE('',*,*,#46582,.F.) ;
#62822=ORIENTED_EDGE('',*,*,#46736,.F.) ;
#62823=ORIENTED_EDGE('',*,*,#46549,.F.) ;
#62824=ORIENTED_EDGE('',*,*,#46735,.T.) ;
#62825=ORIENTED_EDGE('',*,*,#46522,.F.) ;
#62826=ORIENTED_EDGE('',*,*,#46737,.F.) ;
#62827=ORIENTED_EDGE('',*,*,#46552,.F.) ;
#62828=ORIENTED_EDGE('',*,*,#46736,.T.) ;
#62829=ORIENTED_EDGE('',*,*,#46738,.F.) ;
#62830=ORIENTED_EDGE('',*,*,#46737,.T.) ;
#62831=ORIENTED_EDGE('',*,*,#46519,.F.) ;
#62832=ORIENTED_EDGE('',*,*,#46739,.F.) ;
#62833=ORIENTED_EDGE('',*,*,#46589,.F.) ;
#62834=ORIENTED_EDGE('',*,*,#46738,.T.) ;
#62835=ORIENTED_EDGE('',*,*,#46581,.F.) ;
#62836=ORIENTED_EDGE('',*,*,#46740,.F.) ;
#62837=ORIENTED_EDGE('',*,*,#46555,.F.) ;
#62838=ORIENTED_EDGE('',*,*,#46739,.T.) ;
#62839=ORIENTED_EDGE('',*,*,#44345,.F.) ;
#62840=ORIENTED_EDGE('',*,*,#46741,.F.) ;
#62841=ORIENTED_EDGE('',*,*,#46558,.F.) ;
#62842=ORIENTED_EDGE('',*,*,#46740,.T.) ;
#62843=ORIENTED_EDGE('',*,*,#46742,.F.) ;
#62844=ORIENTED_EDGE('',*,*,#46741,.T.) ;
#62845=ORIENTED_EDGE('',*,*,#46517,.F.) ;
#62846=ORIENTED_EDGE('',*,*,#44328,.F.) ;
#62847=ORIENTED_EDGE('',*,*,#46590,.F.) ;
#62848=ORIENTED_EDGE('',*,*,#46742,.T.) ;
#62849=ORIENTED_EDGE('',*,*,#46580,.F.) ;
#62850=ORIENTED_EDGE('',*,*,#46743,.F.) ;
#62851=ORIENTED_EDGE('',*,*,#46561,.F.) ;
#62852=ORIENTED_EDGE('',*,*,#46564,.F.) ;
#62853=ORIENTED_EDGE('',*,*,#46743,.T.) ;
#62854=ORIENTED_EDGE('',*,*,#46744,.F.) ;
#62855=ORIENTED_EDGE('',*,*,#44327,.T.) ;
#62856=ORIENTED_EDGE('',*,*,#46512,.F.) ;
#62857=ORIENTED_EDGE('',*,*,#46745,.F.) ;
#62858=ORIENTED_EDGE('',*,*,#46591,.F.) ;
#62859=ORIENTED_EDGE('',*,*,#46744,.T.) ;
#62860=ORIENTED_EDGE('',*,*,#46579,.F.) ;
#62861=ORIENTED_EDGE('',*,*,#46746,.F.) ;
#62862=ORIENTED_EDGE('',*,*,#46567,.F.) ;
#62863=ORIENTED_EDGE('',*,*,#46745,.T.) ;
#62864=ORIENTED_EDGE('',*,*,#46509,.F.) ;
#62865=ORIENTED_EDGE('',*,*,#46747,.F.) ;
#62866=ORIENTED_EDGE('',*,*,#46570,.F.) ;
#62867=ORIENTED_EDGE('',*,*,#46746,.T.) ;
#62868=ORIENTED_EDGE('',*,*,#46748,.F.) ;
#62869=ORIENTED_EDGE('',*,*,#46747,.T.) ;
#62870=ORIENTED_EDGE('',*,*,#46506,.F.) ;
#62871=ORIENTED_EDGE('',*,*,#46749,.F.) ;
#62872=ORIENTED_EDGE('',*,*,#46592,.F.) ;
#62873=ORIENTED_EDGE('',*,*,#46748,.T.) ;
#62874=ORIENTED_EDGE('',*,*,#46578,.F.) ;
#62875=ORIENTED_EDGE('',*,*,#46750,.F.) ;
#62876=ORIENTED_EDGE('',*,*,#46573,.F.) ;
#62877=ORIENTED_EDGE('',*,*,#46749,.T.) ;
#62878=ORIENTED_EDGE('',*,*,#46503,.F.) ;
#62879=ORIENTED_EDGE('',*,*,#46751,.F.) ;
#62880=ORIENTED_EDGE('',*,*,#46575,.F.) ;
#62881=ORIENTED_EDGE('',*,*,#46750,.T.) ;
#62882=ORIENTED_EDGE('',*,*,#46577,.F.) ;
#62883=ORIENTED_EDGE('',*,*,#46752,.F.) ;
#62884=ORIENTED_EDGE('',*,*,#46497,.F.) ;
#62885=ORIENTED_EDGE('',*,*,#46751,.T.) ;
#62886=ORIENTED_EDGE('',*,*,#46500,.F.) ;
#62887=ORIENTED_EDGE('',*,*,#46752,.T.) ;
#62888=ORIENTED_EDGE('',*,*,#46576,.F.) ;
#62889=ORIENTED_EDGE('',*,*,#46753,.F.) ;
#62890=ORIENTED_EDGE('',*,*,#45757,.F.) ;
#62891=ORIENTED_EDGE('',*,*,#46754,.F.) ;
#62892=ORIENTED_EDGE('',*,*,#44806,.F.) ;
#62893=ORIENTED_EDGE('',*,*,#45754,.F.) ;
#62894=ORIENTED_EDGE('',*,*,#46753,.T.) ;
#62895=ORIENTED_EDGE('',*,*,#46755,.F.) ;
#62896=ORIENTED_EDGE('',*,*,#46754,.T.) ;
#62897=ORIENTED_EDGE('',*,*,#45760,.F.) ;
#62898=ORIENTED_EDGE('',*,*,#46756,.F.) ;
#62899=ORIENTED_EDGE('',*,*,#46755,.T.) ;
#62900=ORIENTED_EDGE('',*,*,#44805,.F.) ;
#62901=ORIENTED_EDGE('',*,*,#46757,.F.) ;
#62902=ORIENTED_EDGE('',*,*,#45751,.F.) ;
#62903=ORIENTED_EDGE('',*,*,#46756,.T.) ;
#62904=ORIENTED_EDGE('',*,*,#45763,.F.) ;
#62905=ORIENTED_EDGE('',*,*,#46758,.F.) ;
#62906=ORIENTED_EDGE('',*,*,#44807,.F.) ;
#62907=ORIENTED_EDGE('',*,*,#46757,.T.) ;
#62908=ORIENTED_EDGE('',*,*,#44804,.F.) ;
#62909=ORIENTED_EDGE('',*,*,#46759,.F.) ;
#62910=ORIENTED_EDGE('',*,*,#45748,.F.) ;
#62911=ORIENTED_EDGE('',*,*,#46758,.T.) ;
#62912=ORIENTED_EDGE('',*,*,#45766,.F.) ;
#62913=ORIENTED_EDGE('',*,*,#46760,.F.) ;
#62914=ORIENTED_EDGE('',*,*,#44808,.F.) ;
#62915=ORIENTED_EDGE('',*,*,#46759,.T.) ;
#62916=ORIENTED_EDGE('',*,*,#44803,.F.) ;
#62917=ORIENTED_EDGE('',*,*,#44322,.F.) ;
#62918=ORIENTED_EDGE('',*,*,#45745,.F.) ;
#62919=ORIENTED_EDGE('',*,*,#46760,.T.) ;
#62920=ORIENTED_EDGE('',*,*,#45769,.F.) ;
#62921=ORIENTED_EDGE('',*,*,#46761,.F.) ;
#62922=ORIENTED_EDGE('',*,*,#44809,.F.) ;
#62923=ORIENTED_EDGE('',*,*,#46761,.T.) ;
#62924=ORIENTED_EDGE('',*,*,#45772,.F.) ;
#62925=ORIENTED_EDGE('',*,*,#46762,.F.) ;
#62926=ORIENTED_EDGE('',*,*,#44810,.F.) ;
#62927=ORIENTED_EDGE('',*,*,#44320,.T.) ;
#62928=ORIENTED_EDGE('',*,*,#44802,.F.) ;
#62929=ORIENTED_EDGE('',*,*,#46763,.F.) ;
#62930=ORIENTED_EDGE('',*,*,#45742,.F.) ;
#62931=ORIENTED_EDGE('',*,*,#46762,.T.) ;
#62932=ORIENTED_EDGE('',*,*,#45775,.F.) ;
#62933=ORIENTED_EDGE('',*,*,#46764,.F.) ;
#62934=ORIENTED_EDGE('',*,*,#44811,.F.) ;
#62935=ORIENTED_EDGE('',*,*,#46763,.T.) ;
#62936=ORIENTED_EDGE('',*,*,#44801,.F.) ;
#62937=ORIENTED_EDGE('',*,*,#46765,.F.) ;
#62938=ORIENTED_EDGE('',*,*,#45740,.F.) ;
#62939=ORIENTED_EDGE('',*,*,#46764,.T.) ;
#62940=ORIENTED_EDGE('',*,*,#45778,.F.) ;
#62941=ORIENTED_EDGE('',*,*,#46766,.F.) ;
#62942=ORIENTED_EDGE('',*,*,#44812,.F.) ;
#62943=ORIENTED_EDGE('',*,*,#46765,.T.) ;
#62944=ORIENTED_EDGE('',*,*,#44800,.F.) ;
#62945=ORIENTED_EDGE('',*,*,#46767,.F.) ;
#62946=ORIENTED_EDGE('',*,*,#45738,.F.) ;
#62947=ORIENTED_EDGE('',*,*,#46766,.T.) ;
#62948=ORIENTED_EDGE('',*,*,#45781,.F.) ;
#62949=ORIENTED_EDGE('',*,*,#46768,.F.) ;
#62950=ORIENTED_EDGE('',*,*,#44813,.F.) ;
#62951=ORIENTED_EDGE('',*,*,#46767,.T.) ;
#62952=ORIENTED_EDGE('',*,*,#44799,.F.) ;
#62953=ORIENTED_EDGE('',*,*,#46769,.F.) ;
#62954=ORIENTED_EDGE('',*,*,#45735,.F.) ;
#62955=ORIENTED_EDGE('',*,*,#46768,.T.) ;
#62956=ORIENTED_EDGE('',*,*,#45784,.F.) ;
#62957=ORIENTED_EDGE('',*,*,#46770,.F.) ;
#62958=ORIENTED_EDGE('',*,*,#44814,.F.) ;
#62959=ORIENTED_EDGE('',*,*,#46769,.T.) ;
#62960=ORIENTED_EDGE('',*,*,#44798,.F.) ;
#62961=ORIENTED_EDGE('',*,*,#46771,.F.) ;
#62962=ORIENTED_EDGE('',*,*,#45732,.F.) ;
#62963=ORIENTED_EDGE('',*,*,#46770,.T.) ;
#62964=ORIENTED_EDGE('',*,*,#45787,.F.) ;
#62965=ORIENTED_EDGE('',*,*,#46772,.F.) ;
#62966=ORIENTED_EDGE('',*,*,#44815,.F.) ;
#62967=ORIENTED_EDGE('',*,*,#45729,.F.) ;
#62968=ORIENTED_EDGE('',*,*,#46771,.T.) ;
#62969=ORIENTED_EDGE('',*,*,#46773,.F.) ;
#62970=ORIENTED_EDGE('',*,*,#46772,.T.) ;
#62971=ORIENTED_EDGE('',*,*,#45790,.F.) ;
#62972=ORIENTED_EDGE('',*,*,#46774,.F.) ;
#62973=ORIENTED_EDGE('',*,*,#44816,.F.) ;
#62974=ORIENTED_EDGE('',*,*,#46773,.T.) ;
#62975=ORIENTED_EDGE('',*,*,#44797,.F.) ;
#62976=ORIENTED_EDGE('',*,*,#46775,.F.) ;
#62977=ORIENTED_EDGE('',*,*,#45726,.F.) ;
#62978=ORIENTED_EDGE('',*,*,#46774,.T.) ;
#62979=ORIENTED_EDGE('',*,*,#45793,.F.) ;
#62980=ORIENTED_EDGE('',*,*,#46776,.F.) ;
#62981=ORIENTED_EDGE('',*,*,#44817,.F.) ;
#62982=ORIENTED_EDGE('',*,*,#45723,.F.) ;
#62983=ORIENTED_EDGE('',*,*,#46775,.T.) ;
#62984=ORIENTED_EDGE('',*,*,#46777,.F.) ;
#62985=ORIENTED_EDGE('',*,*,#46776,.T.) ;
#62986=ORIENTED_EDGE('',*,*,#45796,.F.) ;
#62987=ORIENTED_EDGE('',*,*,#46778,.F.) ;
#62988=ORIENTED_EDGE('',*,*,#44795,.F.) ;
#62989=ORIENTED_EDGE('',*,*,#46777,.T.) ;
#62990=ORIENTED_EDGE('',*,*,#44796,.F.) ;
#62991=ORIENTED_EDGE('',*,*,#46778,.T.) ;
#62992=ORIENTED_EDGE('',*,*,#45798,.F.) ;
#62993=ORIENTED_EDGE('',*,*,#46779,.F.) ;
#62994=ORIENTED_EDGE('',*,*,#45854,.F.) ;
#62995=ORIENTED_EDGE('',*,*,#46780,.F.) ;
#62996=ORIENTED_EDGE('',*,*,#44829,.F.) ;
#62997=ORIENTED_EDGE('',*,*,#45851,.F.) ;
#62998=ORIENTED_EDGE('',*,*,#46779,.T.) ;
#62999=ORIENTED_EDGE('',*,*,#46781,.F.) ;
#63000=ORIENTED_EDGE('',*,*,#46780,.T.) ;
#63001=ORIENTED_EDGE('',*,*,#45857,.F.) ;
#63002=ORIENTED_EDGE('',*,*,#46782,.F.) ;
#63003=ORIENTED_EDGE('',*,*,#46781,.T.) ;
#63004=ORIENTED_EDGE('',*,*,#44828,.F.) ;
#63005=ORIENTED_EDGE('',*,*,#46783,.F.) ;
#63006=ORIENTED_EDGE('',*,*,#45848,.F.) ;
#63007=ORIENTED_EDGE('',*,*,#46782,.T.) ;
#63008=ORIENTED_EDGE('',*,*,#45860,.F.) ;
#63009=ORIENTED_EDGE('',*,*,#46784,.F.) ;
#63010=ORIENTED_EDGE('',*,*,#44830,.F.) ;
#63011=ORIENTED_EDGE('',*,*,#46783,.T.) ;
#63012=ORIENTED_EDGE('',*,*,#44827,.F.) ;
#63013=ORIENTED_EDGE('',*,*,#46785,.F.) ;
#63014=ORIENTED_EDGE('',*,*,#45845,.F.) ;
#63015=ORIENTED_EDGE('',*,*,#46784,.T.) ;
#63016=ORIENTED_EDGE('',*,*,#45863,.F.) ;
#63017=ORIENTED_EDGE('',*,*,#46786,.F.) ;
#63018=ORIENTED_EDGE('',*,*,#44831,.F.) ;
#63019=ORIENTED_EDGE('',*,*,#46785,.T.) ;
#63020=ORIENTED_EDGE('',*,*,#44826,.F.) ;
#63021=ORIENTED_EDGE('',*,*,#44318,.F.) ;
#63022=ORIENTED_EDGE('',*,*,#45842,.F.) ;
#63023=ORIENTED_EDGE('',*,*,#46786,.T.) ;
#63024=ORIENTED_EDGE('',*,*,#45866,.F.) ;
#63025=ORIENTED_EDGE('',*,*,#46787,.F.) ;
#63026=ORIENTED_EDGE('',*,*,#44832,.F.) ;
#63027=ORIENTED_EDGE('',*,*,#46787,.T.) ;
#63028=ORIENTED_EDGE('',*,*,#45869,.F.) ;
#63029=ORIENTED_EDGE('',*,*,#46788,.F.) ;
#63030=ORIENTED_EDGE('',*,*,#44833,.F.) ;
#63031=ORIENTED_EDGE('',*,*,#44316,.T.) ;
#63032=ORIENTED_EDGE('',*,*,#44825,.F.) ;
#63033=ORIENTED_EDGE('',*,*,#46789,.F.) ;
#63034=ORIENTED_EDGE('',*,*,#45839,.F.) ;
#63035=ORIENTED_EDGE('',*,*,#46788,.T.) ;
#63036=ORIENTED_EDGE('',*,*,#45872,.F.) ;
#63037=ORIENTED_EDGE('',*,*,#46790,.F.) ;
#63038=ORIENTED_EDGE('',*,*,#44834,.F.) ;
#63039=ORIENTED_EDGE('',*,*,#46789,.T.) ;
#63040=ORIENTED_EDGE('',*,*,#44824,.F.) ;
#63041=ORIENTED_EDGE('',*,*,#46791,.F.) ;
#63042=ORIENTED_EDGE('',*,*,#45837,.F.) ;
#63043=ORIENTED_EDGE('',*,*,#46790,.T.) ;
#63044=ORIENTED_EDGE('',*,*,#45875,.F.) ;
#63045=ORIENTED_EDGE('',*,*,#46792,.F.) ;
#63046=ORIENTED_EDGE('',*,*,#44835,.F.) ;
#63047=ORIENTED_EDGE('',*,*,#46791,.T.) ;
#63048=ORIENTED_EDGE('',*,*,#44823,.F.) ;
#63049=ORIENTED_EDGE('',*,*,#46793,.F.) ;
#63050=ORIENTED_EDGE('',*,*,#45835,.F.) ;
#63051=ORIENTED_EDGE('',*,*,#46792,.T.) ;
#63052=ORIENTED_EDGE('',*,*,#45878,.F.) ;
#63053=ORIENTED_EDGE('',*,*,#46794,.F.) ;
#63054=ORIENTED_EDGE('',*,*,#44836,.F.) ;
#63055=ORIENTED_EDGE('',*,*,#46793,.T.) ;
#63056=ORIENTED_EDGE('',*,*,#44822,.F.) ;
#63057=ORIENTED_EDGE('',*,*,#46795,.F.) ;
#63058=ORIENTED_EDGE('',*,*,#45832,.F.) ;
#63059=ORIENTED_EDGE('',*,*,#46794,.T.) ;
#63060=ORIENTED_EDGE('',*,*,#45881,.F.) ;
#63061=ORIENTED_EDGE('',*,*,#46796,.F.) ;
#63062=ORIENTED_EDGE('',*,*,#44837,.F.) ;
#63063=ORIENTED_EDGE('',*,*,#46795,.T.) ;
#63064=ORIENTED_EDGE('',*,*,#44821,.F.) ;
#63065=ORIENTED_EDGE('',*,*,#46797,.F.) ;
#63066=ORIENTED_EDGE('',*,*,#45829,.F.) ;
#63067=ORIENTED_EDGE('',*,*,#46796,.T.) ;
#63068=ORIENTED_EDGE('',*,*,#45884,.F.) ;
#63069=ORIENTED_EDGE('',*,*,#46798,.F.) ;
#63070=ORIENTED_EDGE('',*,*,#44838,.F.) ;
#63071=ORIENTED_EDGE('',*,*,#45826,.F.) ;
#63072=ORIENTED_EDGE('',*,*,#46797,.T.) ;
#63073=ORIENTED_EDGE('',*,*,#46799,.F.) ;
#63074=ORIENTED_EDGE('',*,*,#46798,.T.) ;
#63075=ORIENTED_EDGE('',*,*,#45887,.F.) ;
#63076=ORIENTED_EDGE('',*,*,#46800,.F.) ;
#63077=ORIENTED_EDGE('',*,*,#44839,.F.) ;
#63078=ORIENTED_EDGE('',*,*,#46799,.T.) ;
#63079=ORIENTED_EDGE('',*,*,#44820,.F.) ;
#63080=ORIENTED_EDGE('',*,*,#46801,.F.) ;
#63081=ORIENTED_EDGE('',*,*,#45823,.F.) ;
#63082=ORIENTED_EDGE('',*,*,#46800,.T.) ;
#63083=ORIENTED_EDGE('',*,*,#45890,.F.) ;
#63084=ORIENTED_EDGE('',*,*,#46802,.F.) ;
#63085=ORIENTED_EDGE('',*,*,#44840,.F.) ;
#63086=ORIENTED_EDGE('',*,*,#45820,.F.) ;
#63087=ORIENTED_EDGE('',*,*,#46801,.T.) ;
#63088=ORIENTED_EDGE('',*,*,#46803,.F.) ;
#63089=ORIENTED_EDGE('',*,*,#46802,.T.) ;
#63090=ORIENTED_EDGE('',*,*,#45893,.F.) ;
#63091=ORIENTED_EDGE('',*,*,#46804,.F.) ;
#63092=ORIENTED_EDGE('',*,*,#44818,.F.) ;
#63093=ORIENTED_EDGE('',*,*,#46803,.T.) ;
#63094=ORIENTED_EDGE('',*,*,#44819,.F.) ;
#63095=ORIENTED_EDGE('',*,*,#46804,.T.) ;
#63096=ORIENTED_EDGE('',*,*,#45895,.F.) ;
#63097=ORIENTED_EDGE('',*,*,#46805,.F.) ;
#63098=ORIENTED_EDGE('',*,*,#45951,.F.) ;
#63099=ORIENTED_EDGE('',*,*,#46806,.F.) ;
#63100=ORIENTED_EDGE('',*,*,#44852,.F.) ;
#63101=ORIENTED_EDGE('',*,*,#45948,.F.) ;
#63102=ORIENTED_EDGE('',*,*,#46805,.T.) ;
#63103=ORIENTED_EDGE('',*,*,#46807,.F.) ;
#63104=ORIENTED_EDGE('',*,*,#46806,.T.) ;
#63105=ORIENTED_EDGE('',*,*,#45954,.F.) ;
#63106=ORIENTED_EDGE('',*,*,#46808,.F.) ;
#63107=ORIENTED_EDGE('',*,*,#46807,.T.) ;
#63108=ORIENTED_EDGE('',*,*,#44851,.F.) ;
#63109=ORIENTED_EDGE('',*,*,#46809,.F.) ;
#63110=ORIENTED_EDGE('',*,*,#45945,.F.) ;
#63111=ORIENTED_EDGE('',*,*,#46808,.T.) ;
#63112=ORIENTED_EDGE('',*,*,#45957,.F.) ;
#63113=ORIENTED_EDGE('',*,*,#46810,.F.) ;
#63114=ORIENTED_EDGE('',*,*,#44853,.F.) ;
#63115=ORIENTED_EDGE('',*,*,#46809,.T.) ;
#63116=ORIENTED_EDGE('',*,*,#44850,.F.) ;
#63117=ORIENTED_EDGE('',*,*,#46811,.F.) ;
#63118=ORIENTED_EDGE('',*,*,#45942,.F.) ;
#63119=ORIENTED_EDGE('',*,*,#46810,.T.) ;
#63120=ORIENTED_EDGE('',*,*,#45960,.F.) ;
#63121=ORIENTED_EDGE('',*,*,#46812,.F.) ;
#63122=ORIENTED_EDGE('',*,*,#44854,.F.) ;
#63123=ORIENTED_EDGE('',*,*,#46811,.T.) ;
#63124=ORIENTED_EDGE('',*,*,#44849,.F.) ;
#63125=ORIENTED_EDGE('',*,*,#44314,.F.) ;
#63126=ORIENTED_EDGE('',*,*,#45939,.F.) ;
#63127=ORIENTED_EDGE('',*,*,#46812,.T.) ;
#63128=ORIENTED_EDGE('',*,*,#45963,.F.) ;
#63129=ORIENTED_EDGE('',*,*,#46813,.F.) ;
#63130=ORIENTED_EDGE('',*,*,#44855,.F.) ;
#63131=ORIENTED_EDGE('',*,*,#46813,.T.) ;
#63132=ORIENTED_EDGE('',*,*,#45966,.F.) ;
#63133=ORIENTED_EDGE('',*,*,#46814,.F.) ;
#63134=ORIENTED_EDGE('',*,*,#44856,.F.) ;
#63135=ORIENTED_EDGE('',*,*,#44312,.T.) ;
#63136=ORIENTED_EDGE('',*,*,#44848,.F.) ;
#63137=ORIENTED_EDGE('',*,*,#46815,.F.) ;
#63138=ORIENTED_EDGE('',*,*,#45936,.F.) ;
#63139=ORIENTED_EDGE('',*,*,#46814,.T.) ;
#63140=ORIENTED_EDGE('',*,*,#45969,.F.) ;
#63141=ORIENTED_EDGE('',*,*,#46816,.F.) ;
#63142=ORIENTED_EDGE('',*,*,#44857,.F.) ;
#63143=ORIENTED_EDGE('',*,*,#46815,.T.) ;
#63144=ORIENTED_EDGE('',*,*,#44847,.F.) ;
#63145=ORIENTED_EDGE('',*,*,#46817,.F.) ;
#63146=ORIENTED_EDGE('',*,*,#45934,.F.) ;
#63147=ORIENTED_EDGE('',*,*,#46816,.T.) ;
#63148=ORIENTED_EDGE('',*,*,#45972,.F.) ;
#63149=ORIENTED_EDGE('',*,*,#46818,.F.) ;
#63150=ORIENTED_EDGE('',*,*,#44858,.F.) ;
#63151=ORIENTED_EDGE('',*,*,#46817,.T.) ;
#63152=ORIENTED_EDGE('',*,*,#44846,.F.) ;
#63153=ORIENTED_EDGE('',*,*,#46819,.F.) ;
#63154=ORIENTED_EDGE('',*,*,#45932,.F.) ;
#63155=ORIENTED_EDGE('',*,*,#46818,.T.) ;
#63156=ORIENTED_EDGE('',*,*,#45975,.F.) ;
#63157=ORIENTED_EDGE('',*,*,#46820,.F.) ;
#63158=ORIENTED_EDGE('',*,*,#44859,.F.) ;
#63159=ORIENTED_EDGE('',*,*,#46819,.T.) ;
#63160=ORIENTED_EDGE('',*,*,#44845,.F.) ;
#63161=ORIENTED_EDGE('',*,*,#46821,.F.) ;
#63162=ORIENTED_EDGE('',*,*,#45929,.F.) ;
#63163=ORIENTED_EDGE('',*,*,#46820,.T.) ;
#63164=ORIENTED_EDGE('',*,*,#45978,.F.) ;
#63165=ORIENTED_EDGE('',*,*,#46822,.F.) ;
#63166=ORIENTED_EDGE('',*,*,#44860,.F.) ;
#63167=ORIENTED_EDGE('',*,*,#46821,.T.) ;
#63168=ORIENTED_EDGE('',*,*,#44844,.F.) ;
#63169=ORIENTED_EDGE('',*,*,#46823,.F.) ;
#63170=ORIENTED_EDGE('',*,*,#45926,.F.) ;
#63171=ORIENTED_EDGE('',*,*,#46822,.T.) ;
#63172=ORIENTED_EDGE('',*,*,#45981,.F.) ;
#63173=ORIENTED_EDGE('',*,*,#46824,.F.) ;
#63174=ORIENTED_EDGE('',*,*,#44861,.F.) ;
#63175=ORIENTED_EDGE('',*,*,#45923,.F.) ;
#63176=ORIENTED_EDGE('',*,*,#46823,.T.) ;
#63177=ORIENTED_EDGE('',*,*,#46825,.F.) ;
#63178=ORIENTED_EDGE('',*,*,#46824,.T.) ;
#63179=ORIENTED_EDGE('',*,*,#45984,.F.) ;
#63180=ORIENTED_EDGE('',*,*,#46826,.F.) ;
#63181=ORIENTED_EDGE('',*,*,#44862,.F.) ;
#63182=ORIENTED_EDGE('',*,*,#46825,.T.) ;
#63183=ORIENTED_EDGE('',*,*,#44843,.F.) ;
#63184=ORIENTED_EDGE('',*,*,#46827,.F.) ;
#63185=ORIENTED_EDGE('',*,*,#45920,.F.) ;
#63186=ORIENTED_EDGE('',*,*,#46826,.T.) ;
#63187=ORIENTED_EDGE('',*,*,#45987,.F.) ;
#63188=ORIENTED_EDGE('',*,*,#46828,.F.) ;
#63189=ORIENTED_EDGE('',*,*,#44863,.F.) ;
#63190=ORIENTED_EDGE('',*,*,#45917,.F.) ;
#63191=ORIENTED_EDGE('',*,*,#46827,.T.) ;
#63192=ORIENTED_EDGE('',*,*,#46829,.F.) ;
#63193=ORIENTED_EDGE('',*,*,#46828,.T.) ;
#63194=ORIENTED_EDGE('',*,*,#45990,.F.) ;
#63195=ORIENTED_EDGE('',*,*,#46830,.F.) ;
#63196=ORIENTED_EDGE('',*,*,#44841,.F.) ;
#63197=ORIENTED_EDGE('',*,*,#46829,.T.) ;
#63198=ORIENTED_EDGE('',*,*,#44842,.F.) ;
#63199=ORIENTED_EDGE('',*,*,#46830,.T.) ;
#63200=ORIENTED_EDGE('',*,*,#45992,.F.) ;
#63201=ORIENTED_EDGE('',*,*,#46831,.F.) ;
#63202=ORIENTED_EDGE('',*,*,#46048,.F.) ;
#63203=ORIENTED_EDGE('',*,*,#46832,.F.) ;
#63204=ORIENTED_EDGE('',*,*,#44875,.F.) ;
#63205=ORIENTED_EDGE('',*,*,#46045,.F.) ;
#63206=ORIENTED_EDGE('',*,*,#46831,.T.) ;
#63207=ORIENTED_EDGE('',*,*,#46833,.F.) ;
#63208=ORIENTED_EDGE('',*,*,#46832,.T.) ;
#63209=ORIENTED_EDGE('',*,*,#46051,.F.) ;
#63210=ORIENTED_EDGE('',*,*,#46834,.F.) ;
#63211=ORIENTED_EDGE('',*,*,#46833,.T.) ;
#63212=ORIENTED_EDGE('',*,*,#44874,.F.) ;
#63213=ORIENTED_EDGE('',*,*,#46835,.F.) ;
#63214=ORIENTED_EDGE('',*,*,#46042,.F.) ;
#63215=ORIENTED_EDGE('',*,*,#46834,.T.) ;
#63216=ORIENTED_EDGE('',*,*,#46054,.F.) ;
#63217=ORIENTED_EDGE('',*,*,#46836,.F.) ;
#63218=ORIENTED_EDGE('',*,*,#44876,.F.) ;
#63219=ORIENTED_EDGE('',*,*,#46835,.T.) ;
#63220=ORIENTED_EDGE('',*,*,#44873,.F.) ;
#63221=ORIENTED_EDGE('',*,*,#46837,.F.) ;
#63222=ORIENTED_EDGE('',*,*,#46039,.F.) ;
#63223=ORIENTED_EDGE('',*,*,#46836,.T.) ;
#63224=ORIENTED_EDGE('',*,*,#46057,.F.) ;
#63225=ORIENTED_EDGE('',*,*,#46838,.F.) ;
#63226=ORIENTED_EDGE('',*,*,#44877,.F.) ;
#63227=ORIENTED_EDGE('',*,*,#46837,.T.) ;
#63228=ORIENTED_EDGE('',*,*,#44872,.F.) ;
#63229=ORIENTED_EDGE('',*,*,#44310,.F.) ;
#63230=ORIENTED_EDGE('',*,*,#46036,.F.) ;
#63231=ORIENTED_EDGE('',*,*,#46838,.T.) ;
#63232=ORIENTED_EDGE('',*,*,#46060,.F.) ;
#63233=ORIENTED_EDGE('',*,*,#46839,.F.) ;
#63234=ORIENTED_EDGE('',*,*,#44878,.F.) ;
#63235=ORIENTED_EDGE('',*,*,#46839,.T.) ;
#63236=ORIENTED_EDGE('',*,*,#46063,.F.) ;
#63237=ORIENTED_EDGE('',*,*,#46840,.F.) ;
#63238=ORIENTED_EDGE('',*,*,#44879,.F.) ;
#63239=ORIENTED_EDGE('',*,*,#44308,.T.) ;
#63240=ORIENTED_EDGE('',*,*,#44871,.F.) ;
#63241=ORIENTED_EDGE('',*,*,#46841,.F.) ;
#63242=ORIENTED_EDGE('',*,*,#46033,.F.) ;
#63243=ORIENTED_EDGE('',*,*,#46840,.T.) ;
#63244=ORIENTED_EDGE('',*,*,#46066,.F.) ;
#63245=ORIENTED_EDGE('',*,*,#46842,.F.) ;
#63246=ORIENTED_EDGE('',*,*,#44880,.F.) ;
#63247=ORIENTED_EDGE('',*,*,#46841,.T.) ;
#63248=ORIENTED_EDGE('',*,*,#44870,.F.) ;
#63249=ORIENTED_EDGE('',*,*,#46843,.F.) ;
#63250=ORIENTED_EDGE('',*,*,#46031,.F.) ;
#63251=ORIENTED_EDGE('',*,*,#46842,.T.) ;
#63252=ORIENTED_EDGE('',*,*,#46069,.F.) ;
#63253=ORIENTED_EDGE('',*,*,#46844,.F.) ;
#63254=ORIENTED_EDGE('',*,*,#44881,.F.) ;
#63255=ORIENTED_EDGE('',*,*,#46843,.T.) ;
#63256=ORIENTED_EDGE('',*,*,#44869,.F.) ;
#63257=ORIENTED_EDGE('',*,*,#46845,.F.) ;
#63258=ORIENTED_EDGE('',*,*,#46029,.F.) ;
#63259=ORIENTED_EDGE('',*,*,#46844,.T.) ;
#63260=ORIENTED_EDGE('',*,*,#46072,.F.) ;
#63261=ORIENTED_EDGE('',*,*,#46846,.F.) ;
#63262=ORIENTED_EDGE('',*,*,#44882,.F.) ;
#63263=ORIENTED_EDGE('',*,*,#46845,.T.) ;
#63264=ORIENTED_EDGE('',*,*,#44868,.F.) ;
#63265=ORIENTED_EDGE('',*,*,#46847,.F.) ;
#63266=ORIENTED_EDGE('',*,*,#46026,.F.) ;
#63267=ORIENTED_EDGE('',*,*,#46846,.T.) ;
#63268=ORIENTED_EDGE('',*,*,#46075,.F.) ;
#63269=ORIENTED_EDGE('',*,*,#46848,.F.) ;
#63270=ORIENTED_EDGE('',*,*,#44883,.F.) ;
#63271=ORIENTED_EDGE('',*,*,#46847,.T.) ;
#63272=ORIENTED_EDGE('',*,*,#44867,.F.) ;
#63273=ORIENTED_EDGE('',*,*,#46849,.F.) ;
#63274=ORIENTED_EDGE('',*,*,#46023,.F.) ;
#63275=ORIENTED_EDGE('',*,*,#46848,.T.) ;
#63276=ORIENTED_EDGE('',*,*,#46078,.F.) ;
#63277=ORIENTED_EDGE('',*,*,#46850,.F.) ;
#63278=ORIENTED_EDGE('',*,*,#44884,.F.) ;
#63279=ORIENTED_EDGE('',*,*,#46020,.F.) ;
#63280=ORIENTED_EDGE('',*,*,#46849,.T.) ;
#63281=ORIENTED_EDGE('',*,*,#46851,.F.) ;
#63282=ORIENTED_EDGE('',*,*,#46850,.T.) ;
#63283=ORIENTED_EDGE('',*,*,#46081,.F.) ;
#63284=ORIENTED_EDGE('',*,*,#46852,.F.) ;
#63285=ORIENTED_EDGE('',*,*,#44885,.F.) ;
#63286=ORIENTED_EDGE('',*,*,#46851,.T.) ;
#63287=ORIENTED_EDGE('',*,*,#44866,.F.) ;
#63288=ORIENTED_EDGE('',*,*,#46853,.F.) ;
#63289=ORIENTED_EDGE('',*,*,#46017,.F.) ;
#63290=ORIENTED_EDGE('',*,*,#46852,.T.) ;
#63291=ORIENTED_EDGE('',*,*,#46084,.F.) ;
#63292=ORIENTED_EDGE('',*,*,#46854,.F.) ;
#63293=ORIENTED_EDGE('',*,*,#44886,.F.) ;
#63294=ORIENTED_EDGE('',*,*,#46014,.F.) ;
#63295=ORIENTED_EDGE('',*,*,#46853,.T.) ;
#63296=ORIENTED_EDGE('',*,*,#46855,.F.) ;
#63297=ORIENTED_EDGE('',*,*,#46854,.T.) ;
#63298=ORIENTED_EDGE('',*,*,#46087,.F.) ;
#63299=ORIENTED_EDGE('',*,*,#46856,.F.) ;
#63300=ORIENTED_EDGE('',*,*,#44864,.F.) ;
#63301=ORIENTED_EDGE('',*,*,#46855,.T.) ;
#63302=ORIENTED_EDGE('',*,*,#44865,.F.) ;
#63303=ORIENTED_EDGE('',*,*,#46856,.T.) ;
#63304=ORIENTED_EDGE('',*,*,#46089,.F.) ;
#63305=ORIENTED_EDGE('',*,*,#46857,.F.) ;
#63306=ORIENTED_EDGE('',*,*,#46145,.F.) ;
#63307=ORIENTED_EDGE('',*,*,#46858,.F.) ;
#63308=ORIENTED_EDGE('',*,*,#44898,.F.) ;
#63309=ORIENTED_EDGE('',*,*,#46142,.F.) ;
#63310=ORIENTED_EDGE('',*,*,#46857,.T.) ;
#63311=ORIENTED_EDGE('',*,*,#46859,.F.) ;
#63312=ORIENTED_EDGE('',*,*,#46858,.T.) ;
#63313=ORIENTED_EDGE('',*,*,#46148,.F.) ;
#63314=ORIENTED_EDGE('',*,*,#46860,.F.) ;
#63315=ORIENTED_EDGE('',*,*,#46859,.T.) ;
#63316=ORIENTED_EDGE('',*,*,#44897,.F.) ;
#63317=ORIENTED_EDGE('',*,*,#46861,.F.) ;
#63318=ORIENTED_EDGE('',*,*,#46139,.F.) ;
#63319=ORIENTED_EDGE('',*,*,#46860,.T.) ;
#63320=ORIENTED_EDGE('',*,*,#46151,.F.) ;
#63321=ORIENTED_EDGE('',*,*,#46862,.F.) ;
#63322=ORIENTED_EDGE('',*,*,#44899,.F.) ;
#63323=ORIENTED_EDGE('',*,*,#46861,.T.) ;
#63324=ORIENTED_EDGE('',*,*,#44896,.F.) ;
#63325=ORIENTED_EDGE('',*,*,#46863,.F.) ;
#63326=ORIENTED_EDGE('',*,*,#46136,.F.) ;
#63327=ORIENTED_EDGE('',*,*,#46862,.T.) ;
#63328=ORIENTED_EDGE('',*,*,#46154,.F.) ;
#63329=ORIENTED_EDGE('',*,*,#46864,.F.) ;
#63330=ORIENTED_EDGE('',*,*,#44900,.F.) ;
#63331=ORIENTED_EDGE('',*,*,#46863,.T.) ;
#63332=ORIENTED_EDGE('',*,*,#44895,.F.) ;
#63333=ORIENTED_EDGE('',*,*,#44306,.F.) ;
#63334=ORIENTED_EDGE('',*,*,#46133,.F.) ;
#63335=ORIENTED_EDGE('',*,*,#46864,.T.) ;
#63336=ORIENTED_EDGE('',*,*,#46157,.F.) ;
#63337=ORIENTED_EDGE('',*,*,#46865,.F.) ;
#63338=ORIENTED_EDGE('',*,*,#44901,.F.) ;
#63339=ORIENTED_EDGE('',*,*,#46865,.T.) ;
#63340=ORIENTED_EDGE('',*,*,#46160,.F.) ;
#63341=ORIENTED_EDGE('',*,*,#46866,.F.) ;
#63342=ORIENTED_EDGE('',*,*,#44902,.F.) ;
#63343=ORIENTED_EDGE('',*,*,#44304,.T.) ;
#63344=ORIENTED_EDGE('',*,*,#44894,.F.) ;
#63345=ORIENTED_EDGE('',*,*,#46867,.F.) ;
#63346=ORIENTED_EDGE('',*,*,#46130,.F.) ;
#63347=ORIENTED_EDGE('',*,*,#46866,.T.) ;
#63348=ORIENTED_EDGE('',*,*,#46163,.F.) ;
#63349=ORIENTED_EDGE('',*,*,#46868,.F.) ;
#63350=ORIENTED_EDGE('',*,*,#44903,.F.) ;
#63351=ORIENTED_EDGE('',*,*,#46867,.T.) ;
#63352=ORIENTED_EDGE('',*,*,#44893,.F.) ;
#63353=ORIENTED_EDGE('',*,*,#46869,.F.) ;
#63354=ORIENTED_EDGE('',*,*,#46128,.F.) ;
#63355=ORIENTED_EDGE('',*,*,#46868,.T.) ;
#63356=ORIENTED_EDGE('',*,*,#46166,.F.) ;
#63357=ORIENTED_EDGE('',*,*,#46870,.F.) ;
#63358=ORIENTED_EDGE('',*,*,#44904,.F.) ;
#63359=ORIENTED_EDGE('',*,*,#46869,.T.) ;
#63360=ORIENTED_EDGE('',*,*,#44892,.F.) ;
#63361=ORIENTED_EDGE('',*,*,#46871,.F.) ;
#63362=ORIENTED_EDGE('',*,*,#46126,.F.) ;
#63363=ORIENTED_EDGE('',*,*,#46870,.T.) ;
#63364=ORIENTED_EDGE('',*,*,#46169,.F.) ;
#63365=ORIENTED_EDGE('',*,*,#46872,.F.) ;
#63366=ORIENTED_EDGE('',*,*,#44905,.F.) ;
#63367=ORIENTED_EDGE('',*,*,#46871,.T.) ;
#63368=ORIENTED_EDGE('',*,*,#44891,.F.) ;
#63369=ORIENTED_EDGE('',*,*,#46873,.F.) ;
#63370=ORIENTED_EDGE('',*,*,#46123,.F.) ;
#63371=ORIENTED_EDGE('',*,*,#46872,.T.) ;
#63372=ORIENTED_EDGE('',*,*,#46172,.F.) ;
#63373=ORIENTED_EDGE('',*,*,#46874,.F.) ;
#63374=ORIENTED_EDGE('',*,*,#44906,.F.) ;
#63375=ORIENTED_EDGE('',*,*,#46873,.T.) ;
#63376=ORIENTED_EDGE('',*,*,#44890,.F.) ;
#63377=ORIENTED_EDGE('',*,*,#46875,.F.) ;
#63378=ORIENTED_EDGE('',*,*,#46120,.F.) ;
#63379=ORIENTED_EDGE('',*,*,#46874,.T.) ;
#63380=ORIENTED_EDGE('',*,*,#46175,.F.) ;
#63381=ORIENTED_EDGE('',*,*,#46876,.F.) ;
#63382=ORIENTED_EDGE('',*,*,#44907,.F.) ;
#63383=ORIENTED_EDGE('',*,*,#46117,.F.) ;
#63384=ORIENTED_EDGE('',*,*,#46875,.T.) ;
#63385=ORIENTED_EDGE('',*,*,#46877,.F.) ;
#63386=ORIENTED_EDGE('',*,*,#46876,.T.) ;
#63387=ORIENTED_EDGE('',*,*,#46178,.F.) ;
#63388=ORIENTED_EDGE('',*,*,#46878,.F.) ;
#63389=ORIENTED_EDGE('',*,*,#44908,.F.) ;
#63390=ORIENTED_EDGE('',*,*,#46877,.T.) ;
#63391=ORIENTED_EDGE('',*,*,#44889,.F.) ;
#63392=ORIENTED_EDGE('',*,*,#46879,.F.) ;
#63393=ORIENTED_EDGE('',*,*,#46114,.F.) ;
#63394=ORIENTED_EDGE('',*,*,#46878,.T.) ;
#63395=ORIENTED_EDGE('',*,*,#46181,.F.) ;
#63396=ORIENTED_EDGE('',*,*,#46880,.F.) ;
#63397=ORIENTED_EDGE('',*,*,#44909,.F.) ;
#63398=ORIENTED_EDGE('',*,*,#46111,.F.) ;
#63399=ORIENTED_EDGE('',*,*,#46879,.T.) ;
#63400=ORIENTED_EDGE('',*,*,#46881,.F.) ;
#63401=ORIENTED_EDGE('',*,*,#46880,.T.) ;
#63402=ORIENTED_EDGE('',*,*,#46184,.F.) ;
#63403=ORIENTED_EDGE('',*,*,#46882,.F.) ;
#63404=ORIENTED_EDGE('',*,*,#44887,.F.) ;
#63405=ORIENTED_EDGE('',*,*,#46881,.T.) ;
#63406=ORIENTED_EDGE('',*,*,#44888,.F.) ;
#63407=ORIENTED_EDGE('',*,*,#46882,.T.) ;
#63408=ORIENTED_EDGE('',*,*,#46186,.F.) ;
#63409=ORIENTED_EDGE('',*,*,#46883,.F.) ;
#63410=ORIENTED_EDGE('',*,*,#46242,.F.) ;
#63411=ORIENTED_EDGE('',*,*,#46884,.F.) ;
#63412=ORIENTED_EDGE('',*,*,#44921,.F.) ;
#63413=ORIENTED_EDGE('',*,*,#46239,.F.) ;
#63414=ORIENTED_EDGE('',*,*,#46883,.T.) ;
#63415=ORIENTED_EDGE('',*,*,#46885,.F.) ;
#63416=ORIENTED_EDGE('',*,*,#46884,.T.) ;
#63417=ORIENTED_EDGE('',*,*,#46245,.F.) ;
#63418=ORIENTED_EDGE('',*,*,#46886,.F.) ;
#63419=ORIENTED_EDGE('',*,*,#46885,.T.) ;
#63420=ORIENTED_EDGE('',*,*,#44920,.F.) ;
#63421=ORIENTED_EDGE('',*,*,#46887,.F.) ;
#63422=ORIENTED_EDGE('',*,*,#46236,.F.) ;
#63423=ORIENTED_EDGE('',*,*,#46886,.T.) ;
#63424=ORIENTED_EDGE('',*,*,#46248,.F.) ;
#63425=ORIENTED_EDGE('',*,*,#46888,.F.) ;
#63426=ORIENTED_EDGE('',*,*,#44922,.F.) ;
#63427=ORIENTED_EDGE('',*,*,#46887,.T.) ;
#63428=ORIENTED_EDGE('',*,*,#44919,.F.) ;
#63429=ORIENTED_EDGE('',*,*,#46889,.F.) ;
#63430=ORIENTED_EDGE('',*,*,#46233,.F.) ;
#63431=ORIENTED_EDGE('',*,*,#46888,.T.) ;
#63432=ORIENTED_EDGE('',*,*,#46251,.F.) ;
#63433=ORIENTED_EDGE('',*,*,#46890,.F.) ;
#63434=ORIENTED_EDGE('',*,*,#44923,.F.) ;
#63435=ORIENTED_EDGE('',*,*,#46889,.T.) ;
#63436=ORIENTED_EDGE('',*,*,#44918,.F.) ;
#63437=ORIENTED_EDGE('',*,*,#44302,.F.) ;
#63438=ORIENTED_EDGE('',*,*,#46230,.F.) ;
#63439=ORIENTED_EDGE('',*,*,#46890,.T.) ;
#63440=ORIENTED_EDGE('',*,*,#46254,.F.) ;
#63441=ORIENTED_EDGE('',*,*,#46891,.F.) ;
#63442=ORIENTED_EDGE('',*,*,#44924,.F.) ;
#63443=ORIENTED_EDGE('',*,*,#46891,.T.) ;
#63444=ORIENTED_EDGE('',*,*,#46257,.F.) ;
#63445=ORIENTED_EDGE('',*,*,#46892,.F.) ;
#63446=ORIENTED_EDGE('',*,*,#44925,.F.) ;
#63447=ORIENTED_EDGE('',*,*,#44300,.T.) ;
#63448=ORIENTED_EDGE('',*,*,#44917,.F.) ;
#63449=ORIENTED_EDGE('',*,*,#46893,.F.) ;
#63450=ORIENTED_EDGE('',*,*,#46227,.F.) ;
#63451=ORIENTED_EDGE('',*,*,#46892,.T.) ;
#63452=ORIENTED_EDGE('',*,*,#46260,.F.) ;
#63453=ORIENTED_EDGE('',*,*,#46894,.F.) ;
#63454=ORIENTED_EDGE('',*,*,#44926,.F.) ;
#63455=ORIENTED_EDGE('',*,*,#46893,.T.) ;
#63456=ORIENTED_EDGE('',*,*,#44916,.F.) ;
#63457=ORIENTED_EDGE('',*,*,#46895,.F.) ;
#63458=ORIENTED_EDGE('',*,*,#46225,.F.) ;
#63459=ORIENTED_EDGE('',*,*,#46894,.T.) ;
#63460=ORIENTED_EDGE('',*,*,#46263,.F.) ;
#63461=ORIENTED_EDGE('',*,*,#46896,.F.) ;
#63462=ORIENTED_EDGE('',*,*,#44927,.F.) ;
#63463=ORIENTED_EDGE('',*,*,#46895,.T.) ;
#63464=ORIENTED_EDGE('',*,*,#44915,.F.) ;
#63465=ORIENTED_EDGE('',*,*,#46897,.F.) ;
#63466=ORIENTED_EDGE('',*,*,#46223,.F.) ;
#63467=ORIENTED_EDGE('',*,*,#46896,.T.) ;
#63468=ORIENTED_EDGE('',*,*,#46266,.F.) ;
#63469=ORIENTED_EDGE('',*,*,#46898,.F.) ;
#63470=ORIENTED_EDGE('',*,*,#44928,.F.) ;
#63471=ORIENTED_EDGE('',*,*,#46897,.T.) ;
#63472=ORIENTED_EDGE('',*,*,#44914,.F.) ;
#63473=ORIENTED_EDGE('',*,*,#46899,.F.) ;
#63474=ORIENTED_EDGE('',*,*,#46220,.F.) ;
#63475=ORIENTED_EDGE('',*,*,#46898,.T.) ;
#63476=ORIENTED_EDGE('',*,*,#46269,.F.) ;
#63477=ORIENTED_EDGE('',*,*,#46900,.F.) ;
#63478=ORIENTED_EDGE('',*,*,#44929,.F.) ;
#63479=ORIENTED_EDGE('',*,*,#46899,.T.) ;
#63480=ORIENTED_EDGE('',*,*,#44913,.F.) ;
#63481=ORIENTED_EDGE('',*,*,#46901,.F.) ;
#63482=ORIENTED_EDGE('',*,*,#46217,.F.) ;
#63483=ORIENTED_EDGE('',*,*,#46900,.T.) ;
#63484=ORIENTED_EDGE('',*,*,#46272,.F.) ;
#63485=ORIENTED_EDGE('',*,*,#46902,.F.) ;
#63486=ORIENTED_EDGE('',*,*,#44930,.F.) ;
#63487=ORIENTED_EDGE('',*,*,#46214,.F.) ;
#63488=ORIENTED_EDGE('',*,*,#46901,.T.) ;
#63489=ORIENTED_EDGE('',*,*,#46903,.F.) ;
#63490=ORIENTED_EDGE('',*,*,#46902,.T.) ;
#63491=ORIENTED_EDGE('',*,*,#46275,.F.) ;
#63492=ORIENTED_EDGE('',*,*,#46904,.F.) ;
#63493=ORIENTED_EDGE('',*,*,#44931,.F.) ;
#63494=ORIENTED_EDGE('',*,*,#46903,.T.) ;
#63495=ORIENTED_EDGE('',*,*,#44912,.F.) ;
#63496=ORIENTED_EDGE('',*,*,#46905,.F.) ;
#63497=ORIENTED_EDGE('',*,*,#46211,.F.) ;
#63498=ORIENTED_EDGE('',*,*,#46904,.T.) ;
#63499=ORIENTED_EDGE('',*,*,#46278,.F.) ;
#63500=ORIENTED_EDGE('',*,*,#46906,.F.) ;
#63501=ORIENTED_EDGE('',*,*,#44932,.F.) ;
#63502=ORIENTED_EDGE('',*,*,#46208,.F.) ;
#63503=ORIENTED_EDGE('',*,*,#46905,.T.) ;
#63504=ORIENTED_EDGE('',*,*,#46907,.F.) ;
#63505=ORIENTED_EDGE('',*,*,#46906,.T.) ;
#63506=ORIENTED_EDGE('',*,*,#46281,.F.) ;
#63507=ORIENTED_EDGE('',*,*,#46908,.F.) ;
#63508=ORIENTED_EDGE('',*,*,#44910,.F.) ;
#63509=ORIENTED_EDGE('',*,*,#46907,.T.) ;
#63510=ORIENTED_EDGE('',*,*,#44911,.F.) ;
#63511=ORIENTED_EDGE('',*,*,#46908,.T.) ;
#63512=ORIENTED_EDGE('',*,*,#46283,.F.) ;
#63513=ORIENTED_EDGE('',*,*,#46909,.F.) ;
#63514=ORIENTED_EDGE('',*,*,#46339,.F.) ;
#63515=ORIENTED_EDGE('',*,*,#46910,.F.) ;
#63516=ORIENTED_EDGE('',*,*,#44944,.F.) ;
#63517=ORIENTED_EDGE('',*,*,#46336,.F.) ;
#63518=ORIENTED_EDGE('',*,*,#46909,.T.) ;
#63519=ORIENTED_EDGE('',*,*,#46911,.F.) ;
#63520=ORIENTED_EDGE('',*,*,#46910,.T.) ;
#63521=ORIENTED_EDGE('',*,*,#46342,.F.) ;
#63522=ORIENTED_EDGE('',*,*,#46912,.F.) ;
#63523=ORIENTED_EDGE('',*,*,#46911,.T.) ;
#63524=ORIENTED_EDGE('',*,*,#44943,.F.) ;
#63525=ORIENTED_EDGE('',*,*,#46913,.F.) ;
#63526=ORIENTED_EDGE('',*,*,#46333,.F.) ;
#63527=ORIENTED_EDGE('',*,*,#46912,.T.) ;
#63528=ORIENTED_EDGE('',*,*,#46345,.F.) ;
#63529=ORIENTED_EDGE('',*,*,#46914,.F.) ;
#63530=ORIENTED_EDGE('',*,*,#44945,.F.) ;
#63531=ORIENTED_EDGE('',*,*,#46913,.T.) ;
#63532=ORIENTED_EDGE('',*,*,#44942,.F.) ;
#63533=ORIENTED_EDGE('',*,*,#46915,.F.) ;
#63534=ORIENTED_EDGE('',*,*,#46330,.F.) ;
#63535=ORIENTED_EDGE('',*,*,#46914,.T.) ;
#63536=ORIENTED_EDGE('',*,*,#46348,.F.) ;
#63537=ORIENTED_EDGE('',*,*,#46916,.F.) ;
#63538=ORIENTED_EDGE('',*,*,#44946,.F.) ;
#63539=ORIENTED_EDGE('',*,*,#46915,.T.) ;
#63540=ORIENTED_EDGE('',*,*,#44941,.F.) ;
#63541=ORIENTED_EDGE('',*,*,#44298,.F.) ;
#63542=ORIENTED_EDGE('',*,*,#46327,.F.) ;
#63543=ORIENTED_EDGE('',*,*,#46916,.T.) ;
#63544=ORIENTED_EDGE('',*,*,#46351,.F.) ;
#63545=ORIENTED_EDGE('',*,*,#46917,.F.) ;
#63546=ORIENTED_EDGE('',*,*,#44947,.F.) ;
#63547=ORIENTED_EDGE('',*,*,#46917,.T.) ;
#63548=ORIENTED_EDGE('',*,*,#46354,.F.) ;
#63549=ORIENTED_EDGE('',*,*,#46918,.F.) ;
#63550=ORIENTED_EDGE('',*,*,#44948,.F.) ;
#63551=ORIENTED_EDGE('',*,*,#44296,.T.) ;
#63552=ORIENTED_EDGE('',*,*,#44940,.F.) ;
#63553=ORIENTED_EDGE('',*,*,#46919,.F.) ;
#63554=ORIENTED_EDGE('',*,*,#46324,.F.) ;
#63555=ORIENTED_EDGE('',*,*,#46918,.T.) ;
#63556=ORIENTED_EDGE('',*,*,#46357,.F.) ;
#63557=ORIENTED_EDGE('',*,*,#46920,.F.) ;
#63558=ORIENTED_EDGE('',*,*,#44949,.F.) ;
#63559=ORIENTED_EDGE('',*,*,#46919,.T.) ;
#63560=ORIENTED_EDGE('',*,*,#44939,.F.) ;
#63561=ORIENTED_EDGE('',*,*,#46921,.F.) ;
#63562=ORIENTED_EDGE('',*,*,#46322,.F.) ;
#63563=ORIENTED_EDGE('',*,*,#46920,.T.) ;
#63564=ORIENTED_EDGE('',*,*,#46360,.F.) ;
#63565=ORIENTED_EDGE('',*,*,#46922,.F.) ;
#63566=ORIENTED_EDGE('',*,*,#44950,.F.) ;
#63567=ORIENTED_EDGE('',*,*,#46921,.T.) ;
#63568=ORIENTED_EDGE('',*,*,#44938,.F.) ;
#63569=ORIENTED_EDGE('',*,*,#46923,.F.) ;
#63570=ORIENTED_EDGE('',*,*,#46320,.F.) ;
#63571=ORIENTED_EDGE('',*,*,#46922,.T.) ;
#63572=ORIENTED_EDGE('',*,*,#46363,.F.) ;
#63573=ORIENTED_EDGE('',*,*,#46924,.F.) ;
#63574=ORIENTED_EDGE('',*,*,#44951,.F.) ;
#63575=ORIENTED_EDGE('',*,*,#46923,.T.) ;
#63576=ORIENTED_EDGE('',*,*,#44937,.F.) ;
#63577=ORIENTED_EDGE('',*,*,#46925,.F.) ;
#63578=ORIENTED_EDGE('',*,*,#46317,.F.) ;
#63579=ORIENTED_EDGE('',*,*,#46924,.T.) ;
#63580=ORIENTED_EDGE('',*,*,#46366,.F.) ;
#63581=ORIENTED_EDGE('',*,*,#46926,.F.) ;
#63582=ORIENTED_EDGE('',*,*,#44952,.F.) ;
#63583=ORIENTED_EDGE('',*,*,#46925,.T.) ;
#63584=ORIENTED_EDGE('',*,*,#44936,.F.) ;
#63585=ORIENTED_EDGE('',*,*,#46927,.F.) ;
#63586=ORIENTED_EDGE('',*,*,#46314,.F.) ;
#63587=ORIENTED_EDGE('',*,*,#46926,.T.) ;
#63588=ORIENTED_EDGE('',*,*,#46369,.F.) ;
#63589=ORIENTED_EDGE('',*,*,#46928,.F.) ;
#63590=ORIENTED_EDGE('',*,*,#44953,.F.) ;
#63591=ORIENTED_EDGE('',*,*,#46311,.F.) ;
#63592=ORIENTED_EDGE('',*,*,#46927,.T.) ;
#63593=ORIENTED_EDGE('',*,*,#46929,.F.) ;
#63594=ORIENTED_EDGE('',*,*,#46928,.T.) ;
#63595=ORIENTED_EDGE('',*,*,#46372,.F.) ;
#63596=ORIENTED_EDGE('',*,*,#46930,.F.) ;
#63597=ORIENTED_EDGE('',*,*,#44954,.F.) ;
#63598=ORIENTED_EDGE('',*,*,#46929,.T.) ;
#63599=ORIENTED_EDGE('',*,*,#44935,.F.) ;
#63600=ORIENTED_EDGE('',*,*,#46931,.F.) ;
#63601=ORIENTED_EDGE('',*,*,#46308,.F.) ;
#63602=ORIENTED_EDGE('',*,*,#46930,.T.) ;
#63603=ORIENTED_EDGE('',*,*,#46375,.F.) ;
#63604=ORIENTED_EDGE('',*,*,#46932,.F.) ;
#63605=ORIENTED_EDGE('',*,*,#44955,.F.) ;
#63606=ORIENTED_EDGE('',*,*,#46305,.F.) ;
#63607=ORIENTED_EDGE('',*,*,#46931,.T.) ;
#63608=ORIENTED_EDGE('',*,*,#46933,.F.) ;
#63609=ORIENTED_EDGE('',*,*,#46932,.T.) ;
#63610=ORIENTED_EDGE('',*,*,#46378,.F.) ;
#63611=ORIENTED_EDGE('',*,*,#46934,.F.) ;
#63612=ORIENTED_EDGE('',*,*,#44933,.F.) ;
#63613=ORIENTED_EDGE('',*,*,#46933,.T.) ;
#63614=ORIENTED_EDGE('',*,*,#44934,.F.) ;
#63615=ORIENTED_EDGE('',*,*,#46934,.T.) ;
#63616=ORIENTED_EDGE('',*,*,#46380,.F.) ;
#63617=ORIENTED_EDGE('',*,*,#46935,.F.) ;
#63618=ORIENTED_EDGE('',*,*,#46436,.F.) ;
#63619=ORIENTED_EDGE('',*,*,#46936,.F.) ;
#63620=ORIENTED_EDGE('',*,*,#44967,.F.) ;
#63621=ORIENTED_EDGE('',*,*,#46433,.F.) ;
#63622=ORIENTED_EDGE('',*,*,#46935,.T.) ;
#63623=ORIENTED_EDGE('',*,*,#46937,.F.) ;
#63624=ORIENTED_EDGE('',*,*,#46936,.T.) ;
#63625=ORIENTED_EDGE('',*,*,#46439,.F.) ;
#63626=ORIENTED_EDGE('',*,*,#46938,.F.) ;
#63627=ORIENTED_EDGE('',*,*,#46937,.T.) ;
#63628=ORIENTED_EDGE('',*,*,#44966,.F.) ;
#63629=ORIENTED_EDGE('',*,*,#46939,.F.) ;
#63630=ORIENTED_EDGE('',*,*,#46430,.F.) ;
#63631=ORIENTED_EDGE('',*,*,#46938,.T.) ;
#63632=ORIENTED_EDGE('',*,*,#46442,.F.) ;
#63633=ORIENTED_EDGE('',*,*,#46940,.F.) ;
#63634=ORIENTED_EDGE('',*,*,#44968,.F.) ;
#63635=ORIENTED_EDGE('',*,*,#46939,.T.) ;
#63636=ORIENTED_EDGE('',*,*,#44965,.F.) ;
#63637=ORIENTED_EDGE('',*,*,#46941,.F.) ;
#63638=ORIENTED_EDGE('',*,*,#46427,.F.) ;
#63639=ORIENTED_EDGE('',*,*,#46940,.T.) ;
#63640=ORIENTED_EDGE('',*,*,#46445,.F.) ;
#63641=ORIENTED_EDGE('',*,*,#46942,.F.) ;
#63642=ORIENTED_EDGE('',*,*,#44969,.F.) ;
#63643=ORIENTED_EDGE('',*,*,#46941,.T.) ;
#63644=ORIENTED_EDGE('',*,*,#44964,.F.) ;
#63645=ORIENTED_EDGE('',*,*,#44294,.F.) ;
#63646=ORIENTED_EDGE('',*,*,#46424,.F.) ;
#63647=ORIENTED_EDGE('',*,*,#46942,.T.) ;
#63648=ORIENTED_EDGE('',*,*,#46448,.F.) ;
#63649=ORIENTED_EDGE('',*,*,#46943,.F.) ;
#63650=ORIENTED_EDGE('',*,*,#44970,.F.) ;
#63651=ORIENTED_EDGE('',*,*,#46943,.T.) ;
#63652=ORIENTED_EDGE('',*,*,#46451,.F.) ;
#63653=ORIENTED_EDGE('',*,*,#46944,.F.) ;
#63654=ORIENTED_EDGE('',*,*,#44971,.F.) ;
#63655=ORIENTED_EDGE('',*,*,#44292,.T.) ;
#63656=ORIENTED_EDGE('',*,*,#44963,.F.) ;
#63657=ORIENTED_EDGE('',*,*,#46945,.F.) ;
#63658=ORIENTED_EDGE('',*,*,#46421,.F.) ;
#63659=ORIENTED_EDGE('',*,*,#46944,.T.) ;
#63660=ORIENTED_EDGE('',*,*,#46454,.F.) ;
#63661=ORIENTED_EDGE('',*,*,#46946,.F.) ;
#63662=ORIENTED_EDGE('',*,*,#44972,.F.) ;
#63663=ORIENTED_EDGE('',*,*,#46945,.T.) ;
#63664=ORIENTED_EDGE('',*,*,#44962,.F.) ;
#63665=ORIENTED_EDGE('',*,*,#46947,.F.) ;
#63666=ORIENTED_EDGE('',*,*,#46419,.F.) ;
#63667=ORIENTED_EDGE('',*,*,#46946,.T.) ;
#63668=ORIENTED_EDGE('',*,*,#46457,.F.) ;
#63669=ORIENTED_EDGE('',*,*,#46948,.F.) ;
#63670=ORIENTED_EDGE('',*,*,#44973,.F.) ;
#63671=ORIENTED_EDGE('',*,*,#46947,.T.) ;
#63672=ORIENTED_EDGE('',*,*,#44961,.F.) ;
#63673=ORIENTED_EDGE('',*,*,#46949,.F.) ;
#63674=ORIENTED_EDGE('',*,*,#46417,.F.) ;
#63675=ORIENTED_EDGE('',*,*,#46948,.T.) ;
#63676=ORIENTED_EDGE('',*,*,#46460,.F.) ;
#63677=ORIENTED_EDGE('',*,*,#46950,.F.) ;
#63678=ORIENTED_EDGE('',*,*,#44974,.F.) ;
#63679=ORIENTED_EDGE('',*,*,#46949,.T.) ;
#63680=ORIENTED_EDGE('',*,*,#44960,.F.) ;
#63681=ORIENTED_EDGE('',*,*,#46951,.F.) ;
#63682=ORIENTED_EDGE('',*,*,#46414,.F.) ;
#63683=ORIENTED_EDGE('',*,*,#46950,.T.) ;
#63684=ORIENTED_EDGE('',*,*,#46463,.F.) ;
#63685=ORIENTED_EDGE('',*,*,#46952,.F.) ;
#63686=ORIENTED_EDGE('',*,*,#44975,.F.) ;
#63687=ORIENTED_EDGE('',*,*,#46951,.T.) ;
#63688=ORIENTED_EDGE('',*,*,#44959,.F.) ;
#63689=ORIENTED_EDGE('',*,*,#46953,.F.) ;
#63690=ORIENTED_EDGE('',*,*,#46411,.F.) ;
#63691=ORIENTED_EDGE('',*,*,#46952,.T.) ;
#63692=ORIENTED_EDGE('',*,*,#46466,.F.) ;
#63693=ORIENTED_EDGE('',*,*,#46954,.F.) ;
#63694=ORIENTED_EDGE('',*,*,#44976,.F.) ;
#63695=ORIENTED_EDGE('',*,*,#46408,.F.) ;
#63696=ORIENTED_EDGE('',*,*,#46953,.T.) ;
#63697=ORIENTED_EDGE('',*,*,#46955,.F.) ;
#63698=ORIENTED_EDGE('',*,*,#46954,.T.) ;
#63699=ORIENTED_EDGE('',*,*,#46469,.F.) ;
#63700=ORIENTED_EDGE('',*,*,#46956,.F.) ;
#63701=ORIENTED_EDGE('',*,*,#44977,.F.) ;
#63702=ORIENTED_EDGE('',*,*,#46955,.T.) ;
#63703=ORIENTED_EDGE('',*,*,#44958,.F.) ;
#63704=ORIENTED_EDGE('',*,*,#46957,.F.) ;
#63705=ORIENTED_EDGE('',*,*,#46405,.F.) ;
#63706=ORIENTED_EDGE('',*,*,#46956,.T.) ;
#63707=ORIENTED_EDGE('',*,*,#46472,.F.) ;
#63708=ORIENTED_EDGE('',*,*,#46958,.F.) ;
#63709=ORIENTED_EDGE('',*,*,#44978,.F.) ;
#63710=ORIENTED_EDGE('',*,*,#46402,.F.) ;
#63711=ORIENTED_EDGE('',*,*,#46957,.T.) ;
#63712=ORIENTED_EDGE('',*,*,#46959,.F.) ;
#63713=ORIENTED_EDGE('',*,*,#46958,.T.) ;
#63714=ORIENTED_EDGE('',*,*,#46475,.F.) ;
#63715=ORIENTED_EDGE('',*,*,#46960,.F.) ;
#63716=ORIENTED_EDGE('',*,*,#44956,.F.) ;
#63717=ORIENTED_EDGE('',*,*,#46959,.T.) ;
#63718=ORIENTED_EDGE('',*,*,#44957,.F.) ;
#63719=ORIENTED_EDGE('',*,*,#46960,.T.) ;
#63720=ORIENTED_EDGE('',*,*,#46477,.F.) ;
#63721=ORIENTED_EDGE('',*,*,#46961,.F.) ;
#63722=ORIENTED_EDGE('',*,*,#46533,.F.) ;
#63723=ORIENTED_EDGE('',*,*,#46962,.F.) ;
#63724=ORIENTED_EDGE('',*,*,#44990,.F.) ;
#63725=ORIENTED_EDGE('',*,*,#46530,.F.) ;
#63726=ORIENTED_EDGE('',*,*,#46961,.T.) ;
#63727=ORIENTED_EDGE('',*,*,#46963,.F.) ;
#63728=ORIENTED_EDGE('',*,*,#46962,.T.) ;
#63729=ORIENTED_EDGE('',*,*,#46536,.F.) ;
#63730=ORIENTED_EDGE('',*,*,#46964,.F.) ;
#63731=ORIENTED_EDGE('',*,*,#46963,.T.) ;
#63732=ORIENTED_EDGE('',*,*,#44989,.F.) ;
#63733=ORIENTED_EDGE('',*,*,#46965,.F.) ;
#63734=ORIENTED_EDGE('',*,*,#46527,.F.) ;
#63735=ORIENTED_EDGE('',*,*,#46964,.T.) ;
#63736=ORIENTED_EDGE('',*,*,#46539,.F.) ;
#63737=ORIENTED_EDGE('',*,*,#46966,.F.) ;
#63738=ORIENTED_EDGE('',*,*,#44991,.F.) ;
#63739=ORIENTED_EDGE('',*,*,#46965,.T.) ;
#63740=ORIENTED_EDGE('',*,*,#44988,.F.) ;
#63741=ORIENTED_EDGE('',*,*,#46967,.F.) ;
#63742=ORIENTED_EDGE('',*,*,#46524,.F.) ;
#63743=ORIENTED_EDGE('',*,*,#46966,.T.) ;
#63744=ORIENTED_EDGE('',*,*,#46542,.F.) ;
#63745=ORIENTED_EDGE('',*,*,#46968,.F.) ;
#63746=ORIENTED_EDGE('',*,*,#44992,.F.) ;
#63747=ORIENTED_EDGE('',*,*,#46967,.T.) ;
#63748=ORIENTED_EDGE('',*,*,#44987,.F.) ;
#63749=ORIENTED_EDGE('',*,*,#44290,.F.) ;
#63750=ORIENTED_EDGE('',*,*,#46521,.F.) ;
#63751=ORIENTED_EDGE('',*,*,#46968,.T.) ;
#63752=ORIENTED_EDGE('',*,*,#46545,.F.) ;
#63753=ORIENTED_EDGE('',*,*,#46969,.F.) ;
#63754=ORIENTED_EDGE('',*,*,#44993,.F.) ;
#63755=ORIENTED_EDGE('',*,*,#46969,.T.) ;
#63756=ORIENTED_EDGE('',*,*,#46548,.F.) ;
#63757=ORIENTED_EDGE('',*,*,#46970,.F.) ;
#63758=ORIENTED_EDGE('',*,*,#44994,.F.) ;
#63759=ORIENTED_EDGE('',*,*,#44288,.T.) ;
#63760=ORIENTED_EDGE('',*,*,#44986,.F.) ;
#63761=ORIENTED_EDGE('',*,*,#46971,.F.) ;
#63762=ORIENTED_EDGE('',*,*,#46518,.F.) ;
#63763=ORIENTED_EDGE('',*,*,#46970,.T.) ;
#63764=ORIENTED_EDGE('',*,*,#46551,.F.) ;
#63765=ORIENTED_EDGE('',*,*,#46972,.F.) ;
#63766=ORIENTED_EDGE('',*,*,#44995,.F.) ;
#63767=ORIENTED_EDGE('',*,*,#46971,.T.) ;
#63768=ORIENTED_EDGE('',*,*,#44985,.F.) ;
#63769=ORIENTED_EDGE('',*,*,#46973,.F.) ;
#63770=ORIENTED_EDGE('',*,*,#46516,.F.) ;
#63771=ORIENTED_EDGE('',*,*,#46972,.T.) ;
#63772=ORIENTED_EDGE('',*,*,#46554,.F.) ;
#63773=ORIENTED_EDGE('',*,*,#46974,.F.) ;
#63774=ORIENTED_EDGE('',*,*,#44996,.F.) ;
#63775=ORIENTED_EDGE('',*,*,#46973,.T.) ;
#63776=ORIENTED_EDGE('',*,*,#44984,.F.) ;
#63777=ORIENTED_EDGE('',*,*,#46975,.F.) ;
#63778=ORIENTED_EDGE('',*,*,#46514,.F.) ;
#63779=ORIENTED_EDGE('',*,*,#46974,.T.) ;
#63780=ORIENTED_EDGE('',*,*,#46557,.F.) ;
#63781=ORIENTED_EDGE('',*,*,#46976,.F.) ;
#63782=ORIENTED_EDGE('',*,*,#44997,.F.) ;
#63783=ORIENTED_EDGE('',*,*,#46975,.T.) ;
#63784=ORIENTED_EDGE('',*,*,#44983,.F.) ;
#63785=ORIENTED_EDGE('',*,*,#46977,.F.) ;
#63786=ORIENTED_EDGE('',*,*,#46511,.F.) ;
#63787=ORIENTED_EDGE('',*,*,#46976,.T.) ;
#63788=ORIENTED_EDGE('',*,*,#46560,.F.) ;
#63789=ORIENTED_EDGE('',*,*,#46978,.F.) ;
#63790=ORIENTED_EDGE('',*,*,#44998,.F.) ;
#63791=ORIENTED_EDGE('',*,*,#46977,.T.) ;
#63792=ORIENTED_EDGE('',*,*,#44982,.F.) ;
#63793=ORIENTED_EDGE('',*,*,#46979,.F.) ;
#63794=ORIENTED_EDGE('',*,*,#46508,.F.) ;
#63795=ORIENTED_EDGE('',*,*,#46978,.T.) ;
#63796=ORIENTED_EDGE('',*,*,#46563,.F.) ;
#63797=ORIENTED_EDGE('',*,*,#46980,.F.) ;
#63798=ORIENTED_EDGE('',*,*,#44999,.F.) ;
#63799=ORIENTED_EDGE('',*,*,#46505,.F.) ;
#63800=ORIENTED_EDGE('',*,*,#46979,.T.) ;
#63801=ORIENTED_EDGE('',*,*,#46981,.F.) ;
#63802=ORIENTED_EDGE('',*,*,#46980,.T.) ;
#63803=ORIENTED_EDGE('',*,*,#46566,.F.) ;
#63804=ORIENTED_EDGE('',*,*,#46982,.F.) ;
#63805=ORIENTED_EDGE('',*,*,#45000,.F.) ;
#63806=ORIENTED_EDGE('',*,*,#46981,.T.) ;
#63807=ORIENTED_EDGE('',*,*,#44981,.F.) ;
#63808=ORIENTED_EDGE('',*,*,#46983,.F.) ;
#63809=ORIENTED_EDGE('',*,*,#46502,.F.) ;
#63810=ORIENTED_EDGE('',*,*,#46982,.T.) ;
#63811=ORIENTED_EDGE('',*,*,#46569,.F.) ;
#63812=ORIENTED_EDGE('',*,*,#46984,.F.) ;
#63813=ORIENTED_EDGE('',*,*,#45001,.F.) ;
#63814=ORIENTED_EDGE('',*,*,#46499,.F.) ;
#63815=ORIENTED_EDGE('',*,*,#46983,.T.) ;
#63816=ORIENTED_EDGE('',*,*,#46985,.F.) ;
#63817=ORIENTED_EDGE('',*,*,#46984,.T.) ;
#63818=ORIENTED_EDGE('',*,*,#46572,.F.) ;
#63819=ORIENTED_EDGE('',*,*,#46986,.F.) ;
#63820=ORIENTED_EDGE('',*,*,#44979,.F.) ;
#63821=ORIENTED_EDGE('',*,*,#46985,.T.) ;
#63822=ORIENTED_EDGE('',*,*,#44980,.F.) ;
#63823=ORIENTED_EDGE('',*,*,#46986,.T.) ;
#63824=ORIENTED_EDGE('',*,*,#46574,.F.) ;
#63825=ORIENTED_EDGE('',*,*,#46987,.F.) ;
#63826=ORIENTED_EDGE('',*,*,#45580,.F.) ;
#63827=ORIENTED_EDGE('',*,*,#46988,.F.) ;
#63828=ORIENTED_EDGE('',*,*,#45538,.F.) ;
#63829=ORIENTED_EDGE('',*,*,#46989,.F.) ;
#63830=ORIENTED_EDGE('',*,*,#45581,.F.) ;
#63831=ORIENTED_EDGE('',*,*,#46990,.F.) ;
#63832=ORIENTED_EDGE('',*,*,#45575,.F.) ;
#63833=ORIENTED_EDGE('',*,*,#46991,.F.) ;
#63834=ORIENTED_EDGE('',*,*,#46989,.T.) ;
#63835=ORIENTED_EDGE('',*,*,#46992,.F.) ;
#63836=ORIENTED_EDGE('',*,*,#46993,.F.) ;
#63837=ORIENTED_EDGE('',*,*,#46988,.T.) ;
#63838=ORIENTED_EDGE('',*,*,#46994,.F.) ;
#63839=ORIENTED_EDGE('',*,*,#46987,.T.) ;
#63840=ORIENTED_EDGE('',*,*,#45537,.T.) ;
#63841=ORIENTED_EDGE('',*,*,#46995,.F.) ;
#63842=ORIENTED_EDGE('',*,*,#46990,.T.) ;
#63843=ORIENTED_EDGE('',*,*,#46992,.T.) ;
#63844=ORIENTED_EDGE('',*,*,#45578,.F.) ;
#63845=ORIENTED_EDGE('',*,*,#46996,.F.) ;
#63846=ORIENTED_EDGE('',*,*,#44276,.T.) ;
#63847=ORIENTED_EDGE('',*,*,#46997,.T.) ;
#63848=ORIENTED_EDGE('',*,*,#46998,.F.) ;
#63849=ORIENTED_EDGE('',*,*,#46991,.T.) ;
#63850=ORIENTED_EDGE('',*,*,#46999,.F.) ;
#63851=ORIENTED_EDGE('',*,*,#47000,.T.) ;
#63852=ORIENTED_EDGE('',*,*,#47001,.F.) ;
#63853=ORIENTED_EDGE('',*,*,#44474,.F.) ;
#63854=ORIENTED_EDGE('',*,*,#47002,.F.) ;
#63855=ORIENTED_EDGE('',*,*,#45582,.F.) ;
#63856=ORIENTED_EDGE('',*,*,#46994,.T.) ;
#63857=ORIENTED_EDGE('',*,*,#45579,.F.) ;
#63858=ORIENTED_EDGE('',*,*,#47003,.F.) ;
#63859=ORIENTED_EDGE('',*,*,#45585,.F.) ;
#63860=ORIENTED_EDGE('',*,*,#46993,.T.) ;
#63861=ORIENTED_EDGE('',*,*,#45584,.F.) ;
#63862=ORIENTED_EDGE('',*,*,#47004,.F.) ;
#63863=ORIENTED_EDGE('',*,*,#45529,.F.) ;
#63864=ORIENTED_EDGE('',*,*,#46995,.T.) ;
#63865=ORIENTED_EDGE('',*,*,#45536,.F.) ;
#63866=ORIENTED_EDGE('',*,*,#47005,.F.) ;
#63867=ORIENTED_EDGE('',*,*,#45576,.F.) ;
#63868=ORIENTED_EDGE('',*,*,#47006,.F.) ;
#63869=ORIENTED_EDGE('',*,*,#45577,.F.) ;
#63870=ORIENTED_EDGE('',*,*,#47007,.F.) ;
#63871=ORIENTED_EDGE('',*,*,#45572,.F.) ;
#63872=ORIENTED_EDGE('',*,*,#46996,.T.) ;
#63873=ORIENTED_EDGE('',*,*,#47006,.T.) ;
#63874=ORIENTED_EDGE('',*,*,#44277,.F.) ;
#63875=ORIENTED_EDGE('',*,*,#47002,.T.) ;
#63876=ORIENTED_EDGE('',*,*,#44484,.T.) ;
#63877=ORIENTED_EDGE('',*,*,#47008,.F.) ;
#63878=ORIENTED_EDGE('',*,*,#47003,.T.) ;
#63879=ORIENTED_EDGE('',*,*,#47009,.F.) ;
#63880=ORIENTED_EDGE('',*,*,#47004,.T.) ;
#63881=ORIENTED_EDGE('',*,*,#47010,.F.) ;
#63882=ORIENTED_EDGE('',*,*,#44571,.T.) ;
#63883=ORIENTED_EDGE('',*,*,#47005,.T.) ;
#63884=ORIENTED_EDGE('',*,*,#45535,.T.) ;
#63885=ORIENTED_EDGE('',*,*,#47011,.F.) ;
#63886=ORIENTED_EDGE('',*,*,#47007,.T.) ;
#63887=ORIENTED_EDGE('',*,*,#47008,.T.) ;
#63888=ORIENTED_EDGE('',*,*,#44483,.F.) ;
#63889=ORIENTED_EDGE('',*,*,#47012,.F.) ;
#63890=ORIENTED_EDGE('',*,*,#45586,.F.) ;
#63891=ORIENTED_EDGE('',*,*,#47010,.T.) ;
#63892=ORIENTED_EDGE('',*,*,#45583,.F.) ;
#63893=ORIENTED_EDGE('',*,*,#47013,.F.) ;
#63894=ORIENTED_EDGE('',*,*,#44572,.F.) ;
#63895=ORIENTED_EDGE('',*,*,#45530,.F.) ;
#63896=ORIENTED_EDGE('',*,*,#47009,.T.) ;
#63897=ORIENTED_EDGE('',*,*,#47014,.F.) ;
#63898=ORIENTED_EDGE('',*,*,#47015,.F.) ;
#63899=ORIENTED_EDGE('',*,*,#47011,.T.) ;
#63900=ORIENTED_EDGE('',*,*,#45534,.F.) ;
#63901=ORIENTED_EDGE('',*,*,#47016,.F.) ;
#63902=ORIENTED_EDGE('',*,*,#45573,.F.) ;
#63903=ORIENTED_EDGE('',*,*,#47017,.F.) ;
#63904=ORIENTED_EDGE('',*,*,#45574,.F.) ;
#63905=ORIENTED_EDGE('',*,*,#47018,.F.) ;
#63906=ORIENTED_EDGE('',*,*,#45568,.F.) ;
#63907=ORIENTED_EDGE('',*,*,#44279,.T.) ;
#63908=ORIENTED_EDGE('',*,*,#47017,.T.) ;
#63909=ORIENTED_EDGE('',*,*,#47019,.F.) ;
#63910=ORIENTED_EDGE('',*,*,#44478,.T.) ;
#63911=ORIENTED_EDGE('',*,*,#47013,.T.) ;
#63912=ORIENTED_EDGE('',*,*,#47012,.T.) ;
#63913=ORIENTED_EDGE('',*,*,#47020,.F.) ;
#63914=ORIENTED_EDGE('',*,*,#47021,.F.) ;
#63915=ORIENTED_EDGE('',*,*,#44591,.F.) ;
#63916=ORIENTED_EDGE('',*,*,#47022,.F.) ;
#63917=ORIENTED_EDGE('',*,*,#47023,.F.) ;
#63918=ORIENTED_EDGE('',*,*,#47014,.T.) ;
#63919=ORIENTED_EDGE('',*,*,#44575,.F.) ;
#63920=ORIENTED_EDGE('',*,*,#47022,.T.) ;
#63921=ORIENTED_EDGE('',*,*,#44743,.F.) ;
#63922=ORIENTED_EDGE('',*,*,#47015,.T.) ;
#63923=ORIENTED_EDGE('',*,*,#47024,.F.) ;
#63924=ORIENTED_EDGE('',*,*,#47025,.F.) ;
#63925=ORIENTED_EDGE('',*,*,#47018,.T.) ;
#63926=ORIENTED_EDGE('',*,*,#47016,.T.) ;
#63927=ORIENTED_EDGE('',*,*,#47026,.F.) ;
#63928=ORIENTED_EDGE('',*,*,#47019,.T.) ;
#63929=ORIENTED_EDGE('',*,*,#45571,.F.) ;
#63930=ORIENTED_EDGE('',*,*,#47027,.F.) ;
#63931=ORIENTED_EDGE('',*,*,#44479,.F.) ;
#63932=ORIENTED_EDGE('',*,*,#47020,.T.) ;
#63933=ORIENTED_EDGE('',*,*,#44482,.F.) ;
#63934=ORIENTED_EDGE('',*,*,#47028,.F.) ;
#63935=ORIENTED_EDGE('',*,*,#44573,.F.) ;
#63936=ORIENTED_EDGE('',*,*,#47021,.T.) ;
#63937=ORIENTED_EDGE('',*,*,#44574,.F.) ;
#63938=ORIENTED_EDGE('',*,*,#47029,.F.) ;
#63939=ORIENTED_EDGE('',*,*,#44666,.F.) ;
#63940=ORIENTED_EDGE('',*,*,#47023,.T.) ;
#63941=ORIENTED_EDGE('',*,*,#44742,.T.) ;
#63942=ORIENTED_EDGE('',*,*,#47030,.F.) ;
#63943=ORIENTED_EDGE('',*,*,#47024,.T.) ;
#63944=ORIENTED_EDGE('',*,*,#45531,.F.) ;
#63945=ORIENTED_EDGE('',*,*,#47025,.T.) ;
#63946=ORIENTED_EDGE('',*,*,#47031,.F.) ;
#63947=ORIENTED_EDGE('',*,*,#47032,.F.) ;
#63948=ORIENTED_EDGE('',*,*,#47026,.T.) ;
#63949=ORIENTED_EDGE('',*,*,#45533,.F.) ;
#63950=ORIENTED_EDGE('',*,*,#47033,.F.) ;
#63951=ORIENTED_EDGE('',*,*,#45569,.F.) ;
#63952=ORIENTED_EDGE('',*,*,#47034,.F.) ;
#63953=ORIENTED_EDGE('',*,*,#45570,.F.) ;
#63954=ORIENTED_EDGE('',*,*,#47035,.F.) ;
#63955=ORIENTED_EDGE('',*,*,#44570,.F.) ;
#63956=ORIENTED_EDGE('',*,*,#47027,.T.) ;
#63957=ORIENTED_EDGE('',*,*,#47034,.T.) ;
#63958=ORIENTED_EDGE('',*,*,#47036,.F.) ;
#63959=ORIENTED_EDGE('',*,*,#47029,.T.) ;
#63960=ORIENTED_EDGE('',*,*,#47028,.T.) ;
#63961=ORIENTED_EDGE('',*,*,#47037,.F.) ;
#63962=ORIENTED_EDGE('',*,*,#44667,.T.) ;
#63963=ORIENTED_EDGE('',*,*,#47038,.F.) ;
#63964=ORIENTED_EDGE('',*,*,#47031,.T.) ;
#63965=ORIENTED_EDGE('',*,*,#47030,.T.) ;
#63966=ORIENTED_EDGE('',*,*,#44741,.F.) ;
#63967=ORIENTED_EDGE('',*,*,#47032,.T.) ;
#63968=ORIENTED_EDGE('',*,*,#47039,.F.) ;
#63969=ORIENTED_EDGE('',*,*,#47040,.F.) ;
#63970=ORIENTED_EDGE('',*,*,#47035,.T.) ;
#63971=ORIENTED_EDGE('',*,*,#47033,.T.) ;
#63972=ORIENTED_EDGE('',*,*,#47041,.F.) ;
#63973=ORIENTED_EDGE('',*,*,#44566,.T.) ;
#63974=ORIENTED_EDGE('',*,*,#47036,.T.) ;
#63975=ORIENTED_EDGE('',*,*,#44569,.F.) ;
#63976=ORIENTED_EDGE('',*,*,#47042,.F.) ;
#63977=ORIENTED_EDGE('',*,*,#44480,.F.) ;
#63978=ORIENTED_EDGE('',*,*,#47037,.T.) ;
#63979=ORIENTED_EDGE('',*,*,#44481,.F.) ;
#63980=ORIENTED_EDGE('',*,*,#47043,.F.) ;
#63981=ORIENTED_EDGE('',*,*,#44668,.F.) ;
#63982=ORIENTED_EDGE('',*,*,#47038,.T.) ;
#63983=ORIENTED_EDGE('',*,*,#44740,.T.) ;
#63984=ORIENTED_EDGE('',*,*,#47044,.F.) ;
#63985=ORIENTED_EDGE('',*,*,#47039,.T.) ;
#63986=ORIENTED_EDGE('',*,*,#45532,.F.) ;
#63987=ORIENTED_EDGE('',*,*,#47040,.T.) ;
#63988=ORIENTED_EDGE('',*,*,#47045,.F.) ;
#63989=ORIENTED_EDGE('',*,*,#47041,.T.) ;
#63990=ORIENTED_EDGE('',*,*,#47043,.T.) ;
#63991=ORIENTED_EDGE('',*,*,#47042,.T.) ;
#63992=ORIENTED_EDGE('',*,*,#47046,.F.) ;
#63993=ORIENTED_EDGE('',*,*,#44669,.T.) ;
#63994=ORIENTED_EDGE('',*,*,#47044,.T.) ;
#63995=ORIENTED_EDGE('',*,*,#44739,.F.) ;
#63996=ORIENTED_EDGE('',*,*,#47047,.F.) ;
#63997=ORIENTED_EDGE('',*,*,#44567,.F.) ;
#63998=ORIENTED_EDGE('',*,*,#47045,.T.) ;
#63999=ORIENTED_EDGE('',*,*,#47046,.T.) ;
#64000=ORIENTED_EDGE('',*,*,#44568,.F.) ;
#64001=ORIENTED_EDGE('',*,*,#47048,.F.) ;
#64002=ORIENTED_EDGE('',*,*,#44670,.F.) ;
#64003=ORIENTED_EDGE('',*,*,#47047,.T.) ;
#64004=ORIENTED_EDGE('',*,*,#44597,.F.) ;
#64005=ORIENTED_EDGE('',*,*,#47048,.T.) ;
#64006=ORIENTED_EDGE('',*,*,#47049,.F.) ;
#64007=ORIENTED_EDGE('',*,*,#46440,.F.) ;
#64008=ORIENTED_EDGE('',*,*,#47050,.F.) ;
#64009=ORIENTED_EDGE('',*,*,#46487,.F.) ;
#64010=ORIENTED_EDGE('',*,*,#47050,.T.) ;
#64011=ORIENTED_EDGE('',*,*,#46437,.F.) ;
#64012=ORIENTED_EDGE('',*,*,#47051,.F.) ;
#64013=ORIENTED_EDGE('',*,*,#46488,.F.) ;
#64014=ORIENTED_EDGE('',*,*,#46443,.F.) ;
#64015=ORIENTED_EDGE('',*,*,#47049,.T.) ;
#64016=ORIENTED_EDGE('',*,*,#47052,.F.) ;
#64017=ORIENTED_EDGE('',*,*,#47051,.T.) ;
#64018=ORIENTED_EDGE('',*,*,#46434,.F.) ;
#64019=ORIENTED_EDGE('',*,*,#47053,.F.) ;
#64020=ORIENTED_EDGE('',*,*,#46489,.F.) ;
#64021=ORIENTED_EDGE('',*,*,#47052,.T.) ;
#64022=ORIENTED_EDGE('',*,*,#46486,.F.) ;
#64023=ORIENTED_EDGE('',*,*,#47054,.F.) ;
#64024=ORIENTED_EDGE('',*,*,#46446,.F.) ;
#64025=ORIENTED_EDGE('',*,*,#47053,.T.) ;
#64026=ORIENTED_EDGE('',*,*,#46431,.F.) ;
#64027=ORIENTED_EDGE('',*,*,#47055,.F.) ;
#64028=ORIENTED_EDGE('',*,*,#46490,.F.) ;
#64029=ORIENTED_EDGE('',*,*,#46449,.F.) ;
#64030=ORIENTED_EDGE('',*,*,#47054,.T.) ;
#64031=ORIENTED_EDGE('',*,*,#47056,.F.) ;
#64032=ORIENTED_EDGE('',*,*,#47055,.T.) ;
#64033=ORIENTED_EDGE('',*,*,#46428,.F.) ;
#64034=ORIENTED_EDGE('',*,*,#47057,.F.) ;
#64035=ORIENTED_EDGE('',*,*,#46491,.F.) ;
#64036=ORIENTED_EDGE('',*,*,#47056,.T.) ;
#64037=ORIENTED_EDGE('',*,*,#46485,.F.) ;
#64038=ORIENTED_EDGE('',*,*,#47058,.F.) ;
#64039=ORIENTED_EDGE('',*,*,#46452,.F.) ;
#64040=ORIENTED_EDGE('',*,*,#47057,.T.) ;
#64041=ORIENTED_EDGE('',*,*,#46425,.F.) ;
#64042=ORIENTED_EDGE('',*,*,#47059,.F.) ;
#64043=ORIENTED_EDGE('',*,*,#46455,.F.) ;
#64044=ORIENTED_EDGE('',*,*,#47058,.T.) ;
#64045=ORIENTED_EDGE('',*,*,#47060,.F.) ;
#64046=ORIENTED_EDGE('',*,*,#47059,.T.) ;
#64047=ORIENTED_EDGE('',*,*,#46422,.F.) ;
#64048=ORIENTED_EDGE('',*,*,#47061,.F.) ;
#64049=ORIENTED_EDGE('',*,*,#46492,.F.) ;
#64050=ORIENTED_EDGE('',*,*,#47060,.T.) ;
#64051=ORIENTED_EDGE('',*,*,#46484,.F.) ;
#64052=ORIENTED_EDGE('',*,*,#47062,.F.) ;
#64053=ORIENTED_EDGE('',*,*,#46458,.F.) ;
#64054=ORIENTED_EDGE('',*,*,#47061,.T.) ;
#64055=ORIENTED_EDGE('',*,*,#44348,.F.) ;
#64056=ORIENTED_EDGE('',*,*,#47063,.F.) ;
#64057=ORIENTED_EDGE('',*,*,#46461,.F.) ;
#64058=ORIENTED_EDGE('',*,*,#47062,.T.) ;
#64059=ORIENTED_EDGE('',*,*,#47064,.F.) ;
#64060=ORIENTED_EDGE('',*,*,#47063,.T.) ;
#64061=ORIENTED_EDGE('',*,*,#46420,.F.) ;
#64062=ORIENTED_EDGE('',*,*,#44275,.F.) ;
#64063=ORIENTED_EDGE('',*,*,#46493,.F.) ;
#64064=ORIENTED_EDGE('',*,*,#47064,.T.) ;
#64065=ORIENTED_EDGE('',*,*,#46483,.F.) ;
#64066=ORIENTED_EDGE('',*,*,#47065,.F.) ;
#64067=ORIENTED_EDGE('',*,*,#46464,.F.) ;
#64068=ORIENTED_EDGE('',*,*,#46467,.F.) ;
#64069=ORIENTED_EDGE('',*,*,#47065,.T.) ;
#64070=ORIENTED_EDGE('',*,*,#47066,.F.) ;
#64071=ORIENTED_EDGE('',*,*,#44274,.T.) ;
#64072=ORIENTED_EDGE('',*,*,#46415,.F.) ;
#64073=ORIENTED_EDGE('',*,*,#47067,.F.) ;
#64074=ORIENTED_EDGE('',*,*,#46494,.F.) ;
#64075=ORIENTED_EDGE('',*,*,#47066,.T.) ;
#64076=ORIENTED_EDGE('',*,*,#46482,.F.) ;
#64077=ORIENTED_EDGE('',*,*,#47068,.F.) ;
#64078=ORIENTED_EDGE('',*,*,#46470,.F.) ;
#64079=ORIENTED_EDGE('',*,*,#47067,.T.) ;
#64080=ORIENTED_EDGE('',*,*,#46412,.F.) ;
#64081=ORIENTED_EDGE('',*,*,#47069,.F.) ;
#64082=ORIENTED_EDGE('',*,*,#46473,.F.) ;
#64083=ORIENTED_EDGE('',*,*,#47068,.T.) ;
#64084=ORIENTED_EDGE('',*,*,#47070,.F.) ;
#64085=ORIENTED_EDGE('',*,*,#47069,.T.) ;
#64086=ORIENTED_EDGE('',*,*,#46409,.F.) ;
#64087=ORIENTED_EDGE('',*,*,#47071,.F.) ;
#64088=ORIENTED_EDGE('',*,*,#46495,.F.) ;
#64089=ORIENTED_EDGE('',*,*,#47070,.T.) ;
#64090=ORIENTED_EDGE('',*,*,#46481,.F.) ;
#64091=ORIENTED_EDGE('',*,*,#47072,.F.) ;
#64092=ORIENTED_EDGE('',*,*,#46476,.F.) ;
#64093=ORIENTED_EDGE('',*,*,#47071,.T.) ;
#64094=ORIENTED_EDGE('',*,*,#46406,.F.) ;
#64095=ORIENTED_EDGE('',*,*,#47073,.F.) ;
#64096=ORIENTED_EDGE('',*,*,#46478,.F.) ;
#64097=ORIENTED_EDGE('',*,*,#47072,.T.) ;
#64098=ORIENTED_EDGE('',*,*,#46480,.F.) ;
#64099=ORIENTED_EDGE('',*,*,#47074,.F.) ;
#64100=ORIENTED_EDGE('',*,*,#46400,.F.) ;
#64101=ORIENTED_EDGE('',*,*,#47073,.T.) ;
#64102=ORIENTED_EDGE('',*,*,#46403,.F.) ;
#64103=ORIENTED_EDGE('',*,*,#47074,.T.) ;
#64104=ORIENTED_EDGE('',*,*,#46479,.F.) ;
#64105=ORIENTED_EDGE('',*,*,#47075,.F.) ;
#64106=ORIENTED_EDGE('',*,*,#45599,.F.) ;
#64107=ORIENTED_EDGE('',*,*,#47076,.F.) ;
#64108=ORIENTED_EDGE('',*,*,#45528,.F.) ;
#64109=ORIENTED_EDGE('',*,*,#47077,.F.) ;
#64110=ORIENTED_EDGE('',*,*,#45600,.F.) ;
#64111=ORIENTED_EDGE('',*,*,#47078,.F.) ;
#64112=ORIENTED_EDGE('',*,*,#45594,.F.) ;
#64113=ORIENTED_EDGE('',*,*,#47079,.F.) ;
#64114=ORIENTED_EDGE('',*,*,#47077,.T.) ;
#64115=ORIENTED_EDGE('',*,*,#47080,.F.) ;
#64116=ORIENTED_EDGE('',*,*,#47081,.F.) ;
#64117=ORIENTED_EDGE('',*,*,#47076,.T.) ;
#64118=ORIENTED_EDGE('',*,*,#47082,.F.) ;
#64119=ORIENTED_EDGE('',*,*,#47075,.T.) ;
#64120=ORIENTED_EDGE('',*,*,#45527,.T.) ;
#64121=ORIENTED_EDGE('',*,*,#47083,.F.) ;
#64122=ORIENTED_EDGE('',*,*,#47078,.T.) ;
#64123=ORIENTED_EDGE('',*,*,#47080,.T.) ;
#64124=ORIENTED_EDGE('',*,*,#45597,.F.) ;
#64125=ORIENTED_EDGE('',*,*,#47084,.F.) ;
#64126=ORIENTED_EDGE('',*,*,#44259,.T.) ;
#64127=ORIENTED_EDGE('',*,*,#47085,.T.) ;
#64128=ORIENTED_EDGE('',*,*,#47086,.F.) ;
#64129=ORIENTED_EDGE('',*,*,#47079,.T.) ;
#64130=ORIENTED_EDGE('',*,*,#47087,.F.) ;
#64131=ORIENTED_EDGE('',*,*,#47088,.T.) ;
#64132=ORIENTED_EDGE('',*,*,#47089,.F.) ;
#64133=ORIENTED_EDGE('',*,*,#44463,.F.) ;
#64134=ORIENTED_EDGE('',*,*,#47090,.F.) ;
#64135=ORIENTED_EDGE('',*,*,#45601,.F.) ;
#64136=ORIENTED_EDGE('',*,*,#47082,.T.) ;
#64137=ORIENTED_EDGE('',*,*,#45598,.F.) ;
#64138=ORIENTED_EDGE('',*,*,#47091,.F.) ;
#64139=ORIENTED_EDGE('',*,*,#45604,.F.) ;
#64140=ORIENTED_EDGE('',*,*,#47081,.T.) ;
#64141=ORIENTED_EDGE('',*,*,#45603,.F.) ;
#64142=ORIENTED_EDGE('',*,*,#47092,.F.) ;
#64143=ORIENTED_EDGE('',*,*,#45519,.F.) ;
#64144=ORIENTED_EDGE('',*,*,#47083,.T.) ;
#64145=ORIENTED_EDGE('',*,*,#45526,.F.) ;
#64146=ORIENTED_EDGE('',*,*,#47093,.F.) ;
#64147=ORIENTED_EDGE('',*,*,#45595,.F.) ;
#64148=ORIENTED_EDGE('',*,*,#47094,.F.) ;
#64149=ORIENTED_EDGE('',*,*,#45596,.F.) ;
#64150=ORIENTED_EDGE('',*,*,#47095,.F.) ;
#64151=ORIENTED_EDGE('',*,*,#45591,.F.) ;
#64152=ORIENTED_EDGE('',*,*,#47084,.T.) ;
#64153=ORIENTED_EDGE('',*,*,#47094,.T.) ;
#64154=ORIENTED_EDGE('',*,*,#44260,.F.) ;
#64155=ORIENTED_EDGE('',*,*,#47090,.T.) ;
#64156=ORIENTED_EDGE('',*,*,#44473,.T.) ;
#64157=ORIENTED_EDGE('',*,*,#47096,.F.) ;
#64158=ORIENTED_EDGE('',*,*,#47091,.T.) ;
#64159=ORIENTED_EDGE('',*,*,#47097,.F.) ;
#64160=ORIENTED_EDGE('',*,*,#47092,.T.) ;
#64161=ORIENTED_EDGE('',*,*,#47098,.F.) ;
#64162=ORIENTED_EDGE('',*,*,#44561,.T.) ;
#64163=ORIENTED_EDGE('',*,*,#47093,.T.) ;
#64164=ORIENTED_EDGE('',*,*,#45525,.T.) ;
#64165=ORIENTED_EDGE('',*,*,#47099,.F.) ;
#64166=ORIENTED_EDGE('',*,*,#47095,.T.) ;
#64167=ORIENTED_EDGE('',*,*,#47096,.T.) ;
#64168=ORIENTED_EDGE('',*,*,#44472,.F.) ;
#64169=ORIENTED_EDGE('',*,*,#47100,.F.) ;
#64170=ORIENTED_EDGE('',*,*,#45605,.F.) ;
#64171=ORIENTED_EDGE('',*,*,#47098,.T.) ;
#64172=ORIENTED_EDGE('',*,*,#45602,.F.) ;
#64173=ORIENTED_EDGE('',*,*,#47101,.F.) ;
#64174=ORIENTED_EDGE('',*,*,#44562,.F.) ;
#64175=ORIENTED_EDGE('',*,*,#45520,.F.) ;
#64176=ORIENTED_EDGE('',*,*,#47097,.T.) ;
#64177=ORIENTED_EDGE('',*,*,#47102,.F.) ;
#64178=ORIENTED_EDGE('',*,*,#47103,.F.) ;
#64179=ORIENTED_EDGE('',*,*,#47099,.T.) ;
#64180=ORIENTED_EDGE('',*,*,#45524,.F.) ;
#64181=ORIENTED_EDGE('',*,*,#47104,.F.) ;
#64182=ORIENTED_EDGE('',*,*,#45592,.F.) ;
#64183=ORIENTED_EDGE('',*,*,#47105,.F.) ;
#64184=ORIENTED_EDGE('',*,*,#45593,.F.) ;
#64185=ORIENTED_EDGE('',*,*,#47106,.F.) ;
#64186=ORIENTED_EDGE('',*,*,#45587,.F.) ;
#64187=ORIENTED_EDGE('',*,*,#44262,.T.) ;
#64188=ORIENTED_EDGE('',*,*,#47105,.T.) ;
#64189=ORIENTED_EDGE('',*,*,#47107,.F.) ;
#64190=ORIENTED_EDGE('',*,*,#44467,.T.) ;
#64191=ORIENTED_EDGE('',*,*,#47101,.T.) ;
#64192=ORIENTED_EDGE('',*,*,#47100,.T.) ;
#64193=ORIENTED_EDGE('',*,*,#47108,.F.) ;
#64194=ORIENTED_EDGE('',*,*,#47109,.F.) ;
#64195=ORIENTED_EDGE('',*,*,#44595,.F.) ;
#64196=ORIENTED_EDGE('',*,*,#47110,.F.) ;
#64197=ORIENTED_EDGE('',*,*,#47111,.F.) ;
#64198=ORIENTED_EDGE('',*,*,#47102,.T.) ;
#64199=ORIENTED_EDGE('',*,*,#44565,.F.) ;
#64200=ORIENTED_EDGE('',*,*,#47110,.T.) ;
#64201=ORIENTED_EDGE('',*,*,#44738,.F.) ;
#64202=ORIENTED_EDGE('',*,*,#47103,.T.) ;
#64203=ORIENTED_EDGE('',*,*,#47112,.F.) ;
#64204=ORIENTED_EDGE('',*,*,#47113,.F.) ;
#64205=ORIENTED_EDGE('',*,*,#47106,.T.) ;
#64206=ORIENTED_EDGE('',*,*,#47104,.T.) ;
#64207=ORIENTED_EDGE('',*,*,#47114,.F.) ;
#64208=ORIENTED_EDGE('',*,*,#47107,.T.) ;
#64209=ORIENTED_EDGE('',*,*,#45590,.F.) ;
#64210=ORIENTED_EDGE('',*,*,#47115,.F.) ;
#64211=ORIENTED_EDGE('',*,*,#44468,.F.) ;
#64212=ORIENTED_EDGE('',*,*,#47108,.T.) ;
#64213=ORIENTED_EDGE('',*,*,#44471,.F.) ;
#64214=ORIENTED_EDGE('',*,*,#47116,.F.) ;
#64215=ORIENTED_EDGE('',*,*,#44563,.F.) ;
#64216=ORIENTED_EDGE('',*,*,#47109,.T.) ;
#64217=ORIENTED_EDGE('',*,*,#44564,.F.) ;
#64218=ORIENTED_EDGE('',*,*,#47117,.F.) ;
#64219=ORIENTED_EDGE('',*,*,#44671,.F.) ;
#64220=ORIENTED_EDGE('',*,*,#47111,.T.) ;
#64221=ORIENTED_EDGE('',*,*,#44737,.T.) ;
#64222=ORIENTED_EDGE('',*,*,#47118,.F.) ;
#64223=ORIENTED_EDGE('',*,*,#47112,.T.) ;
#64224=ORIENTED_EDGE('',*,*,#45521,.F.) ;
#64225=ORIENTED_EDGE('',*,*,#47113,.T.) ;
#64226=ORIENTED_EDGE('',*,*,#47119,.F.) ;
#64227=ORIENTED_EDGE('',*,*,#47120,.F.) ;
#64228=ORIENTED_EDGE('',*,*,#47114,.T.) ;
#64229=ORIENTED_EDGE('',*,*,#45523,.F.) ;
#64230=ORIENTED_EDGE('',*,*,#47121,.F.) ;
#64231=ORIENTED_EDGE('',*,*,#45588,.F.) ;
#64232=ORIENTED_EDGE('',*,*,#47122,.F.) ;
#64233=ORIENTED_EDGE('',*,*,#45589,.F.) ;
#64234=ORIENTED_EDGE('',*,*,#47123,.F.) ;
#64235=ORIENTED_EDGE('',*,*,#44560,.F.) ;
#64236=ORIENTED_EDGE('',*,*,#47115,.T.) ;
#64237=ORIENTED_EDGE('',*,*,#47122,.T.) ;
#64238=ORIENTED_EDGE('',*,*,#47124,.F.) ;
#64239=ORIENTED_EDGE('',*,*,#47117,.T.) ;
#64240=ORIENTED_EDGE('',*,*,#47116,.T.) ;
#64241=ORIENTED_EDGE('',*,*,#47125,.F.) ;
#64242=ORIENTED_EDGE('',*,*,#44672,.T.) ;
#64243=ORIENTED_EDGE('',*,*,#47126,.F.) ;
#64244=ORIENTED_EDGE('',*,*,#47119,.T.) ;
#64245=ORIENTED_EDGE('',*,*,#47118,.T.) ;
#64246=ORIENTED_EDGE('',*,*,#44736,.F.) ;
#64247=ORIENTED_EDGE('',*,*,#47120,.T.) ;
#64248=ORIENTED_EDGE('',*,*,#47127,.F.) ;
#64249=ORIENTED_EDGE('',*,*,#47128,.F.) ;
#64250=ORIENTED_EDGE('',*,*,#47123,.T.) ;
#64251=ORIENTED_EDGE('',*,*,#47121,.T.) ;
#64252=ORIENTED_EDGE('',*,*,#47129,.F.) ;
#64253=ORIENTED_EDGE('',*,*,#44556,.T.) ;
#64254=ORIENTED_EDGE('',*,*,#47124,.T.) ;
#64255=ORIENTED_EDGE('',*,*,#44559,.F.) ;
#64256=ORIENTED_EDGE('',*,*,#47130,.F.) ;
#64257=ORIENTED_EDGE('',*,*,#44469,.F.) ;
#64258=ORIENTED_EDGE('',*,*,#47125,.T.) ;
#64259=ORIENTED_EDGE('',*,*,#44470,.F.) ;
#64260=ORIENTED_EDGE('',*,*,#47131,.F.) ;
#64261=ORIENTED_EDGE('',*,*,#44673,.F.) ;
#64262=ORIENTED_EDGE('',*,*,#47126,.T.) ;
#64263=ORIENTED_EDGE('',*,*,#44735,.T.) ;
#64264=ORIENTED_EDGE('',*,*,#47132,.F.) ;
#64265=ORIENTED_EDGE('',*,*,#47127,.T.) ;
#64266=ORIENTED_EDGE('',*,*,#45522,.F.) ;
#64267=ORIENTED_EDGE('',*,*,#47128,.T.) ;
#64268=ORIENTED_EDGE('',*,*,#47133,.F.) ;
#64269=ORIENTED_EDGE('',*,*,#47129,.T.) ;
#64270=ORIENTED_EDGE('',*,*,#47131,.T.) ;
#64271=ORIENTED_EDGE('',*,*,#47130,.T.) ;
#64272=ORIENTED_EDGE('',*,*,#47134,.F.) ;
#64273=ORIENTED_EDGE('',*,*,#44674,.T.) ;
#64274=ORIENTED_EDGE('',*,*,#47132,.T.) ;
#64275=ORIENTED_EDGE('',*,*,#44734,.F.) ;
#64276=ORIENTED_EDGE('',*,*,#47135,.F.) ;
#64277=ORIENTED_EDGE('',*,*,#44557,.F.) ;
#64278=ORIENTED_EDGE('',*,*,#47133,.T.) ;
#64279=ORIENTED_EDGE('',*,*,#47134,.T.) ;
#64280=ORIENTED_EDGE('',*,*,#44558,.F.) ;
#64281=ORIENTED_EDGE('',*,*,#47136,.F.) ;
#64282=ORIENTED_EDGE('',*,*,#44675,.F.) ;
#64283=ORIENTED_EDGE('',*,*,#47135,.T.) ;
#64284=ORIENTED_EDGE('',*,*,#44601,.F.) ;
#64285=ORIENTED_EDGE('',*,*,#47136,.T.) ;
#64286=ORIENTED_EDGE('',*,*,#47137,.F.) ;
#64287=ORIENTED_EDGE('',*,*,#46343,.F.) ;
#64288=ORIENTED_EDGE('',*,*,#47138,.F.) ;
#64289=ORIENTED_EDGE('',*,*,#46390,.F.) ;
#64290=ORIENTED_EDGE('',*,*,#47138,.T.) ;
#64291=ORIENTED_EDGE('',*,*,#46340,.F.) ;
#64292=ORIENTED_EDGE('',*,*,#47139,.F.) ;
#64293=ORIENTED_EDGE('',*,*,#46391,.F.) ;
#64294=ORIENTED_EDGE('',*,*,#46346,.F.) ;
#64295=ORIENTED_EDGE('',*,*,#47137,.T.) ;
#64296=ORIENTED_EDGE('',*,*,#47140,.F.) ;
#64297=ORIENTED_EDGE('',*,*,#47139,.T.) ;
#64298=ORIENTED_EDGE('',*,*,#46337,.F.) ;
#64299=ORIENTED_EDGE('',*,*,#47141,.F.) ;
#64300=ORIENTED_EDGE('',*,*,#46392,.F.) ;
#64301=ORIENTED_EDGE('',*,*,#47140,.T.) ;
#64302=ORIENTED_EDGE('',*,*,#46389,.F.) ;
#64303=ORIENTED_EDGE('',*,*,#47142,.F.) ;
#64304=ORIENTED_EDGE('',*,*,#46349,.F.) ;
#64305=ORIENTED_EDGE('',*,*,#47141,.T.) ;
#64306=ORIENTED_EDGE('',*,*,#46334,.F.) ;
#64307=ORIENTED_EDGE('',*,*,#47143,.F.) ;
#64308=ORIENTED_EDGE('',*,*,#46393,.F.) ;
#64309=ORIENTED_EDGE('',*,*,#46352,.F.) ;
#64310=ORIENTED_EDGE('',*,*,#47142,.T.) ;
#64311=ORIENTED_EDGE('',*,*,#47144,.F.) ;
#64312=ORIENTED_EDGE('',*,*,#47143,.T.) ;
#64313=ORIENTED_EDGE('',*,*,#46331,.F.) ;
#64314=ORIENTED_EDGE('',*,*,#47145,.F.) ;
#64315=ORIENTED_EDGE('',*,*,#46394,.F.) ;
#64316=ORIENTED_EDGE('',*,*,#47144,.T.) ;
#64317=ORIENTED_EDGE('',*,*,#46388,.F.) ;
#64318=ORIENTED_EDGE('',*,*,#47146,.F.) ;
#64319=ORIENTED_EDGE('',*,*,#46355,.F.) ;
#64320=ORIENTED_EDGE('',*,*,#47145,.T.) ;
#64321=ORIENTED_EDGE('',*,*,#46328,.F.) ;
#64322=ORIENTED_EDGE('',*,*,#47147,.F.) ;
#64323=ORIENTED_EDGE('',*,*,#46358,.F.) ;
#64324=ORIENTED_EDGE('',*,*,#47146,.T.) ;
#64325=ORIENTED_EDGE('',*,*,#47148,.F.) ;
#64326=ORIENTED_EDGE('',*,*,#47147,.T.) ;
#64327=ORIENTED_EDGE('',*,*,#46325,.F.) ;
#64328=ORIENTED_EDGE('',*,*,#47149,.F.) ;
#64329=ORIENTED_EDGE('',*,*,#46395,.F.) ;
#64330=ORIENTED_EDGE('',*,*,#47148,.T.) ;
#64331=ORIENTED_EDGE('',*,*,#46387,.F.) ;
#64332=ORIENTED_EDGE('',*,*,#47150,.F.) ;
#64333=ORIENTED_EDGE('',*,*,#46361,.F.) ;
#64334=ORIENTED_EDGE('',*,*,#47149,.T.) ;
#64335=ORIENTED_EDGE('',*,*,#44351,.F.) ;
#64336=ORIENTED_EDGE('',*,*,#47151,.F.) ;
#64337=ORIENTED_EDGE('',*,*,#46364,.F.) ;
#64338=ORIENTED_EDGE('',*,*,#47150,.T.) ;
#64339=ORIENTED_EDGE('',*,*,#47152,.F.) ;
#64340=ORIENTED_EDGE('',*,*,#47151,.T.) ;
#64341=ORIENTED_EDGE('',*,*,#46323,.F.) ;
#64342=ORIENTED_EDGE('',*,*,#44258,.F.) ;
#64343=ORIENTED_EDGE('',*,*,#46396,.F.) ;
#64344=ORIENTED_EDGE('',*,*,#47152,.T.) ;
#64345=ORIENTED_EDGE('',*,*,#46386,.F.) ;
#64346=ORIENTED_EDGE('',*,*,#47153,.F.) ;
#64347=ORIENTED_EDGE('',*,*,#46367,.F.) ;
#64348=ORIENTED_EDGE('',*,*,#46370,.F.) ;
#64349=ORIENTED_EDGE('',*,*,#47153,.T.) ;
#64350=ORIENTED_EDGE('',*,*,#47154,.F.) ;
#64351=ORIENTED_EDGE('',*,*,#44257,.T.) ;
#64352=ORIENTED_EDGE('',*,*,#46318,.F.) ;
#64353=ORIENTED_EDGE('',*,*,#47155,.F.) ;
#64354=ORIENTED_EDGE('',*,*,#46397,.F.) ;
#64355=ORIENTED_EDGE('',*,*,#47154,.T.) ;
#64356=ORIENTED_EDGE('',*,*,#46385,.F.) ;
#64357=ORIENTED_EDGE('',*,*,#47156,.F.) ;
#64358=ORIENTED_EDGE('',*,*,#46373,.F.) ;
#64359=ORIENTED_EDGE('',*,*,#47155,.T.) ;
#64360=ORIENTED_EDGE('',*,*,#46315,.F.) ;
#64361=ORIENTED_EDGE('',*,*,#47157,.F.) ;
#64362=ORIENTED_EDGE('',*,*,#46376,.F.) ;
#64363=ORIENTED_EDGE('',*,*,#47156,.T.) ;
#64364=ORIENTED_EDGE('',*,*,#47158,.F.) ;
#64365=ORIENTED_EDGE('',*,*,#47157,.T.) ;
#64366=ORIENTED_EDGE('',*,*,#46312,.F.) ;
#64367=ORIENTED_EDGE('',*,*,#47159,.F.) ;
#64368=ORIENTED_EDGE('',*,*,#46398,.F.) ;
#64369=ORIENTED_EDGE('',*,*,#47158,.T.) ;
#64370=ORIENTED_EDGE('',*,*,#46384,.F.) ;
#64371=ORIENTED_EDGE('',*,*,#47160,.F.) ;
#64372=ORIENTED_EDGE('',*,*,#46379,.F.) ;
#64373=ORIENTED_EDGE('',*,*,#47159,.T.) ;
#64374=ORIENTED_EDGE('',*,*,#46309,.F.) ;
#64375=ORIENTED_EDGE('',*,*,#47161,.F.) ;
#64376=ORIENTED_EDGE('',*,*,#46381,.F.) ;
#64377=ORIENTED_EDGE('',*,*,#47160,.T.) ;
#64378=ORIENTED_EDGE('',*,*,#46383,.F.) ;
#64379=ORIENTED_EDGE('',*,*,#47162,.F.) ;
#64380=ORIENTED_EDGE('',*,*,#46303,.F.) ;
#64381=ORIENTED_EDGE('',*,*,#47161,.T.) ;
#64382=ORIENTED_EDGE('',*,*,#46306,.F.) ;
#64383=ORIENTED_EDGE('',*,*,#47162,.T.) ;
#64384=ORIENTED_EDGE('',*,*,#46382,.F.) ;
#64385=ORIENTED_EDGE('',*,*,#47163,.F.) ;
#64386=ORIENTED_EDGE('',*,*,#45618,.F.) ;
#64387=ORIENTED_EDGE('',*,*,#47164,.F.) ;
#64388=ORIENTED_EDGE('',*,*,#45518,.F.) ;
#64389=ORIENTED_EDGE('',*,*,#47165,.F.) ;
#64390=ORIENTED_EDGE('',*,*,#45619,.F.) ;
#64391=ORIENTED_EDGE('',*,*,#47166,.F.) ;
#64392=ORIENTED_EDGE('',*,*,#45613,.F.) ;
#64393=ORIENTED_EDGE('',*,*,#47167,.F.) ;
#64394=ORIENTED_EDGE('',*,*,#47165,.T.) ;
#64395=ORIENTED_EDGE('',*,*,#47168,.F.) ;
#64396=ORIENTED_EDGE('',*,*,#47169,.F.) ;
#64397=ORIENTED_EDGE('',*,*,#47164,.T.) ;
#64398=ORIENTED_EDGE('',*,*,#47170,.F.) ;
#64399=ORIENTED_EDGE('',*,*,#47163,.T.) ;
#64400=ORIENTED_EDGE('',*,*,#45517,.T.) ;
#64401=ORIENTED_EDGE('',*,*,#47171,.F.) ;
#64402=ORIENTED_EDGE('',*,*,#47166,.T.) ;
#64403=ORIENTED_EDGE('',*,*,#47168,.T.) ;
#64404=ORIENTED_EDGE('',*,*,#45616,.F.) ;
#64405=ORIENTED_EDGE('',*,*,#47172,.F.) ;
#64406=ORIENTED_EDGE('',*,*,#44242,.T.) ;
#64407=ORIENTED_EDGE('',*,*,#47173,.T.) ;
#64408=ORIENTED_EDGE('',*,*,#47174,.F.) ;
#64409=ORIENTED_EDGE('',*,*,#47167,.T.) ;
#64410=ORIENTED_EDGE('',*,*,#47175,.F.) ;
#64411=ORIENTED_EDGE('',*,*,#47176,.T.) ;
#64412=ORIENTED_EDGE('',*,*,#47177,.F.) ;
#64413=ORIENTED_EDGE('',*,*,#44452,.F.) ;
#64414=ORIENTED_EDGE('',*,*,#47178,.F.) ;
#64415=ORIENTED_EDGE('',*,*,#45620,.F.) ;
#64416=ORIENTED_EDGE('',*,*,#47170,.T.) ;
#64417=ORIENTED_EDGE('',*,*,#45617,.F.) ;
#64418=ORIENTED_EDGE('',*,*,#47179,.F.) ;
#64419=ORIENTED_EDGE('',*,*,#45623,.F.) ;
#64420=ORIENTED_EDGE('',*,*,#47169,.T.) ;
#64421=ORIENTED_EDGE('',*,*,#45622,.F.) ;
#64422=ORIENTED_EDGE('',*,*,#47180,.F.) ;
#64423=ORIENTED_EDGE('',*,*,#45509,.F.) ;
#64424=ORIENTED_EDGE('',*,*,#47171,.T.) ;
#64425=ORIENTED_EDGE('',*,*,#45516,.F.) ;
#64426=ORIENTED_EDGE('',*,*,#47181,.F.) ;
#64427=ORIENTED_EDGE('',*,*,#45614,.F.) ;
#64428=ORIENTED_EDGE('',*,*,#47182,.F.) ;
#64429=ORIENTED_EDGE('',*,*,#45615,.F.) ;
#64430=ORIENTED_EDGE('',*,*,#47183,.F.) ;
#64431=ORIENTED_EDGE('',*,*,#45610,.F.) ;
#64432=ORIENTED_EDGE('',*,*,#47172,.T.) ;
#64433=ORIENTED_EDGE('',*,*,#47182,.T.) ;
#64434=ORIENTED_EDGE('',*,*,#44243,.F.) ;
#64435=ORIENTED_EDGE('',*,*,#47178,.T.) ;
#64436=ORIENTED_EDGE('',*,*,#44462,.T.) ;
#64437=ORIENTED_EDGE('',*,*,#47184,.F.) ;
#64438=ORIENTED_EDGE('',*,*,#47179,.T.) ;
#64439=ORIENTED_EDGE('',*,*,#47185,.F.) ;
#64440=ORIENTED_EDGE('',*,*,#47180,.T.) ;
#64441=ORIENTED_EDGE('',*,*,#47186,.F.) ;
#64442=ORIENTED_EDGE('',*,*,#44551,.T.) ;
#64443=ORIENTED_EDGE('',*,*,#47181,.T.) ;
#64444=ORIENTED_EDGE('',*,*,#45515,.T.) ;
#64445=ORIENTED_EDGE('',*,*,#47187,.F.) ;
#64446=ORIENTED_EDGE('',*,*,#47183,.T.) ;
#64447=ORIENTED_EDGE('',*,*,#47184,.T.) ;
#64448=ORIENTED_EDGE('',*,*,#44461,.F.) ;
#64449=ORIENTED_EDGE('',*,*,#47188,.F.) ;
#64450=ORIENTED_EDGE('',*,*,#45624,.F.) ;
#64451=ORIENTED_EDGE('',*,*,#47186,.T.) ;
#64452=ORIENTED_EDGE('',*,*,#45621,.F.) ;
#64453=ORIENTED_EDGE('',*,*,#47189,.F.) ;
#64454=ORIENTED_EDGE('',*,*,#44552,.F.) ;
#64455=ORIENTED_EDGE('',*,*,#45510,.F.) ;
#64456=ORIENTED_EDGE('',*,*,#47185,.T.) ;
#64457=ORIENTED_EDGE('',*,*,#47190,.F.) ;
#64458=ORIENTED_EDGE('',*,*,#47191,.F.) ;
#64459=ORIENTED_EDGE('',*,*,#47187,.T.) ;
#64460=ORIENTED_EDGE('',*,*,#45514,.F.) ;
#64461=ORIENTED_EDGE('',*,*,#47192,.F.) ;
#64462=ORIENTED_EDGE('',*,*,#45611,.F.) ;
#64463=ORIENTED_EDGE('',*,*,#47193,.F.) ;
#64464=ORIENTED_EDGE('',*,*,#45612,.F.) ;
#64465=ORIENTED_EDGE('',*,*,#47194,.F.) ;
#64466=ORIENTED_EDGE('',*,*,#45606,.F.) ;
#64467=ORIENTED_EDGE('',*,*,#44245,.T.) ;
#64468=ORIENTED_EDGE('',*,*,#47193,.T.) ;
#64469=ORIENTED_EDGE('',*,*,#47195,.F.) ;
#64470=ORIENTED_EDGE('',*,*,#44456,.T.) ;
#64471=ORIENTED_EDGE('',*,*,#47189,.T.) ;
#64472=ORIENTED_EDGE('',*,*,#47188,.T.) ;
#64473=ORIENTED_EDGE('',*,*,#47196,.F.) ;
#64474=ORIENTED_EDGE('',*,*,#47197,.F.) ;
#64475=ORIENTED_EDGE('',*,*,#44599,.F.) ;
#64476=ORIENTED_EDGE('',*,*,#47198,.F.) ;
#64477=ORIENTED_EDGE('',*,*,#47199,.F.) ;
#64478=ORIENTED_EDGE('',*,*,#47190,.T.) ;
#64479=ORIENTED_EDGE('',*,*,#44555,.F.) ;
#64480=ORIENTED_EDGE('',*,*,#47198,.T.) ;
#64481=ORIENTED_EDGE('',*,*,#44733,.F.) ;
#64482=ORIENTED_EDGE('',*,*,#47191,.T.) ;
#64483=ORIENTED_EDGE('',*,*,#47200,.F.) ;
#64484=ORIENTED_EDGE('',*,*,#47201,.F.) ;
#64485=ORIENTED_EDGE('',*,*,#47194,.T.) ;
#64486=ORIENTED_EDGE('',*,*,#47192,.T.) ;
#64487=ORIENTED_EDGE('',*,*,#47202,.F.) ;
#64488=ORIENTED_EDGE('',*,*,#47195,.T.) ;
#64489=ORIENTED_EDGE('',*,*,#45609,.F.) ;
#64490=ORIENTED_EDGE('',*,*,#47203,.F.) ;
#64491=ORIENTED_EDGE('',*,*,#44457,.F.) ;
#64492=ORIENTED_EDGE('',*,*,#47196,.T.) ;
#64493=ORIENTED_EDGE('',*,*,#44460,.F.) ;
#64494=ORIENTED_EDGE('',*,*,#47204,.F.) ;
#64495=ORIENTED_EDGE('',*,*,#44553,.F.) ;
#64496=ORIENTED_EDGE('',*,*,#47197,.T.) ;
#64497=ORIENTED_EDGE('',*,*,#44554,.F.) ;
#64498=ORIENTED_EDGE('',*,*,#47205,.F.) ;
#64499=ORIENTED_EDGE('',*,*,#44676,.F.) ;
#64500=ORIENTED_EDGE('',*,*,#47199,.T.) ;
#64501=ORIENTED_EDGE('',*,*,#44732,.T.) ;
#64502=ORIENTED_EDGE('',*,*,#47206,.F.) ;
#64503=ORIENTED_EDGE('',*,*,#47200,.T.) ;
#64504=ORIENTED_EDGE('',*,*,#45511,.F.) ;
#64505=ORIENTED_EDGE('',*,*,#47201,.T.) ;
#64506=ORIENTED_EDGE('',*,*,#47207,.F.) ;
#64507=ORIENTED_EDGE('',*,*,#47208,.F.) ;
#64508=ORIENTED_EDGE('',*,*,#47202,.T.) ;
#64509=ORIENTED_EDGE('',*,*,#45513,.F.) ;
#64510=ORIENTED_EDGE('',*,*,#47209,.F.) ;
#64511=ORIENTED_EDGE('',*,*,#45607,.F.) ;
#64512=ORIENTED_EDGE('',*,*,#47210,.F.) ;
#64513=ORIENTED_EDGE('',*,*,#45608,.F.) ;
#64514=ORIENTED_EDGE('',*,*,#47211,.F.) ;
#64515=ORIENTED_EDGE('',*,*,#44550,.F.) ;
#64516=ORIENTED_EDGE('',*,*,#47203,.T.) ;
#64517=ORIENTED_EDGE('',*,*,#47210,.T.) ;
#64518=ORIENTED_EDGE('',*,*,#47212,.F.) ;
#64519=ORIENTED_EDGE('',*,*,#47205,.T.) ;
#64520=ORIENTED_EDGE('',*,*,#47204,.T.) ;
#64521=ORIENTED_EDGE('',*,*,#47213,.F.) ;
#64522=ORIENTED_EDGE('',*,*,#44677,.T.) ;
#64523=ORIENTED_EDGE('',*,*,#47214,.F.) ;
#64524=ORIENTED_EDGE('',*,*,#47207,.T.) ;
#64525=ORIENTED_EDGE('',*,*,#47206,.T.) ;
#64526=ORIENTED_EDGE('',*,*,#44731,.F.) ;
#64527=ORIENTED_EDGE('',*,*,#47208,.T.) ;
#64528=ORIENTED_EDGE('',*,*,#47215,.F.) ;
#64529=ORIENTED_EDGE('',*,*,#47216,.F.) ;
#64530=ORIENTED_EDGE('',*,*,#47211,.T.) ;
#64531=ORIENTED_EDGE('',*,*,#47209,.T.) ;
#64532=ORIENTED_EDGE('',*,*,#47217,.F.) ;
#64533=ORIENTED_EDGE('',*,*,#44546,.T.) ;
#64534=ORIENTED_EDGE('',*,*,#47212,.T.) ;
#64535=ORIENTED_EDGE('',*,*,#44549,.F.) ;
#64536=ORIENTED_EDGE('',*,*,#47218,.F.) ;
#64537=ORIENTED_EDGE('',*,*,#44458,.F.) ;
#64538=ORIENTED_EDGE('',*,*,#47213,.T.) ;
#64539=ORIENTED_EDGE('',*,*,#44459,.F.) ;
#64540=ORIENTED_EDGE('',*,*,#47219,.F.) ;
#64541=ORIENTED_EDGE('',*,*,#44678,.F.) ;
#64542=ORIENTED_EDGE('',*,*,#47214,.T.) ;
#64543=ORIENTED_EDGE('',*,*,#44730,.T.) ;
#64544=ORIENTED_EDGE('',*,*,#47220,.F.) ;
#64545=ORIENTED_EDGE('',*,*,#47215,.T.) ;
#64546=ORIENTED_EDGE('',*,*,#45512,.F.) ;
#64547=ORIENTED_EDGE('',*,*,#47216,.T.) ;
#64548=ORIENTED_EDGE('',*,*,#47221,.F.) ;
#64549=ORIENTED_EDGE('',*,*,#47217,.T.) ;
#64550=ORIENTED_EDGE('',*,*,#47219,.T.) ;
#64551=ORIENTED_EDGE('',*,*,#47218,.T.) ;
#64552=ORIENTED_EDGE('',*,*,#47222,.F.) ;
#64553=ORIENTED_EDGE('',*,*,#44679,.T.) ;
#64554=ORIENTED_EDGE('',*,*,#47220,.T.) ;
#64555=ORIENTED_EDGE('',*,*,#44729,.F.) ;
#64556=ORIENTED_EDGE('',*,*,#47223,.F.) ;
#64557=ORIENTED_EDGE('',*,*,#44547,.F.) ;
#64558=ORIENTED_EDGE('',*,*,#47221,.T.) ;
#64559=ORIENTED_EDGE('',*,*,#47222,.T.) ;
#64560=ORIENTED_EDGE('',*,*,#44548,.F.) ;
#64561=ORIENTED_EDGE('',*,*,#47224,.F.) ;
#64562=ORIENTED_EDGE('',*,*,#44680,.F.) ;
#64563=ORIENTED_EDGE('',*,*,#47223,.T.) ;
#64564=ORIENTED_EDGE('',*,*,#44605,.F.) ;
#64565=ORIENTED_EDGE('',*,*,#47224,.T.) ;
#64566=ORIENTED_EDGE('',*,*,#47225,.F.) ;
#64567=ORIENTED_EDGE('',*,*,#46246,.F.) ;
#64568=ORIENTED_EDGE('',*,*,#47226,.F.) ;
#64569=ORIENTED_EDGE('',*,*,#46293,.F.) ;
#64570=ORIENTED_EDGE('',*,*,#47226,.T.) ;
#64571=ORIENTED_EDGE('',*,*,#46243,.F.) ;
#64572=ORIENTED_EDGE('',*,*,#47227,.F.) ;
#64573=ORIENTED_EDGE('',*,*,#46294,.F.) ;
#64574=ORIENTED_EDGE('',*,*,#46249,.F.) ;
#64575=ORIENTED_EDGE('',*,*,#47225,.T.) ;
#64576=ORIENTED_EDGE('',*,*,#47228,.F.) ;
#64577=ORIENTED_EDGE('',*,*,#47227,.T.) ;
#64578=ORIENTED_EDGE('',*,*,#46240,.F.) ;
#64579=ORIENTED_EDGE('',*,*,#47229,.F.) ;
#64580=ORIENTED_EDGE('',*,*,#46295,.F.) ;
#64581=ORIENTED_EDGE('',*,*,#47228,.T.) ;
#64582=ORIENTED_EDGE('',*,*,#46292,.F.) ;
#64583=ORIENTED_EDGE('',*,*,#47230,.F.) ;
#64584=ORIENTED_EDGE('',*,*,#46252,.F.) ;
#64585=ORIENTED_EDGE('',*,*,#47229,.T.) ;
#64586=ORIENTED_EDGE('',*,*,#46237,.F.) ;
#64587=ORIENTED_EDGE('',*,*,#47231,.F.) ;
#64588=ORIENTED_EDGE('',*,*,#46296,.F.) ;
#64589=ORIENTED_EDGE('',*,*,#46255,.F.) ;
#64590=ORIENTED_EDGE('',*,*,#47230,.T.) ;
#64591=ORIENTED_EDGE('',*,*,#47232,.F.) ;
#64592=ORIENTED_EDGE('',*,*,#47231,.T.) ;
#64593=ORIENTED_EDGE('',*,*,#46234,.F.) ;
#64594=ORIENTED_EDGE('',*,*,#47233,.F.) ;
#64595=ORIENTED_EDGE('',*,*,#46297,.F.) ;
#64596=ORIENTED_EDGE('',*,*,#47232,.T.) ;
#64597=ORIENTED_EDGE('',*,*,#46291,.F.) ;
#64598=ORIENTED_EDGE('',*,*,#47234,.F.) ;
#64599=ORIENTED_EDGE('',*,*,#46258,.F.) ;
#64600=ORIENTED_EDGE('',*,*,#47233,.T.) ;
#64601=ORIENTED_EDGE('',*,*,#46231,.F.) ;
#64602=ORIENTED_EDGE('',*,*,#47235,.F.) ;
#64603=ORIENTED_EDGE('',*,*,#46261,.F.) ;
#64604=ORIENTED_EDGE('',*,*,#47234,.T.) ;
#64605=ORIENTED_EDGE('',*,*,#47236,.F.) ;
#64606=ORIENTED_EDGE('',*,*,#47235,.T.) ;
#64607=ORIENTED_EDGE('',*,*,#46228,.F.) ;
#64608=ORIENTED_EDGE('',*,*,#47237,.F.) ;
#64609=ORIENTED_EDGE('',*,*,#46298,.F.) ;
#64610=ORIENTED_EDGE('',*,*,#47236,.T.) ;
#64611=ORIENTED_EDGE('',*,*,#46290,.F.) ;
#64612=ORIENTED_EDGE('',*,*,#47238,.F.) ;
#64613=ORIENTED_EDGE('',*,*,#46264,.F.) ;
#64614=ORIENTED_EDGE('',*,*,#47237,.T.) ;
#64615=ORIENTED_EDGE('',*,*,#44354,.F.) ;
#64616=ORIENTED_EDGE('',*,*,#47239,.F.) ;
#64617=ORIENTED_EDGE('',*,*,#46267,.F.) ;
#64618=ORIENTED_EDGE('',*,*,#47238,.T.) ;
#64619=ORIENTED_EDGE('',*,*,#47240,.F.) ;
#64620=ORIENTED_EDGE('',*,*,#47239,.T.) ;
#64621=ORIENTED_EDGE('',*,*,#46226,.F.) ;
#64622=ORIENTED_EDGE('',*,*,#44241,.F.) ;
#64623=ORIENTED_EDGE('',*,*,#46299,.F.) ;
#64624=ORIENTED_EDGE('',*,*,#47240,.T.) ;
#64625=ORIENTED_EDGE('',*,*,#46289,.F.) ;
#64626=ORIENTED_EDGE('',*,*,#47241,.F.) ;
#64627=ORIENTED_EDGE('',*,*,#46270,.F.) ;
#64628=ORIENTED_EDGE('',*,*,#46273,.F.) ;
#64629=ORIENTED_EDGE('',*,*,#47241,.T.) ;
#64630=ORIENTED_EDGE('',*,*,#47242,.F.) ;
#64631=ORIENTED_EDGE('',*,*,#44240,.T.) ;
#64632=ORIENTED_EDGE('',*,*,#46221,.F.) ;
#64633=ORIENTED_EDGE('',*,*,#47243,.F.) ;
#64634=ORIENTED_EDGE('',*,*,#46300,.F.) ;
#64635=ORIENTED_EDGE('',*,*,#47242,.T.) ;
#64636=ORIENTED_EDGE('',*,*,#46288,.F.) ;
#64637=ORIENTED_EDGE('',*,*,#47244,.F.) ;
#64638=ORIENTED_EDGE('',*,*,#46276,.F.) ;
#64639=ORIENTED_EDGE('',*,*,#47243,.T.) ;
#64640=ORIENTED_EDGE('',*,*,#46218,.F.) ;
#64641=ORIENTED_EDGE('',*,*,#47245,.F.) ;
#64642=ORIENTED_EDGE('',*,*,#46279,.F.) ;
#64643=ORIENTED_EDGE('',*,*,#47244,.T.) ;
#64644=ORIENTED_EDGE('',*,*,#47246,.F.) ;
#64645=ORIENTED_EDGE('',*,*,#47245,.T.) ;
#64646=ORIENTED_EDGE('',*,*,#46215,.F.) ;
#64647=ORIENTED_EDGE('',*,*,#47247,.F.) ;
#64648=ORIENTED_EDGE('',*,*,#46301,.F.) ;
#64649=ORIENTED_EDGE('',*,*,#47246,.T.) ;
#64650=ORIENTED_EDGE('',*,*,#46287,.F.) ;
#64651=ORIENTED_EDGE('',*,*,#47248,.F.) ;
#64652=ORIENTED_EDGE('',*,*,#46282,.F.) ;
#64653=ORIENTED_EDGE('',*,*,#47247,.T.) ;
#64654=ORIENTED_EDGE('',*,*,#46212,.F.) ;
#64655=ORIENTED_EDGE('',*,*,#47249,.F.) ;
#64656=ORIENTED_EDGE('',*,*,#46284,.F.) ;
#64657=ORIENTED_EDGE('',*,*,#47248,.T.) ;
#64658=ORIENTED_EDGE('',*,*,#46286,.F.) ;
#64659=ORIENTED_EDGE('',*,*,#47250,.F.) ;
#64660=ORIENTED_EDGE('',*,*,#46206,.F.) ;
#64661=ORIENTED_EDGE('',*,*,#47249,.T.) ;
#64662=ORIENTED_EDGE('',*,*,#46209,.F.) ;
#64663=ORIENTED_EDGE('',*,*,#47250,.T.) ;
#64664=ORIENTED_EDGE('',*,*,#46285,.F.) ;
#64665=ORIENTED_EDGE('',*,*,#47251,.F.) ;
#64666=ORIENTED_EDGE('',*,*,#45637,.F.) ;
#64667=ORIENTED_EDGE('',*,*,#47252,.F.) ;
#64668=ORIENTED_EDGE('',*,*,#45508,.F.) ;
#64669=ORIENTED_EDGE('',*,*,#47253,.F.) ;
#64670=ORIENTED_EDGE('',*,*,#45638,.F.) ;
#64671=ORIENTED_EDGE('',*,*,#47254,.F.) ;
#64672=ORIENTED_EDGE('',*,*,#45632,.F.) ;
#64673=ORIENTED_EDGE('',*,*,#47255,.F.) ;
#64674=ORIENTED_EDGE('',*,*,#47253,.T.) ;
#64675=ORIENTED_EDGE('',*,*,#47256,.F.) ;
#64676=ORIENTED_EDGE('',*,*,#47257,.F.) ;
#64677=ORIENTED_EDGE('',*,*,#47252,.T.) ;
#64678=ORIENTED_EDGE('',*,*,#47258,.F.) ;
#64679=ORIENTED_EDGE('',*,*,#47251,.T.) ;
#64680=ORIENTED_EDGE('',*,*,#45507,.T.) ;
#64681=ORIENTED_EDGE('',*,*,#47259,.F.) ;
#64682=ORIENTED_EDGE('',*,*,#47254,.T.) ;
#64683=ORIENTED_EDGE('',*,*,#47256,.T.) ;
#64684=ORIENTED_EDGE('',*,*,#45635,.F.) ;
#64685=ORIENTED_EDGE('',*,*,#47260,.F.) ;
#64686=ORIENTED_EDGE('',*,*,#44225,.T.) ;
#64687=ORIENTED_EDGE('',*,*,#47261,.T.) ;
#64688=ORIENTED_EDGE('',*,*,#47262,.F.) ;
#64689=ORIENTED_EDGE('',*,*,#47255,.T.) ;
#64690=ORIENTED_EDGE('',*,*,#47263,.F.) ;
#64691=ORIENTED_EDGE('',*,*,#47264,.T.) ;
#64692=ORIENTED_EDGE('',*,*,#47265,.F.) ;
#64693=ORIENTED_EDGE('',*,*,#44441,.F.) ;
#64694=ORIENTED_EDGE('',*,*,#47266,.F.) ;
#64695=ORIENTED_EDGE('',*,*,#45639,.F.) ;
#64696=ORIENTED_EDGE('',*,*,#47258,.T.) ;
#64697=ORIENTED_EDGE('',*,*,#45636,.F.) ;
#64698=ORIENTED_EDGE('',*,*,#47267,.F.) ;
#64699=ORIENTED_EDGE('',*,*,#45642,.F.) ;
#64700=ORIENTED_EDGE('',*,*,#47257,.T.) ;
#64701=ORIENTED_EDGE('',*,*,#45641,.F.) ;
#64702=ORIENTED_EDGE('',*,*,#47268,.F.) ;
#64703=ORIENTED_EDGE('',*,*,#45499,.F.) ;
#64704=ORIENTED_EDGE('',*,*,#47259,.T.) ;
#64705=ORIENTED_EDGE('',*,*,#45506,.F.) ;
#64706=ORIENTED_EDGE('',*,*,#47269,.F.) ;
#64707=ORIENTED_EDGE('',*,*,#45633,.F.) ;
#64708=ORIENTED_EDGE('',*,*,#47270,.F.) ;
#64709=ORIENTED_EDGE('',*,*,#45634,.F.) ;
#64710=ORIENTED_EDGE('',*,*,#47271,.F.) ;
#64711=ORIENTED_EDGE('',*,*,#45629,.F.) ;
#64712=ORIENTED_EDGE('',*,*,#47260,.T.) ;
#64713=ORIENTED_EDGE('',*,*,#47270,.T.) ;
#64714=ORIENTED_EDGE('',*,*,#44226,.F.) ;
#64715=ORIENTED_EDGE('',*,*,#47266,.T.) ;
#64716=ORIENTED_EDGE('',*,*,#44451,.T.) ;
#64717=ORIENTED_EDGE('',*,*,#47272,.F.) ;
#64718=ORIENTED_EDGE('',*,*,#47267,.T.) ;
#64719=ORIENTED_EDGE('',*,*,#47273,.F.) ;
#64720=ORIENTED_EDGE('',*,*,#47268,.T.) ;
#64721=ORIENTED_EDGE('',*,*,#47274,.F.) ;
#64722=ORIENTED_EDGE('',*,*,#44541,.T.) ;
#64723=ORIENTED_EDGE('',*,*,#47269,.T.) ;
#64724=ORIENTED_EDGE('',*,*,#45505,.T.) ;
#64725=ORIENTED_EDGE('',*,*,#47275,.F.) ;
#64726=ORIENTED_EDGE('',*,*,#47271,.T.) ;
#64727=ORIENTED_EDGE('',*,*,#47272,.T.) ;
#64728=ORIENTED_EDGE('',*,*,#44450,.F.) ;
#64729=ORIENTED_EDGE('',*,*,#47276,.F.) ;
#64730=ORIENTED_EDGE('',*,*,#45643,.F.) ;
#64731=ORIENTED_EDGE('',*,*,#47274,.T.) ;
#64732=ORIENTED_EDGE('',*,*,#45640,.F.) ;
#64733=ORIENTED_EDGE('',*,*,#47277,.F.) ;
#64734=ORIENTED_EDGE('',*,*,#44542,.F.) ;
#64735=ORIENTED_EDGE('',*,*,#45500,.F.) ;
#64736=ORIENTED_EDGE('',*,*,#47273,.T.) ;
#64737=ORIENTED_EDGE('',*,*,#47278,.F.) ;
#64738=ORIENTED_EDGE('',*,*,#47279,.F.) ;
#64739=ORIENTED_EDGE('',*,*,#47275,.T.) ;
#64740=ORIENTED_EDGE('',*,*,#45504,.F.) ;
#64741=ORIENTED_EDGE('',*,*,#47280,.F.) ;
#64742=ORIENTED_EDGE('',*,*,#45630,.F.) ;
#64743=ORIENTED_EDGE('',*,*,#47281,.F.) ;
#64744=ORIENTED_EDGE('',*,*,#45631,.F.) ;
#64745=ORIENTED_EDGE('',*,*,#47282,.F.) ;
#64746=ORIENTED_EDGE('',*,*,#45625,.F.) ;
#64747=ORIENTED_EDGE('',*,*,#44228,.T.) ;
#64748=ORIENTED_EDGE('',*,*,#47281,.T.) ;
#64749=ORIENTED_EDGE('',*,*,#47283,.F.) ;
#64750=ORIENTED_EDGE('',*,*,#44445,.T.) ;
#64751=ORIENTED_EDGE('',*,*,#47277,.T.) ;
#64752=ORIENTED_EDGE('',*,*,#47276,.T.) ;
#64753=ORIENTED_EDGE('',*,*,#47284,.F.) ;
#64754=ORIENTED_EDGE('',*,*,#47285,.F.) ;
#64755=ORIENTED_EDGE('',*,*,#44603,.F.) ;
#64756=ORIENTED_EDGE('',*,*,#47286,.F.) ;
#64757=ORIENTED_EDGE('',*,*,#47287,.F.) ;
#64758=ORIENTED_EDGE('',*,*,#47278,.T.) ;
#64759=ORIENTED_EDGE('',*,*,#44545,.F.) ;
#64760=ORIENTED_EDGE('',*,*,#47286,.T.) ;
#64761=ORIENTED_EDGE('',*,*,#44728,.F.) ;
#64762=ORIENTED_EDGE('',*,*,#47279,.T.) ;
#64763=ORIENTED_EDGE('',*,*,#47288,.F.) ;
#64764=ORIENTED_EDGE('',*,*,#47289,.F.) ;
#64765=ORIENTED_EDGE('',*,*,#47282,.T.) ;
#64766=ORIENTED_EDGE('',*,*,#47280,.T.) ;
#64767=ORIENTED_EDGE('',*,*,#47290,.F.) ;
#64768=ORIENTED_EDGE('',*,*,#47283,.T.) ;
#64769=ORIENTED_EDGE('',*,*,#45628,.F.) ;
#64770=ORIENTED_EDGE('',*,*,#47291,.F.) ;
#64771=ORIENTED_EDGE('',*,*,#44446,.F.) ;
#64772=ORIENTED_EDGE('',*,*,#47284,.T.) ;
#64773=ORIENTED_EDGE('',*,*,#44449,.F.) ;
#64774=ORIENTED_EDGE('',*,*,#47292,.F.) ;
#64775=ORIENTED_EDGE('',*,*,#44543,.F.) ;
#64776=ORIENTED_EDGE('',*,*,#47285,.T.) ;
#64777=ORIENTED_EDGE('',*,*,#44544,.F.) ;
#64778=ORIENTED_EDGE('',*,*,#47293,.F.) ;
#64779=ORIENTED_EDGE('',*,*,#44681,.F.) ;
#64780=ORIENTED_EDGE('',*,*,#47287,.T.) ;
#64781=ORIENTED_EDGE('',*,*,#44727,.T.) ;
#64782=ORIENTED_EDGE('',*,*,#47294,.F.) ;
#64783=ORIENTED_EDGE('',*,*,#47288,.T.) ;
#64784=ORIENTED_EDGE('',*,*,#45501,.F.) ;
#64785=ORIENTED_EDGE('',*,*,#47289,.T.) ;
#64786=ORIENTED_EDGE('',*,*,#47295,.F.) ;
#64787=ORIENTED_EDGE('',*,*,#47296,.F.) ;
#64788=ORIENTED_EDGE('',*,*,#47290,.T.) ;
#64789=ORIENTED_EDGE('',*,*,#45503,.F.) ;
#64790=ORIENTED_EDGE('',*,*,#47297,.F.) ;
#64791=ORIENTED_EDGE('',*,*,#45626,.F.) ;
#64792=ORIENTED_EDGE('',*,*,#47298,.F.) ;
#64793=ORIENTED_EDGE('',*,*,#45627,.F.) ;
#64794=ORIENTED_EDGE('',*,*,#47299,.F.) ;
#64795=ORIENTED_EDGE('',*,*,#44540,.F.) ;
#64796=ORIENTED_EDGE('',*,*,#47291,.T.) ;
#64797=ORIENTED_EDGE('',*,*,#47298,.T.) ;
#64798=ORIENTED_EDGE('',*,*,#47300,.F.) ;
#64799=ORIENTED_EDGE('',*,*,#47293,.T.) ;
#64800=ORIENTED_EDGE('',*,*,#47292,.T.) ;
#64801=ORIENTED_EDGE('',*,*,#47301,.F.) ;
#64802=ORIENTED_EDGE('',*,*,#44682,.T.) ;
#64803=ORIENTED_EDGE('',*,*,#47302,.F.) ;
#64804=ORIENTED_EDGE('',*,*,#47295,.T.) ;
#64805=ORIENTED_EDGE('',*,*,#47294,.T.) ;
#64806=ORIENTED_EDGE('',*,*,#44726,.F.) ;
#64807=ORIENTED_EDGE('',*,*,#47296,.T.) ;
#64808=ORIENTED_EDGE('',*,*,#47303,.F.) ;
#64809=ORIENTED_EDGE('',*,*,#47304,.F.) ;
#64810=ORIENTED_EDGE('',*,*,#47299,.T.) ;
#64811=ORIENTED_EDGE('',*,*,#47297,.T.) ;
#64812=ORIENTED_EDGE('',*,*,#47305,.F.) ;
#64813=ORIENTED_EDGE('',*,*,#44536,.T.) ;
#64814=ORIENTED_EDGE('',*,*,#47300,.T.) ;
#64815=ORIENTED_EDGE('',*,*,#44539,.F.) ;
#64816=ORIENTED_EDGE('',*,*,#47306,.F.) ;
#64817=ORIENTED_EDGE('',*,*,#44447,.F.) ;
#64818=ORIENTED_EDGE('',*,*,#47301,.T.) ;
#64819=ORIENTED_EDGE('',*,*,#44448,.F.) ;
#64820=ORIENTED_EDGE('',*,*,#47307,.F.) ;
#64821=ORIENTED_EDGE('',*,*,#44683,.F.) ;
#64822=ORIENTED_EDGE('',*,*,#47302,.T.) ;
#64823=ORIENTED_EDGE('',*,*,#44725,.T.) ;
#64824=ORIENTED_EDGE('',*,*,#47308,.F.) ;
#64825=ORIENTED_EDGE('',*,*,#47303,.T.) ;
#64826=ORIENTED_EDGE('',*,*,#45502,.F.) ;
#64827=ORIENTED_EDGE('',*,*,#47304,.T.) ;
#64828=ORIENTED_EDGE('',*,*,#47309,.F.) ;
#64829=ORIENTED_EDGE('',*,*,#47305,.T.) ;
#64830=ORIENTED_EDGE('',*,*,#47307,.T.) ;
#64831=ORIENTED_EDGE('',*,*,#47306,.T.) ;
#64832=ORIENTED_EDGE('',*,*,#47310,.F.) ;
#64833=ORIENTED_EDGE('',*,*,#44684,.T.) ;
#64834=ORIENTED_EDGE('',*,*,#47308,.T.) ;
#64835=ORIENTED_EDGE('',*,*,#44724,.F.) ;
#64836=ORIENTED_EDGE('',*,*,#47311,.F.) ;
#64837=ORIENTED_EDGE('',*,*,#44537,.F.) ;
#64838=ORIENTED_EDGE('',*,*,#47309,.T.) ;
#64839=ORIENTED_EDGE('',*,*,#47310,.T.) ;
#64840=ORIENTED_EDGE('',*,*,#44538,.F.) ;
#64841=ORIENTED_EDGE('',*,*,#47312,.F.) ;
#64842=ORIENTED_EDGE('',*,*,#44685,.F.) ;
#64843=ORIENTED_EDGE('',*,*,#47311,.T.) ;
#64844=ORIENTED_EDGE('',*,*,#44609,.F.) ;
#64845=ORIENTED_EDGE('',*,*,#47312,.T.) ;
#64846=ORIENTED_EDGE('',*,*,#47313,.F.) ;
#64847=ORIENTED_EDGE('',*,*,#46149,.F.) ;
#64848=ORIENTED_EDGE('',*,*,#47314,.F.) ;
#64849=ORIENTED_EDGE('',*,*,#46196,.F.) ;
#64850=ORIENTED_EDGE('',*,*,#47314,.T.) ;
#64851=ORIENTED_EDGE('',*,*,#46146,.F.) ;
#64852=ORIENTED_EDGE('',*,*,#47315,.F.) ;
#64853=ORIENTED_EDGE('',*,*,#46197,.F.) ;
#64854=ORIENTED_EDGE('',*,*,#46152,.F.) ;
#64855=ORIENTED_EDGE('',*,*,#47313,.T.) ;
#64856=ORIENTED_EDGE('',*,*,#47316,.F.) ;
#64857=ORIENTED_EDGE('',*,*,#47315,.T.) ;
#64858=ORIENTED_EDGE('',*,*,#46143,.F.) ;
#64859=ORIENTED_EDGE('',*,*,#47317,.F.) ;
#64860=ORIENTED_EDGE('',*,*,#46198,.F.) ;
#64861=ORIENTED_EDGE('',*,*,#47316,.T.) ;
#64862=ORIENTED_EDGE('',*,*,#46195,.F.) ;
#64863=ORIENTED_EDGE('',*,*,#47318,.F.) ;
#64864=ORIENTED_EDGE('',*,*,#46155,.F.) ;
#64865=ORIENTED_EDGE('',*,*,#47317,.T.) ;
#64866=ORIENTED_EDGE('',*,*,#46140,.F.) ;
#64867=ORIENTED_EDGE('',*,*,#47319,.F.) ;
#64868=ORIENTED_EDGE('',*,*,#46199,.F.) ;
#64869=ORIENTED_EDGE('',*,*,#46158,.F.) ;
#64870=ORIENTED_EDGE('',*,*,#47318,.T.) ;
#64871=ORIENTED_EDGE('',*,*,#47320,.F.) ;
#64872=ORIENTED_EDGE('',*,*,#47319,.T.) ;
#64873=ORIENTED_EDGE('',*,*,#46137,.F.) ;
#64874=ORIENTED_EDGE('',*,*,#47321,.F.) ;
#64875=ORIENTED_EDGE('',*,*,#46200,.F.) ;
#64876=ORIENTED_EDGE('',*,*,#47320,.T.) ;
#64877=ORIENTED_EDGE('',*,*,#46194,.F.) ;
#64878=ORIENTED_EDGE('',*,*,#47322,.F.) ;
#64879=ORIENTED_EDGE('',*,*,#46161,.F.) ;
#64880=ORIENTED_EDGE('',*,*,#47321,.T.) ;
#64881=ORIENTED_EDGE('',*,*,#46134,.F.) ;
#64882=ORIENTED_EDGE('',*,*,#47323,.F.) ;
#64883=ORIENTED_EDGE('',*,*,#46164,.F.) ;
#64884=ORIENTED_EDGE('',*,*,#47322,.T.) ;
#64885=ORIENTED_EDGE('',*,*,#47324,.F.) ;
#64886=ORIENTED_EDGE('',*,*,#47323,.T.) ;
#64887=ORIENTED_EDGE('',*,*,#46131,.F.) ;
#64888=ORIENTED_EDGE('',*,*,#47325,.F.) ;
#64889=ORIENTED_EDGE('',*,*,#46201,.F.) ;
#64890=ORIENTED_EDGE('',*,*,#47324,.T.) ;
#64891=ORIENTED_EDGE('',*,*,#46193,.F.) ;
#64892=ORIENTED_EDGE('',*,*,#47326,.F.) ;
#64893=ORIENTED_EDGE('',*,*,#46167,.F.) ;
#64894=ORIENTED_EDGE('',*,*,#47325,.T.) ;
#64895=ORIENTED_EDGE('',*,*,#44357,.F.) ;
#64896=ORIENTED_EDGE('',*,*,#47327,.F.) ;
#64897=ORIENTED_EDGE('',*,*,#46170,.F.) ;
#64898=ORIENTED_EDGE('',*,*,#47326,.T.) ;
#64899=ORIENTED_EDGE('',*,*,#47328,.F.) ;
#64900=ORIENTED_EDGE('',*,*,#47327,.T.) ;
#64901=ORIENTED_EDGE('',*,*,#46129,.F.) ;
#64902=ORIENTED_EDGE('',*,*,#44224,.F.) ;
#64903=ORIENTED_EDGE('',*,*,#46202,.F.) ;
#64904=ORIENTED_EDGE('',*,*,#47328,.T.) ;
#64905=ORIENTED_EDGE('',*,*,#46192,.F.) ;
#64906=ORIENTED_EDGE('',*,*,#47329,.F.) ;
#64907=ORIENTED_EDGE('',*,*,#46173,.F.) ;
#64908=ORIENTED_EDGE('',*,*,#46176,.F.) ;
#64909=ORIENTED_EDGE('',*,*,#47329,.T.) ;
#64910=ORIENTED_EDGE('',*,*,#47330,.F.) ;
#64911=ORIENTED_EDGE('',*,*,#44223,.T.) ;
#64912=ORIENTED_EDGE('',*,*,#46124,.F.) ;
#64913=ORIENTED_EDGE('',*,*,#47331,.F.) ;
#64914=ORIENTED_EDGE('',*,*,#46203,.F.) ;
#64915=ORIENTED_EDGE('',*,*,#47330,.T.) ;
#64916=ORIENTED_EDGE('',*,*,#46191,.F.) ;
#64917=ORIENTED_EDGE('',*,*,#47332,.F.) ;
#64918=ORIENTED_EDGE('',*,*,#46179,.F.) ;
#64919=ORIENTED_EDGE('',*,*,#47331,.T.) ;
#64920=ORIENTED_EDGE('',*,*,#46121,.F.) ;
#64921=ORIENTED_EDGE('',*,*,#47333,.F.) ;
#64922=ORIENTED_EDGE('',*,*,#46182,.F.) ;
#64923=ORIENTED_EDGE('',*,*,#47332,.T.) ;
#64924=ORIENTED_EDGE('',*,*,#47334,.F.) ;
#64925=ORIENTED_EDGE('',*,*,#47333,.T.) ;
#64926=ORIENTED_EDGE('',*,*,#46118,.F.) ;
#64927=ORIENTED_EDGE('',*,*,#47335,.F.) ;
#64928=ORIENTED_EDGE('',*,*,#46204,.F.) ;
#64929=ORIENTED_EDGE('',*,*,#47334,.T.) ;
#64930=ORIENTED_EDGE('',*,*,#46190,.F.) ;
#64931=ORIENTED_EDGE('',*,*,#47336,.F.) ;
#64932=ORIENTED_EDGE('',*,*,#46185,.F.) ;
#64933=ORIENTED_EDGE('',*,*,#47335,.T.) ;
#64934=ORIENTED_EDGE('',*,*,#46115,.F.) ;
#64935=ORIENTED_EDGE('',*,*,#47337,.F.) ;
#64936=ORIENTED_EDGE('',*,*,#46187,.F.) ;
#64937=ORIENTED_EDGE('',*,*,#47336,.T.) ;
#64938=ORIENTED_EDGE('',*,*,#46189,.F.) ;
#64939=ORIENTED_EDGE('',*,*,#47338,.F.) ;
#64940=ORIENTED_EDGE('',*,*,#46109,.F.) ;
#64941=ORIENTED_EDGE('',*,*,#47337,.T.) ;
#64942=ORIENTED_EDGE('',*,*,#46112,.F.) ;
#64943=ORIENTED_EDGE('',*,*,#47338,.T.) ;
#64944=ORIENTED_EDGE('',*,*,#46188,.F.) ;
#64945=ORIENTED_EDGE('',*,*,#47339,.F.) ;
#64946=ORIENTED_EDGE('',*,*,#45656,.F.) ;
#64947=ORIENTED_EDGE('',*,*,#47340,.F.) ;
#64948=ORIENTED_EDGE('',*,*,#45498,.F.) ;
#64949=ORIENTED_EDGE('',*,*,#47341,.F.) ;
#64950=ORIENTED_EDGE('',*,*,#45657,.F.) ;
#64951=ORIENTED_EDGE('',*,*,#47342,.F.) ;
#64952=ORIENTED_EDGE('',*,*,#45651,.F.) ;
#64953=ORIENTED_EDGE('',*,*,#47343,.F.) ;
#64954=ORIENTED_EDGE('',*,*,#47341,.T.) ;
#64955=ORIENTED_EDGE('',*,*,#47344,.F.) ;
#64956=ORIENTED_EDGE('',*,*,#47345,.F.) ;
#64957=ORIENTED_EDGE('',*,*,#47340,.T.) ;
#64958=ORIENTED_EDGE('',*,*,#47346,.F.) ;
#64959=ORIENTED_EDGE('',*,*,#47339,.T.) ;
#64960=ORIENTED_EDGE('',*,*,#45497,.T.) ;
#64961=ORIENTED_EDGE('',*,*,#47347,.F.) ;
#64962=ORIENTED_EDGE('',*,*,#47342,.T.) ;
#64963=ORIENTED_EDGE('',*,*,#47344,.T.) ;
#64964=ORIENTED_EDGE('',*,*,#45654,.F.) ;
#64965=ORIENTED_EDGE('',*,*,#47348,.F.) ;
#64966=ORIENTED_EDGE('',*,*,#44208,.T.) ;
#64967=ORIENTED_EDGE('',*,*,#47349,.T.) ;
#64968=ORIENTED_EDGE('',*,*,#47350,.F.) ;
#64969=ORIENTED_EDGE('',*,*,#47343,.T.) ;
#64970=ORIENTED_EDGE('',*,*,#47351,.F.) ;
#64971=ORIENTED_EDGE('',*,*,#47352,.T.) ;
#64972=ORIENTED_EDGE('',*,*,#47353,.F.) ;
#64973=ORIENTED_EDGE('',*,*,#44430,.F.) ;
#64974=ORIENTED_EDGE('',*,*,#47354,.F.) ;
#64975=ORIENTED_EDGE('',*,*,#45658,.F.) ;
#64976=ORIENTED_EDGE('',*,*,#47346,.T.) ;
#64977=ORIENTED_EDGE('',*,*,#45655,.F.) ;
#64978=ORIENTED_EDGE('',*,*,#47355,.F.) ;
#64979=ORIENTED_EDGE('',*,*,#45661,.F.) ;
#64980=ORIENTED_EDGE('',*,*,#47345,.T.) ;
#64981=ORIENTED_EDGE('',*,*,#45660,.F.) ;
#64982=ORIENTED_EDGE('',*,*,#47356,.F.) ;
#64983=ORIENTED_EDGE('',*,*,#45489,.F.) ;
#64984=ORIENTED_EDGE('',*,*,#47347,.T.) ;
#64985=ORIENTED_EDGE('',*,*,#45496,.F.) ;
#64986=ORIENTED_EDGE('',*,*,#47357,.F.) ;
#64987=ORIENTED_EDGE('',*,*,#45652,.F.) ;
#64988=ORIENTED_EDGE('',*,*,#47358,.F.) ;
#64989=ORIENTED_EDGE('',*,*,#45653,.F.) ;
#64990=ORIENTED_EDGE('',*,*,#47359,.F.) ;
#64991=ORIENTED_EDGE('',*,*,#45648,.F.) ;
#64992=ORIENTED_EDGE('',*,*,#47348,.T.) ;
#64993=ORIENTED_EDGE('',*,*,#47358,.T.) ;
#64994=ORIENTED_EDGE('',*,*,#44209,.F.) ;
#64995=ORIENTED_EDGE('',*,*,#47354,.T.) ;
#64996=ORIENTED_EDGE('',*,*,#44440,.T.) ;
#64997=ORIENTED_EDGE('',*,*,#47360,.F.) ;
#64998=ORIENTED_EDGE('',*,*,#47355,.T.) ;
#64999=ORIENTED_EDGE('',*,*,#47361,.F.) ;
#65000=ORIENTED_EDGE('',*,*,#47356,.T.) ;
#65001=ORIENTED_EDGE('',*,*,#47362,.F.) ;
#65002=ORIENTED_EDGE('',*,*,#44531,.T.) ;
#65003=ORIENTED_EDGE('',*,*,#47357,.T.) ;
#65004=ORIENTED_EDGE('',*,*,#45495,.T.) ;
#65005=ORIENTED_EDGE('',*,*,#47363,.F.) ;
#65006=ORIENTED_EDGE('',*,*,#47359,.T.) ;
#65007=ORIENTED_EDGE('',*,*,#47360,.T.) ;
#65008=ORIENTED_EDGE('',*,*,#44439,.F.) ;
#65009=ORIENTED_EDGE('',*,*,#47364,.F.) ;
#65010=ORIENTED_EDGE('',*,*,#45662,.F.) ;
#65011=ORIENTED_EDGE('',*,*,#47362,.T.) ;
#65012=ORIENTED_EDGE('',*,*,#45659,.F.) ;
#65013=ORIENTED_EDGE('',*,*,#47365,.F.) ;
#65014=ORIENTED_EDGE('',*,*,#44532,.F.) ;
#65015=ORIENTED_EDGE('',*,*,#45490,.F.) ;
#65016=ORIENTED_EDGE('',*,*,#47361,.T.) ;
#65017=ORIENTED_EDGE('',*,*,#47366,.F.) ;
#65018=ORIENTED_EDGE('',*,*,#47367,.F.) ;
#65019=ORIENTED_EDGE('',*,*,#47363,.T.) ;
#65020=ORIENTED_EDGE('',*,*,#45494,.F.) ;
#65021=ORIENTED_EDGE('',*,*,#47368,.F.) ;
#65022=ORIENTED_EDGE('',*,*,#45649,.F.) ;
#65023=ORIENTED_EDGE('',*,*,#47369,.F.) ;
#65024=ORIENTED_EDGE('',*,*,#45650,.F.) ;
#65025=ORIENTED_EDGE('',*,*,#47370,.F.) ;
#65026=ORIENTED_EDGE('',*,*,#45644,.F.) ;
#65027=ORIENTED_EDGE('',*,*,#44211,.T.) ;
#65028=ORIENTED_EDGE('',*,*,#47369,.T.) ;
#65029=ORIENTED_EDGE('',*,*,#47371,.F.) ;
#65030=ORIENTED_EDGE('',*,*,#44434,.T.) ;
#65031=ORIENTED_EDGE('',*,*,#47365,.T.) ;
#65032=ORIENTED_EDGE('',*,*,#47364,.T.) ;
#65033=ORIENTED_EDGE('',*,*,#47372,.F.) ;
#65034=ORIENTED_EDGE('',*,*,#47373,.F.) ;
#65035=ORIENTED_EDGE('',*,*,#44607,.F.) ;
#65036=ORIENTED_EDGE('',*,*,#47374,.F.) ;
#65037=ORIENTED_EDGE('',*,*,#47375,.F.) ;
#65038=ORIENTED_EDGE('',*,*,#47366,.T.) ;
#65039=ORIENTED_EDGE('',*,*,#44535,.F.) ;
#65040=ORIENTED_EDGE('',*,*,#47374,.T.) ;
#65041=ORIENTED_EDGE('',*,*,#44723,.F.) ;
#65042=ORIENTED_EDGE('',*,*,#47367,.T.) ;
#65043=ORIENTED_EDGE('',*,*,#47376,.F.) ;
#65044=ORIENTED_EDGE('',*,*,#47377,.F.) ;
#65045=ORIENTED_EDGE('',*,*,#47370,.T.) ;
#65046=ORIENTED_EDGE('',*,*,#47368,.T.) ;
#65047=ORIENTED_EDGE('',*,*,#47378,.F.) ;
#65048=ORIENTED_EDGE('',*,*,#47371,.T.) ;
#65049=ORIENTED_EDGE('',*,*,#45647,.F.) ;
#65050=ORIENTED_EDGE('',*,*,#47379,.F.) ;
#65051=ORIENTED_EDGE('',*,*,#44435,.F.) ;
#65052=ORIENTED_EDGE('',*,*,#47372,.T.) ;
#65053=ORIENTED_EDGE('',*,*,#44438,.F.) ;
#65054=ORIENTED_EDGE('',*,*,#47380,.F.) ;
#65055=ORIENTED_EDGE('',*,*,#44533,.F.) ;
#65056=ORIENTED_EDGE('',*,*,#47373,.T.) ;
#65057=ORIENTED_EDGE('',*,*,#44534,.F.) ;
#65058=ORIENTED_EDGE('',*,*,#47381,.F.) ;
#65059=ORIENTED_EDGE('',*,*,#44686,.F.) ;
#65060=ORIENTED_EDGE('',*,*,#47375,.T.) ;
#65061=ORIENTED_EDGE('',*,*,#44722,.T.) ;
#65062=ORIENTED_EDGE('',*,*,#47382,.F.) ;
#65063=ORIENTED_EDGE('',*,*,#47376,.T.) ;
#65064=ORIENTED_EDGE('',*,*,#45491,.F.) ;
#65065=ORIENTED_EDGE('',*,*,#47377,.T.) ;
#65066=ORIENTED_EDGE('',*,*,#47383,.F.) ;
#65067=ORIENTED_EDGE('',*,*,#47384,.F.) ;
#65068=ORIENTED_EDGE('',*,*,#47378,.T.) ;
#65069=ORIENTED_EDGE('',*,*,#45493,.F.) ;
#65070=ORIENTED_EDGE('',*,*,#47385,.F.) ;
#65071=ORIENTED_EDGE('',*,*,#45645,.F.) ;
#65072=ORIENTED_EDGE('',*,*,#47386,.F.) ;
#65073=ORIENTED_EDGE('',*,*,#45646,.F.) ;
#65074=ORIENTED_EDGE('',*,*,#47387,.F.) ;
#65075=ORIENTED_EDGE('',*,*,#44530,.F.) ;
#65076=ORIENTED_EDGE('',*,*,#47379,.T.) ;
#65077=ORIENTED_EDGE('',*,*,#47386,.T.) ;
#65078=ORIENTED_EDGE('',*,*,#47388,.F.) ;
#65079=ORIENTED_EDGE('',*,*,#47381,.T.) ;
#65080=ORIENTED_EDGE('',*,*,#47380,.T.) ;
#65081=ORIENTED_EDGE('',*,*,#47389,.F.) ;
#65082=ORIENTED_EDGE('',*,*,#44687,.T.) ;
#65083=ORIENTED_EDGE('',*,*,#47390,.F.) ;
#65084=ORIENTED_EDGE('',*,*,#47383,.T.) ;
#65085=ORIENTED_EDGE('',*,*,#47382,.T.) ;
#65086=ORIENTED_EDGE('',*,*,#44721,.F.) ;
#65087=ORIENTED_EDGE('',*,*,#47384,.T.) ;
#65088=ORIENTED_EDGE('',*,*,#47391,.F.) ;
#65089=ORIENTED_EDGE('',*,*,#47392,.F.) ;
#65090=ORIENTED_EDGE('',*,*,#47387,.T.) ;
#65091=ORIENTED_EDGE('',*,*,#47385,.T.) ;
#65092=ORIENTED_EDGE('',*,*,#47393,.F.) ;
#65093=ORIENTED_EDGE('',*,*,#44526,.T.) ;
#65094=ORIENTED_EDGE('',*,*,#47388,.T.) ;
#65095=ORIENTED_EDGE('',*,*,#44529,.F.) ;
#65096=ORIENTED_EDGE('',*,*,#47394,.F.) ;
#65097=ORIENTED_EDGE('',*,*,#44436,.F.) ;
#65098=ORIENTED_EDGE('',*,*,#47389,.T.) ;
#65099=ORIENTED_EDGE('',*,*,#44437,.F.) ;
#65100=ORIENTED_EDGE('',*,*,#47395,.F.) ;
#65101=ORIENTED_EDGE('',*,*,#44688,.F.) ;
#65102=ORIENTED_EDGE('',*,*,#47390,.T.) ;
#65103=ORIENTED_EDGE('',*,*,#44720,.T.) ;
#65104=ORIENTED_EDGE('',*,*,#47396,.F.) ;
#65105=ORIENTED_EDGE('',*,*,#47391,.T.) ;
#65106=ORIENTED_EDGE('',*,*,#45492,.F.) ;
#65107=ORIENTED_EDGE('',*,*,#47392,.T.) ;
#65108=ORIENTED_EDGE('',*,*,#47397,.F.) ;
#65109=ORIENTED_EDGE('',*,*,#47393,.T.) ;
#65110=ORIENTED_EDGE('',*,*,#47395,.T.) ;
#65111=ORIENTED_EDGE('',*,*,#47394,.T.) ;
#65112=ORIENTED_EDGE('',*,*,#47398,.F.) ;
#65113=ORIENTED_EDGE('',*,*,#44689,.T.) ;
#65114=ORIENTED_EDGE('',*,*,#47396,.T.) ;
#65115=ORIENTED_EDGE('',*,*,#44719,.F.) ;
#65116=ORIENTED_EDGE('',*,*,#47399,.F.) ;
#65117=ORIENTED_EDGE('',*,*,#44527,.F.) ;
#65118=ORIENTED_EDGE('',*,*,#47397,.T.) ;
#65119=ORIENTED_EDGE('',*,*,#47398,.T.) ;
#65120=ORIENTED_EDGE('',*,*,#44528,.F.) ;
#65121=ORIENTED_EDGE('',*,*,#47400,.F.) ;
#65122=ORIENTED_EDGE('',*,*,#44690,.F.) ;
#65123=ORIENTED_EDGE('',*,*,#47399,.T.) ;
#65124=ORIENTED_EDGE('',*,*,#44613,.F.) ;
#65125=ORIENTED_EDGE('',*,*,#47400,.T.) ;
#65126=ORIENTED_EDGE('',*,*,#47401,.F.) ;
#65127=ORIENTED_EDGE('',*,*,#46052,.F.) ;
#65128=ORIENTED_EDGE('',*,*,#47402,.F.) ;
#65129=ORIENTED_EDGE('',*,*,#46099,.F.) ;
#65130=ORIENTED_EDGE('',*,*,#47402,.T.) ;
#65131=ORIENTED_EDGE('',*,*,#46049,.F.) ;
#65132=ORIENTED_EDGE('',*,*,#47403,.F.) ;
#65133=ORIENTED_EDGE('',*,*,#46100,.F.) ;
#65134=ORIENTED_EDGE('',*,*,#46055,.F.) ;
#65135=ORIENTED_EDGE('',*,*,#47401,.T.) ;
#65136=ORIENTED_EDGE('',*,*,#47404,.F.) ;
#65137=ORIENTED_EDGE('',*,*,#47403,.T.) ;
#65138=ORIENTED_EDGE('',*,*,#46046,.F.) ;
#65139=ORIENTED_EDGE('',*,*,#47405,.F.) ;
#65140=ORIENTED_EDGE('',*,*,#46101,.F.) ;
#65141=ORIENTED_EDGE('',*,*,#47404,.T.) ;
#65142=ORIENTED_EDGE('',*,*,#46098,.F.) ;
#65143=ORIENTED_EDGE('',*,*,#47406,.F.) ;
#65144=ORIENTED_EDGE('',*,*,#46058,.F.) ;
#65145=ORIENTED_EDGE('',*,*,#47405,.T.) ;
#65146=ORIENTED_EDGE('',*,*,#46043,.F.) ;
#65147=ORIENTED_EDGE('',*,*,#47407,.F.) ;
#65148=ORIENTED_EDGE('',*,*,#46102,.F.) ;
#65149=ORIENTED_EDGE('',*,*,#46061,.F.) ;
#65150=ORIENTED_EDGE('',*,*,#47406,.T.) ;
#65151=ORIENTED_EDGE('',*,*,#47408,.F.) ;
#65152=ORIENTED_EDGE('',*,*,#47407,.T.) ;
#65153=ORIENTED_EDGE('',*,*,#46040,.F.) ;
#65154=ORIENTED_EDGE('',*,*,#47409,.F.) ;
#65155=ORIENTED_EDGE('',*,*,#46103,.F.) ;
#65156=ORIENTED_EDGE('',*,*,#47408,.T.) ;
#65157=ORIENTED_EDGE('',*,*,#46097,.F.) ;
#65158=ORIENTED_EDGE('',*,*,#47410,.F.) ;
#65159=ORIENTED_EDGE('',*,*,#46064,.F.) ;
#65160=ORIENTED_EDGE('',*,*,#47409,.T.) ;
#65161=ORIENTED_EDGE('',*,*,#46037,.F.) ;
#65162=ORIENTED_EDGE('',*,*,#47411,.F.) ;
#65163=ORIENTED_EDGE('',*,*,#46067,.F.) ;
#65164=ORIENTED_EDGE('',*,*,#47410,.T.) ;
#65165=ORIENTED_EDGE('',*,*,#47412,.F.) ;
#65166=ORIENTED_EDGE('',*,*,#47411,.T.) ;
#65167=ORIENTED_EDGE('',*,*,#46034,.F.) ;
#65168=ORIENTED_EDGE('',*,*,#47413,.F.) ;
#65169=ORIENTED_EDGE('',*,*,#46104,.F.) ;
#65170=ORIENTED_EDGE('',*,*,#47412,.T.) ;
#65171=ORIENTED_EDGE('',*,*,#46096,.F.) ;
#65172=ORIENTED_EDGE('',*,*,#47414,.F.) ;
#65173=ORIENTED_EDGE('',*,*,#46070,.F.) ;
#65174=ORIENTED_EDGE('',*,*,#47413,.T.) ;
#65175=ORIENTED_EDGE('',*,*,#44360,.F.) ;
#65176=ORIENTED_EDGE('',*,*,#47415,.F.) ;
#65177=ORIENTED_EDGE('',*,*,#46073,.F.) ;
#65178=ORIENTED_EDGE('',*,*,#47414,.T.) ;
#65179=ORIENTED_EDGE('',*,*,#47416,.F.) ;
#65180=ORIENTED_EDGE('',*,*,#47415,.T.) ;
#65181=ORIENTED_EDGE('',*,*,#46032,.F.) ;
#65182=ORIENTED_EDGE('',*,*,#44207,.F.) ;
#65183=ORIENTED_EDGE('',*,*,#46105,.F.) ;
#65184=ORIENTED_EDGE('',*,*,#47416,.T.) ;
#65185=ORIENTED_EDGE('',*,*,#46095,.F.) ;
#65186=ORIENTED_EDGE('',*,*,#47417,.F.) ;
#65187=ORIENTED_EDGE('',*,*,#46076,.F.) ;
#65188=ORIENTED_EDGE('',*,*,#46079,.F.) ;
#65189=ORIENTED_EDGE('',*,*,#47417,.T.) ;
#65190=ORIENTED_EDGE('',*,*,#47418,.F.) ;
#65191=ORIENTED_EDGE('',*,*,#44206,.T.) ;
#65192=ORIENTED_EDGE('',*,*,#46027,.F.) ;
#65193=ORIENTED_EDGE('',*,*,#47419,.F.) ;
#65194=ORIENTED_EDGE('',*,*,#46106,.F.) ;
#65195=ORIENTED_EDGE('',*,*,#47418,.T.) ;
#65196=ORIENTED_EDGE('',*,*,#46094,.F.) ;
#65197=ORIENTED_EDGE('',*,*,#47420,.F.) ;
#65198=ORIENTED_EDGE('',*,*,#46082,.F.) ;
#65199=ORIENTED_EDGE('',*,*,#47419,.T.) ;
#65200=ORIENTED_EDGE('',*,*,#46024,.F.) ;
#65201=ORIENTED_EDGE('',*,*,#47421,.F.) ;
#65202=ORIENTED_EDGE('',*,*,#46085,.F.) ;
#65203=ORIENTED_EDGE('',*,*,#47420,.T.) ;
#65204=ORIENTED_EDGE('',*,*,#47422,.F.) ;
#65205=ORIENTED_EDGE('',*,*,#47421,.T.) ;
#65206=ORIENTED_EDGE('',*,*,#46021,.F.) ;
#65207=ORIENTED_EDGE('',*,*,#47423,.F.) ;
#65208=ORIENTED_EDGE('',*,*,#46107,.F.) ;
#65209=ORIENTED_EDGE('',*,*,#47422,.T.) ;
#65210=ORIENTED_EDGE('',*,*,#46093,.F.) ;
#65211=ORIENTED_EDGE('',*,*,#47424,.F.) ;
#65212=ORIENTED_EDGE('',*,*,#46088,.F.) ;
#65213=ORIENTED_EDGE('',*,*,#47423,.T.) ;
#65214=ORIENTED_EDGE('',*,*,#46018,.F.) ;
#65215=ORIENTED_EDGE('',*,*,#47425,.F.) ;
#65216=ORIENTED_EDGE('',*,*,#46090,.F.) ;
#65217=ORIENTED_EDGE('',*,*,#47424,.T.) ;
#65218=ORIENTED_EDGE('',*,*,#46092,.F.) ;
#65219=ORIENTED_EDGE('',*,*,#47426,.F.) ;
#65220=ORIENTED_EDGE('',*,*,#46012,.F.) ;
#65221=ORIENTED_EDGE('',*,*,#47425,.T.) ;
#65222=ORIENTED_EDGE('',*,*,#46015,.F.) ;
#65223=ORIENTED_EDGE('',*,*,#47426,.T.) ;
#65224=ORIENTED_EDGE('',*,*,#46091,.F.) ;
#65225=ORIENTED_EDGE('',*,*,#47427,.F.) ;
#65226=ORIENTED_EDGE('',*,*,#45675,.F.) ;
#65227=ORIENTED_EDGE('',*,*,#47428,.F.) ;
#65228=ORIENTED_EDGE('',*,*,#45488,.F.) ;
#65229=ORIENTED_EDGE('',*,*,#47429,.F.) ;
#65230=ORIENTED_EDGE('',*,*,#45676,.F.) ;
#65231=ORIENTED_EDGE('',*,*,#47430,.F.) ;
#65232=ORIENTED_EDGE('',*,*,#45670,.F.) ;
#65233=ORIENTED_EDGE('',*,*,#47431,.F.) ;
#65234=ORIENTED_EDGE('',*,*,#47429,.T.) ;
#65235=ORIENTED_EDGE('',*,*,#47432,.F.) ;
#65236=ORIENTED_EDGE('',*,*,#47433,.F.) ;
#65237=ORIENTED_EDGE('',*,*,#47428,.T.) ;
#65238=ORIENTED_EDGE('',*,*,#47434,.F.) ;
#65239=ORIENTED_EDGE('',*,*,#47427,.T.) ;
#65240=ORIENTED_EDGE('',*,*,#45487,.T.) ;
#65241=ORIENTED_EDGE('',*,*,#47435,.F.) ;
#65242=ORIENTED_EDGE('',*,*,#47430,.T.) ;
#65243=ORIENTED_EDGE('',*,*,#47432,.T.) ;
#65244=ORIENTED_EDGE('',*,*,#45673,.F.) ;
#65245=ORIENTED_EDGE('',*,*,#47436,.F.) ;
#65246=ORIENTED_EDGE('',*,*,#44191,.T.) ;
#65247=ORIENTED_EDGE('',*,*,#47437,.T.) ;
#65248=ORIENTED_EDGE('',*,*,#47438,.F.) ;
#65249=ORIENTED_EDGE('',*,*,#47431,.T.) ;
#65250=ORIENTED_EDGE('',*,*,#47439,.F.) ;
#65251=ORIENTED_EDGE('',*,*,#47440,.T.) ;
#65252=ORIENTED_EDGE('',*,*,#47441,.F.) ;
#65253=ORIENTED_EDGE('',*,*,#44419,.F.) ;
#65254=ORIENTED_EDGE('',*,*,#47442,.F.) ;
#65255=ORIENTED_EDGE('',*,*,#45677,.F.) ;
#65256=ORIENTED_EDGE('',*,*,#47434,.T.) ;
#65257=ORIENTED_EDGE('',*,*,#45674,.F.) ;
#65258=ORIENTED_EDGE('',*,*,#47443,.F.) ;
#65259=ORIENTED_EDGE('',*,*,#45680,.F.) ;
#65260=ORIENTED_EDGE('',*,*,#47433,.T.) ;
#65261=ORIENTED_EDGE('',*,*,#45679,.F.) ;
#65262=ORIENTED_EDGE('',*,*,#47444,.F.) ;
#65263=ORIENTED_EDGE('',*,*,#45479,.F.) ;
#65264=ORIENTED_EDGE('',*,*,#47435,.T.) ;
#65265=ORIENTED_EDGE('',*,*,#45486,.F.) ;
#65266=ORIENTED_EDGE('',*,*,#47445,.F.) ;
#65267=ORIENTED_EDGE('',*,*,#45671,.F.) ;
#65268=ORIENTED_EDGE('',*,*,#47446,.F.) ;
#65269=ORIENTED_EDGE('',*,*,#45672,.F.) ;
#65270=ORIENTED_EDGE('',*,*,#47447,.F.) ;
#65271=ORIENTED_EDGE('',*,*,#45667,.F.) ;
#65272=ORIENTED_EDGE('',*,*,#47436,.T.) ;
#65273=ORIENTED_EDGE('',*,*,#47446,.T.) ;
#65274=ORIENTED_EDGE('',*,*,#44192,.F.) ;
#65275=ORIENTED_EDGE('',*,*,#47442,.T.) ;
#65276=ORIENTED_EDGE('',*,*,#44429,.T.) ;
#65277=ORIENTED_EDGE('',*,*,#47448,.F.) ;
#65278=ORIENTED_EDGE('',*,*,#47443,.T.) ;
#65279=ORIENTED_EDGE('',*,*,#47449,.F.) ;
#65280=ORIENTED_EDGE('',*,*,#47444,.T.) ;
#65281=ORIENTED_EDGE('',*,*,#47450,.F.) ;
#65282=ORIENTED_EDGE('',*,*,#44521,.T.) ;
#65283=ORIENTED_EDGE('',*,*,#47445,.T.) ;
#65284=ORIENTED_EDGE('',*,*,#45485,.T.) ;
#65285=ORIENTED_EDGE('',*,*,#47451,.F.) ;
#65286=ORIENTED_EDGE('',*,*,#47447,.T.) ;
#65287=ORIENTED_EDGE('',*,*,#47448,.T.) ;
#65288=ORIENTED_EDGE('',*,*,#44428,.F.) ;
#65289=ORIENTED_EDGE('',*,*,#47452,.F.) ;
#65290=ORIENTED_EDGE('',*,*,#45681,.F.) ;
#65291=ORIENTED_EDGE('',*,*,#47450,.T.) ;
#65292=ORIENTED_EDGE('',*,*,#45678,.F.) ;
#65293=ORIENTED_EDGE('',*,*,#47453,.F.) ;
#65294=ORIENTED_EDGE('',*,*,#44522,.F.) ;
#65295=ORIENTED_EDGE('',*,*,#45480,.F.) ;
#65296=ORIENTED_EDGE('',*,*,#47449,.T.) ;
#65297=ORIENTED_EDGE('',*,*,#47454,.F.) ;
#65298=ORIENTED_EDGE('',*,*,#47455,.F.) ;
#65299=ORIENTED_EDGE('',*,*,#47451,.T.) ;
#65300=ORIENTED_EDGE('',*,*,#45484,.F.) ;
#65301=ORIENTED_EDGE('',*,*,#47456,.F.) ;
#65302=ORIENTED_EDGE('',*,*,#45668,.F.) ;
#65303=ORIENTED_EDGE('',*,*,#47457,.F.) ;
#65304=ORIENTED_EDGE('',*,*,#45669,.F.) ;
#65305=ORIENTED_EDGE('',*,*,#47458,.F.) ;
#65306=ORIENTED_EDGE('',*,*,#45663,.F.) ;
#65307=ORIENTED_EDGE('',*,*,#44194,.T.) ;
#65308=ORIENTED_EDGE('',*,*,#47457,.T.) ;
#65309=ORIENTED_EDGE('',*,*,#47459,.F.) ;
#65310=ORIENTED_EDGE('',*,*,#44423,.T.) ;
#65311=ORIENTED_EDGE('',*,*,#47453,.T.) ;
#65312=ORIENTED_EDGE('',*,*,#47452,.T.) ;
#65313=ORIENTED_EDGE('',*,*,#47460,.F.) ;
#65314=ORIENTED_EDGE('',*,*,#47461,.F.) ;
#65315=ORIENTED_EDGE('',*,*,#44611,.F.) ;
#65316=ORIENTED_EDGE('',*,*,#47462,.F.) ;
#65317=ORIENTED_EDGE('',*,*,#47463,.F.) ;
#65318=ORIENTED_EDGE('',*,*,#47454,.T.) ;
#65319=ORIENTED_EDGE('',*,*,#44525,.F.) ;
#65320=ORIENTED_EDGE('',*,*,#47462,.T.) ;
#65321=ORIENTED_EDGE('',*,*,#44718,.F.) ;
#65322=ORIENTED_EDGE('',*,*,#47455,.T.) ;
#65323=ORIENTED_EDGE('',*,*,#47464,.F.) ;
#65324=ORIENTED_EDGE('',*,*,#47465,.F.) ;
#65325=ORIENTED_EDGE('',*,*,#47458,.T.) ;
#65326=ORIENTED_EDGE('',*,*,#47456,.T.) ;
#65327=ORIENTED_EDGE('',*,*,#47466,.F.) ;
#65328=ORIENTED_EDGE('',*,*,#47459,.T.) ;
#65329=ORIENTED_EDGE('',*,*,#45666,.F.) ;
#65330=ORIENTED_EDGE('',*,*,#47467,.F.) ;
#65331=ORIENTED_EDGE('',*,*,#44424,.F.) ;
#65332=ORIENTED_EDGE('',*,*,#47460,.T.) ;
#65333=ORIENTED_EDGE('',*,*,#44427,.F.) ;
#65334=ORIENTED_EDGE('',*,*,#47468,.F.) ;
#65335=ORIENTED_EDGE('',*,*,#44523,.F.) ;
#65336=ORIENTED_EDGE('',*,*,#47461,.T.) ;
#65337=ORIENTED_EDGE('',*,*,#44524,.F.) ;
#65338=ORIENTED_EDGE('',*,*,#47469,.F.) ;
#65339=ORIENTED_EDGE('',*,*,#44691,.F.) ;
#65340=ORIENTED_EDGE('',*,*,#47463,.T.) ;
#65341=ORIENTED_EDGE('',*,*,#44717,.T.) ;
#65342=ORIENTED_EDGE('',*,*,#47470,.F.) ;
#65343=ORIENTED_EDGE('',*,*,#47464,.T.) ;
#65344=ORIENTED_EDGE('',*,*,#45481,.F.) ;
#65345=ORIENTED_EDGE('',*,*,#47465,.T.) ;
#65346=ORIENTED_EDGE('',*,*,#47471,.F.) ;
#65347=ORIENTED_EDGE('',*,*,#47472,.F.) ;
#65348=ORIENTED_EDGE('',*,*,#47466,.T.) ;
#65349=ORIENTED_EDGE('',*,*,#45483,.F.) ;
#65350=ORIENTED_EDGE('',*,*,#47473,.F.) ;
#65351=ORIENTED_EDGE('',*,*,#45664,.F.) ;
#65352=ORIENTED_EDGE('',*,*,#47474,.F.) ;
#65353=ORIENTED_EDGE('',*,*,#45665,.F.) ;
#65354=ORIENTED_EDGE('',*,*,#47475,.F.) ;
#65355=ORIENTED_EDGE('',*,*,#44520,.F.) ;
#65356=ORIENTED_EDGE('',*,*,#47467,.T.) ;
#65357=ORIENTED_EDGE('',*,*,#47474,.T.) ;
#65358=ORIENTED_EDGE('',*,*,#47476,.F.) ;
#65359=ORIENTED_EDGE('',*,*,#47469,.T.) ;
#65360=ORIENTED_EDGE('',*,*,#47468,.T.) ;
#65361=ORIENTED_EDGE('',*,*,#47477,.F.) ;
#65362=ORIENTED_EDGE('',*,*,#44692,.T.) ;
#65363=ORIENTED_EDGE('',*,*,#47478,.F.) ;
#65364=ORIENTED_EDGE('',*,*,#47471,.T.) ;
#65365=ORIENTED_EDGE('',*,*,#47470,.T.) ;
#65366=ORIENTED_EDGE('',*,*,#44716,.F.) ;
#65367=ORIENTED_EDGE('',*,*,#47472,.T.) ;
#65368=ORIENTED_EDGE('',*,*,#47479,.F.) ;
#65369=ORIENTED_EDGE('',*,*,#47480,.F.) ;
#65370=ORIENTED_EDGE('',*,*,#47475,.T.) ;
#65371=ORIENTED_EDGE('',*,*,#47473,.T.) ;
#65372=ORIENTED_EDGE('',*,*,#47481,.F.) ;
#65373=ORIENTED_EDGE('',*,*,#44516,.T.) ;
#65374=ORIENTED_EDGE('',*,*,#47476,.T.) ;
#65375=ORIENTED_EDGE('',*,*,#44519,.F.) ;
#65376=ORIENTED_EDGE('',*,*,#47482,.F.) ;
#65377=ORIENTED_EDGE('',*,*,#44425,.F.) ;
#65378=ORIENTED_EDGE('',*,*,#47477,.T.) ;
#65379=ORIENTED_EDGE('',*,*,#44426,.F.) ;
#65380=ORIENTED_EDGE('',*,*,#47483,.F.) ;
#65381=ORIENTED_EDGE('',*,*,#44693,.F.) ;
#65382=ORIENTED_EDGE('',*,*,#47478,.T.) ;
#65383=ORIENTED_EDGE('',*,*,#44715,.T.) ;
#65384=ORIENTED_EDGE('',*,*,#47484,.F.) ;
#65385=ORIENTED_EDGE('',*,*,#47479,.T.) ;
#65386=ORIENTED_EDGE('',*,*,#45482,.F.) ;
#65387=ORIENTED_EDGE('',*,*,#47480,.T.) ;
#65388=ORIENTED_EDGE('',*,*,#47485,.F.) ;
#65389=ORIENTED_EDGE('',*,*,#47481,.T.) ;
#65390=ORIENTED_EDGE('',*,*,#47483,.T.) ;
#65391=ORIENTED_EDGE('',*,*,#47482,.T.) ;
#65392=ORIENTED_EDGE('',*,*,#47486,.F.) ;
#65393=ORIENTED_EDGE('',*,*,#44694,.T.) ;
#65394=ORIENTED_EDGE('',*,*,#47484,.T.) ;
#65395=ORIENTED_EDGE('',*,*,#44714,.F.) ;
#65396=ORIENTED_EDGE('',*,*,#47487,.F.) ;
#65397=ORIENTED_EDGE('',*,*,#44517,.F.) ;
#65398=ORIENTED_EDGE('',*,*,#47485,.T.) ;
#65399=ORIENTED_EDGE('',*,*,#47486,.T.) ;
#65400=ORIENTED_EDGE('',*,*,#44518,.F.) ;
#65401=ORIENTED_EDGE('',*,*,#47488,.F.) ;
#65402=ORIENTED_EDGE('',*,*,#44695,.F.) ;
#65403=ORIENTED_EDGE('',*,*,#47487,.T.) ;
#65404=ORIENTED_EDGE('',*,*,#44617,.F.) ;
#65405=ORIENTED_EDGE('',*,*,#47488,.T.) ;
#65406=ORIENTED_EDGE('',*,*,#47489,.F.) ;
#65407=ORIENTED_EDGE('',*,*,#45955,.F.) ;
#65408=ORIENTED_EDGE('',*,*,#47490,.F.) ;
#65409=ORIENTED_EDGE('',*,*,#46002,.F.) ;
#65410=ORIENTED_EDGE('',*,*,#47490,.T.) ;
#65411=ORIENTED_EDGE('',*,*,#45952,.F.) ;
#65412=ORIENTED_EDGE('',*,*,#47491,.F.) ;
#65413=ORIENTED_EDGE('',*,*,#46003,.F.) ;
#65414=ORIENTED_EDGE('',*,*,#45958,.F.) ;
#65415=ORIENTED_EDGE('',*,*,#47489,.T.) ;
#65416=ORIENTED_EDGE('',*,*,#47492,.F.) ;
#65417=ORIENTED_EDGE('',*,*,#47491,.T.) ;
#65418=ORIENTED_EDGE('',*,*,#45949,.F.) ;
#65419=ORIENTED_EDGE('',*,*,#47493,.F.) ;
#65420=ORIENTED_EDGE('',*,*,#46004,.F.) ;
#65421=ORIENTED_EDGE('',*,*,#47492,.T.) ;
#65422=ORIENTED_EDGE('',*,*,#46001,.F.) ;
#65423=ORIENTED_EDGE('',*,*,#47494,.F.) ;
#65424=ORIENTED_EDGE('',*,*,#45961,.F.) ;
#65425=ORIENTED_EDGE('',*,*,#47493,.T.) ;
#65426=ORIENTED_EDGE('',*,*,#45946,.F.) ;
#65427=ORIENTED_EDGE('',*,*,#47495,.F.) ;
#65428=ORIENTED_EDGE('',*,*,#46005,.F.) ;
#65429=ORIENTED_EDGE('',*,*,#45964,.F.) ;
#65430=ORIENTED_EDGE('',*,*,#47494,.T.) ;
#65431=ORIENTED_EDGE('',*,*,#47496,.F.) ;
#65432=ORIENTED_EDGE('',*,*,#47495,.T.) ;
#65433=ORIENTED_EDGE('',*,*,#45943,.F.) ;
#65434=ORIENTED_EDGE('',*,*,#47497,.F.) ;
#65435=ORIENTED_EDGE('',*,*,#46006,.F.) ;
#65436=ORIENTED_EDGE('',*,*,#47496,.T.) ;
#65437=ORIENTED_EDGE('',*,*,#46000,.F.) ;
#65438=ORIENTED_EDGE('',*,*,#47498,.F.) ;
#65439=ORIENTED_EDGE('',*,*,#45967,.F.) ;
#65440=ORIENTED_EDGE('',*,*,#47497,.T.) ;
#65441=ORIENTED_EDGE('',*,*,#45940,.F.) ;
#65442=ORIENTED_EDGE('',*,*,#47499,.F.) ;
#65443=ORIENTED_EDGE('',*,*,#45970,.F.) ;
#65444=ORIENTED_EDGE('',*,*,#47498,.T.) ;
#65445=ORIENTED_EDGE('',*,*,#47500,.F.) ;
#65446=ORIENTED_EDGE('',*,*,#47499,.T.) ;
#65447=ORIENTED_EDGE('',*,*,#45937,.F.) ;
#65448=ORIENTED_EDGE('',*,*,#47501,.F.) ;
#65449=ORIENTED_EDGE('',*,*,#46007,.F.) ;
#65450=ORIENTED_EDGE('',*,*,#47500,.T.) ;
#65451=ORIENTED_EDGE('',*,*,#45999,.F.) ;
#65452=ORIENTED_EDGE('',*,*,#47502,.F.) ;
#65453=ORIENTED_EDGE('',*,*,#45973,.F.) ;
#65454=ORIENTED_EDGE('',*,*,#47501,.T.) ;
#65455=ORIENTED_EDGE('',*,*,#44363,.F.) ;
#65456=ORIENTED_EDGE('',*,*,#47503,.F.) ;
#65457=ORIENTED_EDGE('',*,*,#45976,.F.) ;
#65458=ORIENTED_EDGE('',*,*,#47502,.T.) ;
#65459=ORIENTED_EDGE('',*,*,#47504,.F.) ;
#65460=ORIENTED_EDGE('',*,*,#47503,.T.) ;
#65461=ORIENTED_EDGE('',*,*,#45935,.F.) ;
#65462=ORIENTED_EDGE('',*,*,#44190,.F.) ;
#65463=ORIENTED_EDGE('',*,*,#46008,.F.) ;
#65464=ORIENTED_EDGE('',*,*,#47504,.T.) ;
#65465=ORIENTED_EDGE('',*,*,#45998,.F.) ;
#65466=ORIENTED_EDGE('',*,*,#47505,.F.) ;
#65467=ORIENTED_EDGE('',*,*,#45979,.F.) ;
#65468=ORIENTED_EDGE('',*,*,#45982,.F.) ;
#65469=ORIENTED_EDGE('',*,*,#47505,.T.) ;
#65470=ORIENTED_EDGE('',*,*,#47506,.F.) ;
#65471=ORIENTED_EDGE('',*,*,#44189,.T.) ;
#65472=ORIENTED_EDGE('',*,*,#45930,.F.) ;
#65473=ORIENTED_EDGE('',*,*,#47507,.F.) ;
#65474=ORIENTED_EDGE('',*,*,#46009,.F.) ;
#65475=ORIENTED_EDGE('',*,*,#47506,.T.) ;
#65476=ORIENTED_EDGE('',*,*,#45997,.F.) ;
#65477=ORIENTED_EDGE('',*,*,#47508,.F.) ;
#65478=ORIENTED_EDGE('',*,*,#45985,.F.) ;
#65479=ORIENTED_EDGE('',*,*,#47507,.T.) ;
#65480=ORIENTED_EDGE('',*,*,#45927,.F.) ;
#65481=ORIENTED_EDGE('',*,*,#47509,.F.) ;
#65482=ORIENTED_EDGE('',*,*,#45988,.F.) ;
#65483=ORIENTED_EDGE('',*,*,#47508,.T.) ;
#65484=ORIENTED_EDGE('',*,*,#47510,.F.) ;
#65485=ORIENTED_EDGE('',*,*,#47509,.T.) ;
#65486=ORIENTED_EDGE('',*,*,#45924,.F.) ;
#65487=ORIENTED_EDGE('',*,*,#47511,.F.) ;
#65488=ORIENTED_EDGE('',*,*,#46010,.F.) ;
#65489=ORIENTED_EDGE('',*,*,#47510,.T.) ;
#65490=ORIENTED_EDGE('',*,*,#45996,.F.) ;
#65491=ORIENTED_EDGE('',*,*,#47512,.F.) ;
#65492=ORIENTED_EDGE('',*,*,#45991,.F.) ;
#65493=ORIENTED_EDGE('',*,*,#47511,.T.) ;
#65494=ORIENTED_EDGE('',*,*,#45921,.F.) ;
#65495=ORIENTED_EDGE('',*,*,#47513,.F.) ;
#65496=ORIENTED_EDGE('',*,*,#45993,.F.) ;
#65497=ORIENTED_EDGE('',*,*,#47512,.T.) ;
#65498=ORIENTED_EDGE('',*,*,#45995,.F.) ;
#65499=ORIENTED_EDGE('',*,*,#47514,.F.) ;
#65500=ORIENTED_EDGE('',*,*,#45915,.F.) ;
#65501=ORIENTED_EDGE('',*,*,#47513,.T.) ;
#65502=ORIENTED_EDGE('',*,*,#45918,.F.) ;
#65503=ORIENTED_EDGE('',*,*,#47514,.T.) ;
#65504=ORIENTED_EDGE('',*,*,#45994,.F.) ;
#65505=ORIENTED_EDGE('',*,*,#47515,.F.) ;
#65506=ORIENTED_EDGE('',*,*,#45694,.F.) ;
#65507=ORIENTED_EDGE('',*,*,#47516,.F.) ;
#65508=ORIENTED_EDGE('',*,*,#45478,.F.) ;
#65509=ORIENTED_EDGE('',*,*,#47517,.F.) ;
#65510=ORIENTED_EDGE('',*,*,#45695,.F.) ;
#65511=ORIENTED_EDGE('',*,*,#47518,.F.) ;
#65512=ORIENTED_EDGE('',*,*,#45689,.F.) ;
#65513=ORIENTED_EDGE('',*,*,#47519,.F.) ;
#65514=ORIENTED_EDGE('',*,*,#47517,.T.) ;
#65515=ORIENTED_EDGE('',*,*,#47520,.F.) ;
#65516=ORIENTED_EDGE('',*,*,#47521,.F.) ;
#65517=ORIENTED_EDGE('',*,*,#47516,.T.) ;
#65518=ORIENTED_EDGE('',*,*,#47522,.F.) ;
#65519=ORIENTED_EDGE('',*,*,#47515,.T.) ;
#65520=ORIENTED_EDGE('',*,*,#45477,.T.) ;
#65521=ORIENTED_EDGE('',*,*,#47523,.F.) ;
#65522=ORIENTED_EDGE('',*,*,#47518,.T.) ;
#65523=ORIENTED_EDGE('',*,*,#47520,.T.) ;
#65524=ORIENTED_EDGE('',*,*,#45692,.F.) ;
#65525=ORIENTED_EDGE('',*,*,#47524,.F.) ;
#65526=ORIENTED_EDGE('',*,*,#44174,.T.) ;
#65527=ORIENTED_EDGE('',*,*,#47525,.T.) ;
#65528=ORIENTED_EDGE('',*,*,#47526,.F.) ;
#65529=ORIENTED_EDGE('',*,*,#47519,.T.) ;
#65530=ORIENTED_EDGE('',*,*,#47527,.F.) ;
#65531=ORIENTED_EDGE('',*,*,#47528,.T.) ;
#65532=ORIENTED_EDGE('',*,*,#47529,.F.) ;
#65533=ORIENTED_EDGE('',*,*,#44408,.F.) ;
#65534=ORIENTED_EDGE('',*,*,#47530,.F.) ;
#65535=ORIENTED_EDGE('',*,*,#45696,.F.) ;
#65536=ORIENTED_EDGE('',*,*,#47522,.T.) ;
#65537=ORIENTED_EDGE('',*,*,#45693,.F.) ;
#65538=ORIENTED_EDGE('',*,*,#47531,.F.) ;
#65539=ORIENTED_EDGE('',*,*,#45699,.F.) ;
#65540=ORIENTED_EDGE('',*,*,#47521,.T.) ;
#65541=ORIENTED_EDGE('',*,*,#45698,.F.) ;
#65542=ORIENTED_EDGE('',*,*,#47532,.F.) ;
#65543=ORIENTED_EDGE('',*,*,#45469,.F.) ;
#65544=ORIENTED_EDGE('',*,*,#47523,.T.) ;
#65545=ORIENTED_EDGE('',*,*,#45476,.F.) ;
#65546=ORIENTED_EDGE('',*,*,#47533,.F.) ;
#65547=ORIENTED_EDGE('',*,*,#45690,.F.) ;
#65548=ORIENTED_EDGE('',*,*,#47534,.F.) ;
#65549=ORIENTED_EDGE('',*,*,#45691,.F.) ;
#65550=ORIENTED_EDGE('',*,*,#47535,.F.) ;
#65551=ORIENTED_EDGE('',*,*,#45686,.F.) ;
#65552=ORIENTED_EDGE('',*,*,#47524,.T.) ;
#65553=ORIENTED_EDGE('',*,*,#47534,.T.) ;
#65554=ORIENTED_EDGE('',*,*,#44175,.F.) ;
#65555=ORIENTED_EDGE('',*,*,#47530,.T.) ;
#65556=ORIENTED_EDGE('',*,*,#44418,.T.) ;
#65557=ORIENTED_EDGE('',*,*,#47536,.F.) ;
#65558=ORIENTED_EDGE('',*,*,#47531,.T.) ;
#65559=ORIENTED_EDGE('',*,*,#47537,.F.) ;
#65560=ORIENTED_EDGE('',*,*,#47532,.T.) ;
#65561=ORIENTED_EDGE('',*,*,#47538,.F.) ;
#65562=ORIENTED_EDGE('',*,*,#44511,.T.) ;
#65563=ORIENTED_EDGE('',*,*,#47533,.T.) ;
#65564=ORIENTED_EDGE('',*,*,#45475,.T.) ;
#65565=ORIENTED_EDGE('',*,*,#47539,.F.) ;
#65566=ORIENTED_EDGE('',*,*,#47535,.T.) ;
#65567=ORIENTED_EDGE('',*,*,#47536,.T.) ;
#65568=ORIENTED_EDGE('',*,*,#44417,.F.) ;
#65569=ORIENTED_EDGE('',*,*,#47540,.F.) ;
#65570=ORIENTED_EDGE('',*,*,#45700,.F.) ;
#65571=ORIENTED_EDGE('',*,*,#47538,.T.) ;
#65572=ORIENTED_EDGE('',*,*,#45697,.F.) ;
#65573=ORIENTED_EDGE('',*,*,#47541,.F.) ;
#65574=ORIENTED_EDGE('',*,*,#44512,.F.) ;
#65575=ORIENTED_EDGE('',*,*,#45470,.F.) ;
#65576=ORIENTED_EDGE('',*,*,#47537,.T.) ;
#65577=ORIENTED_EDGE('',*,*,#47542,.F.) ;
#65578=ORIENTED_EDGE('',*,*,#47543,.F.) ;
#65579=ORIENTED_EDGE('',*,*,#47539,.T.) ;
#65580=ORIENTED_EDGE('',*,*,#45474,.F.) ;
#65581=ORIENTED_EDGE('',*,*,#47544,.F.) ;
#65582=ORIENTED_EDGE('',*,*,#45687,.F.) ;
#65583=ORIENTED_EDGE('',*,*,#47545,.F.) ;
#65584=ORIENTED_EDGE('',*,*,#45688,.F.) ;
#65585=ORIENTED_EDGE('',*,*,#47546,.F.) ;
#65586=ORIENTED_EDGE('',*,*,#45682,.F.) ;
#65587=ORIENTED_EDGE('',*,*,#44177,.T.) ;
#65588=ORIENTED_EDGE('',*,*,#47545,.T.) ;
#65589=ORIENTED_EDGE('',*,*,#47547,.F.) ;
#65590=ORIENTED_EDGE('',*,*,#44412,.T.) ;
#65591=ORIENTED_EDGE('',*,*,#47541,.T.) ;
#65592=ORIENTED_EDGE('',*,*,#47540,.T.) ;
#65593=ORIENTED_EDGE('',*,*,#47548,.F.) ;
#65594=ORIENTED_EDGE('',*,*,#47549,.F.) ;
#65595=ORIENTED_EDGE('',*,*,#44615,.F.) ;
#65596=ORIENTED_EDGE('',*,*,#47550,.F.) ;
#65597=ORIENTED_EDGE('',*,*,#47551,.F.) ;
#65598=ORIENTED_EDGE('',*,*,#47542,.T.) ;
#65599=ORIENTED_EDGE('',*,*,#44515,.F.) ;
#65600=ORIENTED_EDGE('',*,*,#47550,.T.) ;
#65601=ORIENTED_EDGE('',*,*,#44713,.F.) ;
#65602=ORIENTED_EDGE('',*,*,#47543,.T.) ;
#65603=ORIENTED_EDGE('',*,*,#47552,.F.) ;
#65604=ORIENTED_EDGE('',*,*,#47553,.F.) ;
#65605=ORIENTED_EDGE('',*,*,#47546,.T.) ;
#65606=ORIENTED_EDGE('',*,*,#47544,.T.) ;
#65607=ORIENTED_EDGE('',*,*,#47554,.F.) ;
#65608=ORIENTED_EDGE('',*,*,#47547,.T.) ;
#65609=ORIENTED_EDGE('',*,*,#45685,.F.) ;
#65610=ORIENTED_EDGE('',*,*,#47555,.F.) ;
#65611=ORIENTED_EDGE('',*,*,#44413,.F.) ;
#65612=ORIENTED_EDGE('',*,*,#47548,.T.) ;
#65613=ORIENTED_EDGE('',*,*,#44416,.F.) ;
#65614=ORIENTED_EDGE('',*,*,#47556,.F.) ;
#65615=ORIENTED_EDGE('',*,*,#44513,.F.) ;
#65616=ORIENTED_EDGE('',*,*,#47549,.T.) ;
#65617=ORIENTED_EDGE('',*,*,#44514,.F.) ;
#65618=ORIENTED_EDGE('',*,*,#47557,.F.) ;
#65619=ORIENTED_EDGE('',*,*,#44696,.F.) ;
#65620=ORIENTED_EDGE('',*,*,#47551,.T.) ;
#65621=ORIENTED_EDGE('',*,*,#44712,.T.) ;
#65622=ORIENTED_EDGE('',*,*,#47558,.F.) ;
#65623=ORIENTED_EDGE('',*,*,#47552,.T.) ;
#65624=ORIENTED_EDGE('',*,*,#45471,.F.) ;
#65625=ORIENTED_EDGE('',*,*,#47553,.T.) ;
#65626=ORIENTED_EDGE('',*,*,#47559,.F.) ;
#65627=ORIENTED_EDGE('',*,*,#47560,.F.) ;
#65628=ORIENTED_EDGE('',*,*,#47554,.T.) ;
#65629=ORIENTED_EDGE('',*,*,#45473,.F.) ;
#65630=ORIENTED_EDGE('',*,*,#47561,.F.) ;
#65631=ORIENTED_EDGE('',*,*,#45683,.F.) ;
#65632=ORIENTED_EDGE('',*,*,#47562,.F.) ;
#65633=ORIENTED_EDGE('',*,*,#45684,.F.) ;
#65634=ORIENTED_EDGE('',*,*,#47563,.F.) ;
#65635=ORIENTED_EDGE('',*,*,#44510,.F.) ;
#65636=ORIENTED_EDGE('',*,*,#47555,.T.) ;
#65637=ORIENTED_EDGE('',*,*,#47562,.T.) ;
#65638=ORIENTED_EDGE('',*,*,#47564,.F.) ;
#65639=ORIENTED_EDGE('',*,*,#47557,.T.) ;
#65640=ORIENTED_EDGE('',*,*,#47556,.T.) ;
#65641=ORIENTED_EDGE('',*,*,#47565,.F.) ;
#65642=ORIENTED_EDGE('',*,*,#44697,.T.) ;
#65643=ORIENTED_EDGE('',*,*,#47566,.F.) ;
#65644=ORIENTED_EDGE('',*,*,#47559,.T.) ;
#65645=ORIENTED_EDGE('',*,*,#47558,.T.) ;
#65646=ORIENTED_EDGE('',*,*,#44711,.F.) ;
#65647=ORIENTED_EDGE('',*,*,#47560,.T.) ;
#65648=ORIENTED_EDGE('',*,*,#47567,.F.) ;
#65649=ORIENTED_EDGE('',*,*,#47568,.F.) ;
#65650=ORIENTED_EDGE('',*,*,#47563,.T.) ;
#65651=ORIENTED_EDGE('',*,*,#47561,.T.) ;
#65652=ORIENTED_EDGE('',*,*,#47569,.F.) ;
#65653=ORIENTED_EDGE('',*,*,#44506,.T.) ;
#65654=ORIENTED_EDGE('',*,*,#47564,.T.) ;
#65655=ORIENTED_EDGE('',*,*,#44509,.F.) ;
#65656=ORIENTED_EDGE('',*,*,#47570,.F.) ;
#65657=ORIENTED_EDGE('',*,*,#44414,.F.) ;
#65658=ORIENTED_EDGE('',*,*,#47565,.T.) ;
#65659=ORIENTED_EDGE('',*,*,#44415,.F.) ;
#65660=ORIENTED_EDGE('',*,*,#47571,.F.) ;
#65661=ORIENTED_EDGE('',*,*,#44698,.F.) ;
#65662=ORIENTED_EDGE('',*,*,#47566,.T.) ;
#65663=ORIENTED_EDGE('',*,*,#44710,.T.) ;
#65664=ORIENTED_EDGE('',*,*,#47572,.F.) ;
#65665=ORIENTED_EDGE('',*,*,#47567,.T.) ;
#65666=ORIENTED_EDGE('',*,*,#45472,.F.) ;
#65667=ORIENTED_EDGE('',*,*,#47568,.T.) ;
#65668=ORIENTED_EDGE('',*,*,#47573,.F.) ;
#65669=ORIENTED_EDGE('',*,*,#47569,.T.) ;
#65670=ORIENTED_EDGE('',*,*,#47571,.T.) ;
#65671=ORIENTED_EDGE('',*,*,#47570,.T.) ;
#65672=ORIENTED_EDGE('',*,*,#47574,.F.) ;
#65673=ORIENTED_EDGE('',*,*,#44699,.T.) ;
#65674=ORIENTED_EDGE('',*,*,#47572,.T.) ;
#65675=ORIENTED_EDGE('',*,*,#44709,.F.) ;
#65676=ORIENTED_EDGE('',*,*,#47575,.F.) ;
#65677=ORIENTED_EDGE('',*,*,#44507,.F.) ;
#65678=ORIENTED_EDGE('',*,*,#47573,.T.) ;
#65679=ORIENTED_EDGE('',*,*,#47574,.T.) ;
#65680=ORIENTED_EDGE('',*,*,#44508,.F.) ;
#65681=ORIENTED_EDGE('',*,*,#47576,.F.) ;
#65682=ORIENTED_EDGE('',*,*,#44700,.F.) ;
#65683=ORIENTED_EDGE('',*,*,#47575,.T.) ;
#65684=ORIENTED_EDGE('',*,*,#44621,.F.) ;
#65685=ORIENTED_EDGE('',*,*,#47576,.T.) ;
#65686=ORIENTED_EDGE('',*,*,#47577,.F.) ;
#65687=ORIENTED_EDGE('',*,*,#45858,.F.) ;
#65688=ORIENTED_EDGE('',*,*,#47578,.F.) ;
#65689=ORIENTED_EDGE('',*,*,#45905,.F.) ;
#65690=ORIENTED_EDGE('',*,*,#47578,.T.) ;
#65691=ORIENTED_EDGE('',*,*,#45855,.F.) ;
#65692=ORIENTED_EDGE('',*,*,#47579,.F.) ;
#65693=ORIENTED_EDGE('',*,*,#45906,.F.) ;
#65694=ORIENTED_EDGE('',*,*,#45861,.F.) ;
#65695=ORIENTED_EDGE('',*,*,#47577,.T.) ;
#65696=ORIENTED_EDGE('',*,*,#47580,.F.) ;
#65697=ORIENTED_EDGE('',*,*,#47579,.T.) ;
#65698=ORIENTED_EDGE('',*,*,#45852,.F.) ;
#65699=ORIENTED_EDGE('',*,*,#47581,.F.) ;
#65700=ORIENTED_EDGE('',*,*,#45907,.F.) ;
#65701=ORIENTED_EDGE('',*,*,#47580,.T.) ;
#65702=ORIENTED_EDGE('',*,*,#45904,.F.) ;
#65703=ORIENTED_EDGE('',*,*,#47582,.F.) ;
#65704=ORIENTED_EDGE('',*,*,#45864,.F.) ;
#65705=ORIENTED_EDGE('',*,*,#47581,.T.) ;
#65706=ORIENTED_EDGE('',*,*,#45849,.F.) ;
#65707=ORIENTED_EDGE('',*,*,#47583,.F.) ;
#65708=ORIENTED_EDGE('',*,*,#45908,.F.) ;
#65709=ORIENTED_EDGE('',*,*,#45867,.F.) ;
#65710=ORIENTED_EDGE('',*,*,#47582,.T.) ;
#65711=ORIENTED_EDGE('',*,*,#47584,.F.) ;
#65712=ORIENTED_EDGE('',*,*,#47583,.T.) ;
#65713=ORIENTED_EDGE('',*,*,#45846,.F.) ;
#65714=ORIENTED_EDGE('',*,*,#47585,.F.) ;
#65715=ORIENTED_EDGE('',*,*,#45909,.F.) ;
#65716=ORIENTED_EDGE('',*,*,#47584,.T.) ;
#65717=ORIENTED_EDGE('',*,*,#45903,.F.) ;
#65718=ORIENTED_EDGE('',*,*,#47586,.F.) ;
#65719=ORIENTED_EDGE('',*,*,#45870,.F.) ;
#65720=ORIENTED_EDGE('',*,*,#47585,.T.) ;
#65721=ORIENTED_EDGE('',*,*,#45843,.F.) ;
#65722=ORIENTED_EDGE('',*,*,#47587,.F.) ;
#65723=ORIENTED_EDGE('',*,*,#45873,.F.) ;
#65724=ORIENTED_EDGE('',*,*,#47586,.T.) ;
#65725=ORIENTED_EDGE('',*,*,#47588,.F.) ;
#65726=ORIENTED_EDGE('',*,*,#47587,.T.) ;
#65727=ORIENTED_EDGE('',*,*,#45840,.F.) ;
#65728=ORIENTED_EDGE('',*,*,#47589,.F.) ;
#65729=ORIENTED_EDGE('',*,*,#45910,.F.) ;
#65730=ORIENTED_EDGE('',*,*,#47588,.T.) ;
#65731=ORIENTED_EDGE('',*,*,#45902,.F.) ;
#65732=ORIENTED_EDGE('',*,*,#47590,.F.) ;
#65733=ORIENTED_EDGE('',*,*,#45876,.F.) ;
#65734=ORIENTED_EDGE('',*,*,#47589,.T.) ;
#65735=ORIENTED_EDGE('',*,*,#44366,.F.) ;
#65736=ORIENTED_EDGE('',*,*,#47591,.F.) ;
#65737=ORIENTED_EDGE('',*,*,#45879,.F.) ;
#65738=ORIENTED_EDGE('',*,*,#47590,.T.) ;
#65739=ORIENTED_EDGE('',*,*,#47592,.F.) ;
#65740=ORIENTED_EDGE('',*,*,#47591,.T.) ;
#65741=ORIENTED_EDGE('',*,*,#45838,.F.) ;
#65742=ORIENTED_EDGE('',*,*,#44173,.F.) ;
#65743=ORIENTED_EDGE('',*,*,#45911,.F.) ;
#65744=ORIENTED_EDGE('',*,*,#47592,.T.) ;
#65745=ORIENTED_EDGE('',*,*,#45901,.F.) ;
#65746=ORIENTED_EDGE('',*,*,#47593,.F.) ;
#65747=ORIENTED_EDGE('',*,*,#45882,.F.) ;
#65748=ORIENTED_EDGE('',*,*,#45885,.F.) ;
#65749=ORIENTED_EDGE('',*,*,#47593,.T.) ;
#65750=ORIENTED_EDGE('',*,*,#47594,.F.) ;
#65751=ORIENTED_EDGE('',*,*,#44172,.T.) ;
#65752=ORIENTED_EDGE('',*,*,#45833,.F.) ;
#65753=ORIENTED_EDGE('',*,*,#47595,.F.) ;
#65754=ORIENTED_EDGE('',*,*,#45912,.F.) ;
#65755=ORIENTED_EDGE('',*,*,#47594,.T.) ;
#65756=ORIENTED_EDGE('',*,*,#45900,.F.) ;
#65757=ORIENTED_EDGE('',*,*,#47596,.F.) ;
#65758=ORIENTED_EDGE('',*,*,#45888,.F.) ;
#65759=ORIENTED_EDGE('',*,*,#47595,.T.) ;
#65760=ORIENTED_EDGE('',*,*,#45830,.F.) ;
#65761=ORIENTED_EDGE('',*,*,#47597,.F.) ;
#65762=ORIENTED_EDGE('',*,*,#45891,.F.) ;
#65763=ORIENTED_EDGE('',*,*,#47596,.T.) ;
#65764=ORIENTED_EDGE('',*,*,#47598,.F.) ;
#65765=ORIENTED_EDGE('',*,*,#47597,.T.) ;
#65766=ORIENTED_EDGE('',*,*,#45827,.F.) ;
#65767=ORIENTED_EDGE('',*,*,#47599,.F.) ;
#65768=ORIENTED_EDGE('',*,*,#45913,.F.) ;
#65769=ORIENTED_EDGE('',*,*,#47598,.T.) ;
#65770=ORIENTED_EDGE('',*,*,#45899,.F.) ;
#65771=ORIENTED_EDGE('',*,*,#47600,.F.) ;
#65772=ORIENTED_EDGE('',*,*,#45894,.F.) ;
#65773=ORIENTED_EDGE('',*,*,#47599,.T.) ;
#65774=ORIENTED_EDGE('',*,*,#45824,.F.) ;
#65775=ORIENTED_EDGE('',*,*,#47601,.F.) ;
#65776=ORIENTED_EDGE('',*,*,#45896,.F.) ;
#65777=ORIENTED_EDGE('',*,*,#47600,.T.) ;
#65778=ORIENTED_EDGE('',*,*,#45898,.F.) ;
#65779=ORIENTED_EDGE('',*,*,#47602,.F.) ;
#65780=ORIENTED_EDGE('',*,*,#45818,.F.) ;
#65781=ORIENTED_EDGE('',*,*,#47601,.T.) ;
#65782=ORIENTED_EDGE('',*,*,#45821,.F.) ;
#65783=ORIENTED_EDGE('',*,*,#47602,.T.) ;
#65784=ORIENTED_EDGE('',*,*,#45897,.F.) ;
#65785=ORIENTED_EDGE('',*,*,#47603,.F.) ;
#65786=ORIENTED_EDGE('',*,*,#45713,.F.) ;
#65787=ORIENTED_EDGE('',*,*,#47604,.F.) ;
#65788=ORIENTED_EDGE('',*,*,#45468,.F.) ;
#65789=ORIENTED_EDGE('',*,*,#47605,.F.) ;
#65790=ORIENTED_EDGE('',*,*,#45714,.F.) ;
#65791=ORIENTED_EDGE('',*,*,#47606,.F.) ;
#65792=ORIENTED_EDGE('',*,*,#45708,.F.) ;
#65793=ORIENTED_EDGE('',*,*,#47607,.F.) ;
#65794=ORIENTED_EDGE('',*,*,#47605,.T.) ;
#65795=ORIENTED_EDGE('',*,*,#47608,.F.) ;
#65796=ORIENTED_EDGE('',*,*,#47609,.F.) ;
#65797=ORIENTED_EDGE('',*,*,#47604,.T.) ;
#65798=ORIENTED_EDGE('',*,*,#47610,.F.) ;
#65799=ORIENTED_EDGE('',*,*,#47603,.T.) ;
#65800=ORIENTED_EDGE('',*,*,#45467,.T.) ;
#65801=ORIENTED_EDGE('',*,*,#47611,.F.) ;
#65802=ORIENTED_EDGE('',*,*,#47606,.T.) ;
#65803=ORIENTED_EDGE('',*,*,#47608,.T.) ;
#65804=ORIENTED_EDGE('',*,*,#45711,.F.) ;
#65805=ORIENTED_EDGE('',*,*,#47612,.F.) ;
#65806=ORIENTED_EDGE('',*,*,#44157,.T.) ;
#65807=ORIENTED_EDGE('',*,*,#47613,.T.) ;
#65808=ORIENTED_EDGE('',*,*,#47614,.F.) ;
#65809=ORIENTED_EDGE('',*,*,#47607,.T.) ;
#65810=ORIENTED_EDGE('',*,*,#47615,.F.) ;
#65811=ORIENTED_EDGE('',*,*,#47616,.T.) ;
#65812=ORIENTED_EDGE('',*,*,#47617,.F.) ;
#65813=ORIENTED_EDGE('',*,*,#44397,.F.) ;
#65814=ORIENTED_EDGE('',*,*,#47618,.F.) ;
#65815=ORIENTED_EDGE('',*,*,#45715,.F.) ;
#65816=ORIENTED_EDGE('',*,*,#47610,.T.) ;
#65817=ORIENTED_EDGE('',*,*,#45712,.F.) ;
#65818=ORIENTED_EDGE('',*,*,#47619,.F.) ;
#65819=ORIENTED_EDGE('',*,*,#45718,.F.) ;
#65820=ORIENTED_EDGE('',*,*,#47609,.T.) ;
#65821=ORIENTED_EDGE('',*,*,#45717,.F.) ;
#65822=ORIENTED_EDGE('',*,*,#47620,.F.) ;
#65823=ORIENTED_EDGE('',*,*,#45459,.F.) ;
#65824=ORIENTED_EDGE('',*,*,#47611,.T.) ;
#65825=ORIENTED_EDGE('',*,*,#45466,.F.) ;
#65826=ORIENTED_EDGE('',*,*,#47621,.F.) ;
#65827=ORIENTED_EDGE('',*,*,#45709,.F.) ;
#65828=ORIENTED_EDGE('',*,*,#47622,.F.) ;
#65829=ORIENTED_EDGE('',*,*,#45710,.F.) ;
#65830=ORIENTED_EDGE('',*,*,#47623,.F.) ;
#65831=ORIENTED_EDGE('',*,*,#45705,.F.) ;
#65832=ORIENTED_EDGE('',*,*,#47612,.T.) ;
#65833=ORIENTED_EDGE('',*,*,#47622,.T.) ;
#65834=ORIENTED_EDGE('',*,*,#44158,.F.) ;
#65835=ORIENTED_EDGE('',*,*,#47618,.T.) ;
#65836=ORIENTED_EDGE('',*,*,#44407,.T.) ;
#65837=ORIENTED_EDGE('',*,*,#47624,.F.) ;
#65838=ORIENTED_EDGE('',*,*,#47619,.T.) ;
#65839=ORIENTED_EDGE('',*,*,#47625,.F.) ;
#65840=ORIENTED_EDGE('',*,*,#47620,.T.) ;
#65841=ORIENTED_EDGE('',*,*,#47626,.F.) ;
#65842=ORIENTED_EDGE('',*,*,#44501,.T.) ;
#65843=ORIENTED_EDGE('',*,*,#47621,.T.) ;
#65844=ORIENTED_EDGE('',*,*,#45465,.T.) ;
#65845=ORIENTED_EDGE('',*,*,#47627,.F.) ;
#65846=ORIENTED_EDGE('',*,*,#47623,.T.) ;
#65847=ORIENTED_EDGE('',*,*,#47624,.T.) ;
#65848=ORIENTED_EDGE('',*,*,#44406,.F.) ;
#65849=ORIENTED_EDGE('',*,*,#47628,.F.) ;
#65850=ORIENTED_EDGE('',*,*,#45719,.F.) ;
#65851=ORIENTED_EDGE('',*,*,#47626,.T.) ;
#65852=ORIENTED_EDGE('',*,*,#45716,.F.) ;
#65853=ORIENTED_EDGE('',*,*,#47629,.F.) ;
#65854=ORIENTED_EDGE('',*,*,#44502,.F.) ;
#65855=ORIENTED_EDGE('',*,*,#45460,.F.) ;
#65856=ORIENTED_EDGE('',*,*,#47625,.T.) ;
#65857=ORIENTED_EDGE('',*,*,#47630,.F.) ;
#65858=ORIENTED_EDGE('',*,*,#47631,.F.) ;
#65859=ORIENTED_EDGE('',*,*,#47627,.T.) ;
#65860=ORIENTED_EDGE('',*,*,#45464,.F.) ;
#65861=ORIENTED_EDGE('',*,*,#47632,.F.) ;
#65862=ORIENTED_EDGE('',*,*,#45706,.F.) ;
#65863=ORIENTED_EDGE('',*,*,#47633,.F.) ;
#65864=ORIENTED_EDGE('',*,*,#45707,.F.) ;
#65865=ORIENTED_EDGE('',*,*,#47634,.F.) ;
#65866=ORIENTED_EDGE('',*,*,#45701,.F.) ;
#65867=ORIENTED_EDGE('',*,*,#44160,.T.) ;
#65868=ORIENTED_EDGE('',*,*,#47633,.T.) ;
#65869=ORIENTED_EDGE('',*,*,#47635,.F.) ;
#65870=ORIENTED_EDGE('',*,*,#44401,.T.) ;
#65871=ORIENTED_EDGE('',*,*,#47629,.T.) ;
#65872=ORIENTED_EDGE('',*,*,#47628,.T.) ;
#65873=ORIENTED_EDGE('',*,*,#47636,.F.) ;
#65874=ORIENTED_EDGE('',*,*,#47637,.F.) ;
#65875=ORIENTED_EDGE('',*,*,#44619,.F.) ;
#65876=ORIENTED_EDGE('',*,*,#47638,.F.) ;
#65877=ORIENTED_EDGE('',*,*,#47639,.F.) ;
#65878=ORIENTED_EDGE('',*,*,#47630,.T.) ;
#65879=ORIENTED_EDGE('',*,*,#44505,.F.) ;
#65880=ORIENTED_EDGE('',*,*,#47638,.T.) ;
#65881=ORIENTED_EDGE('',*,*,#44708,.F.) ;
#65882=ORIENTED_EDGE('',*,*,#47631,.T.) ;
#65883=ORIENTED_EDGE('',*,*,#47640,.F.) ;
#65884=ORIENTED_EDGE('',*,*,#47641,.F.) ;
#65885=ORIENTED_EDGE('',*,*,#47634,.T.) ;
#65886=ORIENTED_EDGE('',*,*,#47632,.T.) ;
#65887=ORIENTED_EDGE('',*,*,#47642,.F.) ;
#65888=ORIENTED_EDGE('',*,*,#47635,.T.) ;
#65889=ORIENTED_EDGE('',*,*,#45704,.F.) ;
#65890=ORIENTED_EDGE('',*,*,#47643,.F.) ;
#65891=ORIENTED_EDGE('',*,*,#44402,.F.) ;
#65892=ORIENTED_EDGE('',*,*,#47636,.T.) ;
#65893=ORIENTED_EDGE('',*,*,#44405,.F.) ;
#65894=ORIENTED_EDGE('',*,*,#47644,.F.) ;
#65895=ORIENTED_EDGE('',*,*,#44503,.F.) ;
#65896=ORIENTED_EDGE('',*,*,#47637,.T.) ;
#65897=ORIENTED_EDGE('',*,*,#44504,.F.) ;
#65898=ORIENTED_EDGE('',*,*,#47645,.F.) ;
#65899=ORIENTED_EDGE('',*,*,#44701,.F.) ;
#65900=ORIENTED_EDGE('',*,*,#47639,.T.) ;
#65901=ORIENTED_EDGE('',*,*,#44707,.T.) ;
#65902=ORIENTED_EDGE('',*,*,#47646,.F.) ;
#65903=ORIENTED_EDGE('',*,*,#47640,.T.) ;
#65904=ORIENTED_EDGE('',*,*,#45461,.F.) ;
#65905=ORIENTED_EDGE('',*,*,#47641,.T.) ;
#65906=ORIENTED_EDGE('',*,*,#47647,.F.) ;
#65907=ORIENTED_EDGE('',*,*,#47648,.F.) ;
#65908=ORIENTED_EDGE('',*,*,#47642,.T.) ;
#65909=ORIENTED_EDGE('',*,*,#45463,.F.) ;
#65910=ORIENTED_EDGE('',*,*,#47649,.F.) ;
#65911=ORIENTED_EDGE('',*,*,#45702,.F.) ;
#65912=ORIENTED_EDGE('',*,*,#47650,.F.) ;
#65913=ORIENTED_EDGE('',*,*,#45703,.F.) ;
#65914=ORIENTED_EDGE('',*,*,#47651,.F.) ;
#65915=ORIENTED_EDGE('',*,*,#44500,.F.) ;
#65916=ORIENTED_EDGE('',*,*,#47643,.T.) ;
#65917=ORIENTED_EDGE('',*,*,#47650,.T.) ;
#65918=ORIENTED_EDGE('',*,*,#47652,.F.) ;
#65919=ORIENTED_EDGE('',*,*,#47645,.T.) ;
#65920=ORIENTED_EDGE('',*,*,#47644,.T.) ;
#65921=ORIENTED_EDGE('',*,*,#47653,.F.) ;
#65922=ORIENTED_EDGE('',*,*,#44702,.T.) ;
#65923=ORIENTED_EDGE('',*,*,#47654,.F.) ;
#65924=ORIENTED_EDGE('',*,*,#47647,.T.) ;
#65925=ORIENTED_EDGE('',*,*,#47646,.T.) ;
#65926=ORIENTED_EDGE('',*,*,#44759,.F.) ;
#65927=ORIENTED_EDGE('',*,*,#47648,.T.) ;
#65928=ORIENTED_EDGE('',*,*,#47655,.F.) ;
#65929=ORIENTED_EDGE('',*,*,#47656,.F.) ;
#65930=ORIENTED_EDGE('',*,*,#47651,.T.) ;
#65931=ORIENTED_EDGE('',*,*,#47649,.T.) ;
#65932=ORIENTED_EDGE('',*,*,#47657,.F.) ;
#65933=ORIENTED_EDGE('',*,*,#44496,.T.) ;
#65934=ORIENTED_EDGE('',*,*,#47652,.T.) ;
#65935=ORIENTED_EDGE('',*,*,#44499,.F.) ;
#65936=ORIENTED_EDGE('',*,*,#47658,.F.) ;
#65937=ORIENTED_EDGE('',*,*,#44403,.F.) ;
#65938=ORIENTED_EDGE('',*,*,#47653,.T.) ;
#65939=ORIENTED_EDGE('',*,*,#44404,.F.) ;
#65940=ORIENTED_EDGE('',*,*,#47659,.F.) ;
#65941=ORIENTED_EDGE('',*,*,#44703,.F.) ;
#65942=ORIENTED_EDGE('',*,*,#47654,.T.) ;
#65943=ORIENTED_EDGE('',*,*,#44758,.T.) ;
#65944=ORIENTED_EDGE('',*,*,#47660,.F.) ;
#65945=ORIENTED_EDGE('',*,*,#47655,.T.) ;
#65946=ORIENTED_EDGE('',*,*,#45462,.F.) ;
#65947=ORIENTED_EDGE('',*,*,#47656,.T.) ;
#65948=ORIENTED_EDGE('',*,*,#47661,.F.) ;
#65949=ORIENTED_EDGE('',*,*,#47657,.T.) ;
#65950=ORIENTED_EDGE('',*,*,#47659,.T.) ;
#65951=ORIENTED_EDGE('',*,*,#47658,.T.) ;
#65952=ORIENTED_EDGE('',*,*,#47662,.F.) ;
#65953=ORIENTED_EDGE('',*,*,#44651,.T.) ;
#65954=ORIENTED_EDGE('',*,*,#47660,.T.) ;
#65955=ORIENTED_EDGE('',*,*,#44757,.F.) ;
#65956=ORIENTED_EDGE('',*,*,#47663,.F.) ;
#65957=ORIENTED_EDGE('',*,*,#44497,.F.) ;
#65958=ORIENTED_EDGE('',*,*,#47661,.T.) ;
#65959=ORIENTED_EDGE('',*,*,#47662,.T.) ;
#65960=ORIENTED_EDGE('',*,*,#44498,.F.) ;
#65961=ORIENTED_EDGE('',*,*,#47664,.F.) ;
#65962=ORIENTED_EDGE('',*,*,#44652,.F.) ;
#65963=ORIENTED_EDGE('',*,*,#47663,.T.) ;
#65964=ORIENTED_EDGE('',*,*,#44704,.F.) ;
#65965=ORIENTED_EDGE('',*,*,#47664,.T.) ;
#65966=ORIENTED_EDGE('',*,*,#47665,.F.) ;
#65967=ORIENTED_EDGE('',*,*,#45761,.F.) ;
#65968=ORIENTED_EDGE('',*,*,#47666,.F.) ;
#65969=ORIENTED_EDGE('',*,*,#45808,.F.) ;
#65970=ORIENTED_EDGE('',*,*,#47666,.T.) ;
#65971=ORIENTED_EDGE('',*,*,#45758,.F.) ;
#65972=ORIENTED_EDGE('',*,*,#47667,.F.) ;
#65973=ORIENTED_EDGE('',*,*,#45809,.F.) ;
#65974=ORIENTED_EDGE('',*,*,#45764,.F.) ;
#65975=ORIENTED_EDGE('',*,*,#47665,.T.) ;
#65976=ORIENTED_EDGE('',*,*,#47668,.F.) ;
#65977=ORIENTED_EDGE('',*,*,#47667,.T.) ;
#65978=ORIENTED_EDGE('',*,*,#45755,.F.) ;
#65979=ORIENTED_EDGE('',*,*,#47669,.F.) ;
#65980=ORIENTED_EDGE('',*,*,#45810,.F.) ;
#65981=ORIENTED_EDGE('',*,*,#47668,.T.) ;
#65982=ORIENTED_EDGE('',*,*,#45807,.F.) ;
#65983=ORIENTED_EDGE('',*,*,#47670,.F.) ;
#65984=ORIENTED_EDGE('',*,*,#45767,.F.) ;
#65985=ORIENTED_EDGE('',*,*,#47669,.T.) ;
#65986=ORIENTED_EDGE('',*,*,#45752,.F.) ;
#65987=ORIENTED_EDGE('',*,*,#47671,.F.) ;
#65988=ORIENTED_EDGE('',*,*,#45811,.F.) ;
#65989=ORIENTED_EDGE('',*,*,#45770,.F.) ;
#65990=ORIENTED_EDGE('',*,*,#47670,.T.) ;
#65991=ORIENTED_EDGE('',*,*,#47672,.F.) ;
#65992=ORIENTED_EDGE('',*,*,#47671,.T.) ;
#65993=ORIENTED_EDGE('',*,*,#45749,.F.) ;
#65994=ORIENTED_EDGE('',*,*,#47673,.F.) ;
#65995=ORIENTED_EDGE('',*,*,#45812,.F.) ;
#65996=ORIENTED_EDGE('',*,*,#47672,.T.) ;
#65997=ORIENTED_EDGE('',*,*,#45806,.F.) ;
#65998=ORIENTED_EDGE('',*,*,#47674,.F.) ;
#65999=ORIENTED_EDGE('',*,*,#45773,.F.) ;
#66000=ORIENTED_EDGE('',*,*,#47673,.T.) ;
#66001=ORIENTED_EDGE('',*,*,#45746,.F.) ;
#66002=ORIENTED_EDGE('',*,*,#47675,.F.) ;
#66003=ORIENTED_EDGE('',*,*,#45776,.F.) ;
#66004=ORIENTED_EDGE('',*,*,#47674,.T.) ;
#66005=ORIENTED_EDGE('',*,*,#47676,.F.) ;
#66006=ORIENTED_EDGE('',*,*,#47675,.T.) ;
#66007=ORIENTED_EDGE('',*,*,#45743,.F.) ;
#66008=ORIENTED_EDGE('',*,*,#47677,.F.) ;
#66009=ORIENTED_EDGE('',*,*,#45813,.F.) ;
#66010=ORIENTED_EDGE('',*,*,#47676,.T.) ;
#66011=ORIENTED_EDGE('',*,*,#45805,.F.) ;
#66012=ORIENTED_EDGE('',*,*,#47678,.F.) ;
#66013=ORIENTED_EDGE('',*,*,#45779,.F.) ;
#66014=ORIENTED_EDGE('',*,*,#47677,.T.) ;
#66015=ORIENTED_EDGE('',*,*,#44369,.F.) ;
#66016=ORIENTED_EDGE('',*,*,#47679,.F.) ;
#66017=ORIENTED_EDGE('',*,*,#45782,.F.) ;
#66018=ORIENTED_EDGE('',*,*,#47678,.T.) ;
#66019=ORIENTED_EDGE('',*,*,#47680,.F.) ;
#66020=ORIENTED_EDGE('',*,*,#47679,.T.) ;
#66021=ORIENTED_EDGE('',*,*,#45741,.F.) ;
#66022=ORIENTED_EDGE('',*,*,#44156,.F.) ;
#66023=ORIENTED_EDGE('',*,*,#45814,.F.) ;
#66024=ORIENTED_EDGE('',*,*,#47680,.T.) ;
#66025=ORIENTED_EDGE('',*,*,#45804,.F.) ;
#66026=ORIENTED_EDGE('',*,*,#47681,.F.) ;
#66027=ORIENTED_EDGE('',*,*,#45785,.F.) ;
#66028=ORIENTED_EDGE('',*,*,#45788,.F.) ;
#66029=ORIENTED_EDGE('',*,*,#47681,.T.) ;
#66030=ORIENTED_EDGE('',*,*,#47682,.F.) ;
#66031=ORIENTED_EDGE('',*,*,#44155,.T.) ;
#66032=ORIENTED_EDGE('',*,*,#45736,.F.) ;
#66033=ORIENTED_EDGE('',*,*,#47683,.F.) ;
#66034=ORIENTED_EDGE('',*,*,#45815,.F.) ;
#66035=ORIENTED_EDGE('',*,*,#47682,.T.) ;
#66036=ORIENTED_EDGE('',*,*,#45803,.F.) ;
#66037=ORIENTED_EDGE('',*,*,#47684,.F.) ;
#66038=ORIENTED_EDGE('',*,*,#45791,.F.) ;
#66039=ORIENTED_EDGE('',*,*,#47683,.T.) ;
#66040=ORIENTED_EDGE('',*,*,#45733,.F.) ;
#66041=ORIENTED_EDGE('',*,*,#47685,.F.) ;
#66042=ORIENTED_EDGE('',*,*,#45794,.F.) ;
#66043=ORIENTED_EDGE('',*,*,#47684,.T.) ;
#66044=ORIENTED_EDGE('',*,*,#47686,.F.) ;
#66045=ORIENTED_EDGE('',*,*,#47685,.T.) ;
#66046=ORIENTED_EDGE('',*,*,#45730,.F.) ;
#66047=ORIENTED_EDGE('',*,*,#47687,.F.) ;
#66048=ORIENTED_EDGE('',*,*,#45816,.F.) ;
#66049=ORIENTED_EDGE('',*,*,#47686,.T.) ;
#66050=ORIENTED_EDGE('',*,*,#45802,.F.) ;
#66051=ORIENTED_EDGE('',*,*,#47688,.F.) ;
#66052=ORIENTED_EDGE('',*,*,#45797,.F.) ;
#66053=ORIENTED_EDGE('',*,*,#47687,.T.) ;
#66054=ORIENTED_EDGE('',*,*,#45727,.F.) ;
#66055=ORIENTED_EDGE('',*,*,#47689,.F.) ;
#66056=ORIENTED_EDGE('',*,*,#45799,.F.) ;
#66057=ORIENTED_EDGE('',*,*,#47688,.T.) ;
#66058=ORIENTED_EDGE('',*,*,#45801,.F.) ;
#66059=ORIENTED_EDGE('',*,*,#47690,.F.) ;
#66060=ORIENTED_EDGE('',*,*,#45721,.F.) ;
#66061=ORIENTED_EDGE('',*,*,#47689,.T.) ;
#66062=ORIENTED_EDGE('',*,*,#45724,.F.) ;
#66063=ORIENTED_EDGE('',*,*,#47690,.T.) ;
#66064=ORIENTED_EDGE('',*,*,#45800,.F.) ;
#66065=ORIENTED_EDGE('',*,*,#47691,.T.) ;
#66066=ORIENTED_EDGE('',*,*,#47692,.T.) ;
#66067=ORIENTED_EDGE('',*,*,#47693,.T.) ;
#66068=ORIENTED_EDGE('',*,*,#47694,.T.) ;
#66069=ORIENTED_EDGE('',*,*,#47695,.T.) ;
#66070=ORIENTED_EDGE('',*,*,#47696,.T.) ;
#66071=ORIENTED_EDGE('',*,*,#47697,.T.) ;
#66072=ORIENTED_EDGE('',*,*,#47698,.T.) ;
#66073=ORIENTED_EDGE('',*,*,#47699,.T.) ;
#66074=ORIENTED_EDGE('',*,*,#47700,.T.) ;
#66075=ORIENTED_EDGE('',*,*,#47701,.T.) ;
#66076=ORIENTED_EDGE('',*,*,#47702,.T.) ;
#66077=ORIENTED_EDGE('',*,*,#47703,.T.) ;
#66078=ORIENTED_EDGE('',*,*,#47704,.T.) ;
#66079=ORIENTED_EDGE('',*,*,#47705,.T.) ;
#66080=ORIENTED_EDGE('',*,*,#47706,.T.) ;
#66081=ORIENTED_EDGE('',*,*,#47707,.T.) ;
#66082=ORIENTED_EDGE('',*,*,#47708,.T.) ;
#66083=ORIENTED_EDGE('',*,*,#47709,.F.) ;
#66084=ORIENTED_EDGE('',*,*,#47710,.T.) ;
#66085=ORIENTED_EDGE('',*,*,#47711,.T.) ;
#66086=ORIENTED_EDGE('',*,*,#47712,.T.) ;
#66087=ORIENTED_EDGE('',*,*,#46679,.T.) ;
#66088=ORIENTED_EDGE('',*,*,#47713,.T.) ;
#66089=ORIENTED_EDGE('',*,*,#47714,.T.) ;
#66090=ORIENTED_EDGE('',*,*,#47715,.T.) ;
#66091=ORIENTED_EDGE('',*,*,#47716,.T.) ;
#66092=ORIENTED_EDGE('',*,*,#47717,.T.) ;
#66093=ORIENTED_EDGE('',*,*,#44334,.T.) ;
#66094=ORIENTED_EDGE('',*,*,#47718,.T.) ;
#66095=ORIENTED_EDGE('',*,*,#47719,.T.) ;
#66096=ORIENTED_EDGE('',*,*,#47720,.T.) ;
#66097=ORIENTED_EDGE('',*,*,#46676,.T.) ;
#66098=ORIENTED_EDGE('',*,*,#47721,.T.) ;
#66099=ORIENTED_EDGE('',*,*,#47691,.F.) ;
#66100=ORIENTED_EDGE('',*,*,#47722,.T.) ;
#66101=ORIENTED_EDGE('',*,*,#46677,.T.) ;
#66102=ORIENTED_EDGE('',*,*,#47709,.T.) ;
#66103=ORIENTED_EDGE('',*,*,#47723,.T.) ;
#66104=ORIENTED_EDGE('',*,*,#44487,.F.) ;
#66105=ORIENTED_EDGE('',*,*,#47724,.T.) ;
#66106=ORIENTED_EDGE('',*,*,#47725,.T.) ;
#66107=ORIENTED_EDGE('',*,*,#47726,.T.) ;
#66108=ORIENTED_EDGE('',*,*,#47727,.T.) ;
#66109=ORIENTED_EDGE('',*,*,#47728,.T.) ;
#66110=ORIENTED_EDGE('',*,*,#47729,.T.) ;
#66111=ORIENTED_EDGE('',*,*,#47730,.T.) ;
#66112=ORIENTED_EDGE('',*,*,#46595,.F.) ;
#66113=ORIENTED_EDGE('',*,*,#47731,.T.) ;
#66114=ORIENTED_EDGE('',*,*,#46599,.F.) ;
#66115=ORIENTED_EDGE('',*,*,#47732,.T.) ;
#66116=ORIENTED_EDGE('',*,*,#47733,.T.) ;
#66117=ORIENTED_EDGE('',*,*,#47734,.T.) ;
#66118=ORIENTED_EDGE('',*,*,#47735,.T.) ;
#66119=ORIENTED_EDGE('',*,*,#47736,.T.) ;
#66120=ORIENTED_EDGE('',*,*,#47737,.T.) ;
#66121=ORIENTED_EDGE('',*,*,#47738,.T.) ;
#66122=ORIENTED_EDGE('',*,*,#47739,.T.) ;
#66123=ORIENTED_EDGE('',*,*,#47740,.T.) ;
#66124=ORIENTED_EDGE('',*,*,#47741,.T.) ;
#66125=ORIENTED_EDGE('',*,*,#47742,.T.) ;
#66126=ORIENTED_EDGE('',*,*,#47743,.T.) ;
#66127=ORIENTED_EDGE('',*,*,#47744,.T.) ;
#66128=ORIENTED_EDGE('',*,*,#46593,.T.) ;
#66129=ORIENTED_EDGE('',*,*,#47745,.T.) ;
#66130=ORIENTED_EDGE('',*,*,#46597,.F.) ;
#66131=ORIENTED_EDGE('',*,*,#47746,.T.) ;
#66132=ORIENTED_EDGE('',*,*,#47747,.T.) ;
#66133=ORIENTED_EDGE('',*,*,#47748,.T.) ;
#66134=ORIENTED_EDGE('',*,*,#47749,.T.) ;
#66135=ORIENTED_EDGE('',*,*,#47750,.T.) ;
#66136=ORIENTED_EDGE('',*,*,#47751,.T.) ;
#66137=ORIENTED_EDGE('',*,*,#47752,.T.) ;
#66138=ORIENTED_EDGE('',*,*,#47753,.T.) ;
#66139=ORIENTED_EDGE('',*,*,#47754,.T.) ;
#66140=ORIENTED_EDGE('',*,*,#47755,.T.) ;
#66141=ORIENTED_EDGE('',*,*,#47756,.T.) ;
#66142=ORIENTED_EDGE('',*,*,#47757,.T.) ;
#66143=ORIENTED_EDGE('',*,*,#47758,.T.) ;
#66144=ORIENTED_EDGE('',*,*,#47759,.T.) ;
#66145=ORIENTED_EDGE('',*,*,#47760,.T.) ;
#66146=ORIENTED_EDGE('',*,*,#47761,.T.) ;
#66147=ORIENTED_EDGE('',*,*,#47762,.T.) ;
#66148=ORIENTED_EDGE('',*,*,#47763,.T.) ;
#66149=ORIENTED_EDGE('',*,*,#47764,.T.) ;
#66150=ORIENTED_EDGE('',*,*,#47765,.T.) ;
#66151=ORIENTED_EDGE('',*,*,#47766,.T.) ;
#66152=ORIENTED_EDGE('',*,*,#47767,.F.) ;
#66153=ORIENTED_EDGE('',*,*,#47768,.T.) ;
#66154=ORIENTED_EDGE('',*,*,#47769,.T.) ;
#66155=ORIENTED_EDGE('',*,*,#47770,.T.) ;
#66156=ORIENTED_EDGE('',*,*,#47001,.T.) ;
#66157=ORIENTED_EDGE('',*,*,#47771,.T.) ;
#66158=ORIENTED_EDGE('',*,*,#47772,.T.) ;
#66159=ORIENTED_EDGE('',*,*,#47773,.T.) ;
#66160=ORIENTED_EDGE('',*,*,#47774,.T.) ;
#66161=ORIENTED_EDGE('',*,*,#47775,.T.) ;
#66162=ORIENTED_EDGE('',*,*,#44281,.T.) ;
#66163=ORIENTED_EDGE('',*,*,#47776,.T.) ;
#66164=ORIENTED_EDGE('',*,*,#47777,.T.) ;
#66165=ORIENTED_EDGE('',*,*,#47778,.T.) ;
#66166=ORIENTED_EDGE('',*,*,#46998,.T.) ;
#66167=ORIENTED_EDGE('',*,*,#47779,.T.) ;
#66168=ORIENTED_EDGE('',*,*,#47749,.F.) ;
#66169=ORIENTED_EDGE('',*,*,#47780,.T.) ;
#66170=ORIENTED_EDGE('',*,*,#46999,.T.) ;
#66171=ORIENTED_EDGE('',*,*,#47767,.T.) ;
#66172=ORIENTED_EDGE('',*,*,#47781,.T.) ;
#66173=ORIENTED_EDGE('',*,*,#44476,.F.) ;
#66174=ORIENTED_EDGE('',*,*,#47782,.T.) ;
#66175=ORIENTED_EDGE('',*,*,#47783,.T.) ;
#66176=ORIENTED_EDGE('',*,*,#47784,.T.) ;
#66177=ORIENTED_EDGE('',*,*,#47785,.T.) ;
#66178=ORIENTED_EDGE('',*,*,#47786,.T.) ;
#66179=ORIENTED_EDGE('',*,*,#47787,.T.) ;
#66180=ORIENTED_EDGE('',*,*,#47788,.T.) ;
#66181=ORIENTED_EDGE('',*,*,#46603,.F.) ;
#66182=ORIENTED_EDGE('',*,*,#47789,.T.) ;
#66183=ORIENTED_EDGE('',*,*,#46607,.F.) ;
#66184=ORIENTED_EDGE('',*,*,#47790,.T.) ;
#66185=ORIENTED_EDGE('',*,*,#47791,.T.) ;
#66186=ORIENTED_EDGE('',*,*,#47792,.T.) ;
#66187=ORIENTED_EDGE('',*,*,#47793,.T.) ;
#66188=ORIENTED_EDGE('',*,*,#47794,.T.) ;
#66189=ORIENTED_EDGE('',*,*,#47795,.T.) ;
#66190=ORIENTED_EDGE('',*,*,#47796,.T.) ;
#66191=ORIENTED_EDGE('',*,*,#47797,.T.) ;
#66192=ORIENTED_EDGE('',*,*,#47798,.T.) ;
#66193=ORIENTED_EDGE('',*,*,#47799,.T.) ;
#66194=ORIENTED_EDGE('',*,*,#47800,.T.) ;
#66195=ORIENTED_EDGE('',*,*,#47801,.T.) ;
#66196=ORIENTED_EDGE('',*,*,#47802,.T.) ;
#66197=ORIENTED_EDGE('',*,*,#46601,.T.) ;
#66198=ORIENTED_EDGE('',*,*,#47803,.T.) ;
#66199=ORIENTED_EDGE('',*,*,#46605,.F.) ;
#66200=ORIENTED_EDGE('',*,*,#47804,.T.) ;
#66201=ORIENTED_EDGE('',*,*,#47805,.T.) ;
#66202=ORIENTED_EDGE('',*,*,#47806,.T.) ;
#66203=ORIENTED_EDGE('',*,*,#47807,.T.) ;
#66204=ORIENTED_EDGE('',*,*,#47808,.T.) ;
#66205=ORIENTED_EDGE('',*,*,#47809,.T.) ;
#66206=ORIENTED_EDGE('',*,*,#47810,.T.) ;
#66207=ORIENTED_EDGE('',*,*,#47811,.T.) ;
#66208=ORIENTED_EDGE('',*,*,#47812,.T.) ;
#66209=ORIENTED_EDGE('',*,*,#47813,.T.) ;
#66210=ORIENTED_EDGE('',*,*,#47814,.T.) ;
#66211=ORIENTED_EDGE('',*,*,#47815,.T.) ;
#66212=ORIENTED_EDGE('',*,*,#47816,.T.) ;
#66213=ORIENTED_EDGE('',*,*,#47817,.T.) ;
#66214=ORIENTED_EDGE('',*,*,#47818,.T.) ;
#66215=ORIENTED_EDGE('',*,*,#47819,.T.) ;
#66216=ORIENTED_EDGE('',*,*,#47820,.T.) ;
#66217=ORIENTED_EDGE('',*,*,#47821,.T.) ;
#66218=ORIENTED_EDGE('',*,*,#47822,.T.) ;
#66219=ORIENTED_EDGE('',*,*,#47823,.T.) ;
#66220=ORIENTED_EDGE('',*,*,#47824,.T.) ;
#66221=ORIENTED_EDGE('',*,*,#47825,.F.) ;
#66222=ORIENTED_EDGE('',*,*,#47826,.T.) ;
#66223=ORIENTED_EDGE('',*,*,#47827,.T.) ;
#66224=ORIENTED_EDGE('',*,*,#47828,.T.) ;
#66225=ORIENTED_EDGE('',*,*,#47089,.T.) ;
#66226=ORIENTED_EDGE('',*,*,#47829,.T.) ;
#66227=ORIENTED_EDGE('',*,*,#47830,.T.) ;
#66228=ORIENTED_EDGE('',*,*,#47831,.T.) ;
#66229=ORIENTED_EDGE('',*,*,#47832,.T.) ;
#66230=ORIENTED_EDGE('',*,*,#47833,.T.) ;
#66231=ORIENTED_EDGE('',*,*,#44264,.T.) ;
#66232=ORIENTED_EDGE('',*,*,#47834,.T.) ;
#66233=ORIENTED_EDGE('',*,*,#47835,.T.) ;
#66234=ORIENTED_EDGE('',*,*,#47836,.T.) ;
#66235=ORIENTED_EDGE('',*,*,#47086,.T.) ;
#66236=ORIENTED_EDGE('',*,*,#47837,.T.) ;
#66237=ORIENTED_EDGE('',*,*,#47807,.F.) ;
#66238=ORIENTED_EDGE('',*,*,#47838,.T.) ;
#66239=ORIENTED_EDGE('',*,*,#47087,.T.) ;
#66240=ORIENTED_EDGE('',*,*,#47825,.T.) ;
#66241=ORIENTED_EDGE('',*,*,#47839,.T.) ;
#66242=ORIENTED_EDGE('',*,*,#44465,.F.) ;
#66243=ORIENTED_EDGE('',*,*,#47840,.T.) ;
#66244=ORIENTED_EDGE('',*,*,#47841,.T.) ;
#66245=ORIENTED_EDGE('',*,*,#47842,.T.) ;
#66246=ORIENTED_EDGE('',*,*,#47843,.T.) ;
#66247=ORIENTED_EDGE('',*,*,#47844,.T.) ;
#66248=ORIENTED_EDGE('',*,*,#47845,.T.) ;
#66249=ORIENTED_EDGE('',*,*,#47846,.T.) ;
#66250=ORIENTED_EDGE('',*,*,#46611,.F.) ;
#66251=ORIENTED_EDGE('',*,*,#47847,.T.) ;
#66252=ORIENTED_EDGE('',*,*,#46615,.F.) ;
#66253=ORIENTED_EDGE('',*,*,#47848,.T.) ;
#66254=ORIENTED_EDGE('',*,*,#47849,.T.) ;
#66255=ORIENTED_EDGE('',*,*,#47850,.T.) ;
#66256=ORIENTED_EDGE('',*,*,#47851,.T.) ;
#66257=ORIENTED_EDGE('',*,*,#47852,.T.) ;
#66258=ORIENTED_EDGE('',*,*,#47853,.T.) ;
#66259=ORIENTED_EDGE('',*,*,#47854,.T.) ;
#66260=ORIENTED_EDGE('',*,*,#47855,.T.) ;
#66261=ORIENTED_EDGE('',*,*,#47856,.T.) ;
#66262=ORIENTED_EDGE('',*,*,#47857,.T.) ;
#66263=ORIENTED_EDGE('',*,*,#47858,.T.) ;
#66264=ORIENTED_EDGE('',*,*,#47859,.T.) ;
#66265=ORIENTED_EDGE('',*,*,#47860,.T.) ;
#66266=ORIENTED_EDGE('',*,*,#46609,.T.) ;
#66267=ORIENTED_EDGE('',*,*,#47861,.T.) ;
#66268=ORIENTED_EDGE('',*,*,#46613,.F.) ;
#66269=ORIENTED_EDGE('',*,*,#47862,.T.) ;
#66270=ORIENTED_EDGE('',*,*,#47863,.T.) ;
#66271=ORIENTED_EDGE('',*,*,#47864,.T.) ;
#66272=ORIENTED_EDGE('',*,*,#47865,.T.) ;
#66273=ORIENTED_EDGE('',*,*,#47866,.T.) ;
#66274=ORIENTED_EDGE('',*,*,#47867,.T.) ;
#66275=ORIENTED_EDGE('',*,*,#47868,.T.) ;
#66276=ORIENTED_EDGE('',*,*,#47869,.T.) ;
#66277=ORIENTED_EDGE('',*,*,#47870,.T.) ;
#66278=ORIENTED_EDGE('',*,*,#47871,.T.) ;
#66279=ORIENTED_EDGE('',*,*,#47872,.T.) ;
#66280=ORIENTED_EDGE('',*,*,#47873,.T.) ;
#66281=ORIENTED_EDGE('',*,*,#47874,.T.) ;
#66282=ORIENTED_EDGE('',*,*,#47875,.T.) ;
#66283=ORIENTED_EDGE('',*,*,#47876,.T.) ;
#66284=ORIENTED_EDGE('',*,*,#47877,.T.) ;
#66285=ORIENTED_EDGE('',*,*,#47878,.T.) ;
#66286=ORIENTED_EDGE('',*,*,#47879,.T.) ;
#66287=ORIENTED_EDGE('',*,*,#47880,.T.) ;
#66288=ORIENTED_EDGE('',*,*,#47881,.T.) ;
#66289=ORIENTED_EDGE('',*,*,#47882,.T.) ;
#66290=ORIENTED_EDGE('',*,*,#47883,.F.) ;
#66291=ORIENTED_EDGE('',*,*,#47884,.T.) ;
#66292=ORIENTED_EDGE('',*,*,#47885,.T.) ;
#66293=ORIENTED_EDGE('',*,*,#47886,.T.) ;
#66294=ORIENTED_EDGE('',*,*,#47177,.T.) ;
#66295=ORIENTED_EDGE('',*,*,#47887,.T.) ;
#66296=ORIENTED_EDGE('',*,*,#47888,.T.) ;
#66297=ORIENTED_EDGE('',*,*,#47889,.T.) ;
#66298=ORIENTED_EDGE('',*,*,#47890,.T.) ;
#66299=ORIENTED_EDGE('',*,*,#47891,.T.) ;
#66300=ORIENTED_EDGE('',*,*,#44247,.T.) ;
#66301=ORIENTED_EDGE('',*,*,#47892,.T.) ;
#66302=ORIENTED_EDGE('',*,*,#47893,.T.) ;
#66303=ORIENTED_EDGE('',*,*,#47894,.T.) ;
#66304=ORIENTED_EDGE('',*,*,#47174,.T.) ;
#66305=ORIENTED_EDGE('',*,*,#47895,.T.) ;
#66306=ORIENTED_EDGE('',*,*,#47865,.F.) ;
#66307=ORIENTED_EDGE('',*,*,#47896,.T.) ;
#66308=ORIENTED_EDGE('',*,*,#47175,.T.) ;
#66309=ORIENTED_EDGE('',*,*,#47883,.T.) ;
#66310=ORIENTED_EDGE('',*,*,#47897,.T.) ;
#66311=ORIENTED_EDGE('',*,*,#44454,.F.) ;
#66312=ORIENTED_EDGE('',*,*,#47898,.T.) ;
#66313=ORIENTED_EDGE('',*,*,#47899,.T.) ;
#66314=ORIENTED_EDGE('',*,*,#47900,.T.) ;
#66315=ORIENTED_EDGE('',*,*,#47901,.T.) ;
#66316=ORIENTED_EDGE('',*,*,#47902,.T.) ;
#66317=ORIENTED_EDGE('',*,*,#47903,.T.) ;
#66318=ORIENTED_EDGE('',*,*,#47904,.T.) ;
#66319=ORIENTED_EDGE('',*,*,#46619,.F.) ;
#66320=ORIENTED_EDGE('',*,*,#47905,.T.) ;
#66321=ORIENTED_EDGE('',*,*,#46623,.F.) ;
#66322=ORIENTED_EDGE('',*,*,#47906,.T.) ;
#66323=ORIENTED_EDGE('',*,*,#47907,.T.) ;
#66324=ORIENTED_EDGE('',*,*,#47908,.T.) ;
#66325=ORIENTED_EDGE('',*,*,#47909,.T.) ;
#66326=ORIENTED_EDGE('',*,*,#47910,.T.) ;
#66327=ORIENTED_EDGE('',*,*,#47911,.T.) ;
#66328=ORIENTED_EDGE('',*,*,#47912,.T.) ;
#66329=ORIENTED_EDGE('',*,*,#47913,.T.) ;
#66330=ORIENTED_EDGE('',*,*,#47914,.T.) ;
#66331=ORIENTED_EDGE('',*,*,#47915,.T.) ;
#66332=ORIENTED_EDGE('',*,*,#47916,.T.) ;
#66333=ORIENTED_EDGE('',*,*,#47917,.T.) ;
#66334=ORIENTED_EDGE('',*,*,#47918,.T.) ;
#66335=ORIENTED_EDGE('',*,*,#46617,.T.) ;
#66336=ORIENTED_EDGE('',*,*,#47919,.T.) ;
#66337=ORIENTED_EDGE('',*,*,#46621,.F.) ;
#66338=ORIENTED_EDGE('',*,*,#47920,.T.) ;
#66339=ORIENTED_EDGE('',*,*,#47921,.T.) ;
#66340=ORIENTED_EDGE('',*,*,#47922,.T.) ;
#66341=ORIENTED_EDGE('',*,*,#47923,.T.) ;
#66342=ORIENTED_EDGE('',*,*,#47924,.T.) ;
#66343=ORIENTED_EDGE('',*,*,#47925,.T.) ;
#66344=ORIENTED_EDGE('',*,*,#47926,.T.) ;
#66345=ORIENTED_EDGE('',*,*,#47927,.T.) ;
#66346=ORIENTED_EDGE('',*,*,#47928,.T.) ;
#66347=ORIENTED_EDGE('',*,*,#47929,.T.) ;
#66348=ORIENTED_EDGE('',*,*,#47930,.T.) ;
#66349=ORIENTED_EDGE('',*,*,#47931,.T.) ;
#66350=ORIENTED_EDGE('',*,*,#47932,.T.) ;
#66351=ORIENTED_EDGE('',*,*,#47933,.T.) ;
#66352=ORIENTED_EDGE('',*,*,#47934,.T.) ;
#66353=ORIENTED_EDGE('',*,*,#47935,.T.) ;
#66354=ORIENTED_EDGE('',*,*,#47936,.T.) ;
#66355=ORIENTED_EDGE('',*,*,#47937,.T.) ;
#66356=ORIENTED_EDGE('',*,*,#47938,.T.) ;
#66357=ORIENTED_EDGE('',*,*,#47939,.T.) ;
#66358=ORIENTED_EDGE('',*,*,#47940,.T.) ;
#66359=ORIENTED_EDGE('',*,*,#47941,.F.) ;
#66360=ORIENTED_EDGE('',*,*,#47942,.T.) ;
#66361=ORIENTED_EDGE('',*,*,#47943,.T.) ;
#66362=ORIENTED_EDGE('',*,*,#47944,.T.) ;
#66363=ORIENTED_EDGE('',*,*,#47265,.T.) ;
#66364=ORIENTED_EDGE('',*,*,#47945,.T.) ;
#66365=ORIENTED_EDGE('',*,*,#47946,.T.) ;
#66366=ORIENTED_EDGE('',*,*,#47947,.T.) ;
#66367=ORIENTED_EDGE('',*,*,#47948,.T.) ;
#66368=ORIENTED_EDGE('',*,*,#47949,.T.) ;
#66369=ORIENTED_EDGE('',*,*,#44230,.T.) ;
#66370=ORIENTED_EDGE('',*,*,#47950,.T.) ;
#66371=ORIENTED_EDGE('',*,*,#47951,.T.) ;
#66372=ORIENTED_EDGE('',*,*,#47952,.T.) ;
#66373=ORIENTED_EDGE('',*,*,#47262,.T.) ;
#66374=ORIENTED_EDGE('',*,*,#47953,.T.) ;
#66375=ORIENTED_EDGE('',*,*,#47923,.F.) ;
#66376=ORIENTED_EDGE('',*,*,#47954,.T.) ;
#66377=ORIENTED_EDGE('',*,*,#47263,.T.) ;
#66378=ORIENTED_EDGE('',*,*,#47941,.T.) ;
#66379=ORIENTED_EDGE('',*,*,#47955,.T.) ;
#66380=ORIENTED_EDGE('',*,*,#44443,.F.) ;
#66381=ORIENTED_EDGE('',*,*,#47956,.T.) ;
#66382=ORIENTED_EDGE('',*,*,#47957,.T.) ;
#66383=ORIENTED_EDGE('',*,*,#47958,.T.) ;
#66384=ORIENTED_EDGE('',*,*,#47959,.T.) ;
#66385=ORIENTED_EDGE('',*,*,#47960,.T.) ;
#66386=ORIENTED_EDGE('',*,*,#47961,.T.) ;
#66387=ORIENTED_EDGE('',*,*,#47962,.T.) ;
#66388=ORIENTED_EDGE('',*,*,#46627,.F.) ;
#66389=ORIENTED_EDGE('',*,*,#47963,.T.) ;
#66390=ORIENTED_EDGE('',*,*,#46631,.F.) ;
#66391=ORIENTED_EDGE('',*,*,#47964,.T.) ;
#66392=ORIENTED_EDGE('',*,*,#47965,.T.) ;
#66393=ORIENTED_EDGE('',*,*,#47966,.T.) ;
#66394=ORIENTED_EDGE('',*,*,#47967,.T.) ;
#66395=ORIENTED_EDGE('',*,*,#47968,.T.) ;
#66396=ORIENTED_EDGE('',*,*,#47969,.T.) ;
#66397=ORIENTED_EDGE('',*,*,#47970,.T.) ;
#66398=ORIENTED_EDGE('',*,*,#47971,.T.) ;
#66399=ORIENTED_EDGE('',*,*,#47972,.T.) ;
#66400=ORIENTED_EDGE('',*,*,#47973,.T.) ;
#66401=ORIENTED_EDGE('',*,*,#47974,.T.) ;
#66402=ORIENTED_EDGE('',*,*,#47975,.T.) ;
#66403=ORIENTED_EDGE('',*,*,#47976,.T.) ;
#66404=ORIENTED_EDGE('',*,*,#46625,.T.) ;
#66405=ORIENTED_EDGE('',*,*,#47977,.T.) ;
#66406=ORIENTED_EDGE('',*,*,#46629,.F.) ;
#66407=ORIENTED_EDGE('',*,*,#47978,.T.) ;
#66408=ORIENTED_EDGE('',*,*,#47979,.T.) ;
#66409=ORIENTED_EDGE('',*,*,#47980,.T.) ;
#66410=ORIENTED_EDGE('',*,*,#47981,.T.) ;
#66411=ORIENTED_EDGE('',*,*,#47982,.T.) ;
#66412=ORIENTED_EDGE('',*,*,#47983,.T.) ;
#66413=ORIENTED_EDGE('',*,*,#47984,.T.) ;
#66414=ORIENTED_EDGE('',*,*,#47985,.T.) ;
#66415=ORIENTED_EDGE('',*,*,#47986,.T.) ;
#66416=ORIENTED_EDGE('',*,*,#47987,.T.) ;
#66417=ORIENTED_EDGE('',*,*,#47988,.T.) ;
#66418=ORIENTED_EDGE('',*,*,#47989,.T.) ;
#66419=ORIENTED_EDGE('',*,*,#47990,.T.) ;
#66420=ORIENTED_EDGE('',*,*,#47991,.T.) ;
#66421=ORIENTED_EDGE('',*,*,#47992,.T.) ;
#66422=ORIENTED_EDGE('',*,*,#47993,.T.) ;
#66423=ORIENTED_EDGE('',*,*,#47994,.T.) ;
#66424=ORIENTED_EDGE('',*,*,#47995,.T.) ;
#66425=ORIENTED_EDGE('',*,*,#47996,.T.) ;
#66426=ORIENTED_EDGE('',*,*,#47997,.T.) ;
#66427=ORIENTED_EDGE('',*,*,#47998,.T.) ;
#66428=ORIENTED_EDGE('',*,*,#47999,.F.) ;
#66429=ORIENTED_EDGE('',*,*,#48000,.T.) ;
#66430=ORIENTED_EDGE('',*,*,#48001,.T.) ;
#66431=ORIENTED_EDGE('',*,*,#48002,.T.) ;
#66432=ORIENTED_EDGE('',*,*,#47353,.T.) ;
#66433=ORIENTED_EDGE('',*,*,#48003,.T.) ;
#66434=ORIENTED_EDGE('',*,*,#48004,.T.) ;
#66435=ORIENTED_EDGE('',*,*,#48005,.T.) ;
#66436=ORIENTED_EDGE('',*,*,#48006,.T.) ;
#66437=ORIENTED_EDGE('',*,*,#48007,.T.) ;
#66438=ORIENTED_EDGE('',*,*,#44213,.T.) ;
#66439=ORIENTED_EDGE('',*,*,#48008,.T.) ;
#66440=ORIENTED_EDGE('',*,*,#48009,.T.) ;
#66441=ORIENTED_EDGE('',*,*,#48010,.T.) ;
#66442=ORIENTED_EDGE('',*,*,#47350,.T.) ;
#66443=ORIENTED_EDGE('',*,*,#48011,.T.) ;
#66444=ORIENTED_EDGE('',*,*,#47981,.F.) ;
#66445=ORIENTED_EDGE('',*,*,#48012,.T.) ;
#66446=ORIENTED_EDGE('',*,*,#47351,.T.) ;
#66447=ORIENTED_EDGE('',*,*,#47999,.T.) ;
#66448=ORIENTED_EDGE('',*,*,#48013,.T.) ;
#66449=ORIENTED_EDGE('',*,*,#44432,.F.) ;
#66450=ORIENTED_EDGE('',*,*,#48014,.T.) ;
#66451=ORIENTED_EDGE('',*,*,#48015,.T.) ;
#66452=ORIENTED_EDGE('',*,*,#48016,.T.) ;
#66453=ORIENTED_EDGE('',*,*,#48017,.T.) ;
#66454=ORIENTED_EDGE('',*,*,#48018,.T.) ;
#66455=ORIENTED_EDGE('',*,*,#48019,.T.) ;
#66456=ORIENTED_EDGE('',*,*,#48020,.T.) ;
#66457=ORIENTED_EDGE('',*,*,#46635,.F.) ;
#66458=ORIENTED_EDGE('',*,*,#48021,.T.) ;
#66459=ORIENTED_EDGE('',*,*,#46639,.F.) ;
#66460=ORIENTED_EDGE('',*,*,#48022,.T.) ;
#66461=ORIENTED_EDGE('',*,*,#48023,.T.) ;
#66462=ORIENTED_EDGE('',*,*,#48024,.T.) ;
#66463=ORIENTED_EDGE('',*,*,#48025,.T.) ;
#66464=ORIENTED_EDGE('',*,*,#48026,.T.) ;
#66465=ORIENTED_EDGE('',*,*,#48027,.T.) ;
#66466=ORIENTED_EDGE('',*,*,#48028,.T.) ;
#66467=ORIENTED_EDGE('',*,*,#48029,.T.) ;
#66468=ORIENTED_EDGE('',*,*,#48030,.T.) ;
#66469=ORIENTED_EDGE('',*,*,#48031,.T.) ;
#66470=ORIENTED_EDGE('',*,*,#48032,.T.) ;
#66471=ORIENTED_EDGE('',*,*,#48033,.T.) ;
#66472=ORIENTED_EDGE('',*,*,#48034,.T.) ;
#66473=ORIENTED_EDGE('',*,*,#46633,.T.) ;
#66474=ORIENTED_EDGE('',*,*,#48035,.T.) ;
#66475=ORIENTED_EDGE('',*,*,#46637,.F.) ;
#66476=ORIENTED_EDGE('',*,*,#48036,.T.) ;
#66477=ORIENTED_EDGE('',*,*,#48037,.T.) ;
#66478=ORIENTED_EDGE('',*,*,#48038,.T.) ;
#66479=ORIENTED_EDGE('',*,*,#48039,.T.) ;
#66480=ORIENTED_EDGE('',*,*,#48040,.T.) ;
#66481=ORIENTED_EDGE('',*,*,#48041,.T.) ;
#66482=ORIENTED_EDGE('',*,*,#48042,.T.) ;
#66483=ORIENTED_EDGE('',*,*,#48043,.T.) ;
#66484=ORIENTED_EDGE('',*,*,#48044,.T.) ;
#66485=ORIENTED_EDGE('',*,*,#48045,.T.) ;
#66486=ORIENTED_EDGE('',*,*,#48046,.T.) ;
#66487=ORIENTED_EDGE('',*,*,#48047,.T.) ;
#66488=ORIENTED_EDGE('',*,*,#48048,.T.) ;
#66489=ORIENTED_EDGE('',*,*,#48049,.T.) ;
#66490=ORIENTED_EDGE('',*,*,#48050,.T.) ;
#66491=ORIENTED_EDGE('',*,*,#48051,.T.) ;
#66492=ORIENTED_EDGE('',*,*,#48052,.T.) ;
#66493=ORIENTED_EDGE('',*,*,#48053,.T.) ;
#66494=ORIENTED_EDGE('',*,*,#48054,.T.) ;
#66495=ORIENTED_EDGE('',*,*,#48055,.T.) ;
#66496=ORIENTED_EDGE('',*,*,#48056,.T.) ;
#66497=ORIENTED_EDGE('',*,*,#48057,.F.) ;
#66498=ORIENTED_EDGE('',*,*,#48058,.T.) ;
#66499=ORIENTED_EDGE('',*,*,#48059,.T.) ;
#66500=ORIENTED_EDGE('',*,*,#48060,.T.) ;
#66501=ORIENTED_EDGE('',*,*,#47441,.T.) ;
#66502=ORIENTED_EDGE('',*,*,#48061,.T.) ;
#66503=ORIENTED_EDGE('',*,*,#48062,.T.) ;
#66504=ORIENTED_EDGE('',*,*,#48063,.T.) ;
#66505=ORIENTED_EDGE('',*,*,#48064,.T.) ;
#66506=ORIENTED_EDGE('',*,*,#48065,.T.) ;
#66507=ORIENTED_EDGE('',*,*,#44196,.T.) ;
#66508=ORIENTED_EDGE('',*,*,#48066,.T.) ;
#66509=ORIENTED_EDGE('',*,*,#48067,.T.) ;
#66510=ORIENTED_EDGE('',*,*,#48068,.T.) ;
#66511=ORIENTED_EDGE('',*,*,#47438,.T.) ;
#66512=ORIENTED_EDGE('',*,*,#48069,.T.) ;
#66513=ORIENTED_EDGE('',*,*,#48039,.F.) ;
#66514=ORIENTED_EDGE('',*,*,#48070,.T.) ;
#66515=ORIENTED_EDGE('',*,*,#47439,.T.) ;
#66516=ORIENTED_EDGE('',*,*,#48057,.T.) ;
#66517=ORIENTED_EDGE('',*,*,#48071,.T.) ;
#66518=ORIENTED_EDGE('',*,*,#44421,.F.) ;
#66519=ORIENTED_EDGE('',*,*,#48072,.T.) ;
#66520=ORIENTED_EDGE('',*,*,#48073,.T.) ;
#66521=ORIENTED_EDGE('',*,*,#48074,.T.) ;
#66522=ORIENTED_EDGE('',*,*,#48075,.T.) ;
#66523=ORIENTED_EDGE('',*,*,#48076,.T.) ;
#66524=ORIENTED_EDGE('',*,*,#48077,.T.) ;
#66525=ORIENTED_EDGE('',*,*,#48078,.T.) ;
#66526=ORIENTED_EDGE('',*,*,#46643,.F.) ;
#66527=ORIENTED_EDGE('',*,*,#48079,.T.) ;
#66528=ORIENTED_EDGE('',*,*,#46647,.F.) ;
#66529=ORIENTED_EDGE('',*,*,#48080,.T.) ;
#66530=ORIENTED_EDGE('',*,*,#48081,.T.) ;
#66531=ORIENTED_EDGE('',*,*,#48082,.T.) ;
#66532=ORIENTED_EDGE('',*,*,#48083,.T.) ;
#66533=ORIENTED_EDGE('',*,*,#48084,.T.) ;
#66534=ORIENTED_EDGE('',*,*,#48085,.T.) ;
#66535=ORIENTED_EDGE('',*,*,#48086,.T.) ;
#66536=ORIENTED_EDGE('',*,*,#48087,.T.) ;
#66537=ORIENTED_EDGE('',*,*,#48088,.T.) ;
#66538=ORIENTED_EDGE('',*,*,#48089,.T.) ;
#66539=ORIENTED_EDGE('',*,*,#48090,.T.) ;
#66540=ORIENTED_EDGE('',*,*,#48091,.T.) ;
#66541=ORIENTED_EDGE('',*,*,#48092,.T.) ;
#66542=ORIENTED_EDGE('',*,*,#46641,.T.) ;
#66543=ORIENTED_EDGE('',*,*,#48093,.T.) ;
#66544=ORIENTED_EDGE('',*,*,#46645,.F.) ;
#66545=ORIENTED_EDGE('',*,*,#48094,.T.) ;
#66546=ORIENTED_EDGE('',*,*,#48095,.T.) ;
#66547=ORIENTED_EDGE('',*,*,#48096,.T.) ;
#66548=ORIENTED_EDGE('',*,*,#48097,.T.) ;
#66549=ORIENTED_EDGE('',*,*,#48098,.T.) ;
#66550=ORIENTED_EDGE('',*,*,#48099,.T.) ;
#66551=ORIENTED_EDGE('',*,*,#48100,.T.) ;
#66552=ORIENTED_EDGE('',*,*,#48101,.T.) ;
#66553=ORIENTED_EDGE('',*,*,#48102,.T.) ;
#66554=ORIENTED_EDGE('',*,*,#48103,.T.) ;
#66555=ORIENTED_EDGE('',*,*,#48104,.T.) ;
#66556=ORIENTED_EDGE('',*,*,#48105,.T.) ;
#66557=ORIENTED_EDGE('',*,*,#48106,.T.) ;
#66558=ORIENTED_EDGE('',*,*,#48107,.T.) ;
#66559=ORIENTED_EDGE('',*,*,#48108,.T.) ;
#66560=ORIENTED_EDGE('',*,*,#48109,.T.) ;
#66561=ORIENTED_EDGE('',*,*,#48110,.T.) ;
#66562=ORIENTED_EDGE('',*,*,#48111,.T.) ;
#66563=ORIENTED_EDGE('',*,*,#48112,.T.) ;
#66564=ORIENTED_EDGE('',*,*,#48113,.T.) ;
#66565=ORIENTED_EDGE('',*,*,#48114,.T.) ;
#66566=ORIENTED_EDGE('',*,*,#48115,.F.) ;
#66567=ORIENTED_EDGE('',*,*,#48116,.T.) ;
#66568=ORIENTED_EDGE('',*,*,#48117,.T.) ;
#66569=ORIENTED_EDGE('',*,*,#48118,.T.) ;
#66570=ORIENTED_EDGE('',*,*,#47529,.T.) ;
#66571=ORIENTED_EDGE('',*,*,#48119,.T.) ;
#66572=ORIENTED_EDGE('',*,*,#48120,.T.) ;
#66573=ORIENTED_EDGE('',*,*,#48121,.T.) ;
#66574=ORIENTED_EDGE('',*,*,#48122,.T.) ;
#66575=ORIENTED_EDGE('',*,*,#48123,.T.) ;
#66576=ORIENTED_EDGE('',*,*,#44179,.T.) ;
#66577=ORIENTED_EDGE('',*,*,#48124,.T.) ;
#66578=ORIENTED_EDGE('',*,*,#48125,.T.) ;
#66579=ORIENTED_EDGE('',*,*,#48126,.T.) ;
#66580=ORIENTED_EDGE('',*,*,#47526,.T.) ;
#66581=ORIENTED_EDGE('',*,*,#48127,.T.) ;
#66582=ORIENTED_EDGE('',*,*,#48097,.F.) ;
#66583=ORIENTED_EDGE('',*,*,#48128,.T.) ;
#66584=ORIENTED_EDGE('',*,*,#47527,.T.) ;
#66585=ORIENTED_EDGE('',*,*,#48115,.T.) ;
#66586=ORIENTED_EDGE('',*,*,#48129,.T.) ;
#66587=ORIENTED_EDGE('',*,*,#44410,.F.) ;
#66588=ORIENTED_EDGE('',*,*,#48130,.T.) ;
#66589=ORIENTED_EDGE('',*,*,#48131,.T.) ;
#66590=ORIENTED_EDGE('',*,*,#48132,.T.) ;
#66591=ORIENTED_EDGE('',*,*,#48133,.T.) ;
#66592=ORIENTED_EDGE('',*,*,#48134,.T.) ;
#66593=ORIENTED_EDGE('',*,*,#48135,.T.) ;
#66594=ORIENTED_EDGE('',*,*,#48136,.T.) ;
#66595=ORIENTED_EDGE('',*,*,#46651,.F.) ;
#66596=ORIENTED_EDGE('',*,*,#48137,.T.) ;
#66597=ORIENTED_EDGE('',*,*,#46655,.F.) ;
#66598=ORIENTED_EDGE('',*,*,#48138,.T.) ;
#66599=ORIENTED_EDGE('',*,*,#48139,.T.) ;
#66600=ORIENTED_EDGE('',*,*,#48140,.T.) ;
#66601=ORIENTED_EDGE('',*,*,#48141,.T.) ;
#66602=ORIENTED_EDGE('',*,*,#48142,.T.) ;
#66603=ORIENTED_EDGE('',*,*,#48143,.T.) ;
#66604=ORIENTED_EDGE('',*,*,#48144,.T.) ;
#66605=ORIENTED_EDGE('',*,*,#48145,.T.) ;
#66606=ORIENTED_EDGE('',*,*,#48146,.T.) ;
#66607=ORIENTED_EDGE('',*,*,#48147,.T.) ;
#66608=ORIENTED_EDGE('',*,*,#48148,.T.) ;
#66609=ORIENTED_EDGE('',*,*,#48149,.T.) ;
#66610=ORIENTED_EDGE('',*,*,#48150,.T.) ;
#66611=ORIENTED_EDGE('',*,*,#46649,.T.) ;
#66612=ORIENTED_EDGE('',*,*,#48151,.T.) ;
#66613=ORIENTED_EDGE('',*,*,#46653,.F.) ;
#66614=ORIENTED_EDGE('',*,*,#48152,.T.) ;
#66615=ORIENTED_EDGE('',*,*,#48153,.T.) ;
#66616=ORIENTED_EDGE('',*,*,#48154,.T.) ;
#66617=ORIENTED_EDGE('',*,*,#48155,.T.) ;
#66618=ORIENTED_EDGE('',*,*,#48156,.T.) ;
#66619=ORIENTED_EDGE('',*,*,#48157,.T.) ;
#66620=ORIENTED_EDGE('',*,*,#48158,.T.) ;
#66621=ORIENTED_EDGE('',*,*,#48159,.T.) ;
#66622=ORIENTED_EDGE('',*,*,#48160,.T.) ;
#66623=ORIENTED_EDGE('',*,*,#48161,.T.) ;
#66624=ORIENTED_EDGE('',*,*,#48162,.T.) ;
#66625=ORIENTED_EDGE('',*,*,#48163,.T.) ;
#66626=ORIENTED_EDGE('',*,*,#48164,.T.) ;
#66627=ORIENTED_EDGE('',*,*,#48165,.T.) ;
#66628=ORIENTED_EDGE('',*,*,#48166,.T.) ;
#66629=ORIENTED_EDGE('',*,*,#48167,.T.) ;
#66630=ORIENTED_EDGE('',*,*,#48168,.T.) ;
#66631=ORIENTED_EDGE('',*,*,#48169,.T.) ;
#66632=ORIENTED_EDGE('',*,*,#48170,.T.) ;
#66633=ORIENTED_EDGE('',*,*,#48171,.T.) ;
#66634=ORIENTED_EDGE('',*,*,#48172,.T.) ;
#66635=ORIENTED_EDGE('',*,*,#48173,.F.) ;
#66636=ORIENTED_EDGE('',*,*,#48174,.T.) ;
#66637=ORIENTED_EDGE('',*,*,#48175,.T.) ;
#66638=ORIENTED_EDGE('',*,*,#48176,.T.) ;
#66639=ORIENTED_EDGE('',*,*,#47617,.T.) ;
#66640=ORIENTED_EDGE('',*,*,#48177,.T.) ;
#66641=ORIENTED_EDGE('',*,*,#48178,.T.) ;
#66642=ORIENTED_EDGE('',*,*,#48179,.T.) ;
#66643=ORIENTED_EDGE('',*,*,#48180,.T.) ;
#66644=ORIENTED_EDGE('',*,*,#48181,.T.) ;
#66645=ORIENTED_EDGE('',*,*,#44162,.T.) ;
#66646=ORIENTED_EDGE('',*,*,#48182,.T.) ;
#66647=ORIENTED_EDGE('',*,*,#48183,.T.) ;
#66648=ORIENTED_EDGE('',*,*,#48184,.T.) ;
#66649=ORIENTED_EDGE('',*,*,#47614,.T.) ;
#66650=ORIENTED_EDGE('',*,*,#48185,.T.) ;
#66651=ORIENTED_EDGE('',*,*,#48155,.F.) ;
#66652=ORIENTED_EDGE('',*,*,#48186,.T.) ;
#66653=ORIENTED_EDGE('',*,*,#47615,.T.) ;
#66654=ORIENTED_EDGE('',*,*,#48173,.T.) ;
#66655=ORIENTED_EDGE('',*,*,#48187,.T.) ;
#66656=ORIENTED_EDGE('',*,*,#44399,.F.) ;
#66657=ORIENTED_EDGE('',*,*,#48188,.T.) ;
#66658=ORIENTED_EDGE('',*,*,#48189,.T.) ;
#66659=ORIENTED_EDGE('',*,*,#48190,.T.) ;
#66660=ORIENTED_EDGE('',*,*,#48191,.T.) ;
#66661=ORIENTED_EDGE('',*,*,#48192,.T.) ;
#66662=ORIENTED_EDGE('',*,*,#48193,.T.) ;
#66663=ORIENTED_EDGE('',*,*,#48194,.T.) ;
#66664=ORIENTED_EDGE('',*,*,#46659,.F.) ;
#66665=ORIENTED_EDGE('',*,*,#48195,.T.) ;
#66666=ORIENTED_EDGE('',*,*,#46663,.F.) ;
#66667=ORIENTED_EDGE('',*,*,#48196,.T.) ;
#66668=ORIENTED_EDGE('',*,*,#48197,.T.) ;
#66669=ORIENTED_EDGE('',*,*,#48198,.T.) ;
#66670=ORIENTED_EDGE('',*,*,#48199,.T.) ;
#66671=ORIENTED_EDGE('',*,*,#48200,.T.) ;
#66672=ORIENTED_EDGE('',*,*,#48201,.T.) ;
#66673=ORIENTED_EDGE('',*,*,#48202,.T.) ;
#66674=ORIENTED_EDGE('',*,*,#48203,.T.) ;
#66675=ORIENTED_EDGE('',*,*,#48204,.T.) ;
#66676=ORIENTED_EDGE('',*,*,#48205,.T.) ;
#66677=ORIENTED_EDGE('',*,*,#48206,.T.) ;
#66678=ORIENTED_EDGE('',*,*,#48207,.T.) ;
#66679=ORIENTED_EDGE('',*,*,#48208,.T.) ;
#66680=ORIENTED_EDGE('',*,*,#46657,.T.) ;
#66681=ORIENTED_EDGE('',*,*,#48209,.T.) ;
#66682=ORIENTED_EDGE('',*,*,#46661,.F.) ;
#66683=ORIENTED_EDGE('',*,*,#48210,.T.) ;
#66684=ORIENTED_EDGE('',*,*,#48211,.T.) ;
#66685=ORIENTED_EDGE('',*,*,#48212,.T.) ;
#66686=ORIENTED_EDGE('',*,*,#48213,.T.) ;
#66687=ORIENTED_EDGE('',*,*,#48214,.T.) ;
#66688=ORIENTED_EDGE('',*,*,#48215,.T.) ;
#66689=ORIENTED_EDGE('',*,*,#48216,.T.) ;
#66690=ORIENTED_EDGE('',*,*,#48217,.T.) ;
#66691=ORIENTED_EDGE('',*,*,#48218,.T.) ;
#66692=ORIENTED_EDGE('',*,*,#48219,.T.) ;
#66693=ORIENTED_EDGE('',*,*,#48220,.T.) ;
#66694=ORIENTED_EDGE('',*,*,#48221,.T.) ;
#66695=ORIENTED_EDGE('',*,*,#48222,.T.) ;
#66696=ORIENTED_EDGE('',*,*,#48223,.T.) ;
#66697=ORIENTED_EDGE('',*,*,#48224,.T.) ;
#66698=ORIENTED_EDGE('',*,*,#48225,.T.) ;
#66699=ORIENTED_EDGE('',*,*,#48226,.T.) ;
#66700=ORIENTED_EDGE('',*,*,#48227,.T.) ;
#66701=ORIENTED_EDGE('',*,*,#48228,.T.) ;
#66702=ORIENTED_EDGE('',*,*,#48229,.T.) ;
#66703=ORIENTED_EDGE('',*,*,#48230,.T.) ;
#66704=ORIENTED_EDGE('',*,*,#48231,.T.) ;
#66705=ORIENTED_EDGE('',*,*,#48232,.T.) ;
#66706=ORIENTED_EDGE('',*,*,#48233,.T.) ;
#66707=ORIENTED_EDGE('',*,*,#48234,.T.) ;
#66708=ORIENTED_EDGE('',*,*,#48235,.T.) ;
#66709=ORIENTED_EDGE('',*,*,#48236,.T.) ;
#66710=ORIENTED_EDGE('',*,*,#48237,.T.) ;
#66711=ORIENTED_EDGE('',*,*,#48238,.T.) ;
#66712=ORIENTED_EDGE('',*,*,#48239,.T.) ;
#66713=ORIENTED_EDGE('',*,*,#48240,.T.) ;
#66714=ORIENTED_EDGE('',*,*,#48241,.T.) ;
#66715=ORIENTED_EDGE('',*,*,#48242,.T.) ;
#66716=ORIENTED_EDGE('',*,*,#48243,.T.) ;
#66717=ORIENTED_EDGE('',*,*,#48244,.T.) ;
#66718=ORIENTED_EDGE('',*,*,#48245,.T.) ;
#66719=ORIENTED_EDGE('',*,*,#48246,.T.) ;
#66720=ORIENTED_EDGE('',*,*,#48247,.T.) ;
#66721=ORIENTED_EDGE('',*,*,#48248,.T.) ;
#66722=ORIENTED_EDGE('',*,*,#48249,.T.) ;
#66723=ORIENTED_EDGE('',*,*,#48250,.T.) ;
#66724=ORIENTED_EDGE('',*,*,#48251,.T.) ;
#66725=ORIENTED_EDGE('',*,*,#48252,.T.) ;
#66726=ORIENTED_EDGE('',*,*,#48253,.T.) ;
#66727=ORIENTED_EDGE('',*,*,#48254,.T.) ;
#66728=ORIENTED_EDGE('',*,*,#48255,.T.) ;
#66729=ORIENTED_EDGE('',*,*,#48256,.T.) ;
#66730=ORIENTED_EDGE('',*,*,#48257,.T.) ;
#66731=ORIENTED_EDGE('',*,*,#48258,.T.) ;
#66732=ORIENTED_EDGE('',*,*,#48259,.T.) ;
#66733=ORIENTED_EDGE('',*,*,#48260,.T.) ;
#66734=ORIENTED_EDGE('',*,*,#48261,.T.) ;
#66735=ORIENTED_EDGE('',*,*,#48262,.T.) ;
#66736=ORIENTED_EDGE('',*,*,#48263,.T.) ;
#66737=ORIENTED_EDGE('',*,*,#48264,.T.) ;
#66738=ORIENTED_EDGE('',*,*,#48265,.T.) ;
#66739=ORIENTED_EDGE('',*,*,#48266,.T.) ;
#66740=ORIENTED_EDGE('',*,*,#48267,.T.) ;
#66741=ORIENTED_EDGE('',*,*,#48268,.T.) ;
#66742=ORIENTED_EDGE('',*,*,#48269,.T.) ;
#66743=ORIENTED_EDGE('',*,*,#48270,.T.) ;
#66744=ORIENTED_EDGE('',*,*,#48271,.T.) ;
#66745=ORIENTED_EDGE('',*,*,#48272,.T.) ;
#66746=ORIENTED_EDGE('',*,*,#48273,.T.) ;
#66747=ORIENTED_EDGE('',*,*,#48274,.T.) ;
#66748=ORIENTED_EDGE('',*,*,#48275,.T.) ;
#66749=ORIENTED_EDGE('',*,*,#48276,.T.) ;
#66750=ORIENTED_EDGE('',*,*,#48277,.T.) ;
#66751=ORIENTED_EDGE('',*,*,#48278,.T.) ;
#66752=ORIENTED_EDGE('',*,*,#48279,.T.) ;
#66753=ORIENTED_EDGE('',*,*,#48280,.T.) ;
#66754=ORIENTED_EDGE('',*,*,#48281,.T.) ;
#66755=ORIENTED_EDGE('',*,*,#48282,.T.) ;
#66756=ORIENTED_EDGE('',*,*,#48283,.T.) ;
#66757=ORIENTED_EDGE('',*,*,#48284,.T.) ;
#66758=ORIENTED_EDGE('',*,*,#48285,.T.) ;
#66759=ORIENTED_EDGE('',*,*,#48286,.T.) ;
#66760=ORIENTED_EDGE('',*,*,#48287,.T.) ;
#66761=ORIENTED_EDGE('',*,*,#48288,.T.) ;
#66762=ORIENTED_EDGE('',*,*,#48289,.T.) ;
#66763=ORIENTED_EDGE('',*,*,#48290,.T.) ;
#66764=ORIENTED_EDGE('',*,*,#48291,.T.) ;
#66765=ORIENTED_EDGE('',*,*,#48292,.T.) ;
#66766=ORIENTED_EDGE('',*,*,#48293,.T.) ;
#66767=ORIENTED_EDGE('',*,*,#48294,.T.) ;
#66768=ORIENTED_EDGE('',*,*,#48295,.T.) ;
#66769=ORIENTED_EDGE('',*,*,#48296,.T.) ;
#66770=ORIENTED_EDGE('',*,*,#48297,.T.) ;
#66771=ORIENTED_EDGE('',*,*,#48298,.T.) ;
#66772=ORIENTED_EDGE('',*,*,#48299,.T.) ;
#66773=ORIENTED_EDGE('',*,*,#48300,.T.) ;
#66774=ORIENTED_EDGE('',*,*,#48301,.T.) ;
#66775=ORIENTED_EDGE('',*,*,#48302,.T.) ;
#66776=ORIENTED_EDGE('',*,*,#48303,.T.) ;
#66777=ORIENTED_EDGE('',*,*,#48304,.T.) ;
#66778=ORIENTED_EDGE('',*,*,#48305,.T.) ;
#66779=ORIENTED_EDGE('',*,*,#48306,.T.) ;
#66780=ORIENTED_EDGE('',*,*,#48307,.T.) ;
#66781=ORIENTED_EDGE('',*,*,#48308,.T.) ;
#66782=ORIENTED_EDGE('',*,*,#48309,.T.) ;
#66783=ORIENTED_EDGE('',*,*,#48310,.T.) ;
#66784=ORIENTED_EDGE('',*,*,#48311,.T.) ;
#66785=ORIENTED_EDGE('',*,*,#48312,.T.) ;
#66786=ORIENTED_EDGE('',*,*,#48313,.T.) ;
#66787=ORIENTED_EDGE('',*,*,#48314,.T.) ;
#66788=ORIENTED_EDGE('',*,*,#48315,.T.) ;
#66789=ORIENTED_EDGE('',*,*,#48316,.T.) ;
#66790=ORIENTED_EDGE('',*,*,#48317,.T.) ;
#66791=ORIENTED_EDGE('',*,*,#48318,.T.) ;
#66792=ORIENTED_EDGE('',*,*,#48319,.T.) ;
#66793=ORIENTED_EDGE('',*,*,#48320,.T.) ;
#66794=ORIENTED_EDGE('',*,*,#48321,.T.) ;
#66795=ORIENTED_EDGE('',*,*,#48322,.T.) ;
#66796=ORIENTED_EDGE('',*,*,#48323,.T.) ;
#66797=ORIENTED_EDGE('',*,*,#48324,.T.) ;
#66798=ORIENTED_EDGE('',*,*,#48325,.T.) ;
#66799=ORIENTED_EDGE('',*,*,#48326,.T.) ;
#66800=ORIENTED_EDGE('',*,*,#48327,.T.) ;
#66801=ORIENTED_EDGE('',*,*,#48328,.T.) ;
#66802=ORIENTED_EDGE('',*,*,#48329,.T.) ;
#66803=ORIENTED_EDGE('',*,*,#48330,.T.) ;
#66804=ORIENTED_EDGE('',*,*,#48331,.T.) ;
#66805=ORIENTED_EDGE('',*,*,#48332,.T.) ;
#66806=ORIENTED_EDGE('',*,*,#48333,.T.) ;
#66807=ORIENTED_EDGE('',*,*,#48334,.T.) ;
#66808=ORIENTED_EDGE('',*,*,#48335,.T.) ;
#66809=ORIENTED_EDGE('',*,*,#48336,.T.) ;
#66810=ORIENTED_EDGE('',*,*,#48337,.T.) ;
#66811=ORIENTED_EDGE('',*,*,#48338,.T.) ;
#66812=ORIENTED_EDGE('',*,*,#48339,.T.) ;
#66813=ORIENTED_EDGE('',*,*,#48340,.T.) ;
#66814=ORIENTED_EDGE('',*,*,#48341,.T.) ;
#66815=ORIENTED_EDGE('',*,*,#48342,.T.) ;
#66816=ORIENTED_EDGE('',*,*,#48343,.T.) ;
#66817=ORIENTED_EDGE('',*,*,#48344,.T.) ;
#66818=ORIENTED_EDGE('',*,*,#48345,.T.) ;
#66819=ORIENTED_EDGE('',*,*,#48346,.T.) ;
#66820=ORIENTED_EDGE('',*,*,#48347,.T.) ;
#66821=ORIENTED_EDGE('',*,*,#48348,.T.) ;
#66822=ORIENTED_EDGE('',*,*,#48349,.T.) ;
#66823=ORIENTED_EDGE('',*,*,#48350,.T.) ;
#66824=ORIENTED_EDGE('',*,*,#48351,.T.) ;
#66825=ORIENTED_EDGE('',*,*,#48352,.T.) ;
#66826=ORIENTED_EDGE('',*,*,#48353,.T.) ;
#66827=ORIENTED_EDGE('',*,*,#48354,.T.) ;
#66828=ORIENTED_EDGE('',*,*,#48355,.T.) ;
#66829=ORIENTED_EDGE('',*,*,#48356,.T.) ;
#66830=ORIENTED_EDGE('',*,*,#48279,.F.) ;
#66831=ORIENTED_EDGE('',*,*,#48357,.T.) ;
#66832=ORIENTED_EDGE('',*,*,#47706,.F.) ;
#66833=ORIENTED_EDGE('',*,*,#48358,.F.) ;
#66834=ORIENTED_EDGE('',*,*,#47703,.F.) ;
#66835=ORIENTED_EDGE('',*,*,#48359,.T.) ;
#66836=ORIENTED_EDGE('',*,*,#47707,.F.) ;
#66837=ORIENTED_EDGE('',*,*,#48360,.T.) ;
#66838=ORIENTED_EDGE('',*,*,#48361,.F.) ;
#66839=ORIENTED_EDGE('',*,*,#48358,.T.) ;
#66840=ORIENTED_EDGE('',*,*,#48362,.F.) ;
#66841=ORIENTED_EDGE('',*,*,#47704,.F.) ;
#66842=ORIENTED_EDGE('',*,*,#48363,.T.) ;
#66843=ORIENTED_EDGE('',*,*,#48281,.F.) ;
#66844=ORIENTED_EDGE('',*,*,#48364,.F.) ;
#66845=ORIENTED_EDGE('',*,*,#48362,.T.) ;
#66846=ORIENTED_EDGE('',*,*,#47705,.F.) ;
#66847=ORIENTED_EDGE('',*,*,#48365,.F.) ;
#66848=ORIENTED_EDGE('',*,*,#47699,.F.) ;
#66849=ORIENTED_EDGE('',*,*,#48361,.T.) ;
#66850=ORIENTED_EDGE('',*,*,#47702,.F.) ;
#66851=ORIENTED_EDGE('',*,*,#48366,.F.) ;
#66852=ORIENTED_EDGE('',*,*,#48280,.F.) ;
#66853=ORIENTED_EDGE('',*,*,#48365,.T.) ;
#66854=ORIENTED_EDGE('',*,*,#48364,.T.) ;
#66855=ORIENTED_EDGE('',*,*,#48367,.F.) ;
#66856=ORIENTED_EDGE('',*,*,#48368,.F.) ;
#66857=ORIENTED_EDGE('',*,*,#48366,.T.) ;
#66858=ORIENTED_EDGE('',*,*,#48369,.F.) ;
#66859=ORIENTED_EDGE('',*,*,#48367,.T.) ;
#66860=ORIENTED_EDGE('',*,*,#48284,.F.) ;
#66861=ORIENTED_EDGE('',*,*,#48370,.F.) ;
#66862=ORIENTED_EDGE('',*,*,#47700,.F.) ;
#66863=ORIENTED_EDGE('',*,*,#48369,.T.) ;
#66864=ORIENTED_EDGE('',*,*,#47701,.F.) ;
#66865=ORIENTED_EDGE('',*,*,#48371,.F.) ;
#66866=ORIENTED_EDGE('',*,*,#47695,.F.) ;
#66867=ORIENTED_EDGE('',*,*,#47698,.F.) ;
#66868=ORIENTED_EDGE('',*,*,#48372,.T.) ;
#66869=ORIENTED_EDGE('',*,*,#48277,.F.) ;
#66870=ORIENTED_EDGE('',*,*,#48368,.T.) ;
#66871=ORIENTED_EDGE('',*,*,#48371,.T.) ;
#66872=ORIENTED_EDGE('',*,*,#48370,.T.) ;
#66873=ORIENTED_EDGE('',*,*,#48373,.F.) ;
#66874=ORIENTED_EDGE('',*,*,#47693,.F.) ;
#66875=ORIENTED_EDGE('',*,*,#48374,.T.) ;
#66876=ORIENTED_EDGE('',*,*,#47697,.F.) ;
#66877=ORIENTED_EDGE('',*,*,#48375,.T.) ;
#66878=ORIENTED_EDGE('',*,*,#48283,.F.) ;
#66879=ORIENTED_EDGE('',*,*,#48376,.T.) ;
#66880=ORIENTED_EDGE('',*,*,#47696,.F.) ;
#66881=ORIENTED_EDGE('',*,*,#48373,.T.) ;
#66882=ORIENTED_EDGE('',*,*,#48351,.F.) ;
#66883=ORIENTED_EDGE('',*,*,#48377,.T.) ;
#66884=ORIENTED_EDGE('',*,*,#47728,.F.) ;
#66885=ORIENTED_EDGE('',*,*,#48378,.F.) ;
#66886=ORIENTED_EDGE('',*,*,#47725,.F.) ;
#66887=ORIENTED_EDGE('',*,*,#48379,.T.) ;
#66888=ORIENTED_EDGE('',*,*,#47729,.F.) ;
#66889=ORIENTED_EDGE('',*,*,#48380,.T.) ;
#66890=ORIENTED_EDGE('',*,*,#48381,.F.) ;
#66891=ORIENTED_EDGE('',*,*,#48378,.T.) ;
#66892=ORIENTED_EDGE('',*,*,#48382,.F.) ;
#66893=ORIENTED_EDGE('',*,*,#47726,.F.) ;
#66894=ORIENTED_EDGE('',*,*,#48383,.T.) ;
#66895=ORIENTED_EDGE('',*,*,#48353,.F.) ;
#66896=ORIENTED_EDGE('',*,*,#48384,.F.) ;
#66897=ORIENTED_EDGE('',*,*,#48382,.T.) ;
#66898=ORIENTED_EDGE('',*,*,#47727,.F.) ;
#66899=ORIENTED_EDGE('',*,*,#48385,.F.) ;
#66900=ORIENTED_EDGE('',*,*,#47741,.F.) ;
#66901=ORIENTED_EDGE('',*,*,#48381,.T.) ;
#66902=ORIENTED_EDGE('',*,*,#47740,.F.) ;
#66903=ORIENTED_EDGE('',*,*,#48386,.F.) ;
#66904=ORIENTED_EDGE('',*,*,#48352,.F.) ;
#66905=ORIENTED_EDGE('',*,*,#48385,.T.) ;
#66906=ORIENTED_EDGE('',*,*,#48384,.T.) ;
#66907=ORIENTED_EDGE('',*,*,#48387,.F.) ;
#66908=ORIENTED_EDGE('',*,*,#48388,.F.) ;
#66909=ORIENTED_EDGE('',*,*,#48386,.T.) ;
#66910=ORIENTED_EDGE('',*,*,#48389,.F.) ;
#66911=ORIENTED_EDGE('',*,*,#48387,.T.) ;
#66912=ORIENTED_EDGE('',*,*,#48356,.F.) ;
#66913=ORIENTED_EDGE('',*,*,#48390,.F.) ;
#66914=ORIENTED_EDGE('',*,*,#47742,.F.) ;
#66915=ORIENTED_EDGE('',*,*,#48389,.T.) ;
#66916=ORIENTED_EDGE('',*,*,#47739,.F.) ;
#66917=ORIENTED_EDGE('',*,*,#48391,.F.) ;
#66918=ORIENTED_EDGE('',*,*,#47735,.F.) ;
#66919=ORIENTED_EDGE('',*,*,#47738,.F.) ;
#66920=ORIENTED_EDGE('',*,*,#48392,.T.) ;
#66921=ORIENTED_EDGE('',*,*,#48349,.F.) ;
#66922=ORIENTED_EDGE('',*,*,#48388,.T.) ;
#66923=ORIENTED_EDGE('',*,*,#48391,.T.) ;
#66924=ORIENTED_EDGE('',*,*,#48390,.T.) ;
#66925=ORIENTED_EDGE('',*,*,#48393,.F.) ;
#66926=ORIENTED_EDGE('',*,*,#47733,.F.) ;
#66927=ORIENTED_EDGE('',*,*,#48394,.T.) ;
#66928=ORIENTED_EDGE('',*,*,#47737,.F.) ;
#66929=ORIENTED_EDGE('',*,*,#48395,.T.) ;
#66930=ORIENTED_EDGE('',*,*,#48355,.F.) ;
#66931=ORIENTED_EDGE('',*,*,#48396,.T.) ;
#66932=ORIENTED_EDGE('',*,*,#47736,.F.) ;
#66933=ORIENTED_EDGE('',*,*,#48393,.T.) ;
#66934=ORIENTED_EDGE('',*,*,#48271,.F.) ;
#66935=ORIENTED_EDGE('',*,*,#48397,.T.) ;
#66936=ORIENTED_EDGE('',*,*,#47764,.F.) ;
#66937=ORIENTED_EDGE('',*,*,#48398,.F.) ;
#66938=ORIENTED_EDGE('',*,*,#47761,.F.) ;
#66939=ORIENTED_EDGE('',*,*,#48399,.T.) ;
#66940=ORIENTED_EDGE('',*,*,#47765,.F.) ;
#66941=ORIENTED_EDGE('',*,*,#48400,.T.) ;
#66942=ORIENTED_EDGE('',*,*,#48401,.F.) ;
#66943=ORIENTED_EDGE('',*,*,#48398,.T.) ;
#66944=ORIENTED_EDGE('',*,*,#48402,.F.) ;
#66945=ORIENTED_EDGE('',*,*,#47762,.F.) ;
#66946=ORIENTED_EDGE('',*,*,#48403,.T.) ;
#66947=ORIENTED_EDGE('',*,*,#48273,.F.) ;
#66948=ORIENTED_EDGE('',*,*,#48404,.F.) ;
#66949=ORIENTED_EDGE('',*,*,#48402,.T.) ;
#66950=ORIENTED_EDGE('',*,*,#47763,.F.) ;
#66951=ORIENTED_EDGE('',*,*,#48405,.F.) ;
#66952=ORIENTED_EDGE('',*,*,#47757,.F.) ;
#66953=ORIENTED_EDGE('',*,*,#48401,.T.) ;
#66954=ORIENTED_EDGE('',*,*,#47760,.F.) ;
#66955=ORIENTED_EDGE('',*,*,#48406,.F.) ;
#66956=ORIENTED_EDGE('',*,*,#48272,.F.) ;
#66957=ORIENTED_EDGE('',*,*,#48405,.T.) ;
#66958=ORIENTED_EDGE('',*,*,#48404,.T.) ;
#66959=ORIENTED_EDGE('',*,*,#48407,.F.) ;
#66960=ORIENTED_EDGE('',*,*,#48408,.F.) ;
#66961=ORIENTED_EDGE('',*,*,#48406,.T.) ;
#66962=ORIENTED_EDGE('',*,*,#48409,.F.) ;
#66963=ORIENTED_EDGE('',*,*,#48407,.T.) ;
#66964=ORIENTED_EDGE('',*,*,#48276,.F.) ;
#66965=ORIENTED_EDGE('',*,*,#48410,.F.) ;
#66966=ORIENTED_EDGE('',*,*,#47758,.F.) ;
#66967=ORIENTED_EDGE('',*,*,#48409,.T.) ;
#66968=ORIENTED_EDGE('',*,*,#47759,.F.) ;
#66969=ORIENTED_EDGE('',*,*,#48411,.F.) ;
#66970=ORIENTED_EDGE('',*,*,#47753,.F.) ;
#66971=ORIENTED_EDGE('',*,*,#47756,.F.) ;
#66972=ORIENTED_EDGE('',*,*,#48412,.T.) ;
#66973=ORIENTED_EDGE('',*,*,#48269,.F.) ;
#66974=ORIENTED_EDGE('',*,*,#48408,.T.) ;
#66975=ORIENTED_EDGE('',*,*,#48411,.T.) ;
#66976=ORIENTED_EDGE('',*,*,#48410,.T.) ;
#66977=ORIENTED_EDGE('',*,*,#48413,.F.) ;
#66978=ORIENTED_EDGE('',*,*,#47751,.F.) ;
#66979=ORIENTED_EDGE('',*,*,#48414,.T.) ;
#66980=ORIENTED_EDGE('',*,*,#47755,.F.) ;
#66981=ORIENTED_EDGE('',*,*,#48415,.T.) ;
#66982=ORIENTED_EDGE('',*,*,#48275,.F.) ;
#66983=ORIENTED_EDGE('',*,*,#48416,.T.) ;
#66984=ORIENTED_EDGE('',*,*,#47754,.F.) ;
#66985=ORIENTED_EDGE('',*,*,#48413,.T.) ;
#66986=ORIENTED_EDGE('',*,*,#48343,.F.) ;
#66987=ORIENTED_EDGE('',*,*,#48417,.T.) ;
#66988=ORIENTED_EDGE('',*,*,#47786,.F.) ;
#66989=ORIENTED_EDGE('',*,*,#48418,.F.) ;
#66990=ORIENTED_EDGE('',*,*,#47783,.F.) ;
#66991=ORIENTED_EDGE('',*,*,#48419,.T.) ;
#66992=ORIENTED_EDGE('',*,*,#47787,.F.) ;
#66993=ORIENTED_EDGE('',*,*,#48420,.T.) ;
#66994=ORIENTED_EDGE('',*,*,#48421,.F.) ;
#66995=ORIENTED_EDGE('',*,*,#48418,.T.) ;
#66996=ORIENTED_EDGE('',*,*,#48422,.F.) ;
#66997=ORIENTED_EDGE('',*,*,#47784,.F.) ;
#66998=ORIENTED_EDGE('',*,*,#48423,.T.) ;
#66999=ORIENTED_EDGE('',*,*,#48345,.F.) ;
#67000=ORIENTED_EDGE('',*,*,#48424,.F.) ;
#67001=ORIENTED_EDGE('',*,*,#48422,.T.) ;
#67002=ORIENTED_EDGE('',*,*,#47785,.F.) ;
#67003=ORIENTED_EDGE('',*,*,#48425,.F.) ;
#67004=ORIENTED_EDGE('',*,*,#47799,.F.) ;
#67005=ORIENTED_EDGE('',*,*,#48421,.T.) ;
#67006=ORIENTED_EDGE('',*,*,#47798,.F.) ;
#67007=ORIENTED_EDGE('',*,*,#48426,.F.) ;
#67008=ORIENTED_EDGE('',*,*,#48344,.F.) ;
#67009=ORIENTED_EDGE('',*,*,#48425,.T.) ;
#67010=ORIENTED_EDGE('',*,*,#48424,.T.) ;
#67011=ORIENTED_EDGE('',*,*,#48427,.F.) ;
#67012=ORIENTED_EDGE('',*,*,#48428,.F.) ;
#67013=ORIENTED_EDGE('',*,*,#48426,.T.) ;
#67014=ORIENTED_EDGE('',*,*,#48429,.F.) ;
#67015=ORIENTED_EDGE('',*,*,#48427,.T.) ;
#67016=ORIENTED_EDGE('',*,*,#48348,.F.) ;
#67017=ORIENTED_EDGE('',*,*,#48430,.F.) ;
#67018=ORIENTED_EDGE('',*,*,#47800,.F.) ;
#67019=ORIENTED_EDGE('',*,*,#48429,.T.) ;
#67020=ORIENTED_EDGE('',*,*,#47797,.F.) ;
#67021=ORIENTED_EDGE('',*,*,#48431,.F.) ;
#67022=ORIENTED_EDGE('',*,*,#47793,.F.) ;
#67023=ORIENTED_EDGE('',*,*,#47796,.F.) ;
#67024=ORIENTED_EDGE('',*,*,#48432,.T.) ;
#67025=ORIENTED_EDGE('',*,*,#48341,.F.) ;
#67026=ORIENTED_EDGE('',*,*,#48428,.T.) ;
#67027=ORIENTED_EDGE('',*,*,#48431,.T.) ;
#67028=ORIENTED_EDGE('',*,*,#48430,.T.) ;
#67029=ORIENTED_EDGE('',*,*,#48433,.F.) ;
#67030=ORIENTED_EDGE('',*,*,#47791,.F.) ;
#67031=ORIENTED_EDGE('',*,*,#48434,.T.) ;
#67032=ORIENTED_EDGE('',*,*,#47795,.F.) ;
#67033=ORIENTED_EDGE('',*,*,#48435,.T.) ;
#67034=ORIENTED_EDGE('',*,*,#48347,.F.) ;
#67035=ORIENTED_EDGE('',*,*,#48436,.T.) ;
#67036=ORIENTED_EDGE('',*,*,#47794,.F.) ;
#67037=ORIENTED_EDGE('',*,*,#48433,.T.) ;
#67038=ORIENTED_EDGE('',*,*,#48263,.F.) ;
#67039=ORIENTED_EDGE('',*,*,#48437,.T.) ;
#67040=ORIENTED_EDGE('',*,*,#47822,.F.) ;
#67041=ORIENTED_EDGE('',*,*,#48438,.F.) ;
#67042=ORIENTED_EDGE('',*,*,#47819,.F.) ;
#67043=ORIENTED_EDGE('',*,*,#48439,.T.) ;
#67044=ORIENTED_EDGE('',*,*,#47823,.F.) ;
#67045=ORIENTED_EDGE('',*,*,#48440,.T.) ;
#67046=ORIENTED_EDGE('',*,*,#48441,.F.) ;
#67047=ORIENTED_EDGE('',*,*,#48438,.T.) ;
#67048=ORIENTED_EDGE('',*,*,#48442,.F.) ;
#67049=ORIENTED_EDGE('',*,*,#47820,.F.) ;
#67050=ORIENTED_EDGE('',*,*,#48443,.T.) ;
#67051=ORIENTED_EDGE('',*,*,#48265,.F.) ;
#67052=ORIENTED_EDGE('',*,*,#48444,.F.) ;
#67053=ORIENTED_EDGE('',*,*,#48442,.T.) ;
#67054=ORIENTED_EDGE('',*,*,#47821,.F.) ;
#67055=ORIENTED_EDGE('',*,*,#48445,.F.) ;
#67056=ORIENTED_EDGE('',*,*,#47815,.F.) ;
#67057=ORIENTED_EDGE('',*,*,#48441,.T.) ;
#67058=ORIENTED_EDGE('',*,*,#47818,.F.) ;
#67059=ORIENTED_EDGE('',*,*,#48446,.F.) ;
#67060=ORIENTED_EDGE('',*,*,#48264,.F.) ;
#67061=ORIENTED_EDGE('',*,*,#48445,.T.) ;
#67062=ORIENTED_EDGE('',*,*,#48444,.T.) ;
#67063=ORIENTED_EDGE('',*,*,#48447,.F.) ;
#67064=ORIENTED_EDGE('',*,*,#48448,.F.) ;
#67065=ORIENTED_EDGE('',*,*,#48446,.T.) ;
#67066=ORIENTED_EDGE('',*,*,#48449,.F.) ;
#67067=ORIENTED_EDGE('',*,*,#48447,.T.) ;
#67068=ORIENTED_EDGE('',*,*,#48268,.F.) ;
#67069=ORIENTED_EDGE('',*,*,#48450,.F.) ;
#67070=ORIENTED_EDGE('',*,*,#47816,.F.) ;
#67071=ORIENTED_EDGE('',*,*,#48449,.T.) ;
#67072=ORIENTED_EDGE('',*,*,#47817,.F.) ;
#67073=ORIENTED_EDGE('',*,*,#48451,.F.) ;
#67074=ORIENTED_EDGE('',*,*,#47811,.F.) ;
#67075=ORIENTED_EDGE('',*,*,#47814,.F.) ;
#67076=ORIENTED_EDGE('',*,*,#48452,.T.) ;
#67077=ORIENTED_EDGE('',*,*,#48261,.F.) ;
#67078=ORIENTED_EDGE('',*,*,#48448,.T.) ;
#67079=ORIENTED_EDGE('',*,*,#48451,.T.) ;
#67080=ORIENTED_EDGE('',*,*,#48450,.T.) ;
#67081=ORIENTED_EDGE('',*,*,#48453,.F.) ;
#67082=ORIENTED_EDGE('',*,*,#47809,.F.) ;
#67083=ORIENTED_EDGE('',*,*,#48454,.T.) ;
#67084=ORIENTED_EDGE('',*,*,#47813,.F.) ;
#67085=ORIENTED_EDGE('',*,*,#48455,.T.) ;
#67086=ORIENTED_EDGE('',*,*,#48267,.F.) ;
#67087=ORIENTED_EDGE('',*,*,#48456,.T.) ;
#67088=ORIENTED_EDGE('',*,*,#47812,.F.) ;
#67089=ORIENTED_EDGE('',*,*,#48453,.T.) ;
#67090=ORIENTED_EDGE('',*,*,#48335,.F.) ;
#67091=ORIENTED_EDGE('',*,*,#48457,.T.) ;
#67092=ORIENTED_EDGE('',*,*,#47844,.F.) ;
#67093=ORIENTED_EDGE('',*,*,#48458,.F.) ;
#67094=ORIENTED_EDGE('',*,*,#47841,.F.) ;
#67095=ORIENTED_EDGE('',*,*,#48459,.T.) ;
#67096=ORIENTED_EDGE('',*,*,#47845,.F.) ;
#67097=ORIENTED_EDGE('',*,*,#48460,.T.) ;
#67098=ORIENTED_EDGE('',*,*,#48461,.F.) ;
#67099=ORIENTED_EDGE('',*,*,#48458,.T.) ;
#67100=ORIENTED_EDGE('',*,*,#48462,.F.) ;
#67101=ORIENTED_EDGE('',*,*,#47842,.F.) ;
#67102=ORIENTED_EDGE('',*,*,#48463,.T.) ;
#67103=ORIENTED_EDGE('',*,*,#48337,.F.) ;
#67104=ORIENTED_EDGE('',*,*,#48464,.F.) ;
#67105=ORIENTED_EDGE('',*,*,#48462,.T.) ;
#67106=ORIENTED_EDGE('',*,*,#47843,.F.) ;
#67107=ORIENTED_EDGE('',*,*,#48465,.F.) ;
#67108=ORIENTED_EDGE('',*,*,#47857,.F.) ;
#67109=ORIENTED_EDGE('',*,*,#48461,.T.) ;
#67110=ORIENTED_EDGE('',*,*,#47856,.F.) ;
#67111=ORIENTED_EDGE('',*,*,#48466,.F.) ;
#67112=ORIENTED_EDGE('',*,*,#48336,.F.) ;
#67113=ORIENTED_EDGE('',*,*,#48465,.T.) ;
#67114=ORIENTED_EDGE('',*,*,#48464,.T.) ;
#67115=ORIENTED_EDGE('',*,*,#48467,.F.) ;
#67116=ORIENTED_EDGE('',*,*,#48468,.F.) ;
#67117=ORIENTED_EDGE('',*,*,#48466,.T.) ;
#67118=ORIENTED_EDGE('',*,*,#48469,.F.) ;
#67119=ORIENTED_EDGE('',*,*,#48467,.T.) ;
#67120=ORIENTED_EDGE('',*,*,#48340,.F.) ;
#67121=ORIENTED_EDGE('',*,*,#48470,.F.) ;
#67122=ORIENTED_EDGE('',*,*,#47858,.F.) ;
#67123=ORIENTED_EDGE('',*,*,#48469,.T.) ;
#67124=ORIENTED_EDGE('',*,*,#47855,.F.) ;
#67125=ORIENTED_EDGE('',*,*,#48471,.F.) ;
#67126=ORIENTED_EDGE('',*,*,#47851,.F.) ;
#67127=ORIENTED_EDGE('',*,*,#47854,.F.) ;
#67128=ORIENTED_EDGE('',*,*,#48472,.T.) ;
#67129=ORIENTED_EDGE('',*,*,#48333,.F.) ;
#67130=ORIENTED_EDGE('',*,*,#48468,.T.) ;
#67131=ORIENTED_EDGE('',*,*,#48471,.T.) ;
#67132=ORIENTED_EDGE('',*,*,#48470,.T.) ;
#67133=ORIENTED_EDGE('',*,*,#48473,.F.) ;
#67134=ORIENTED_EDGE('',*,*,#47849,.F.) ;
#67135=ORIENTED_EDGE('',*,*,#48474,.T.) ;
#67136=ORIENTED_EDGE('',*,*,#47853,.F.) ;
#67137=ORIENTED_EDGE('',*,*,#48475,.T.) ;
#67138=ORIENTED_EDGE('',*,*,#48339,.F.) ;
#67139=ORIENTED_EDGE('',*,*,#48476,.T.) ;
#67140=ORIENTED_EDGE('',*,*,#47852,.F.) ;
#67141=ORIENTED_EDGE('',*,*,#48473,.T.) ;
#67142=ORIENTED_EDGE('',*,*,#48255,.F.) ;
#67143=ORIENTED_EDGE('',*,*,#48477,.T.) ;
#67144=ORIENTED_EDGE('',*,*,#47880,.F.) ;
#67145=ORIENTED_EDGE('',*,*,#48478,.F.) ;
#67146=ORIENTED_EDGE('',*,*,#47877,.F.) ;
#67147=ORIENTED_EDGE('',*,*,#48479,.T.) ;
#67148=ORIENTED_EDGE('',*,*,#47881,.F.) ;
#67149=ORIENTED_EDGE('',*,*,#48480,.T.) ;
#67150=ORIENTED_EDGE('',*,*,#48481,.F.) ;
#67151=ORIENTED_EDGE('',*,*,#48478,.T.) ;
#67152=ORIENTED_EDGE('',*,*,#48482,.F.) ;
#67153=ORIENTED_EDGE('',*,*,#47878,.F.) ;
#67154=ORIENTED_EDGE('',*,*,#48483,.T.) ;
#67155=ORIENTED_EDGE('',*,*,#48257,.F.) ;
#67156=ORIENTED_EDGE('',*,*,#48484,.F.) ;
#67157=ORIENTED_EDGE('',*,*,#48482,.T.) ;
#67158=ORIENTED_EDGE('',*,*,#47879,.F.) ;
#67159=ORIENTED_EDGE('',*,*,#48485,.F.) ;
#67160=ORIENTED_EDGE('',*,*,#47873,.F.) ;
#67161=ORIENTED_EDGE('',*,*,#48481,.T.) ;
#67162=ORIENTED_EDGE('',*,*,#47876,.F.) ;
#67163=ORIENTED_EDGE('',*,*,#48486,.F.) ;
#67164=ORIENTED_EDGE('',*,*,#48256,.F.) ;
#67165=ORIENTED_EDGE('',*,*,#48485,.T.) ;
#67166=ORIENTED_EDGE('',*,*,#48484,.T.) ;
#67167=ORIENTED_EDGE('',*,*,#48487,.F.) ;
#67168=ORIENTED_EDGE('',*,*,#48488,.F.) ;
#67169=ORIENTED_EDGE('',*,*,#48486,.T.) ;
#67170=ORIENTED_EDGE('',*,*,#48489,.F.) ;
#67171=ORIENTED_EDGE('',*,*,#48487,.T.) ;
#67172=ORIENTED_EDGE('',*,*,#48260,.F.) ;
#67173=ORIENTED_EDGE('',*,*,#48490,.F.) ;
#67174=ORIENTED_EDGE('',*,*,#47874,.F.) ;
#67175=ORIENTED_EDGE('',*,*,#48489,.T.) ;
#67176=ORIENTED_EDGE('',*,*,#47875,.F.) ;
#67177=ORIENTED_EDGE('',*,*,#48491,.F.) ;
#67178=ORIENTED_EDGE('',*,*,#47869,.F.) ;
#67179=ORIENTED_EDGE('',*,*,#47872,.F.) ;
#67180=ORIENTED_EDGE('',*,*,#48492,.T.) ;
#67181=ORIENTED_EDGE('',*,*,#48253,.F.) ;
#67182=ORIENTED_EDGE('',*,*,#48488,.T.) ;
#67183=ORIENTED_EDGE('',*,*,#48491,.T.) ;
#67184=ORIENTED_EDGE('',*,*,#48490,.T.) ;
#67185=ORIENTED_EDGE('',*,*,#48493,.F.) ;
#67186=ORIENTED_EDGE('',*,*,#47867,.F.) ;
#67187=ORIENTED_EDGE('',*,*,#48494,.T.) ;
#67188=ORIENTED_EDGE('',*,*,#47871,.F.) ;
#67189=ORIENTED_EDGE('',*,*,#48495,.T.) ;
#67190=ORIENTED_EDGE('',*,*,#48259,.F.) ;
#67191=ORIENTED_EDGE('',*,*,#48496,.T.) ;
#67192=ORIENTED_EDGE('',*,*,#47870,.F.) ;
#67193=ORIENTED_EDGE('',*,*,#48493,.T.) ;
#67194=ORIENTED_EDGE('',*,*,#48327,.F.) ;
#67195=ORIENTED_EDGE('',*,*,#48497,.T.) ;
#67196=ORIENTED_EDGE('',*,*,#47902,.F.) ;
#67197=ORIENTED_EDGE('',*,*,#48498,.F.) ;
#67198=ORIENTED_EDGE('',*,*,#47899,.F.) ;
#67199=ORIENTED_EDGE('',*,*,#48499,.T.) ;
#67200=ORIENTED_EDGE('',*,*,#47903,.F.) ;
#67201=ORIENTED_EDGE('',*,*,#48500,.T.) ;
#67202=ORIENTED_EDGE('',*,*,#48501,.F.) ;
#67203=ORIENTED_EDGE('',*,*,#48498,.T.) ;
#67204=ORIENTED_EDGE('',*,*,#48502,.F.) ;
#67205=ORIENTED_EDGE('',*,*,#47900,.F.) ;
#67206=ORIENTED_EDGE('',*,*,#48503,.T.) ;
#67207=ORIENTED_EDGE('',*,*,#48329,.F.) ;
#67208=ORIENTED_EDGE('',*,*,#48504,.F.) ;
#67209=ORIENTED_EDGE('',*,*,#48502,.T.) ;
#67210=ORIENTED_EDGE('',*,*,#47901,.F.) ;
#67211=ORIENTED_EDGE('',*,*,#48505,.F.) ;
#67212=ORIENTED_EDGE('',*,*,#47915,.F.) ;
#67213=ORIENTED_EDGE('',*,*,#48501,.T.) ;
#67214=ORIENTED_EDGE('',*,*,#47914,.F.) ;
#67215=ORIENTED_EDGE('',*,*,#48506,.F.) ;
#67216=ORIENTED_EDGE('',*,*,#48328,.F.) ;
#67217=ORIENTED_EDGE('',*,*,#48505,.T.) ;
#67218=ORIENTED_EDGE('',*,*,#48504,.T.) ;
#67219=ORIENTED_EDGE('',*,*,#48507,.F.) ;
#67220=ORIENTED_EDGE('',*,*,#48508,.F.) ;
#67221=ORIENTED_EDGE('',*,*,#48506,.T.) ;
#67222=ORIENTED_EDGE('',*,*,#48509,.F.) ;
#67223=ORIENTED_EDGE('',*,*,#48507,.T.) ;
#67224=ORIENTED_EDGE('',*,*,#48332,.F.) ;
#67225=ORIENTED_EDGE('',*,*,#48510,.F.) ;
#67226=ORIENTED_EDGE('',*,*,#47916,.F.) ;
#67227=ORIENTED_EDGE('',*,*,#48509,.T.) ;
#67228=ORIENTED_EDGE('',*,*,#47913,.F.) ;
#67229=ORIENTED_EDGE('',*,*,#48511,.F.) ;
#67230=ORIENTED_EDGE('',*,*,#47909,.F.) ;
#67231=ORIENTED_EDGE('',*,*,#47912,.F.) ;
#67232=ORIENTED_EDGE('',*,*,#48512,.T.) ;
#67233=ORIENTED_EDGE('',*,*,#48325,.F.) ;
#67234=ORIENTED_EDGE('',*,*,#48508,.T.) ;
#67235=ORIENTED_EDGE('',*,*,#48511,.T.) ;
#67236=ORIENTED_EDGE('',*,*,#48510,.T.) ;
#67237=ORIENTED_EDGE('',*,*,#48513,.F.) ;
#67238=ORIENTED_EDGE('',*,*,#47907,.F.) ;
#67239=ORIENTED_EDGE('',*,*,#48514,.T.) ;
#67240=ORIENTED_EDGE('',*,*,#47911,.F.) ;
#67241=ORIENTED_EDGE('',*,*,#48515,.T.) ;
#67242=ORIENTED_EDGE('',*,*,#48331,.F.) ;
#67243=ORIENTED_EDGE('',*,*,#48516,.T.) ;
#67244=ORIENTED_EDGE('',*,*,#47910,.F.) ;
#67245=ORIENTED_EDGE('',*,*,#48513,.T.) ;
#67246=ORIENTED_EDGE('',*,*,#48247,.F.) ;
#67247=ORIENTED_EDGE('',*,*,#48517,.T.) ;
#67248=ORIENTED_EDGE('',*,*,#47938,.F.) ;
#67249=ORIENTED_EDGE('',*,*,#48518,.F.) ;
#67250=ORIENTED_EDGE('',*,*,#47935,.F.) ;
#67251=ORIENTED_EDGE('',*,*,#48519,.T.) ;
#67252=ORIENTED_EDGE('',*,*,#47939,.F.) ;
#67253=ORIENTED_EDGE('',*,*,#48520,.T.) ;
#67254=ORIENTED_EDGE('',*,*,#48521,.F.) ;
#67255=ORIENTED_EDGE('',*,*,#48518,.T.) ;
#67256=ORIENTED_EDGE('',*,*,#48522,.F.) ;
#67257=ORIENTED_EDGE('',*,*,#47936,.F.) ;
#67258=ORIENTED_EDGE('',*,*,#48523,.T.) ;
#67259=ORIENTED_EDGE('',*,*,#48249,.F.) ;
#67260=ORIENTED_EDGE('',*,*,#48524,.F.) ;
#67261=ORIENTED_EDGE('',*,*,#48522,.T.) ;
#67262=ORIENTED_EDGE('',*,*,#47937,.F.) ;
#67263=ORIENTED_EDGE('',*,*,#48525,.F.) ;
#67264=ORIENTED_EDGE('',*,*,#47931,.F.) ;
#67265=ORIENTED_EDGE('',*,*,#48521,.T.) ;
#67266=ORIENTED_EDGE('',*,*,#47934,.F.) ;
#67267=ORIENTED_EDGE('',*,*,#48526,.F.) ;
#67268=ORIENTED_EDGE('',*,*,#48248,.F.) ;
#67269=ORIENTED_EDGE('',*,*,#48525,.T.) ;
#67270=ORIENTED_EDGE('',*,*,#48524,.T.) ;
#67271=ORIENTED_EDGE('',*,*,#48527,.F.) ;
#67272=ORIENTED_EDGE('',*,*,#48528,.F.) ;
#67273=ORIENTED_EDGE('',*,*,#48526,.T.) ;
#67274=ORIENTED_EDGE('',*,*,#48529,.F.) ;
#67275=ORIENTED_EDGE('',*,*,#48527,.T.) ;
#67276=ORIENTED_EDGE('',*,*,#48252,.F.) ;
#67277=ORIENTED_EDGE('',*,*,#48530,.F.) ;
#67278=ORIENTED_EDGE('',*,*,#47932,.F.) ;
#67279=ORIENTED_EDGE('',*,*,#48529,.T.) ;
#67280=ORIENTED_EDGE('',*,*,#47933,.F.) ;
#67281=ORIENTED_EDGE('',*,*,#48531,.F.) ;
#67282=ORIENTED_EDGE('',*,*,#47927,.F.) ;
#67283=ORIENTED_EDGE('',*,*,#47930,.F.) ;
#67284=ORIENTED_EDGE('',*,*,#48532,.T.) ;
#67285=ORIENTED_EDGE('',*,*,#48245,.F.) ;
#67286=ORIENTED_EDGE('',*,*,#48528,.T.) ;
#67287=ORIENTED_EDGE('',*,*,#48531,.T.) ;
#67288=ORIENTED_EDGE('',*,*,#48530,.T.) ;
#67289=ORIENTED_EDGE('',*,*,#48533,.F.) ;
#67290=ORIENTED_EDGE('',*,*,#47925,.F.) ;
#67291=ORIENTED_EDGE('',*,*,#48534,.T.) ;
#67292=ORIENTED_EDGE('',*,*,#47929,.F.) ;
#67293=ORIENTED_EDGE('',*,*,#48535,.T.) ;
#67294=ORIENTED_EDGE('',*,*,#48251,.F.) ;
#67295=ORIENTED_EDGE('',*,*,#48536,.T.) ;
#67296=ORIENTED_EDGE('',*,*,#47928,.F.) ;
#67297=ORIENTED_EDGE('',*,*,#48533,.T.) ;
#67298=ORIENTED_EDGE('',*,*,#48319,.F.) ;
#67299=ORIENTED_EDGE('',*,*,#48537,.T.) ;
#67300=ORIENTED_EDGE('',*,*,#47960,.F.) ;
#67301=ORIENTED_EDGE('',*,*,#48538,.F.) ;
#67302=ORIENTED_EDGE('',*,*,#47957,.F.) ;
#67303=ORIENTED_EDGE('',*,*,#48539,.T.) ;
#67304=ORIENTED_EDGE('',*,*,#47961,.F.) ;
#67305=ORIENTED_EDGE('',*,*,#48540,.T.) ;
#67306=ORIENTED_EDGE('',*,*,#48541,.F.) ;
#67307=ORIENTED_EDGE('',*,*,#48538,.T.) ;
#67308=ORIENTED_EDGE('',*,*,#48542,.F.) ;
#67309=ORIENTED_EDGE('',*,*,#47958,.F.) ;
#67310=ORIENTED_EDGE('',*,*,#48543,.T.) ;
#67311=ORIENTED_EDGE('',*,*,#48321,.F.) ;
#67312=ORIENTED_EDGE('',*,*,#48544,.F.) ;
#67313=ORIENTED_EDGE('',*,*,#48542,.T.) ;
#67314=ORIENTED_EDGE('',*,*,#47959,.F.) ;
#67315=ORIENTED_EDGE('',*,*,#48545,.F.) ;
#67316=ORIENTED_EDGE('',*,*,#47973,.F.) ;
#67317=ORIENTED_EDGE('',*,*,#48541,.T.) ;
#67318=ORIENTED_EDGE('',*,*,#47972,.F.) ;
#67319=ORIENTED_EDGE('',*,*,#48546,.F.) ;
#67320=ORIENTED_EDGE('',*,*,#48320,.F.) ;
#67321=ORIENTED_EDGE('',*,*,#48545,.T.) ;
#67322=ORIENTED_EDGE('',*,*,#48544,.T.) ;
#67323=ORIENTED_EDGE('',*,*,#48547,.F.) ;
#67324=ORIENTED_EDGE('',*,*,#48548,.F.) ;
#67325=ORIENTED_EDGE('',*,*,#48546,.T.) ;
#67326=ORIENTED_EDGE('',*,*,#48549,.F.) ;
#67327=ORIENTED_EDGE('',*,*,#48547,.T.) ;
#67328=ORIENTED_EDGE('',*,*,#48324,.F.) ;
#67329=ORIENTED_EDGE('',*,*,#48550,.F.) ;
#67330=ORIENTED_EDGE('',*,*,#47974,.F.) ;
#67331=ORIENTED_EDGE('',*,*,#48549,.T.) ;
#67332=ORIENTED_EDGE('',*,*,#47971,.F.) ;
#67333=ORIENTED_EDGE('',*,*,#48551,.F.) ;
#67334=ORIENTED_EDGE('',*,*,#47967,.F.) ;
#67335=ORIENTED_EDGE('',*,*,#47970,.F.) ;
#67336=ORIENTED_EDGE('',*,*,#48552,.T.) ;
#67337=ORIENTED_EDGE('',*,*,#48317,.F.) ;
#67338=ORIENTED_EDGE('',*,*,#48548,.T.) ;
#67339=ORIENTED_EDGE('',*,*,#48551,.T.) ;
#67340=ORIENTED_EDGE('',*,*,#48550,.T.) ;
#67341=ORIENTED_EDGE('',*,*,#48553,.F.) ;
#67342=ORIENTED_EDGE('',*,*,#47965,.F.) ;
#67343=ORIENTED_EDGE('',*,*,#48554,.T.) ;
#67344=ORIENTED_EDGE('',*,*,#47969,.F.) ;
#67345=ORIENTED_EDGE('',*,*,#48555,.T.) ;
#67346=ORIENTED_EDGE('',*,*,#48323,.F.) ;
#67347=ORIENTED_EDGE('',*,*,#48556,.T.) ;
#67348=ORIENTED_EDGE('',*,*,#47968,.F.) ;
#67349=ORIENTED_EDGE('',*,*,#48553,.T.) ;
#67350=ORIENTED_EDGE('',*,*,#48239,.F.) ;
#67351=ORIENTED_EDGE('',*,*,#48557,.T.) ;
#67352=ORIENTED_EDGE('',*,*,#47996,.F.) ;
#67353=ORIENTED_EDGE('',*,*,#48558,.F.) ;
#67354=ORIENTED_EDGE('',*,*,#47993,.F.) ;
#67355=ORIENTED_EDGE('',*,*,#48559,.T.) ;
#67356=ORIENTED_EDGE('',*,*,#47997,.F.) ;
#67357=ORIENTED_EDGE('',*,*,#48560,.T.) ;
#67358=ORIENTED_EDGE('',*,*,#48561,.F.) ;
#67359=ORIENTED_EDGE('',*,*,#48558,.T.) ;
#67360=ORIENTED_EDGE('',*,*,#48562,.F.) ;
#67361=ORIENTED_EDGE('',*,*,#47994,.F.) ;
#67362=ORIENTED_EDGE('',*,*,#48563,.T.) ;
#67363=ORIENTED_EDGE('',*,*,#48241,.F.) ;
#67364=ORIENTED_EDGE('',*,*,#48564,.F.) ;
#67365=ORIENTED_EDGE('',*,*,#48562,.T.) ;
#67366=ORIENTED_EDGE('',*,*,#47995,.F.) ;
#67367=ORIENTED_EDGE('',*,*,#48565,.F.) ;
#67368=ORIENTED_EDGE('',*,*,#47989,.F.) ;
#67369=ORIENTED_EDGE('',*,*,#48561,.T.) ;
#67370=ORIENTED_EDGE('',*,*,#47992,.F.) ;
#67371=ORIENTED_EDGE('',*,*,#48566,.F.) ;
#67372=ORIENTED_EDGE('',*,*,#48240,.F.) ;
#67373=ORIENTED_EDGE('',*,*,#48565,.T.) ;
#67374=ORIENTED_EDGE('',*,*,#48564,.T.) ;
#67375=ORIENTED_EDGE('',*,*,#48567,.F.) ;
#67376=ORIENTED_EDGE('',*,*,#48568,.F.) ;
#67377=ORIENTED_EDGE('',*,*,#48566,.T.) ;
#67378=ORIENTED_EDGE('',*,*,#48569,.F.) ;
#67379=ORIENTED_EDGE('',*,*,#48567,.T.) ;
#67380=ORIENTED_EDGE('',*,*,#48244,.F.) ;
#67381=ORIENTED_EDGE('',*,*,#48570,.F.) ;
#67382=ORIENTED_EDGE('',*,*,#47990,.F.) ;
#67383=ORIENTED_EDGE('',*,*,#48569,.T.) ;
#67384=ORIENTED_EDGE('',*,*,#47991,.F.) ;
#67385=ORIENTED_EDGE('',*,*,#48571,.F.) ;
#67386=ORIENTED_EDGE('',*,*,#47985,.F.) ;
#67387=ORIENTED_EDGE('',*,*,#47988,.F.) ;
#67388=ORIENTED_EDGE('',*,*,#48572,.T.) ;
#67389=ORIENTED_EDGE('',*,*,#48237,.F.) ;
#67390=ORIENTED_EDGE('',*,*,#48568,.T.) ;
#67391=ORIENTED_EDGE('',*,*,#48571,.T.) ;
#67392=ORIENTED_EDGE('',*,*,#48570,.T.) ;
#67393=ORIENTED_EDGE('',*,*,#48573,.F.) ;
#67394=ORIENTED_EDGE('',*,*,#47983,.F.) ;
#67395=ORIENTED_EDGE('',*,*,#48574,.T.) ;
#67396=ORIENTED_EDGE('',*,*,#47987,.F.) ;
#67397=ORIENTED_EDGE('',*,*,#48575,.T.) ;
#67398=ORIENTED_EDGE('',*,*,#48243,.F.) ;
#67399=ORIENTED_EDGE('',*,*,#48576,.T.) ;
#67400=ORIENTED_EDGE('',*,*,#47986,.F.) ;
#67401=ORIENTED_EDGE('',*,*,#48573,.T.) ;
#67402=ORIENTED_EDGE('',*,*,#48311,.F.) ;
#67403=ORIENTED_EDGE('',*,*,#48577,.T.) ;
#67404=ORIENTED_EDGE('',*,*,#48018,.F.) ;
#67405=ORIENTED_EDGE('',*,*,#48578,.F.) ;
#67406=ORIENTED_EDGE('',*,*,#48015,.F.) ;
#67407=ORIENTED_EDGE('',*,*,#48579,.T.) ;
#67408=ORIENTED_EDGE('',*,*,#48019,.F.) ;
#67409=ORIENTED_EDGE('',*,*,#48580,.T.) ;
#67410=ORIENTED_EDGE('',*,*,#48581,.F.) ;
#67411=ORIENTED_EDGE('',*,*,#48578,.T.) ;
#67412=ORIENTED_EDGE('',*,*,#48582,.F.) ;
#67413=ORIENTED_EDGE('',*,*,#48016,.F.) ;
#67414=ORIENTED_EDGE('',*,*,#48583,.T.) ;
#67415=ORIENTED_EDGE('',*,*,#48313,.F.) ;
#67416=ORIENTED_EDGE('',*,*,#48584,.F.) ;
#67417=ORIENTED_EDGE('',*,*,#48582,.T.) ;
#67418=ORIENTED_EDGE('',*,*,#48017,.F.) ;
#67419=ORIENTED_EDGE('',*,*,#48585,.F.) ;
#67420=ORIENTED_EDGE('',*,*,#48031,.F.) ;
#67421=ORIENTED_EDGE('',*,*,#48581,.T.) ;
#67422=ORIENTED_EDGE('',*,*,#48030,.F.) ;
#67423=ORIENTED_EDGE('',*,*,#48586,.F.) ;
#67424=ORIENTED_EDGE('',*,*,#48312,.F.) ;
#67425=ORIENTED_EDGE('',*,*,#48585,.T.) ;
#67426=ORIENTED_EDGE('',*,*,#48584,.T.) ;
#67427=ORIENTED_EDGE('',*,*,#48587,.F.) ;
#67428=ORIENTED_EDGE('',*,*,#48588,.F.) ;
#67429=ORIENTED_EDGE('',*,*,#48586,.T.) ;
#67430=ORIENTED_EDGE('',*,*,#48589,.F.) ;
#67431=ORIENTED_EDGE('',*,*,#48587,.T.) ;
#67432=ORIENTED_EDGE('',*,*,#48316,.F.) ;
#67433=ORIENTED_EDGE('',*,*,#48590,.F.) ;
#67434=ORIENTED_EDGE('',*,*,#48032,.F.) ;
#67435=ORIENTED_EDGE('',*,*,#48589,.T.) ;
#67436=ORIENTED_EDGE('',*,*,#48029,.F.) ;
#67437=ORIENTED_EDGE('',*,*,#48591,.F.) ;
#67438=ORIENTED_EDGE('',*,*,#48025,.F.) ;
#67439=ORIENTED_EDGE('',*,*,#48028,.F.) ;
#67440=ORIENTED_EDGE('',*,*,#48592,.T.) ;
#67441=ORIENTED_EDGE('',*,*,#48309,.F.) ;
#67442=ORIENTED_EDGE('',*,*,#48588,.T.) ;
#67443=ORIENTED_EDGE('',*,*,#48591,.T.) ;
#67444=ORIENTED_EDGE('',*,*,#48590,.T.) ;
#67445=ORIENTED_EDGE('',*,*,#48593,.F.) ;
#67446=ORIENTED_EDGE('',*,*,#48023,.F.) ;
#67447=ORIENTED_EDGE('',*,*,#48594,.T.) ;
#67448=ORIENTED_EDGE('',*,*,#48027,.F.) ;
#67449=ORIENTED_EDGE('',*,*,#48595,.T.) ;
#67450=ORIENTED_EDGE('',*,*,#48315,.F.) ;
#67451=ORIENTED_EDGE('',*,*,#48596,.T.) ;
#67452=ORIENTED_EDGE('',*,*,#48026,.F.) ;
#67453=ORIENTED_EDGE('',*,*,#48593,.T.) ;
#67454=ORIENTED_EDGE('',*,*,#48231,.F.) ;
#67455=ORIENTED_EDGE('',*,*,#48597,.T.) ;
#67456=ORIENTED_EDGE('',*,*,#48054,.F.) ;
#67457=ORIENTED_EDGE('',*,*,#48598,.F.) ;
#67458=ORIENTED_EDGE('',*,*,#48051,.F.) ;
#67459=ORIENTED_EDGE('',*,*,#48599,.T.) ;
#67460=ORIENTED_EDGE('',*,*,#48055,.F.) ;
#67461=ORIENTED_EDGE('',*,*,#48600,.T.) ;
#67462=ORIENTED_EDGE('',*,*,#48601,.F.) ;
#67463=ORIENTED_EDGE('',*,*,#48598,.T.) ;
#67464=ORIENTED_EDGE('',*,*,#48602,.F.) ;
#67465=ORIENTED_EDGE('',*,*,#48052,.F.) ;
#67466=ORIENTED_EDGE('',*,*,#48603,.T.) ;
#67467=ORIENTED_EDGE('',*,*,#48233,.F.) ;
#67468=ORIENTED_EDGE('',*,*,#48604,.F.) ;
#67469=ORIENTED_EDGE('',*,*,#48602,.T.) ;
#67470=ORIENTED_EDGE('',*,*,#48053,.F.) ;
#67471=ORIENTED_EDGE('',*,*,#48605,.F.) ;
#67472=ORIENTED_EDGE('',*,*,#48047,.F.) ;
#67473=ORIENTED_EDGE('',*,*,#48601,.T.) ;
#67474=ORIENTED_EDGE('',*,*,#48050,.F.) ;
#67475=ORIENTED_EDGE('',*,*,#48606,.F.) ;
#67476=ORIENTED_EDGE('',*,*,#48232,.F.) ;
#67477=ORIENTED_EDGE('',*,*,#48605,.T.) ;
#67478=ORIENTED_EDGE('',*,*,#48604,.T.) ;
#67479=ORIENTED_EDGE('',*,*,#48607,.F.) ;
#67480=ORIENTED_EDGE('',*,*,#48608,.F.) ;
#67481=ORIENTED_EDGE('',*,*,#48606,.T.) ;
#67482=ORIENTED_EDGE('',*,*,#48609,.F.) ;
#67483=ORIENTED_EDGE('',*,*,#48607,.T.) ;
#67484=ORIENTED_EDGE('',*,*,#48236,.F.) ;
#67485=ORIENTED_EDGE('',*,*,#48610,.F.) ;
#67486=ORIENTED_EDGE('',*,*,#48048,.F.) ;
#67487=ORIENTED_EDGE('',*,*,#48609,.T.) ;
#67488=ORIENTED_EDGE('',*,*,#48049,.F.) ;
#67489=ORIENTED_EDGE('',*,*,#48611,.F.) ;
#67490=ORIENTED_EDGE('',*,*,#48043,.F.) ;
#67491=ORIENTED_EDGE('',*,*,#48046,.F.) ;
#67492=ORIENTED_EDGE('',*,*,#48612,.T.) ;
#67493=ORIENTED_EDGE('',*,*,#48229,.F.) ;
#67494=ORIENTED_EDGE('',*,*,#48608,.T.) ;
#67495=ORIENTED_EDGE('',*,*,#48611,.T.) ;
#67496=ORIENTED_EDGE('',*,*,#48610,.T.) ;
#67497=ORIENTED_EDGE('',*,*,#48613,.F.) ;
#67498=ORIENTED_EDGE('',*,*,#48041,.F.) ;
#67499=ORIENTED_EDGE('',*,*,#48614,.T.) ;
#67500=ORIENTED_EDGE('',*,*,#48045,.F.) ;
#67501=ORIENTED_EDGE('',*,*,#48615,.T.) ;
#67502=ORIENTED_EDGE('',*,*,#48235,.F.) ;
#67503=ORIENTED_EDGE('',*,*,#48616,.T.) ;
#67504=ORIENTED_EDGE('',*,*,#48044,.F.) ;
#67505=ORIENTED_EDGE('',*,*,#48613,.T.) ;
#67506=ORIENTED_EDGE('',*,*,#48303,.F.) ;
#67507=ORIENTED_EDGE('',*,*,#48617,.T.) ;
#67508=ORIENTED_EDGE('',*,*,#48076,.F.) ;
#67509=ORIENTED_EDGE('',*,*,#48618,.F.) ;
#67510=ORIENTED_EDGE('',*,*,#48073,.F.) ;
#67511=ORIENTED_EDGE('',*,*,#48619,.T.) ;
#67512=ORIENTED_EDGE('',*,*,#48077,.F.) ;
#67513=ORIENTED_EDGE('',*,*,#48620,.T.) ;
#67514=ORIENTED_EDGE('',*,*,#48621,.F.) ;
#67515=ORIENTED_EDGE('',*,*,#48618,.T.) ;
#67516=ORIENTED_EDGE('',*,*,#48622,.F.) ;
#67517=ORIENTED_EDGE('',*,*,#48074,.F.) ;
#67518=ORIENTED_EDGE('',*,*,#48623,.T.) ;
#67519=ORIENTED_EDGE('',*,*,#48305,.F.) ;
#67520=ORIENTED_EDGE('',*,*,#48624,.F.) ;
#67521=ORIENTED_EDGE('',*,*,#48622,.T.) ;
#67522=ORIENTED_EDGE('',*,*,#48075,.F.) ;
#67523=ORIENTED_EDGE('',*,*,#48625,.F.) ;
#67524=ORIENTED_EDGE('',*,*,#48089,.F.) ;
#67525=ORIENTED_EDGE('',*,*,#48621,.T.) ;
#67526=ORIENTED_EDGE('',*,*,#48088,.F.) ;
#67527=ORIENTED_EDGE('',*,*,#48626,.F.) ;
#67528=ORIENTED_EDGE('',*,*,#48304,.F.) ;
#67529=ORIENTED_EDGE('',*,*,#48625,.T.) ;
#67530=ORIENTED_EDGE('',*,*,#48624,.T.) ;
#67531=ORIENTED_EDGE('',*,*,#48627,.F.) ;
#67532=ORIENTED_EDGE('',*,*,#48628,.F.) ;
#67533=ORIENTED_EDGE('',*,*,#48626,.T.) ;
#67534=ORIENTED_EDGE('',*,*,#48629,.F.) ;
#67535=ORIENTED_EDGE('',*,*,#48627,.T.) ;
#67536=ORIENTED_EDGE('',*,*,#48308,.F.) ;
#67537=ORIENTED_EDGE('',*,*,#48630,.F.) ;
#67538=ORIENTED_EDGE('',*,*,#48090,.F.) ;
#67539=ORIENTED_EDGE('',*,*,#48629,.T.) ;
#67540=ORIENTED_EDGE('',*,*,#48087,.F.) ;
#67541=ORIENTED_EDGE('',*,*,#48631,.F.) ;
#67542=ORIENTED_EDGE('',*,*,#48083,.F.) ;
#67543=ORIENTED_EDGE('',*,*,#48086,.F.) ;
#67544=ORIENTED_EDGE('',*,*,#48632,.T.) ;
#67545=ORIENTED_EDGE('',*,*,#48301,.F.) ;
#67546=ORIENTED_EDGE('',*,*,#48628,.T.) ;
#67547=ORIENTED_EDGE('',*,*,#48631,.T.) ;
#67548=ORIENTED_EDGE('',*,*,#48630,.T.) ;
#67549=ORIENTED_EDGE('',*,*,#48633,.F.) ;
#67550=ORIENTED_EDGE('',*,*,#48081,.F.) ;
#67551=ORIENTED_EDGE('',*,*,#48634,.T.) ;
#67552=ORIENTED_EDGE('',*,*,#48085,.F.) ;
#67553=ORIENTED_EDGE('',*,*,#48635,.T.) ;
#67554=ORIENTED_EDGE('',*,*,#48307,.F.) ;
#67555=ORIENTED_EDGE('',*,*,#48636,.T.) ;
#67556=ORIENTED_EDGE('',*,*,#48084,.F.) ;
#67557=ORIENTED_EDGE('',*,*,#48633,.T.) ;
#67558=ORIENTED_EDGE('',*,*,#48223,.F.) ;
#67559=ORIENTED_EDGE('',*,*,#48637,.T.) ;
#67560=ORIENTED_EDGE('',*,*,#48112,.F.) ;
#67561=ORIENTED_EDGE('',*,*,#48638,.F.) ;
#67562=ORIENTED_EDGE('',*,*,#48109,.F.) ;
#67563=ORIENTED_EDGE('',*,*,#48639,.T.) ;
#67564=ORIENTED_EDGE('',*,*,#48113,.F.) ;
#67565=ORIENTED_EDGE('',*,*,#48640,.T.) ;
#67566=ORIENTED_EDGE('',*,*,#48641,.F.) ;
#67567=ORIENTED_EDGE('',*,*,#48638,.T.) ;
#67568=ORIENTED_EDGE('',*,*,#48642,.F.) ;
#67569=ORIENTED_EDGE('',*,*,#48110,.F.) ;
#67570=ORIENTED_EDGE('',*,*,#48643,.T.) ;
#67571=ORIENTED_EDGE('',*,*,#48225,.F.) ;
#67572=ORIENTED_EDGE('',*,*,#48644,.F.) ;
#67573=ORIENTED_EDGE('',*,*,#48642,.T.) ;
#67574=ORIENTED_EDGE('',*,*,#48111,.F.) ;
#67575=ORIENTED_EDGE('',*,*,#48645,.F.) ;
#67576=ORIENTED_EDGE('',*,*,#48105,.F.) ;
#67577=ORIENTED_EDGE('',*,*,#48641,.T.) ;
#67578=ORIENTED_EDGE('',*,*,#48108,.F.) ;
#67579=ORIENTED_EDGE('',*,*,#48646,.F.) ;
#67580=ORIENTED_EDGE('',*,*,#48224,.F.) ;
#67581=ORIENTED_EDGE('',*,*,#48645,.T.) ;
#67582=ORIENTED_EDGE('',*,*,#48644,.T.) ;
#67583=ORIENTED_EDGE('',*,*,#48647,.F.) ;
#67584=ORIENTED_EDGE('',*,*,#48648,.F.) ;
#67585=ORIENTED_EDGE('',*,*,#48646,.T.) ;
#67586=ORIENTED_EDGE('',*,*,#48649,.F.) ;
#67587=ORIENTED_EDGE('',*,*,#48647,.T.) ;
#67588=ORIENTED_EDGE('',*,*,#48228,.F.) ;
#67589=ORIENTED_EDGE('',*,*,#48650,.F.) ;
#67590=ORIENTED_EDGE('',*,*,#48106,.F.) ;
#67591=ORIENTED_EDGE('',*,*,#48649,.T.) ;
#67592=ORIENTED_EDGE('',*,*,#48107,.F.) ;
#67593=ORIENTED_EDGE('',*,*,#48651,.F.) ;
#67594=ORIENTED_EDGE('',*,*,#48101,.F.) ;
#67595=ORIENTED_EDGE('',*,*,#48104,.F.) ;
#67596=ORIENTED_EDGE('',*,*,#48652,.T.) ;
#67597=ORIENTED_EDGE('',*,*,#48221,.F.) ;
#67598=ORIENTED_EDGE('',*,*,#48648,.T.) ;
#67599=ORIENTED_EDGE('',*,*,#48651,.T.) ;
#67600=ORIENTED_EDGE('',*,*,#48650,.T.) ;
#67601=ORIENTED_EDGE('',*,*,#48653,.F.) ;
#67602=ORIENTED_EDGE('',*,*,#48099,.F.) ;
#67603=ORIENTED_EDGE('',*,*,#48654,.T.) ;
#67604=ORIENTED_EDGE('',*,*,#48103,.F.) ;
#67605=ORIENTED_EDGE('',*,*,#48655,.T.) ;
#67606=ORIENTED_EDGE('',*,*,#48227,.F.) ;
#67607=ORIENTED_EDGE('',*,*,#48656,.T.) ;
#67608=ORIENTED_EDGE('',*,*,#48102,.F.) ;
#67609=ORIENTED_EDGE('',*,*,#48653,.T.) ;
#67610=ORIENTED_EDGE('',*,*,#48295,.F.) ;
#67611=ORIENTED_EDGE('',*,*,#48657,.T.) ;
#67612=ORIENTED_EDGE('',*,*,#48134,.F.) ;
#67613=ORIENTED_EDGE('',*,*,#48658,.F.) ;
#67614=ORIENTED_EDGE('',*,*,#48131,.F.) ;
#67615=ORIENTED_EDGE('',*,*,#48659,.T.) ;
#67616=ORIENTED_EDGE('',*,*,#48135,.F.) ;
#67617=ORIENTED_EDGE('',*,*,#48660,.T.) ;
#67618=ORIENTED_EDGE('',*,*,#48661,.F.) ;
#67619=ORIENTED_EDGE('',*,*,#48658,.T.) ;
#67620=ORIENTED_EDGE('',*,*,#48662,.F.) ;
#67621=ORIENTED_EDGE('',*,*,#48132,.F.) ;
#67622=ORIENTED_EDGE('',*,*,#48663,.T.) ;
#67623=ORIENTED_EDGE('',*,*,#48297,.F.) ;
#67624=ORIENTED_EDGE('',*,*,#48664,.F.) ;
#67625=ORIENTED_EDGE('',*,*,#48662,.T.) ;
#67626=ORIENTED_EDGE('',*,*,#48133,.F.) ;
#67627=ORIENTED_EDGE('',*,*,#48665,.F.) ;
#67628=ORIENTED_EDGE('',*,*,#48147,.F.) ;
#67629=ORIENTED_EDGE('',*,*,#48661,.T.) ;
#67630=ORIENTED_EDGE('',*,*,#48146,.F.) ;
#67631=ORIENTED_EDGE('',*,*,#48666,.F.) ;
#67632=ORIENTED_EDGE('',*,*,#48296,.F.) ;
#67633=ORIENTED_EDGE('',*,*,#48665,.T.) ;
#67634=ORIENTED_EDGE('',*,*,#48664,.T.) ;
#67635=ORIENTED_EDGE('',*,*,#48667,.F.) ;
#67636=ORIENTED_EDGE('',*,*,#48668,.F.) ;
#67637=ORIENTED_EDGE('',*,*,#48666,.T.) ;
#67638=ORIENTED_EDGE('',*,*,#48669,.F.) ;
#67639=ORIENTED_EDGE('',*,*,#48667,.T.) ;
#67640=ORIENTED_EDGE('',*,*,#48300,.F.) ;
#67641=ORIENTED_EDGE('',*,*,#48670,.F.) ;
#67642=ORIENTED_EDGE('',*,*,#48148,.F.) ;
#67643=ORIENTED_EDGE('',*,*,#48669,.T.) ;
#67644=ORIENTED_EDGE('',*,*,#48145,.F.) ;
#67645=ORIENTED_EDGE('',*,*,#48671,.F.) ;
#67646=ORIENTED_EDGE('',*,*,#48141,.F.) ;
#67647=ORIENTED_EDGE('',*,*,#48144,.F.) ;
#67648=ORIENTED_EDGE('',*,*,#48672,.T.) ;
#67649=ORIENTED_EDGE('',*,*,#48293,.F.) ;
#67650=ORIENTED_EDGE('',*,*,#48668,.T.) ;
#67651=ORIENTED_EDGE('',*,*,#48671,.T.) ;
#67652=ORIENTED_EDGE('',*,*,#48670,.T.) ;
#67653=ORIENTED_EDGE('',*,*,#48673,.F.) ;
#67654=ORIENTED_EDGE('',*,*,#48139,.F.) ;
#67655=ORIENTED_EDGE('',*,*,#48674,.T.) ;
#67656=ORIENTED_EDGE('',*,*,#48143,.F.) ;
#67657=ORIENTED_EDGE('',*,*,#48675,.T.) ;
#67658=ORIENTED_EDGE('',*,*,#48299,.F.) ;
#67659=ORIENTED_EDGE('',*,*,#48676,.T.) ;
#67660=ORIENTED_EDGE('',*,*,#48142,.F.) ;
#67661=ORIENTED_EDGE('',*,*,#48673,.T.) ;
#67662=ORIENTED_EDGE('',*,*,#48215,.F.) ;
#67663=ORIENTED_EDGE('',*,*,#48677,.T.) ;
#67664=ORIENTED_EDGE('',*,*,#48170,.F.) ;
#67665=ORIENTED_EDGE('',*,*,#48678,.F.) ;
#67666=ORIENTED_EDGE('',*,*,#48167,.F.) ;
#67667=ORIENTED_EDGE('',*,*,#48679,.T.) ;
#67668=ORIENTED_EDGE('',*,*,#48171,.F.) ;
#67669=ORIENTED_EDGE('',*,*,#48680,.T.) ;
#67670=ORIENTED_EDGE('',*,*,#48681,.F.) ;
#67671=ORIENTED_EDGE('',*,*,#48678,.T.) ;
#67672=ORIENTED_EDGE('',*,*,#48682,.F.) ;
#67673=ORIENTED_EDGE('',*,*,#48168,.F.) ;
#67674=ORIENTED_EDGE('',*,*,#48683,.T.) ;
#67675=ORIENTED_EDGE('',*,*,#48217,.F.) ;
#67676=ORIENTED_EDGE('',*,*,#48684,.F.) ;
#67677=ORIENTED_EDGE('',*,*,#48682,.T.) ;
#67678=ORIENTED_EDGE('',*,*,#48169,.F.) ;
#67679=ORIENTED_EDGE('',*,*,#48685,.F.) ;
#67680=ORIENTED_EDGE('',*,*,#48163,.F.) ;
#67681=ORIENTED_EDGE('',*,*,#48681,.T.) ;
#67682=ORIENTED_EDGE('',*,*,#48166,.F.) ;
#67683=ORIENTED_EDGE('',*,*,#48686,.F.) ;
#67684=ORIENTED_EDGE('',*,*,#48216,.F.) ;
#67685=ORIENTED_EDGE('',*,*,#48685,.T.) ;
#67686=ORIENTED_EDGE('',*,*,#48684,.T.) ;
#67687=ORIENTED_EDGE('',*,*,#48687,.F.) ;
#67688=ORIENTED_EDGE('',*,*,#48688,.F.) ;
#67689=ORIENTED_EDGE('',*,*,#48686,.T.) ;
#67690=ORIENTED_EDGE('',*,*,#48689,.F.) ;
#67691=ORIENTED_EDGE('',*,*,#48687,.T.) ;
#67692=ORIENTED_EDGE('',*,*,#48220,.F.) ;
#67693=ORIENTED_EDGE('',*,*,#48690,.F.) ;
#67694=ORIENTED_EDGE('',*,*,#48164,.F.) ;
#67695=ORIENTED_EDGE('',*,*,#48689,.T.) ;
#67696=ORIENTED_EDGE('',*,*,#48165,.F.) ;
#67697=ORIENTED_EDGE('',*,*,#48691,.F.) ;
#67698=ORIENTED_EDGE('',*,*,#48159,.F.) ;
#67699=ORIENTED_EDGE('',*,*,#48162,.F.) ;
#67700=ORIENTED_EDGE('',*,*,#48692,.T.) ;
#67701=ORIENTED_EDGE('',*,*,#48213,.F.) ;
#67702=ORIENTED_EDGE('',*,*,#48688,.T.) ;
#67703=ORIENTED_EDGE('',*,*,#48691,.T.) ;
#67704=ORIENTED_EDGE('',*,*,#48690,.T.) ;
#67705=ORIENTED_EDGE('',*,*,#48693,.F.) ;
#67706=ORIENTED_EDGE('',*,*,#48157,.F.) ;
#67707=ORIENTED_EDGE('',*,*,#48694,.T.) ;
#67708=ORIENTED_EDGE('',*,*,#48161,.F.) ;
#67709=ORIENTED_EDGE('',*,*,#48695,.T.) ;
#67710=ORIENTED_EDGE('',*,*,#48219,.F.) ;
#67711=ORIENTED_EDGE('',*,*,#48696,.T.) ;
#67712=ORIENTED_EDGE('',*,*,#48160,.F.) ;
#67713=ORIENTED_EDGE('',*,*,#48693,.T.) ;
#67714=ORIENTED_EDGE('',*,*,#48287,.F.) ;
#67715=ORIENTED_EDGE('',*,*,#48697,.T.) ;
#67716=ORIENTED_EDGE('',*,*,#48192,.F.) ;
#67717=ORIENTED_EDGE('',*,*,#48698,.F.) ;
#67718=ORIENTED_EDGE('',*,*,#48189,.F.) ;
#67719=ORIENTED_EDGE('',*,*,#48699,.T.) ;
#67720=ORIENTED_EDGE('',*,*,#48193,.F.) ;
#67721=ORIENTED_EDGE('',*,*,#48700,.T.) ;
#67722=ORIENTED_EDGE('',*,*,#48701,.F.) ;
#67723=ORIENTED_EDGE('',*,*,#48698,.T.) ;
#67724=ORIENTED_EDGE('',*,*,#48702,.F.) ;
#67725=ORIENTED_EDGE('',*,*,#48190,.F.) ;
#67726=ORIENTED_EDGE('',*,*,#48703,.T.) ;
#67727=ORIENTED_EDGE('',*,*,#48289,.F.) ;
#67728=ORIENTED_EDGE('',*,*,#48704,.F.) ;
#67729=ORIENTED_EDGE('',*,*,#48702,.T.) ;
#67730=ORIENTED_EDGE('',*,*,#48191,.F.) ;
#67731=ORIENTED_EDGE('',*,*,#48705,.F.) ;
#67732=ORIENTED_EDGE('',*,*,#48205,.F.) ;
#67733=ORIENTED_EDGE('',*,*,#48701,.T.) ;
#67734=ORIENTED_EDGE('',*,*,#48204,.F.) ;
#67735=ORIENTED_EDGE('',*,*,#48706,.F.) ;
#67736=ORIENTED_EDGE('',*,*,#48288,.F.) ;
#67737=ORIENTED_EDGE('',*,*,#48705,.T.) ;
#67738=ORIENTED_EDGE('',*,*,#48704,.T.) ;
#67739=ORIENTED_EDGE('',*,*,#48707,.F.) ;
#67740=ORIENTED_EDGE('',*,*,#48708,.F.) ;
#67741=ORIENTED_EDGE('',*,*,#48706,.T.) ;
#67742=ORIENTED_EDGE('',*,*,#48709,.F.) ;
#67743=ORIENTED_EDGE('',*,*,#48707,.T.) ;
#67744=ORIENTED_EDGE('',*,*,#48292,.F.) ;
#67745=ORIENTED_EDGE('',*,*,#48710,.F.) ;
#67746=ORIENTED_EDGE('',*,*,#48206,.F.) ;
#67747=ORIENTED_EDGE('',*,*,#48709,.T.) ;
#67748=ORIENTED_EDGE('',*,*,#48203,.F.) ;
#67749=ORIENTED_EDGE('',*,*,#48711,.F.) ;
#67750=ORIENTED_EDGE('',*,*,#48199,.F.) ;
#67751=ORIENTED_EDGE('',*,*,#48202,.F.) ;
#67752=ORIENTED_EDGE('',*,*,#48712,.T.) ;
#67753=ORIENTED_EDGE('',*,*,#48285,.F.) ;
#67754=ORIENTED_EDGE('',*,*,#48708,.T.) ;
#67755=ORIENTED_EDGE('',*,*,#48711,.T.) ;
#67756=ORIENTED_EDGE('',*,*,#48710,.T.) ;
#67757=ORIENTED_EDGE('',*,*,#48713,.F.) ;
#67758=ORIENTED_EDGE('',*,*,#48197,.F.) ;
#67759=ORIENTED_EDGE('',*,*,#48714,.T.) ;
#67760=ORIENTED_EDGE('',*,*,#48201,.F.) ;
#67761=ORIENTED_EDGE('',*,*,#48715,.T.) ;
#67762=ORIENTED_EDGE('',*,*,#48291,.F.) ;
#67763=ORIENTED_EDGE('',*,*,#48716,.T.) ;
#67764=ORIENTED_EDGE('',*,*,#48200,.F.) ;
#67765=ORIENTED_EDGE('',*,*,#48713,.T.) ;
#67766=ORIENTED_EDGE('',*,*,#44488,.F.) ;
#67767=ORIENTED_EDGE('',*,*,#47723,.F.) ;
#67768=ORIENTED_EDGE('',*,*,#48717,.F.) ;
#67769=ORIENTED_EDGE('',*,*,#47718,.F.) ;
#67770=ORIENTED_EDGE('',*,*,#48717,.T.) ;
#67771=ORIENTED_EDGE('',*,*,#47708,.F.) ;
#67772=ORIENTED_EDGE('',*,*,#48718,.F.) ;
#67773=ORIENTED_EDGE('',*,*,#47719,.F.) ;
#67774=ORIENTED_EDGE('',*,*,#48718,.T.) ;
#67775=ORIENTED_EDGE('',*,*,#48359,.F.) ;
#67776=ORIENTED_EDGE('',*,*,#48357,.F.) ;
#67777=ORIENTED_EDGE('',*,*,#48719,.F.) ;
#67778=ORIENTED_EDGE('',*,*,#48719,.T.) ;
#67779=ORIENTED_EDGE('',*,*,#48278,.F.) ;
#67780=ORIENTED_EDGE('',*,*,#48720,.F.) ;
#67781=ORIENTED_EDGE('',*,*,#47720,.F.) ;
#67782=ORIENTED_EDGE('',*,*,#48720,.T.) ;
#67783=ORIENTED_EDGE('',*,*,#48372,.F.) ;
#67784=ORIENTED_EDGE('',*,*,#48374,.F.) ;
#67785=ORIENTED_EDGE('',*,*,#48721,.F.) ;
#67786=ORIENTED_EDGE('',*,*,#48721,.T.) ;
#67787=ORIENTED_EDGE('',*,*,#47692,.F.) ;
#67788=ORIENTED_EDGE('',*,*,#48722,.F.) ;
#67789=ORIENTED_EDGE('',*,*,#47716,.F.) ;
#67790=ORIENTED_EDGE('',*,*,#44335,.F.) ;
#67791=ORIENTED_EDGE('',*,*,#47717,.F.) ;
#67792=ORIENTED_EDGE('',*,*,#48722,.T.) ;
#67793=ORIENTED_EDGE('',*,*,#47721,.F.) ;
#67794=ORIENTED_EDGE('',*,*,#46675,.F.) ;
#67795=ORIENTED_EDGE('',*,*,#46678,.F.) ;
#67796=ORIENTED_EDGE('',*,*,#47722,.F.) ;
#67797=ORIENTED_EDGE('',*,*,#48723,.F.) ;
#67798=ORIENTED_EDGE('',*,*,#47713,.F.) ;
#67799=ORIENTED_EDGE('',*,*,#48723,.T.) ;
#67800=ORIENTED_EDGE('',*,*,#47694,.F.) ;
#67801=ORIENTED_EDGE('',*,*,#48724,.F.) ;
#67802=ORIENTED_EDGE('',*,*,#47714,.F.) ;
#67803=ORIENTED_EDGE('',*,*,#48724,.T.) ;
#67804=ORIENTED_EDGE('',*,*,#48375,.F.) ;
#67805=ORIENTED_EDGE('',*,*,#48376,.F.) ;
#67806=ORIENTED_EDGE('',*,*,#48725,.F.) ;
#67807=ORIENTED_EDGE('',*,*,#48725,.T.) ;
#67808=ORIENTED_EDGE('',*,*,#48282,.F.) ;
#67809=ORIENTED_EDGE('',*,*,#48726,.F.) ;
#67810=ORIENTED_EDGE('',*,*,#47715,.F.) ;
#67811=ORIENTED_EDGE('',*,*,#48726,.T.) ;
#67812=ORIENTED_EDGE('',*,*,#48363,.F.) ;
#67813=ORIENTED_EDGE('',*,*,#48360,.F.) ;
#67814=ORIENTED_EDGE('',*,*,#48727,.F.) ;
#67815=ORIENTED_EDGE('',*,*,#48727,.T.) ;
#67816=ORIENTED_EDGE('',*,*,#47710,.F.) ;
#67817=ORIENTED_EDGE('',*,*,#48728,.F.) ;
#67818=ORIENTED_EDGE('',*,*,#47711,.F.) ;
#67819=ORIENTED_EDGE('',*,*,#48728,.T.) ;
#67820=ORIENTED_EDGE('',*,*,#47724,.F.) ;
#67821=ORIENTED_EDGE('',*,*,#44486,.F.) ;
#67822=ORIENTED_EDGE('',*,*,#47712,.F.) ;
#67823=ORIENTED_EDGE('',*,*,#46596,.F.) ;
#67824=ORIENTED_EDGE('',*,*,#47730,.F.) ;
#67825=ORIENTED_EDGE('',*,*,#48729,.F.) ;
#67826=ORIENTED_EDGE('',*,*,#47746,.F.) ;
#67827=ORIENTED_EDGE('',*,*,#48729,.T.) ;
#67828=ORIENTED_EDGE('',*,*,#48379,.F.) ;
#67829=ORIENTED_EDGE('',*,*,#48377,.F.) ;
#67830=ORIENTED_EDGE('',*,*,#48730,.F.) ;
#67831=ORIENTED_EDGE('',*,*,#48730,.T.) ;
#67832=ORIENTED_EDGE('',*,*,#48350,.F.) ;
#67833=ORIENTED_EDGE('',*,*,#48731,.F.) ;
#67834=ORIENTED_EDGE('',*,*,#47747,.F.) ;
#67835=ORIENTED_EDGE('',*,*,#48731,.T.) ;
#67836=ORIENTED_EDGE('',*,*,#48392,.F.) ;
#67837=ORIENTED_EDGE('',*,*,#48394,.F.) ;
#67838=ORIENTED_EDGE('',*,*,#48732,.F.) ;
#67839=ORIENTED_EDGE('',*,*,#46598,.F.) ;
#67840=ORIENTED_EDGE('',*,*,#47748,.F.) ;
#67841=ORIENTED_EDGE('',*,*,#48732,.T.) ;
#67842=ORIENTED_EDGE('',*,*,#47732,.F.) ;
#67843=ORIENTED_EDGE('',*,*,#48733,.F.) ;
#67844=ORIENTED_EDGE('',*,*,#47731,.F.) ;
#67845=ORIENTED_EDGE('',*,*,#46594,.F.) ;
#67846=ORIENTED_EDGE('',*,*,#47744,.F.) ;
#67847=ORIENTED_EDGE('',*,*,#48380,.F.) ;
#67848=ORIENTED_EDGE('',*,*,#48733,.T.) ;
#67849=ORIENTED_EDGE('',*,*,#48734,.F.) ;
#67850=ORIENTED_EDGE('',*,*,#48383,.F.) ;
#67851=ORIENTED_EDGE('',*,*,#48734,.T.) ;
#67852=ORIENTED_EDGE('',*,*,#47743,.F.) ;
#67853=ORIENTED_EDGE('',*,*,#48735,.F.) ;
#67854=ORIENTED_EDGE('',*,*,#48354,.F.) ;
#67855=ORIENTED_EDGE('',*,*,#46600,.F.) ;
#67856=ORIENTED_EDGE('',*,*,#47734,.F.) ;
#67857=ORIENTED_EDGE('',*,*,#48736,.F.) ;
#67858=ORIENTED_EDGE('',*,*,#47745,.F.) ;
#67859=ORIENTED_EDGE('',*,*,#48396,.F.) ;
#67860=ORIENTED_EDGE('',*,*,#48735,.T.) ;
#67861=ORIENTED_EDGE('',*,*,#48736,.T.) ;
#67862=ORIENTED_EDGE('',*,*,#48395,.F.) ;
#67863=ORIENTED_EDGE('',*,*,#44477,.F.) ;
#67864=ORIENTED_EDGE('',*,*,#47781,.F.) ;
#67865=ORIENTED_EDGE('',*,*,#48737,.F.) ;
#67866=ORIENTED_EDGE('',*,*,#47776,.F.) ;
#67867=ORIENTED_EDGE('',*,*,#48737,.T.) ;
#67868=ORIENTED_EDGE('',*,*,#47766,.F.) ;
#67869=ORIENTED_EDGE('',*,*,#48738,.F.) ;
#67870=ORIENTED_EDGE('',*,*,#47777,.F.) ;
#67871=ORIENTED_EDGE('',*,*,#48738,.T.) ;
#67872=ORIENTED_EDGE('',*,*,#48399,.F.) ;
#67873=ORIENTED_EDGE('',*,*,#48397,.F.) ;
#67874=ORIENTED_EDGE('',*,*,#48739,.F.) ;
#67875=ORIENTED_EDGE('',*,*,#48739,.T.) ;
#67876=ORIENTED_EDGE('',*,*,#48270,.F.) ;
#67877=ORIENTED_EDGE('',*,*,#48740,.F.) ;
#67878=ORIENTED_EDGE('',*,*,#47778,.F.) ;
#67879=ORIENTED_EDGE('',*,*,#48740,.T.) ;
#67880=ORIENTED_EDGE('',*,*,#48412,.F.) ;
#67881=ORIENTED_EDGE('',*,*,#48414,.F.) ;
#67882=ORIENTED_EDGE('',*,*,#48741,.F.) ;
#67883=ORIENTED_EDGE('',*,*,#48741,.T.) ;
#67884=ORIENTED_EDGE('',*,*,#47750,.F.) ;
#67885=ORIENTED_EDGE('',*,*,#48742,.F.) ;
#67886=ORIENTED_EDGE('',*,*,#47774,.F.) ;
#67887=ORIENTED_EDGE('',*,*,#44282,.F.) ;
#67888=ORIENTED_EDGE('',*,*,#47775,.F.) ;
#67889=ORIENTED_EDGE('',*,*,#48742,.T.) ;
#67890=ORIENTED_EDGE('',*,*,#47779,.F.) ;
#67891=ORIENTED_EDGE('',*,*,#46997,.F.) ;
#67892=ORIENTED_EDGE('',*,*,#47000,.F.) ;
#67893=ORIENTED_EDGE('',*,*,#47780,.F.) ;
#67894=ORIENTED_EDGE('',*,*,#48743,.F.) ;
#67895=ORIENTED_EDGE('',*,*,#47771,.F.) ;
#67896=ORIENTED_EDGE('',*,*,#48743,.T.) ;
#67897=ORIENTED_EDGE('',*,*,#47752,.F.) ;
#67898=ORIENTED_EDGE('',*,*,#48744,.F.) ;
#67899=ORIENTED_EDGE('',*,*,#47772,.F.) ;
#67900=ORIENTED_EDGE('',*,*,#48744,.T.) ;
#67901=ORIENTED_EDGE('',*,*,#48415,.F.) ;
#67902=ORIENTED_EDGE('',*,*,#48416,.F.) ;
#67903=ORIENTED_EDGE('',*,*,#48745,.F.) ;
#67904=ORIENTED_EDGE('',*,*,#48745,.T.) ;
#67905=ORIENTED_EDGE('',*,*,#48274,.F.) ;
#67906=ORIENTED_EDGE('',*,*,#48746,.F.) ;
#67907=ORIENTED_EDGE('',*,*,#47773,.F.) ;
#67908=ORIENTED_EDGE('',*,*,#48746,.T.) ;
#67909=ORIENTED_EDGE('',*,*,#48403,.F.) ;
#67910=ORIENTED_EDGE('',*,*,#48400,.F.) ;
#67911=ORIENTED_EDGE('',*,*,#48747,.F.) ;
#67912=ORIENTED_EDGE('',*,*,#48747,.T.) ;
#67913=ORIENTED_EDGE('',*,*,#47768,.F.) ;
#67914=ORIENTED_EDGE('',*,*,#48748,.F.) ;
#67915=ORIENTED_EDGE('',*,*,#47769,.F.) ;
#67916=ORIENTED_EDGE('',*,*,#48748,.T.) ;
#67917=ORIENTED_EDGE('',*,*,#47782,.F.) ;
#67918=ORIENTED_EDGE('',*,*,#44475,.F.) ;
#67919=ORIENTED_EDGE('',*,*,#47770,.F.) ;
#67920=ORIENTED_EDGE('',*,*,#46604,.F.) ;
#67921=ORIENTED_EDGE('',*,*,#47788,.F.) ;
#67922=ORIENTED_EDGE('',*,*,#48749,.F.) ;
#67923=ORIENTED_EDGE('',*,*,#47804,.F.) ;
#67924=ORIENTED_EDGE('',*,*,#48749,.T.) ;
#67925=ORIENTED_EDGE('',*,*,#48419,.F.) ;
#67926=ORIENTED_EDGE('',*,*,#48417,.F.) ;
#67927=ORIENTED_EDGE('',*,*,#48750,.F.) ;
#67928=ORIENTED_EDGE('',*,*,#48750,.T.) ;
#67929=ORIENTED_EDGE('',*,*,#48342,.F.) ;
#67930=ORIENTED_EDGE('',*,*,#48751,.F.) ;
#67931=ORIENTED_EDGE('',*,*,#47805,.F.) ;
#67932=ORIENTED_EDGE('',*,*,#48751,.T.) ;
#67933=ORIENTED_EDGE('',*,*,#48432,.F.) ;
#67934=ORIENTED_EDGE('',*,*,#48434,.F.) ;
#67935=ORIENTED_EDGE('',*,*,#48752,.F.) ;
#67936=ORIENTED_EDGE('',*,*,#46606,.F.) ;
#67937=ORIENTED_EDGE('',*,*,#47806,.F.) ;
#67938=ORIENTED_EDGE('',*,*,#48752,.T.) ;
#67939=ORIENTED_EDGE('',*,*,#47790,.F.) ;
#67940=ORIENTED_EDGE('',*,*,#48753,.F.) ;
#67941=ORIENTED_EDGE('',*,*,#47789,.F.) ;
#67942=ORIENTED_EDGE('',*,*,#46602,.F.) ;
#67943=ORIENTED_EDGE('',*,*,#47802,.F.) ;
#67944=ORIENTED_EDGE('',*,*,#48420,.F.) ;
#67945=ORIENTED_EDGE('',*,*,#48753,.T.) ;
#67946=ORIENTED_EDGE('',*,*,#48754,.F.) ;
#67947=ORIENTED_EDGE('',*,*,#48423,.F.) ;
#67948=ORIENTED_EDGE('',*,*,#48754,.T.) ;
#67949=ORIENTED_EDGE('',*,*,#47801,.F.) ;
#67950=ORIENTED_EDGE('',*,*,#48755,.F.) ;
#67951=ORIENTED_EDGE('',*,*,#48346,.F.) ;
#67952=ORIENTED_EDGE('',*,*,#46608,.F.) ;
#67953=ORIENTED_EDGE('',*,*,#47792,.F.) ;
#67954=ORIENTED_EDGE('',*,*,#48756,.F.) ;
#67955=ORIENTED_EDGE('',*,*,#47803,.F.) ;
#67956=ORIENTED_EDGE('',*,*,#48436,.F.) ;
#67957=ORIENTED_EDGE('',*,*,#48755,.T.) ;
#67958=ORIENTED_EDGE('',*,*,#48756,.T.) ;
#67959=ORIENTED_EDGE('',*,*,#48435,.F.) ;
#67960=ORIENTED_EDGE('',*,*,#44466,.F.) ;
#67961=ORIENTED_EDGE('',*,*,#47839,.F.) ;
#67962=ORIENTED_EDGE('',*,*,#48757,.F.) ;
#67963=ORIENTED_EDGE('',*,*,#47834,.F.) ;
#67964=ORIENTED_EDGE('',*,*,#48757,.T.) ;
#67965=ORIENTED_EDGE('',*,*,#47824,.F.) ;
#67966=ORIENTED_EDGE('',*,*,#48758,.F.) ;
#67967=ORIENTED_EDGE('',*,*,#47835,.F.) ;
#67968=ORIENTED_EDGE('',*,*,#48758,.T.) ;
#67969=ORIENTED_EDGE('',*,*,#48439,.F.) ;
#67970=ORIENTED_EDGE('',*,*,#48437,.F.) ;
#67971=ORIENTED_EDGE('',*,*,#48759,.F.) ;
#67972=ORIENTED_EDGE('',*,*,#48759,.T.) ;
#67973=ORIENTED_EDGE('',*,*,#48262,.F.) ;
#67974=ORIENTED_EDGE('',*,*,#48760,.F.) ;
#67975=ORIENTED_EDGE('',*,*,#47836,.F.) ;
#67976=ORIENTED_EDGE('',*,*,#48760,.T.) ;
#67977=ORIENTED_EDGE('',*,*,#48452,.F.) ;
#67978=ORIENTED_EDGE('',*,*,#48454,.F.) ;
#67979=ORIENTED_EDGE('',*,*,#48761,.F.) ;
#67980=ORIENTED_EDGE('',*,*,#48761,.T.) ;
#67981=ORIENTED_EDGE('',*,*,#47808,.F.) ;
#67982=ORIENTED_EDGE('',*,*,#48762,.F.) ;
#67983=ORIENTED_EDGE('',*,*,#47832,.F.) ;
#67984=ORIENTED_EDGE('',*,*,#44265,.F.) ;
#67985=ORIENTED_EDGE('',*,*,#47833,.F.) ;
#67986=ORIENTED_EDGE('',*,*,#48762,.T.) ;
#67987=ORIENTED_EDGE('',*,*,#47837,.F.) ;
#67988=ORIENTED_EDGE('',*,*,#47085,.F.) ;
#67989=ORIENTED_EDGE('',*,*,#47088,.F.) ;
#67990=ORIENTED_EDGE('',*,*,#47838,.F.) ;
#67991=ORIENTED_EDGE('',*,*,#48763,.F.) ;
#67992=ORIENTED_EDGE('',*,*,#47829,.F.) ;
#67993=ORIENTED_EDGE('',*,*,#48763,.T.) ;
#67994=ORIENTED_EDGE('',*,*,#47810,.F.) ;
#67995=ORIENTED_EDGE('',*,*,#48764,.F.) ;
#67996=ORIENTED_EDGE('',*,*,#47830,.F.) ;
#67997=ORIENTED_EDGE('',*,*,#48764,.T.) ;
#67998=ORIENTED_EDGE('',*,*,#48455,.F.) ;
#67999=ORIENTED_EDGE('',*,*,#48456,.F.) ;
#68000=ORIENTED_EDGE('',*,*,#48765,.F.) ;
#68001=ORIENTED_EDGE('',*,*,#48765,.T.) ;
#68002=ORIENTED_EDGE('',*,*,#48266,.F.) ;
#68003=ORIENTED_EDGE('',*,*,#48766,.F.) ;
#68004=ORIENTED_EDGE('',*,*,#47831,.F.) ;
#68005=ORIENTED_EDGE('',*,*,#48766,.T.) ;
#68006=ORIENTED_EDGE('',*,*,#48443,.F.) ;
#68007=ORIENTED_EDGE('',*,*,#48440,.F.) ;
#68008=ORIENTED_EDGE('',*,*,#48767,.F.) ;
#68009=ORIENTED_EDGE('',*,*,#48767,.T.) ;
#68010=ORIENTED_EDGE('',*,*,#47826,.F.) ;
#68011=ORIENTED_EDGE('',*,*,#48768,.F.) ;
#68012=ORIENTED_EDGE('',*,*,#47827,.F.) ;
#68013=ORIENTED_EDGE('',*,*,#48768,.T.) ;
#68014=ORIENTED_EDGE('',*,*,#47840,.F.) ;
#68015=ORIENTED_EDGE('',*,*,#44464,.F.) ;
#68016=ORIENTED_EDGE('',*,*,#47828,.F.) ;
#68017=ORIENTED_EDGE('',*,*,#46612,.F.) ;
#68018=ORIENTED_EDGE('',*,*,#47846,.F.) ;
#68019=ORIENTED_EDGE('',*,*,#48769,.F.) ;
#68020=ORIENTED_EDGE('',*,*,#47862,.F.) ;
#68021=ORIENTED_EDGE('',*,*,#48769,.T.) ;
#68022=ORIENTED_EDGE('',*,*,#48459,.F.) ;
#68023=ORIENTED_EDGE('',*,*,#48457,.F.) ;
#68024=ORIENTED_EDGE('',*,*,#48770,.F.) ;
#68025=ORIENTED_EDGE('',*,*,#48770,.T.) ;
#68026=ORIENTED_EDGE('',*,*,#48334,.F.) ;
#68027=ORIENTED_EDGE('',*,*,#48771,.F.) ;
#68028=ORIENTED_EDGE('',*,*,#47863,.F.) ;
#68029=ORIENTED_EDGE('',*,*,#48771,.T.) ;
#68030=ORIENTED_EDGE('',*,*,#48472,.F.) ;
#68031=ORIENTED_EDGE('',*,*,#48474,.F.) ;
#68032=ORIENTED_EDGE('',*,*,#48772,.F.) ;
#68033=ORIENTED_EDGE('',*,*,#46614,.F.) ;
#68034=ORIENTED_EDGE('',*,*,#47864,.F.) ;
#68035=ORIENTED_EDGE('',*,*,#48772,.T.) ;
#68036=ORIENTED_EDGE('',*,*,#47848,.F.) ;
#68037=ORIENTED_EDGE('',*,*,#48773,.F.) ;
#68038=ORIENTED_EDGE('',*,*,#47847,.F.) ;
#68039=ORIENTED_EDGE('',*,*,#46610,.F.) ;
#68040=ORIENTED_EDGE('',*,*,#47860,.F.) ;
#68041=ORIENTED_EDGE('',*,*,#48460,.F.) ;
#68042=ORIENTED_EDGE('',*,*,#48773,.T.) ;
#68043=ORIENTED_EDGE('',*,*,#48774,.F.) ;
#68044=ORIENTED_EDGE('',*,*,#48463,.F.) ;
#68045=ORIENTED_EDGE('',*,*,#48774,.T.) ;
#68046=ORIENTED_EDGE('',*,*,#47859,.F.) ;
#68047=ORIENTED_EDGE('',*,*,#48775,.F.) ;
#68048=ORIENTED_EDGE('',*,*,#48338,.F.) ;
#68049=ORIENTED_EDGE('',*,*,#46616,.F.) ;
#68050=ORIENTED_EDGE('',*,*,#47850,.F.) ;
#68051=ORIENTED_EDGE('',*,*,#48776,.F.) ;
#68052=ORIENTED_EDGE('',*,*,#47861,.F.) ;
#68053=ORIENTED_EDGE('',*,*,#48476,.F.) ;
#68054=ORIENTED_EDGE('',*,*,#48775,.T.) ;
#68055=ORIENTED_EDGE('',*,*,#48776,.T.) ;
#68056=ORIENTED_EDGE('',*,*,#48475,.F.) ;
#68057=ORIENTED_EDGE('',*,*,#44455,.F.) ;
#68058=ORIENTED_EDGE('',*,*,#47897,.F.) ;
#68059=ORIENTED_EDGE('',*,*,#48777,.F.) ;
#68060=ORIENTED_EDGE('',*,*,#47892,.F.) ;
#68061=ORIENTED_EDGE('',*,*,#48777,.T.) ;
#68062=ORIENTED_EDGE('',*,*,#47882,.F.) ;
#68063=ORIENTED_EDGE('',*,*,#48778,.F.) ;
#68064=ORIENTED_EDGE('',*,*,#47893,.F.) ;
#68065=ORIENTED_EDGE('',*,*,#48778,.T.) ;
#68066=ORIENTED_EDGE('',*,*,#48479,.F.) ;
#68067=ORIENTED_EDGE('',*,*,#48477,.F.) ;
#68068=ORIENTED_EDGE('',*,*,#48779,.F.) ;
#68069=ORIENTED_EDGE('',*,*,#48779,.T.) ;
#68070=ORIENTED_EDGE('',*,*,#48254,.F.) ;
#68071=ORIENTED_EDGE('',*,*,#48780,.F.) ;
#68072=ORIENTED_EDGE('',*,*,#47894,.F.) ;
#68073=ORIENTED_EDGE('',*,*,#48780,.T.) ;
#68074=ORIENTED_EDGE('',*,*,#48492,.F.) ;
#68075=ORIENTED_EDGE('',*,*,#48494,.F.) ;
#68076=ORIENTED_EDGE('',*,*,#48781,.F.) ;
#68077=ORIENTED_EDGE('',*,*,#48781,.T.) ;
#68078=ORIENTED_EDGE('',*,*,#47866,.F.) ;
#68079=ORIENTED_EDGE('',*,*,#48782,.F.) ;
#68080=ORIENTED_EDGE('',*,*,#47890,.F.) ;
#68081=ORIENTED_EDGE('',*,*,#44248,.F.) ;
#68082=ORIENTED_EDGE('',*,*,#47891,.F.) ;
#68083=ORIENTED_EDGE('',*,*,#48782,.T.) ;
#68084=ORIENTED_EDGE('',*,*,#47895,.F.) ;
#68085=ORIENTED_EDGE('',*,*,#47173,.F.) ;
#68086=ORIENTED_EDGE('',*,*,#47176,.F.) ;
#68087=ORIENTED_EDGE('',*,*,#47896,.F.) ;
#68088=ORIENTED_EDGE('',*,*,#48783,.F.) ;
#68089=ORIENTED_EDGE('',*,*,#47887,.F.) ;
#68090=ORIENTED_EDGE('',*,*,#48783,.T.) ;
#68091=ORIENTED_EDGE('',*,*,#47868,.F.) ;
#68092=ORIENTED_EDGE('',*,*,#48784,.F.) ;
#68093=ORIENTED_EDGE('',*,*,#47888,.F.) ;
#68094=ORIENTED_EDGE('',*,*,#48784,.T.) ;
#68095=ORIENTED_EDGE('',*,*,#48495,.F.) ;
#68096=ORIENTED_EDGE('',*,*,#48496,.F.) ;
#68097=ORIENTED_EDGE('',*,*,#48785,.F.) ;
#68098=ORIENTED_EDGE('',*,*,#48785,.T.) ;
#68099=ORIENTED_EDGE('',*,*,#48258,.F.) ;
#68100=ORIENTED_EDGE('',*,*,#48786,.F.) ;
#68101=ORIENTED_EDGE('',*,*,#47889,.F.) ;
#68102=ORIENTED_EDGE('',*,*,#48786,.T.) ;
#68103=ORIENTED_EDGE('',*,*,#48483,.F.) ;
#68104=ORIENTED_EDGE('',*,*,#48480,.F.) ;
#68105=ORIENTED_EDGE('',*,*,#48787,.F.) ;
#68106=ORIENTED_EDGE('',*,*,#48787,.T.) ;
#68107=ORIENTED_EDGE('',*,*,#47884,.F.) ;
#68108=ORIENTED_EDGE('',*,*,#48788,.F.) ;
#68109=ORIENTED_EDGE('',*,*,#47885,.F.) ;
#68110=ORIENTED_EDGE('',*,*,#48788,.T.) ;
#68111=ORIENTED_EDGE('',*,*,#47898,.F.) ;
#68112=ORIENTED_EDGE('',*,*,#44453,.F.) ;
#68113=ORIENTED_EDGE('',*,*,#47886,.F.) ;
#68114=ORIENTED_EDGE('',*,*,#46620,.F.) ;
#68115=ORIENTED_EDGE('',*,*,#47904,.F.) ;
#68116=ORIENTED_EDGE('',*,*,#48789,.F.) ;
#68117=ORIENTED_EDGE('',*,*,#47920,.F.) ;
#68118=ORIENTED_EDGE('',*,*,#48789,.T.) ;
#68119=ORIENTED_EDGE('',*,*,#48499,.F.) ;
#68120=ORIENTED_EDGE('',*,*,#48497,.F.) ;
#68121=ORIENTED_EDGE('',*,*,#48790,.F.) ;
#68122=ORIENTED_EDGE('',*,*,#48790,.T.) ;
#68123=ORIENTED_EDGE('',*,*,#48326,.F.) ;
#68124=ORIENTED_EDGE('',*,*,#48791,.F.) ;
#68125=ORIENTED_EDGE('',*,*,#47921,.F.) ;
#68126=ORIENTED_EDGE('',*,*,#48791,.T.) ;
#68127=ORIENTED_EDGE('',*,*,#48512,.F.) ;
#68128=ORIENTED_EDGE('',*,*,#48514,.F.) ;
#68129=ORIENTED_EDGE('',*,*,#48792,.F.) ;
#68130=ORIENTED_EDGE('',*,*,#46622,.F.) ;
#68131=ORIENTED_EDGE('',*,*,#47922,.F.) ;
#68132=ORIENTED_EDGE('',*,*,#48792,.T.) ;
#68133=ORIENTED_EDGE('',*,*,#47906,.F.) ;
#68134=ORIENTED_EDGE('',*,*,#48793,.F.) ;
#68135=ORIENTED_EDGE('',*,*,#47905,.F.) ;
#68136=ORIENTED_EDGE('',*,*,#46618,.F.) ;
#68137=ORIENTED_EDGE('',*,*,#47918,.F.) ;
#68138=ORIENTED_EDGE('',*,*,#48500,.F.) ;
#68139=ORIENTED_EDGE('',*,*,#48793,.T.) ;
#68140=ORIENTED_EDGE('',*,*,#48794,.F.) ;
#68141=ORIENTED_EDGE('',*,*,#48503,.F.) ;
#68142=ORIENTED_EDGE('',*,*,#48794,.T.) ;
#68143=ORIENTED_EDGE('',*,*,#47917,.F.) ;
#68144=ORIENTED_EDGE('',*,*,#48795,.F.) ;
#68145=ORIENTED_EDGE('',*,*,#48330,.F.) ;
#68146=ORIENTED_EDGE('',*,*,#46624,.F.) ;
#68147=ORIENTED_EDGE('',*,*,#47908,.F.) ;
#68148=ORIENTED_EDGE('',*,*,#48796,.F.) ;
#68149=ORIENTED_EDGE('',*,*,#47919,.F.) ;
#68150=ORIENTED_EDGE('',*,*,#48516,.F.) ;
#68151=ORIENTED_EDGE('',*,*,#48795,.T.) ;
#68152=ORIENTED_EDGE('',*,*,#48796,.T.) ;
#68153=ORIENTED_EDGE('',*,*,#48515,.F.) ;
#68154=ORIENTED_EDGE('',*,*,#44444,.F.) ;
#68155=ORIENTED_EDGE('',*,*,#47955,.F.) ;
#68156=ORIENTED_EDGE('',*,*,#48797,.F.) ;
#68157=ORIENTED_EDGE('',*,*,#47950,.F.) ;
#68158=ORIENTED_EDGE('',*,*,#48797,.T.) ;
#68159=ORIENTED_EDGE('',*,*,#47940,.F.) ;
#68160=ORIENTED_EDGE('',*,*,#48798,.F.) ;
#68161=ORIENTED_EDGE('',*,*,#47951,.F.) ;
#68162=ORIENTED_EDGE('',*,*,#48798,.T.) ;
#68163=ORIENTED_EDGE('',*,*,#48519,.F.) ;
#68164=ORIENTED_EDGE('',*,*,#48517,.F.) ;
#68165=ORIENTED_EDGE('',*,*,#48799,.F.) ;
#68166=ORIENTED_EDGE('',*,*,#48799,.T.) ;
#68167=ORIENTED_EDGE('',*,*,#48246,.F.) ;
#68168=ORIENTED_EDGE('',*,*,#48800,.F.) ;
#68169=ORIENTED_EDGE('',*,*,#47952,.F.) ;
#68170=ORIENTED_EDGE('',*,*,#48800,.T.) ;
#68171=ORIENTED_EDGE('',*,*,#48532,.F.) ;
#68172=ORIENTED_EDGE('',*,*,#48534,.F.) ;
#68173=ORIENTED_EDGE('',*,*,#48801,.F.) ;
#68174=ORIENTED_EDGE('',*,*,#48801,.T.) ;
#68175=ORIENTED_EDGE('',*,*,#47924,.F.) ;
#68176=ORIENTED_EDGE('',*,*,#48802,.F.) ;
#68177=ORIENTED_EDGE('',*,*,#47948,.F.) ;
#68178=ORIENTED_EDGE('',*,*,#44231,.F.) ;
#68179=ORIENTED_EDGE('',*,*,#47949,.F.) ;
#68180=ORIENTED_EDGE('',*,*,#48802,.T.) ;
#68181=ORIENTED_EDGE('',*,*,#47953,.F.) ;
#68182=ORIENTED_EDGE('',*,*,#47261,.F.) ;
#68183=ORIENTED_EDGE('',*,*,#47264,.F.) ;
#68184=ORIENTED_EDGE('',*,*,#47954,.F.) ;
#68185=ORIENTED_EDGE('',*,*,#48803,.F.) ;
#68186=ORIENTED_EDGE('',*,*,#47945,.F.) ;
#68187=ORIENTED_EDGE('',*,*,#48803,.T.) ;
#68188=ORIENTED_EDGE('',*,*,#47926,.F.) ;
#68189=ORIENTED_EDGE('',*,*,#48804,.F.) ;
#68190=ORIENTED_EDGE('',*,*,#47946,.F.) ;
#68191=ORIENTED_EDGE('',*,*,#48804,.T.) ;
#68192=ORIENTED_EDGE('',*,*,#48535,.F.) ;
#68193=ORIENTED_EDGE('',*,*,#48536,.F.) ;
#68194=ORIENTED_EDGE('',*,*,#48805,.F.) ;
#68195=ORIENTED_EDGE('',*,*,#48805,.T.) ;
#68196=ORIENTED_EDGE('',*,*,#48250,.F.) ;
#68197=ORIENTED_EDGE('',*,*,#48806,.F.) ;
#68198=ORIENTED_EDGE('',*,*,#47947,.F.) ;
#68199=ORIENTED_EDGE('',*,*,#48806,.T.) ;
#68200=ORIENTED_EDGE('',*,*,#48523,.F.) ;
#68201=ORIENTED_EDGE('',*,*,#48520,.F.) ;
#68202=ORIENTED_EDGE('',*,*,#48807,.F.) ;
#68203=ORIENTED_EDGE('',*,*,#48807,.T.) ;
#68204=ORIENTED_EDGE('',*,*,#47942,.F.) ;
#68205=ORIENTED_EDGE('',*,*,#48808,.F.) ;
#68206=ORIENTED_EDGE('',*,*,#47943,.F.) ;
#68207=ORIENTED_EDGE('',*,*,#48808,.T.) ;
#68208=ORIENTED_EDGE('',*,*,#47956,.F.) ;
#68209=ORIENTED_EDGE('',*,*,#44442,.F.) ;
#68210=ORIENTED_EDGE('',*,*,#47944,.F.) ;
#68211=ORIENTED_EDGE('',*,*,#46628,.F.) ;
#68212=ORIENTED_EDGE('',*,*,#47962,.F.) ;
#68213=ORIENTED_EDGE('',*,*,#48809,.F.) ;
#68214=ORIENTED_EDGE('',*,*,#47978,.F.) ;
#68215=ORIENTED_EDGE('',*,*,#48809,.T.) ;
#68216=ORIENTED_EDGE('',*,*,#48539,.F.) ;
#68217=ORIENTED_EDGE('',*,*,#48537,.F.) ;
#68218=ORIENTED_EDGE('',*,*,#48810,.F.) ;
#68219=ORIENTED_EDGE('',*,*,#48810,.T.) ;
#68220=ORIENTED_EDGE('',*,*,#48318,.F.) ;
#68221=ORIENTED_EDGE('',*,*,#48811,.F.) ;
#68222=ORIENTED_EDGE('',*,*,#47979,.F.) ;
#68223=ORIENTED_EDGE('',*,*,#48811,.T.) ;
#68224=ORIENTED_EDGE('',*,*,#48552,.F.) ;
#68225=ORIENTED_EDGE('',*,*,#48554,.F.) ;
#68226=ORIENTED_EDGE('',*,*,#48812,.F.) ;
#68227=ORIENTED_EDGE('',*,*,#46630,.F.) ;
#68228=ORIENTED_EDGE('',*,*,#47980,.F.) ;
#68229=ORIENTED_EDGE('',*,*,#48812,.T.) ;
#68230=ORIENTED_EDGE('',*,*,#47964,.F.) ;
#68231=ORIENTED_EDGE('',*,*,#48813,.F.) ;
#68232=ORIENTED_EDGE('',*,*,#47963,.F.) ;
#68233=ORIENTED_EDGE('',*,*,#46626,.F.) ;
#68234=ORIENTED_EDGE('',*,*,#47976,.F.) ;
#68235=ORIENTED_EDGE('',*,*,#48540,.F.) ;
#68236=ORIENTED_EDGE('',*,*,#48813,.T.) ;
#68237=ORIENTED_EDGE('',*,*,#48814,.F.) ;
#68238=ORIENTED_EDGE('',*,*,#48543,.F.) ;
#68239=ORIENTED_EDGE('',*,*,#48814,.T.) ;
#68240=ORIENTED_EDGE('',*,*,#47975,.F.) ;
#68241=ORIENTED_EDGE('',*,*,#48815,.F.) ;
#68242=ORIENTED_EDGE('',*,*,#48322,.F.) ;
#68243=ORIENTED_EDGE('',*,*,#46632,.F.) ;
#68244=ORIENTED_EDGE('',*,*,#47966,.F.) ;
#68245=ORIENTED_EDGE('',*,*,#48816,.F.) ;
#68246=ORIENTED_EDGE('',*,*,#47977,.F.) ;
#68247=ORIENTED_EDGE('',*,*,#48556,.F.) ;
#68248=ORIENTED_EDGE('',*,*,#48815,.T.) ;
#68249=ORIENTED_EDGE('',*,*,#48816,.T.) ;
#68250=ORIENTED_EDGE('',*,*,#48555,.F.) ;
#68251=ORIENTED_EDGE('',*,*,#44433,.F.) ;
#68252=ORIENTED_EDGE('',*,*,#48013,.F.) ;
#68253=ORIENTED_EDGE('',*,*,#48817,.F.) ;
#68254=ORIENTED_EDGE('',*,*,#48008,.F.) ;
#68255=ORIENTED_EDGE('',*,*,#48817,.T.) ;
#68256=ORIENTED_EDGE('',*,*,#47998,.F.) ;
#68257=ORIENTED_EDGE('',*,*,#48818,.F.) ;
#68258=ORIENTED_EDGE('',*,*,#48009,.F.) ;
#68259=ORIENTED_EDGE('',*,*,#48818,.T.) ;
#68260=ORIENTED_EDGE('',*,*,#48559,.F.) ;
#68261=ORIENTED_EDGE('',*,*,#48557,.F.) ;
#68262=ORIENTED_EDGE('',*,*,#48819,.F.) ;
#68263=ORIENTED_EDGE('',*,*,#48819,.T.) ;
#68264=ORIENTED_EDGE('',*,*,#48238,.F.) ;
#68265=ORIENTED_EDGE('',*,*,#48820,.F.) ;
#68266=ORIENTED_EDGE('',*,*,#48010,.F.) ;
#68267=ORIENTED_EDGE('',*,*,#48820,.T.) ;
#68268=ORIENTED_EDGE('',*,*,#48572,.F.) ;
#68269=ORIENTED_EDGE('',*,*,#48574,.F.) ;
#68270=ORIENTED_EDGE('',*,*,#48821,.F.) ;
#68271=ORIENTED_EDGE('',*,*,#48821,.T.) ;
#68272=ORIENTED_EDGE('',*,*,#47982,.F.) ;
#68273=ORIENTED_EDGE('',*,*,#48822,.F.) ;
#68274=ORIENTED_EDGE('',*,*,#48006,.F.) ;
#68275=ORIENTED_EDGE('',*,*,#44214,.F.) ;
#68276=ORIENTED_EDGE('',*,*,#48007,.F.) ;
#68277=ORIENTED_EDGE('',*,*,#48822,.T.) ;
#68278=ORIENTED_EDGE('',*,*,#48011,.F.) ;
#68279=ORIENTED_EDGE('',*,*,#47349,.F.) ;
#68280=ORIENTED_EDGE('',*,*,#47352,.F.) ;
#68281=ORIENTED_EDGE('',*,*,#48012,.F.) ;
#68282=ORIENTED_EDGE('',*,*,#48823,.F.) ;
#68283=ORIENTED_EDGE('',*,*,#48003,.F.) ;
#68284=ORIENTED_EDGE('',*,*,#48823,.T.) ;
#68285=ORIENTED_EDGE('',*,*,#47984,.F.) ;
#68286=ORIENTED_EDGE('',*,*,#48824,.F.) ;
#68287=ORIENTED_EDGE('',*,*,#48004,.F.) ;
#68288=ORIENTED_EDGE('',*,*,#48824,.T.) ;
#68289=ORIENTED_EDGE('',*,*,#48575,.F.) ;
#68290=ORIENTED_EDGE('',*,*,#48576,.F.) ;
#68291=ORIENTED_EDGE('',*,*,#48825,.F.) ;
#68292=ORIENTED_EDGE('',*,*,#48825,.T.) ;
#68293=ORIENTED_EDGE('',*,*,#48242,.F.) ;
#68294=ORIENTED_EDGE('',*,*,#48826,.F.) ;
#68295=ORIENTED_EDGE('',*,*,#48005,.F.) ;
#68296=ORIENTED_EDGE('',*,*,#48826,.T.) ;
#68297=ORIENTED_EDGE('',*,*,#48563,.F.) ;
#68298=ORIENTED_EDGE('',*,*,#48560,.F.) ;
#68299=ORIENTED_EDGE('',*,*,#48827,.F.) ;
#68300=ORIENTED_EDGE('',*,*,#48827,.T.) ;
#68301=ORIENTED_EDGE('',*,*,#48000,.F.) ;
#68302=ORIENTED_EDGE('',*,*,#48828,.F.) ;
#68303=ORIENTED_EDGE('',*,*,#48001,.F.) ;
#68304=ORIENTED_EDGE('',*,*,#48828,.T.) ;
#68305=ORIENTED_EDGE('',*,*,#48014,.F.) ;
#68306=ORIENTED_EDGE('',*,*,#44431,.F.) ;
#68307=ORIENTED_EDGE('',*,*,#48002,.F.) ;
#68308=ORIENTED_EDGE('',*,*,#46636,.F.) ;
#68309=ORIENTED_EDGE('',*,*,#48020,.F.) ;
#68310=ORIENTED_EDGE('',*,*,#48829,.F.) ;
#68311=ORIENTED_EDGE('',*,*,#48036,.F.) ;
#68312=ORIENTED_EDGE('',*,*,#48829,.T.) ;
#68313=ORIENTED_EDGE('',*,*,#48579,.F.) ;
#68314=ORIENTED_EDGE('',*,*,#48577,.F.) ;
#68315=ORIENTED_EDGE('',*,*,#48830,.F.) ;
#68316=ORIENTED_EDGE('',*,*,#48830,.T.) ;
#68317=ORIENTED_EDGE('',*,*,#48310,.F.) ;
#68318=ORIENTED_EDGE('',*,*,#48831,.F.) ;
#68319=ORIENTED_EDGE('',*,*,#48037,.F.) ;
#68320=ORIENTED_EDGE('',*,*,#48831,.T.) ;
#68321=ORIENTED_EDGE('',*,*,#48592,.F.) ;
#68322=ORIENTED_EDGE('',*,*,#48594,.F.) ;
#68323=ORIENTED_EDGE('',*,*,#48832,.F.) ;
#68324=ORIENTED_EDGE('',*,*,#46638,.F.) ;
#68325=ORIENTED_EDGE('',*,*,#48038,.F.) ;
#68326=ORIENTED_EDGE('',*,*,#48832,.T.) ;
#68327=ORIENTED_EDGE('',*,*,#48022,.F.) ;
#68328=ORIENTED_EDGE('',*,*,#48833,.F.) ;
#68329=ORIENTED_EDGE('',*,*,#48021,.F.) ;
#68330=ORIENTED_EDGE('',*,*,#46634,.F.) ;
#68331=ORIENTED_EDGE('',*,*,#48034,.F.) ;
#68332=ORIENTED_EDGE('',*,*,#48580,.F.) ;
#68333=ORIENTED_EDGE('',*,*,#48833,.T.) ;
#68334=ORIENTED_EDGE('',*,*,#48834,.F.) ;
#68335=ORIENTED_EDGE('',*,*,#48583,.F.) ;
#68336=ORIENTED_EDGE('',*,*,#48834,.T.) ;
#68337=ORIENTED_EDGE('',*,*,#48033,.F.) ;
#68338=ORIENTED_EDGE('',*,*,#48835,.F.) ;
#68339=ORIENTED_EDGE('',*,*,#48314,.F.) ;
#68340=ORIENTED_EDGE('',*,*,#46640,.F.) ;
#68341=ORIENTED_EDGE('',*,*,#48024,.F.) ;
#68342=ORIENTED_EDGE('',*,*,#48836,.F.) ;
#68343=ORIENTED_EDGE('',*,*,#48035,.F.) ;
#68344=ORIENTED_EDGE('',*,*,#48596,.F.) ;
#68345=ORIENTED_EDGE('',*,*,#48835,.T.) ;
#68346=ORIENTED_EDGE('',*,*,#48836,.T.) ;
#68347=ORIENTED_EDGE('',*,*,#48595,.F.) ;
#68348=ORIENTED_EDGE('',*,*,#44422,.F.) ;
#68349=ORIENTED_EDGE('',*,*,#48071,.F.) ;
#68350=ORIENTED_EDGE('',*,*,#48837,.F.) ;
#68351=ORIENTED_EDGE('',*,*,#48066,.F.) ;
#68352=ORIENTED_EDGE('',*,*,#48837,.T.) ;
#68353=ORIENTED_EDGE('',*,*,#48056,.F.) ;
#68354=ORIENTED_EDGE('',*,*,#48838,.F.) ;
#68355=ORIENTED_EDGE('',*,*,#48067,.F.) ;
#68356=ORIENTED_EDGE('',*,*,#48838,.T.) ;
#68357=ORIENTED_EDGE('',*,*,#48599,.F.) ;
#68358=ORIENTED_EDGE('',*,*,#48597,.F.) ;
#68359=ORIENTED_EDGE('',*,*,#48839,.F.) ;
#68360=ORIENTED_EDGE('',*,*,#48839,.T.) ;
#68361=ORIENTED_EDGE('',*,*,#48230,.F.) ;
#68362=ORIENTED_EDGE('',*,*,#48840,.F.) ;
#68363=ORIENTED_EDGE('',*,*,#48068,.F.) ;
#68364=ORIENTED_EDGE('',*,*,#48840,.T.) ;
#68365=ORIENTED_EDGE('',*,*,#48612,.F.) ;
#68366=ORIENTED_EDGE('',*,*,#48614,.F.) ;
#68367=ORIENTED_EDGE('',*,*,#48841,.F.) ;
#68368=ORIENTED_EDGE('',*,*,#48841,.T.) ;
#68369=ORIENTED_EDGE('',*,*,#48040,.F.) ;
#68370=ORIENTED_EDGE('',*,*,#48842,.F.) ;
#68371=ORIENTED_EDGE('',*,*,#48064,.F.) ;
#68372=ORIENTED_EDGE('',*,*,#44197,.F.) ;
#68373=ORIENTED_EDGE('',*,*,#48065,.F.) ;
#68374=ORIENTED_EDGE('',*,*,#48842,.T.) ;
#68375=ORIENTED_EDGE('',*,*,#48069,.F.) ;
#68376=ORIENTED_EDGE('',*,*,#47437,.F.) ;
#68377=ORIENTED_EDGE('',*,*,#47440,.F.) ;
#68378=ORIENTED_EDGE('',*,*,#48070,.F.) ;
#68379=ORIENTED_EDGE('',*,*,#48843,.F.) ;
#68380=ORIENTED_EDGE('',*,*,#48061,.F.) ;
#68381=ORIENTED_EDGE('',*,*,#48843,.T.) ;
#68382=ORIENTED_EDGE('',*,*,#48042,.F.) ;
#68383=ORIENTED_EDGE('',*,*,#48844,.F.) ;
#68384=ORIENTED_EDGE('',*,*,#48062,.F.) ;
#68385=ORIENTED_EDGE('',*,*,#48844,.T.) ;
#68386=ORIENTED_EDGE('',*,*,#48615,.F.) ;
#68387=ORIENTED_EDGE('',*,*,#48616,.F.) ;
#68388=ORIENTED_EDGE('',*,*,#48845,.F.) ;
#68389=ORIENTED_EDGE('',*,*,#48845,.T.) ;
#68390=ORIENTED_EDGE('',*,*,#48234,.F.) ;
#68391=ORIENTED_EDGE('',*,*,#48846,.F.) ;
#68392=ORIENTED_EDGE('',*,*,#48063,.F.) ;
#68393=ORIENTED_EDGE('',*,*,#48846,.T.) ;
#68394=ORIENTED_EDGE('',*,*,#48603,.F.) ;
#68395=ORIENTED_EDGE('',*,*,#48600,.F.) ;
#68396=ORIENTED_EDGE('',*,*,#48847,.F.) ;
#68397=ORIENTED_EDGE('',*,*,#48847,.T.) ;
#68398=ORIENTED_EDGE('',*,*,#48058,.F.) ;
#68399=ORIENTED_EDGE('',*,*,#48848,.F.) ;
#68400=ORIENTED_EDGE('',*,*,#48059,.F.) ;
#68401=ORIENTED_EDGE('',*,*,#48848,.T.) ;
#68402=ORIENTED_EDGE('',*,*,#48072,.F.) ;
#68403=ORIENTED_EDGE('',*,*,#44420,.F.) ;
#68404=ORIENTED_EDGE('',*,*,#48060,.F.) ;
#68405=ORIENTED_EDGE('',*,*,#46644,.F.) ;
#68406=ORIENTED_EDGE('',*,*,#48078,.F.) ;
#68407=ORIENTED_EDGE('',*,*,#48849,.F.) ;
#68408=ORIENTED_EDGE('',*,*,#48094,.F.) ;
#68409=ORIENTED_EDGE('',*,*,#48849,.T.) ;
#68410=ORIENTED_EDGE('',*,*,#48619,.F.) ;
#68411=ORIENTED_EDGE('',*,*,#48617,.F.) ;
#68412=ORIENTED_EDGE('',*,*,#48850,.F.) ;
#68413=ORIENTED_EDGE('',*,*,#48850,.T.) ;
#68414=ORIENTED_EDGE('',*,*,#48302,.F.) ;
#68415=ORIENTED_EDGE('',*,*,#48851,.F.) ;
#68416=ORIENTED_EDGE('',*,*,#48095,.F.) ;
#68417=ORIENTED_EDGE('',*,*,#48851,.T.) ;
#68418=ORIENTED_EDGE('',*,*,#48632,.F.) ;
#68419=ORIENTED_EDGE('',*,*,#48634,.F.) ;
#68420=ORIENTED_EDGE('',*,*,#48852,.F.) ;
#68421=ORIENTED_EDGE('',*,*,#46646,.F.) ;
#68422=ORIENTED_EDGE('',*,*,#48096,.F.) ;
#68423=ORIENTED_EDGE('',*,*,#48852,.T.) ;
#68424=ORIENTED_EDGE('',*,*,#48080,.F.) ;
#68425=ORIENTED_EDGE('',*,*,#48853,.F.) ;
#68426=ORIENTED_EDGE('',*,*,#48079,.F.) ;
#68427=ORIENTED_EDGE('',*,*,#46642,.F.) ;
#68428=ORIENTED_EDGE('',*,*,#48092,.F.) ;
#68429=ORIENTED_EDGE('',*,*,#48620,.F.) ;
#68430=ORIENTED_EDGE('',*,*,#48853,.T.) ;
#68431=ORIENTED_EDGE('',*,*,#48854,.F.) ;
#68432=ORIENTED_EDGE('',*,*,#48623,.F.) ;
#68433=ORIENTED_EDGE('',*,*,#48854,.T.) ;
#68434=ORIENTED_EDGE('',*,*,#48091,.F.) ;
#68435=ORIENTED_EDGE('',*,*,#48855,.F.) ;
#68436=ORIENTED_EDGE('',*,*,#48306,.F.) ;
#68437=ORIENTED_EDGE('',*,*,#46648,.F.) ;
#68438=ORIENTED_EDGE('',*,*,#48082,.F.) ;
#68439=ORIENTED_EDGE('',*,*,#48856,.F.) ;
#68440=ORIENTED_EDGE('',*,*,#48093,.F.) ;
#68441=ORIENTED_EDGE('',*,*,#48636,.F.) ;
#68442=ORIENTED_EDGE('',*,*,#48855,.T.) ;
#68443=ORIENTED_EDGE('',*,*,#48856,.T.) ;
#68444=ORIENTED_EDGE('',*,*,#48635,.F.) ;
#68445=ORIENTED_EDGE('',*,*,#44411,.F.) ;
#68446=ORIENTED_EDGE('',*,*,#48129,.F.) ;
#68447=ORIENTED_EDGE('',*,*,#48857,.F.) ;
#68448=ORIENTED_EDGE('',*,*,#48124,.F.) ;
#68449=ORIENTED_EDGE('',*,*,#48857,.T.) ;
#68450=ORIENTED_EDGE('',*,*,#48114,.F.) ;
#68451=ORIENTED_EDGE('',*,*,#48858,.F.) ;
#68452=ORIENTED_EDGE('',*,*,#48125,.F.) ;
#68453=ORIENTED_EDGE('',*,*,#48858,.T.) ;
#68454=ORIENTED_EDGE('',*,*,#48639,.F.) ;
#68455=ORIENTED_EDGE('',*,*,#48637,.F.) ;
#68456=ORIENTED_EDGE('',*,*,#48859,.F.) ;
#68457=ORIENTED_EDGE('',*,*,#48859,.T.) ;
#68458=ORIENTED_EDGE('',*,*,#48222,.F.) ;
#68459=ORIENTED_EDGE('',*,*,#48860,.F.) ;
#68460=ORIENTED_EDGE('',*,*,#48126,.F.) ;
#68461=ORIENTED_EDGE('',*,*,#48860,.T.) ;
#68462=ORIENTED_EDGE('',*,*,#48652,.F.) ;
#68463=ORIENTED_EDGE('',*,*,#48654,.F.) ;
#68464=ORIENTED_EDGE('',*,*,#48861,.F.) ;
#68465=ORIENTED_EDGE('',*,*,#48861,.T.) ;
#68466=ORIENTED_EDGE('',*,*,#48098,.F.) ;
#68467=ORIENTED_EDGE('',*,*,#48862,.F.) ;
#68468=ORIENTED_EDGE('',*,*,#48122,.F.) ;
#68469=ORIENTED_EDGE('',*,*,#44180,.F.) ;
#68470=ORIENTED_EDGE('',*,*,#48123,.F.) ;
#68471=ORIENTED_EDGE('',*,*,#48862,.T.) ;
#68472=ORIENTED_EDGE('',*,*,#48127,.F.) ;
#68473=ORIENTED_EDGE('',*,*,#47525,.F.) ;
#68474=ORIENTED_EDGE('',*,*,#47528,.F.) ;
#68475=ORIENTED_EDGE('',*,*,#48128,.F.) ;
#68476=ORIENTED_EDGE('',*,*,#48863,.F.) ;
#68477=ORIENTED_EDGE('',*,*,#48119,.F.) ;
#68478=ORIENTED_EDGE('',*,*,#48863,.T.) ;
#68479=ORIENTED_EDGE('',*,*,#48100,.F.) ;
#68480=ORIENTED_EDGE('',*,*,#48864,.F.) ;
#68481=ORIENTED_EDGE('',*,*,#48120,.F.) ;
#68482=ORIENTED_EDGE('',*,*,#48864,.T.) ;
#68483=ORIENTED_EDGE('',*,*,#48655,.F.) ;
#68484=ORIENTED_EDGE('',*,*,#48656,.F.) ;
#68485=ORIENTED_EDGE('',*,*,#48865,.F.) ;
#68486=ORIENTED_EDGE('',*,*,#48865,.T.) ;
#68487=ORIENTED_EDGE('',*,*,#48226,.F.) ;
#68488=ORIENTED_EDGE('',*,*,#48866,.F.) ;
#68489=ORIENTED_EDGE('',*,*,#48121,.F.) ;
#68490=ORIENTED_EDGE('',*,*,#48866,.T.) ;
#68491=ORIENTED_EDGE('',*,*,#48643,.F.) ;
#68492=ORIENTED_EDGE('',*,*,#48640,.F.) ;
#68493=ORIENTED_EDGE('',*,*,#48867,.F.) ;
#68494=ORIENTED_EDGE('',*,*,#48867,.T.) ;
#68495=ORIENTED_EDGE('',*,*,#48116,.F.) ;
#68496=ORIENTED_EDGE('',*,*,#48868,.F.) ;
#68497=ORIENTED_EDGE('',*,*,#48117,.F.) ;
#68498=ORIENTED_EDGE('',*,*,#48868,.T.) ;
#68499=ORIENTED_EDGE('',*,*,#48130,.F.) ;
#68500=ORIENTED_EDGE('',*,*,#44409,.F.) ;
#68501=ORIENTED_EDGE('',*,*,#48118,.F.) ;
#68502=ORIENTED_EDGE('',*,*,#46652,.F.) ;
#68503=ORIENTED_EDGE('',*,*,#48136,.F.) ;
#68504=ORIENTED_EDGE('',*,*,#48869,.F.) ;
#68505=ORIENTED_EDGE('',*,*,#48152,.F.) ;
#68506=ORIENTED_EDGE('',*,*,#48869,.T.) ;
#68507=ORIENTED_EDGE('',*,*,#48659,.F.) ;
#68508=ORIENTED_EDGE('',*,*,#48657,.F.) ;
#68509=ORIENTED_EDGE('',*,*,#48870,.F.) ;
#68510=ORIENTED_EDGE('',*,*,#48870,.T.) ;
#68511=ORIENTED_EDGE('',*,*,#48294,.F.) ;
#68512=ORIENTED_EDGE('',*,*,#48871,.F.) ;
#68513=ORIENTED_EDGE('',*,*,#48153,.F.) ;
#68514=ORIENTED_EDGE('',*,*,#48871,.T.) ;
#68515=ORIENTED_EDGE('',*,*,#48672,.F.) ;
#68516=ORIENTED_EDGE('',*,*,#48674,.F.) ;
#68517=ORIENTED_EDGE('',*,*,#48872,.F.) ;
#68518=ORIENTED_EDGE('',*,*,#46654,.F.) ;
#68519=ORIENTED_EDGE('',*,*,#48154,.F.) ;
#68520=ORIENTED_EDGE('',*,*,#48872,.T.) ;
#68521=ORIENTED_EDGE('',*,*,#48138,.F.) ;
#68522=ORIENTED_EDGE('',*,*,#48873,.F.) ;
#68523=ORIENTED_EDGE('',*,*,#48137,.F.) ;
#68524=ORIENTED_EDGE('',*,*,#46650,.F.) ;
#68525=ORIENTED_EDGE('',*,*,#48150,.F.) ;
#68526=ORIENTED_EDGE('',*,*,#48660,.F.) ;
#68527=ORIENTED_EDGE('',*,*,#48873,.T.) ;
#68528=ORIENTED_EDGE('',*,*,#48874,.F.) ;
#68529=ORIENTED_EDGE('',*,*,#48663,.F.) ;
#68530=ORIENTED_EDGE('',*,*,#48874,.T.) ;
#68531=ORIENTED_EDGE('',*,*,#48149,.F.) ;
#68532=ORIENTED_EDGE('',*,*,#48875,.F.) ;
#68533=ORIENTED_EDGE('',*,*,#48298,.F.) ;
#68534=ORIENTED_EDGE('',*,*,#46656,.F.) ;
#68535=ORIENTED_EDGE('',*,*,#48140,.F.) ;
#68536=ORIENTED_EDGE('',*,*,#48876,.F.) ;
#68537=ORIENTED_EDGE('',*,*,#48151,.F.) ;
#68538=ORIENTED_EDGE('',*,*,#48676,.F.) ;
#68539=ORIENTED_EDGE('',*,*,#48875,.T.) ;
#68540=ORIENTED_EDGE('',*,*,#48876,.T.) ;
#68541=ORIENTED_EDGE('',*,*,#48675,.F.) ;
#68542=ORIENTED_EDGE('',*,*,#44400,.F.) ;
#68543=ORIENTED_EDGE('',*,*,#48187,.F.) ;
#68544=ORIENTED_EDGE('',*,*,#48877,.F.) ;
#68545=ORIENTED_EDGE('',*,*,#48182,.F.) ;
#68546=ORIENTED_EDGE('',*,*,#48877,.T.) ;
#68547=ORIENTED_EDGE('',*,*,#48172,.F.) ;
#68548=ORIENTED_EDGE('',*,*,#48878,.F.) ;
#68549=ORIENTED_EDGE('',*,*,#48183,.F.) ;
#68550=ORIENTED_EDGE('',*,*,#48878,.T.) ;
#68551=ORIENTED_EDGE('',*,*,#48679,.F.) ;
#68552=ORIENTED_EDGE('',*,*,#48677,.F.) ;
#68553=ORIENTED_EDGE('',*,*,#48879,.F.) ;
#68554=ORIENTED_EDGE('',*,*,#48879,.T.) ;
#68555=ORIENTED_EDGE('',*,*,#48214,.F.) ;
#68556=ORIENTED_EDGE('',*,*,#48880,.F.) ;
#68557=ORIENTED_EDGE('',*,*,#48184,.F.) ;
#68558=ORIENTED_EDGE('',*,*,#48880,.T.) ;
#68559=ORIENTED_EDGE('',*,*,#48692,.F.) ;
#68560=ORIENTED_EDGE('',*,*,#48694,.F.) ;
#68561=ORIENTED_EDGE('',*,*,#48881,.F.) ;
#68562=ORIENTED_EDGE('',*,*,#48881,.T.) ;
#68563=ORIENTED_EDGE('',*,*,#48156,.F.) ;
#68564=ORIENTED_EDGE('',*,*,#48882,.F.) ;
#68565=ORIENTED_EDGE('',*,*,#48180,.F.) ;
#68566=ORIENTED_EDGE('',*,*,#44163,.F.) ;
#68567=ORIENTED_EDGE('',*,*,#48181,.F.) ;
#68568=ORIENTED_EDGE('',*,*,#48882,.T.) ;
#68569=ORIENTED_EDGE('',*,*,#48185,.F.) ;
#68570=ORIENTED_EDGE('',*,*,#47613,.F.) ;
#68571=ORIENTED_EDGE('',*,*,#47616,.F.) ;
#68572=ORIENTED_EDGE('',*,*,#48186,.F.) ;
#68573=ORIENTED_EDGE('',*,*,#48883,.F.) ;
#68574=ORIENTED_EDGE('',*,*,#48177,.F.) ;
#68575=ORIENTED_EDGE('',*,*,#48883,.T.) ;
#68576=ORIENTED_EDGE('',*,*,#48158,.F.) ;
#68577=ORIENTED_EDGE('',*,*,#48884,.F.) ;
#68578=ORIENTED_EDGE('',*,*,#48178,.F.) ;
#68579=ORIENTED_EDGE('',*,*,#48884,.T.) ;
#68580=ORIENTED_EDGE('',*,*,#48695,.F.) ;
#68581=ORIENTED_EDGE('',*,*,#48696,.F.) ;
#68582=ORIENTED_EDGE('',*,*,#48885,.F.) ;
#68583=ORIENTED_EDGE('',*,*,#48885,.T.) ;
#68584=ORIENTED_EDGE('',*,*,#48218,.F.) ;
#68585=ORIENTED_EDGE('',*,*,#48886,.F.) ;
#68586=ORIENTED_EDGE('',*,*,#48179,.F.) ;
#68587=ORIENTED_EDGE('',*,*,#48886,.T.) ;
#68588=ORIENTED_EDGE('',*,*,#48683,.F.) ;
#68589=ORIENTED_EDGE('',*,*,#48680,.F.) ;
#68590=ORIENTED_EDGE('',*,*,#48887,.F.) ;
#68591=ORIENTED_EDGE('',*,*,#48887,.T.) ;
#68592=ORIENTED_EDGE('',*,*,#48174,.F.) ;
#68593=ORIENTED_EDGE('',*,*,#48888,.F.) ;
#68594=ORIENTED_EDGE('',*,*,#48175,.F.) ;
#68595=ORIENTED_EDGE('',*,*,#48888,.T.) ;
#68596=ORIENTED_EDGE('',*,*,#48188,.F.) ;
#68597=ORIENTED_EDGE('',*,*,#44398,.F.) ;
#68598=ORIENTED_EDGE('',*,*,#48176,.F.) ;
#68599=ORIENTED_EDGE('',*,*,#46660,.F.) ;
#68600=ORIENTED_EDGE('',*,*,#48194,.F.) ;
#68601=ORIENTED_EDGE('',*,*,#48889,.F.) ;
#68602=ORIENTED_EDGE('',*,*,#48210,.F.) ;
#68603=ORIENTED_EDGE('',*,*,#48889,.T.) ;
#68604=ORIENTED_EDGE('',*,*,#48699,.F.) ;
#68605=ORIENTED_EDGE('',*,*,#48697,.F.) ;
#68606=ORIENTED_EDGE('',*,*,#48890,.F.) ;
#68607=ORIENTED_EDGE('',*,*,#48890,.T.) ;
#68608=ORIENTED_EDGE('',*,*,#48286,.F.) ;
#68609=ORIENTED_EDGE('',*,*,#48891,.F.) ;
#68610=ORIENTED_EDGE('',*,*,#48211,.F.) ;
#68611=ORIENTED_EDGE('',*,*,#48891,.T.) ;
#68612=ORIENTED_EDGE('',*,*,#48712,.F.) ;
#68613=ORIENTED_EDGE('',*,*,#48714,.F.) ;
#68614=ORIENTED_EDGE('',*,*,#48892,.F.) ;
#68615=ORIENTED_EDGE('',*,*,#46662,.F.) ;
#68616=ORIENTED_EDGE('',*,*,#48212,.F.) ;
#68617=ORIENTED_EDGE('',*,*,#48892,.T.) ;
#68618=ORIENTED_EDGE('',*,*,#48196,.F.) ;
#68619=ORIENTED_EDGE('',*,*,#48893,.F.) ;
#68620=ORIENTED_EDGE('',*,*,#48195,.F.) ;
#68621=ORIENTED_EDGE('',*,*,#46658,.F.) ;
#68622=ORIENTED_EDGE('',*,*,#48208,.F.) ;
#68623=ORIENTED_EDGE('',*,*,#48700,.F.) ;
#68624=ORIENTED_EDGE('',*,*,#48893,.T.) ;
#68625=ORIENTED_EDGE('',*,*,#48894,.F.) ;
#68626=ORIENTED_EDGE('',*,*,#48703,.F.) ;
#68627=ORIENTED_EDGE('',*,*,#48894,.T.) ;
#68628=ORIENTED_EDGE('',*,*,#48207,.F.) ;
#68629=ORIENTED_EDGE('',*,*,#48895,.F.) ;
#68630=ORIENTED_EDGE('',*,*,#48290,.F.) ;
#68631=ORIENTED_EDGE('',*,*,#46664,.F.) ;
#68632=ORIENTED_EDGE('',*,*,#48198,.F.) ;
#68633=ORIENTED_EDGE('',*,*,#48896,.F.) ;
#68634=ORIENTED_EDGE('',*,*,#48209,.F.) ;
#68635=ORIENTED_EDGE('',*,*,#48716,.F.) ;
#68636=ORIENTED_EDGE('',*,*,#48895,.T.) ;
#68637=ORIENTED_EDGE('',*,*,#48896,.T.) ;
#68638=ORIENTED_EDGE('',*,*,#48715,.F.) ;
#79020=TOROIDAL_SURFACE('',#93349,0.9,0.1) ;
#79021=TOROIDAL_SURFACE('',#93354,1.1,0.1) ;
#79022=TOROIDAL_SURFACE('',#93366,0.9,0.1) ;
#79023=TOROIDAL_SURFACE('',#93371,1.1,0.1) ;
#79024=TOROIDAL_SURFACE('',#93383,0.9,0.1) ;
#79025=TOROIDAL_SURFACE('',#93388,1.1,0.1) ;
#79026=TOROIDAL_SURFACE('',#93400,0.9,0.1) ;
#79027=TOROIDAL_SURFACE('',#93405,1.1,0.1) ;
#79028=TOROIDAL_SURFACE('',#93417,0.9,0.1) ;
#79029=TOROIDAL_SURFACE('',#93422,1.1,0.1) ;
#79030=TOROIDAL_SURFACE('',#93434,0.9,0.1) ;
#79031=TOROIDAL_SURFACE('',#93439,1.1,0.1) ;
#79032=TOROIDAL_SURFACE('',#93451,0.9,0.1) ;
#79033=TOROIDAL_SURFACE('',#93456,1.1,0.1) ;
#79034=TOROIDAL_SURFACE('',#93468,0.9,0.1) ;
#79035=TOROIDAL_SURFACE('',#93473,1.1,0.1) ;
#79036=TOROIDAL_SURFACE('',#93485,0.9,0.1) ;
#79037=TOROIDAL_SURFACE('',#93490,0.2,0.1) ;
#79038=TOROIDAL_SURFACE('',#93495,0.2,0.1) ;
#79039=TOROIDAL_SURFACE('',#93500,0.2,0.1) ;
#79040=TOROIDAL_SURFACE('',#93505,0.2,0.1) ;
#79041=TOROIDAL_SURFACE('',#93510,0.2,0.1) ;
#79042=TOROIDAL_SURFACE('',#93515,0.2,0.1) ;
#79043=TOROIDAL_SURFACE('',#93520,0.2,0.1) ;
#79044=TOROIDAL_SURFACE('',#93525,0.2,0.1) ;
#79045=TOROIDAL_SURFACE('',#93530,0.2,0.1) ;
#79046=TOROIDAL_SURFACE('',#93535,1.1,0.1) ;
#79047=TOROIDAL_SURFACE('',#93574,0.9,0.1) ;
#79048=TOROIDAL_SURFACE('',#93579,0.2,0.1) ;
#79049=TOROIDAL_SURFACE('',#93584,1.1,0.1) ;
#79050=TOROIDAL_SURFACE('',#93982,0.2,0.1) ;
#79051=TOROIDAL_SURFACE('',#93998,0.2,0.1) ;
#79052=TOROIDAL_SURFACE('',#94000,0.2,0.1) ;
#79053=TOROIDAL_SURFACE('',#94003,0.2,0.1) ;
#79054=TOROIDAL_SURFACE('',#94016,0.2,0.1) ;
#79055=TOROIDAL_SURFACE('',#94036,0.2,0.1) ;
#79056=TOROIDAL_SURFACE('',#94047,0.2,0.1) ;
#79057=TOROIDAL_SURFACE('',#94054,0.2,0.1) ;
#79058=TOROIDAL_SURFACE('',#94060,0.2,0.1) ;
#79059=TOROIDAL_SURFACE('',#94063,0.2,0.1) ;
#79060=TOROIDAL_SURFACE('',#94077,0.2,0.1) ;
#79061=TOROIDAL_SURFACE('',#94087,0.2,0.1) ;
#79062=TOROIDAL_SURFACE('',#94109,0.2,0.1) ;
#79063=TOROIDAL_SURFACE('',#94119,0.2,0.1) ;
#79064=TOROIDAL_SURFACE('',#94137,0.2,0.1) ;
#79065=TOROIDAL_SURFACE('',#94145,0.2,0.1) ;
#79066=TOROIDAL_SURFACE('',#94159,1.75625,0.1) ;
#79067=TOROIDAL_SURFACE('',#94182,0.2,0.1) ;
#79068=TOROIDAL_SURFACE('',#94184,0.2,0.1) ;
#79069=TOROIDAL_SURFACE('',#94198,0.2,0.1) ;
#79070=TOROIDAL_SURFACE('',#94200,0.2,0.1) ;
#79071=TOROIDAL_SURFACE('',#94205,0.2,0.1) ;
#79072=TOROIDAL_SURFACE('',#94211,0.2,0.1) ;
#79073=TOROIDAL_SURFACE('',#94213,0.2,0.1) ;
#79074=TOROIDAL_SURFACE('',#94217,1.55625,0.1) ;
#79075=TOROIDAL_SURFACE('',#94219,0.199999999999999,0.1) ;
#79076=TOROIDAL_SURFACE('',#94221,0.2,0.1) ;
#79077=TOROIDAL_SURFACE('',#94229,0.2,0.1) ;
#79078=TOROIDAL_SURFACE('',#94237,0.2,0.1) ;
#79079=TOROIDAL_SURFACE('',#94336,0.3,0.1) ;
#79080=TOROIDAL_SURFACE('',#94348,0.9,0.1) ;
#79081=TOROIDAL_SURFACE('',#94349,0.9,0.1) ;
#79082=TOROIDAL_SURFACE('',#94361,0.3,0.1) ;
#79083=TOROIDAL_SURFACE('',#95049,0.2,0.1) ;
#79084=TOROIDAL_SURFACE('',#95065,0.2,0.1) ;
#79085=TOROIDAL_SURFACE('',#95067,0.2,0.1) ;
#79086=TOROIDAL_SURFACE('',#95070,0.2,0.1) ;
#79087=TOROIDAL_SURFACE('',#95083,0.2,0.1) ;
#79088=TOROIDAL_SURFACE('',#95103,0.2,0.1) ;
#79089=TOROIDAL_SURFACE('',#95114,0.2,0.1) ;
#79090=TOROIDAL_SURFACE('',#95121,0.2,0.1) ;
#79091=TOROIDAL_SURFACE('',#95127,0.2,0.1) ;
#79092=TOROIDAL_SURFACE('',#95130,0.2,0.1) ;
#79093=TOROIDAL_SURFACE('',#95140,0.2,0.1) ;
#79094=TOROIDAL_SURFACE('',#95148,0.2,0.1) ;
#79095=TOROIDAL_SURFACE('',#95162,1.75625,0.1) ;
#79096=TOROIDAL_SURFACE('',#95185,0.2,0.1) ;
#79097=TOROIDAL_SURFACE('',#95187,0.2,0.1) ;
#79098=TOROIDAL_SURFACE('',#95201,0.2,0.1) ;
#79099=TOROIDAL_SURFACE('',#95203,0.2,0.1) ;
#79100=TOROIDAL_SURFACE('',#95208,0.2,0.1) ;
#79101=TOROIDAL_SURFACE('',#95214,0.2,0.1) ;
#79102=TOROIDAL_SURFACE('',#95216,0.2,0.1) ;
#79103=TOROIDAL_SURFACE('',#95220,1.55625,0.1) ;
#79104=TOROIDAL_SURFACE('',#95222,0.199999999999999,0.1) ;
#79105=TOROIDAL_SURFACE('',#95224,0.2,0.1) ;
#79106=TOROIDAL_SURFACE('',#95232,0.2,0.1) ;
#79107=TOROIDAL_SURFACE('',#95240,0.2,0.1) ;
#79108=TOROIDAL_SURFACE('',#95254,0.2,0.1) ;
#79109=TOROIDAL_SURFACE('',#95256,0.2,0.1) ;
#79110=TOROIDAL_SURFACE('',#95261,0.2,0.1) ;
#79111=TOROIDAL_SURFACE('',#95267,0.2,0.1) ;
#79112=TOROIDAL_SURFACE('',#95269,0.2,0.1) ;
#79113=TOROIDAL_SURFACE('',#95273,1.55625,0.1) ;
#79114=TOROIDAL_SURFACE('',#95275,0.199999999999999,0.1) ;
#79115=TOROIDAL_SURFACE('',#95277,0.2,0.1) ;
#79116=TOROIDAL_SURFACE('',#95285,0.2,0.1) ;
#79117=TOROIDAL_SURFACE('',#95293,0.2,0.1) ;
#79118=TOROIDAL_SURFACE('',#95307,0.2,0.1) ;
#79119=TOROIDAL_SURFACE('',#95309,0.2,0.1) ;
#79120=TOROIDAL_SURFACE('',#95314,0.2,0.1) ;
#79121=TOROIDAL_SURFACE('',#95320,0.2,0.1) ;
#79122=TOROIDAL_SURFACE('',#95322,0.2,0.1) ;
#79123=TOROIDAL_SURFACE('',#95326,1.55625,0.1) ;
#79124=TOROIDAL_SURFACE('',#95328,0.199999999999999,0.1) ;
#79125=TOROIDAL_SURFACE('',#95330,0.2,0.1) ;
#79126=TOROIDAL_SURFACE('',#95338,0.2,0.1) ;
#79127=TOROIDAL_SURFACE('',#95346,0.2,0.1) ;
#79128=TOROIDAL_SURFACE('',#95360,0.2,0.1) ;
#79129=TOROIDAL_SURFACE('',#95362,0.2,0.1) ;
#79130=TOROIDAL_SURFACE('',#95367,0.2,0.1) ;
#79131=TOROIDAL_SURFACE('',#95373,0.2,0.1) ;
#79132=TOROIDAL_SURFACE('',#95375,0.2,0.1) ;
#79133=TOROIDAL_SURFACE('',#95379,1.55625,0.1) ;
#79134=TOROIDAL_SURFACE('',#95381,0.199999999999999,0.1) ;
#79135=TOROIDAL_SURFACE('',#95383,0.2,0.1) ;
#79136=TOROIDAL_SURFACE('',#95391,0.2,0.1) ;
#79137=TOROIDAL_SURFACE('',#95399,0.2,0.1) ;
#79138=TOROIDAL_SURFACE('',#95413,0.2,0.1) ;
#79139=TOROIDAL_SURFACE('',#95415,0.2,0.1) ;
#79140=TOROIDAL_SURFACE('',#95420,0.2,0.1) ;
#79141=TOROIDAL_SURFACE('',#95426,0.2,0.1) ;
#79142=TOROIDAL_SURFACE('',#95428,0.2,0.1) ;
#79143=TOROIDAL_SURFACE('',#95432,1.55625,0.1) ;
#79144=TOROIDAL_SURFACE('',#95434,0.199999999999999,0.1) ;
#79145=TOROIDAL_SURFACE('',#95436,0.2,0.1) ;
#79146=TOROIDAL_SURFACE('',#95444,0.2,0.1) ;
#79147=TOROIDAL_SURFACE('',#95452,0.2,0.1) ;
#79148=TOROIDAL_SURFACE('',#95466,0.2,0.1) ;
#79149=TOROIDAL_SURFACE('',#95468,0.2,0.1) ;
#79150=TOROIDAL_SURFACE('',#95473,0.2,0.1) ;
#79151=TOROIDAL_SURFACE('',#95479,0.2,0.1) ;
#79152=TOROIDAL_SURFACE('',#95481,0.2,0.1) ;
#79153=TOROIDAL_SURFACE('',#95485,1.55625,0.1) ;
#79154=TOROIDAL_SURFACE('',#95487,0.199999999999999,0.1) ;
#79155=TOROIDAL_SURFACE('',#95489,0.2,0.1) ;
#79156=TOROIDAL_SURFACE('',#95497,0.2,0.1) ;
#79157=TOROIDAL_SURFACE('',#95505,0.2,0.1) ;
#79158=TOROIDAL_SURFACE('',#95519,0.2,0.1) ;
#79159=TOROIDAL_SURFACE('',#95521,0.2,0.1) ;
#79160=TOROIDAL_SURFACE('',#95526,0.2,0.1) ;
#79161=TOROIDAL_SURFACE('',#95532,0.2,0.1) ;
#79162=TOROIDAL_SURFACE('',#95534,0.2,0.1) ;
#79163=TOROIDAL_SURFACE('',#95538,1.55625,0.1) ;
#79164=TOROIDAL_SURFACE('',#95540,0.199999999999999,0.1) ;
#79165=TOROIDAL_SURFACE('',#95542,0.2,0.1) ;
#79166=TOROIDAL_SURFACE('',#95550,0.2,0.1) ;
#79167=TOROIDAL_SURFACE('',#95558,0.2,0.1) ;
#79168=TOROIDAL_SURFACE('',#95572,0.2,0.1) ;
#79169=TOROIDAL_SURFACE('',#95574,0.2,0.1) ;
#79170=TOROIDAL_SURFACE('',#95579,0.2,0.1) ;
#79171=TOROIDAL_SURFACE('',#95585,0.2,0.1) ;
#79172=TOROIDAL_SURFACE('',#95587,0.2,0.1) ;
#79173=TOROIDAL_SURFACE('',#95591,1.55625,0.1) ;
#79174=TOROIDAL_SURFACE('',#95593,0.199999999999999,0.1) ;
#79175=TOROIDAL_SURFACE('',#95595,0.2,0.1) ;
#79176=TOROIDAL_SURFACE('',#95603,0.2,0.1) ;
#79177=TOROIDAL_SURFACE('',#95611,0.2,0.1) ;
#79178=TOROIDAL_SURFACE('',#95625,0.2,0.1) ;
#79179=TOROIDAL_SURFACE('',#95627,0.2,0.1) ;
#79180=TOROIDAL_SURFACE('',#95632,0.2,0.1) ;
#79181=TOROIDAL_SURFACE('',#95638,0.2,0.1) ;
#79182=TOROIDAL_SURFACE('',#95640,0.2,0.1) ;
#79183=TOROIDAL_SURFACE('',#95644,1.55625,0.1) ;
#79184=TOROIDAL_SURFACE('',#95646,0.199999999999999,0.1) ;
#79185=TOROIDAL_SURFACE('',#95648,0.2,0.1) ;
#79186=TOROIDAL_SURFACE('',#95656,0.2,0.1) ;
#79187=TOROIDAL_SURFACE('',#95664,0.2,0.1) ;
#79188=TOROIDAL_SURFACE('',#95679,0.2,0.1) ;
#79189=TOROIDAL_SURFACE('',#95695,0.2,0.1) ;
#79190=TOROIDAL_SURFACE('',#95697,0.2,0.1) ;
#79191=TOROIDAL_SURFACE('',#95700,0.2,0.1) ;
#79192=TOROIDAL_SURFACE('',#95713,0.2,0.1) ;
#79193=TOROIDAL_SURFACE('',#95733,0.2,0.1) ;
#79194=TOROIDAL_SURFACE('',#95744,0.2,0.1) ;
#79195=TOROIDAL_SURFACE('',#95751,0.2,0.1) ;
#79196=TOROIDAL_SURFACE('',#95757,0.2,0.1) ;
#79197=TOROIDAL_SURFACE('',#95760,0.2,0.1) ;
#79198=TOROIDAL_SURFACE('',#95770,0.2,0.1) ;
#79199=TOROIDAL_SURFACE('',#95778,0.2,0.1) ;
#79200=TOROIDAL_SURFACE('',#95792,1.75625,0.1) ;
#79201=TOROIDAL_SURFACE('',#95815,0.2,0.1) ;
#79202=TOROIDAL_SURFACE('',#95817,0.2,0.1) ;
#79203=TOROIDAL_SURFACE('',#95832,0.2,0.1) ;
#79204=TOROIDAL_SURFACE('',#95848,0.2,0.1) ;
#79205=TOROIDAL_SURFACE('',#95850,0.2,0.1) ;
#79206=TOROIDAL_SURFACE('',#95853,0.2,0.1) ;
#79207=TOROIDAL_SURFACE('',#95866,0.2,0.1) ;
#79208=TOROIDAL_SURFACE('',#95886,0.2,0.1) ;
#79209=TOROIDAL_SURFACE('',#95897,0.2,0.1) ;
#79210=TOROIDAL_SURFACE('',#95904,0.2,0.1) ;
#79211=TOROIDAL_SURFACE('',#95910,0.2,0.1) ;
#79212=TOROIDAL_SURFACE('',#95913,0.2,0.1) ;
#79213=TOROIDAL_SURFACE('',#95923,0.2,0.1) ;
#79214=TOROIDAL_SURFACE('',#95931,0.2,0.1) ;
#79215=TOROIDAL_SURFACE('',#95945,1.75625,0.1) ;
#79216=TOROIDAL_SURFACE('',#95968,0.2,0.1) ;
#79217=TOROIDAL_SURFACE('',#95970,0.2,0.1) ;
#79218=TOROIDAL_SURFACE('',#95985,0.2,0.1) ;
#79219=TOROIDAL_SURFACE('',#96001,0.2,0.1) ;
#79220=TOROIDAL_SURFACE('',#96003,0.2,0.1) ;
#79221=TOROIDAL_SURFACE('',#96006,0.2,0.1) ;
#79222=TOROIDAL_SURFACE('',#96019,0.2,0.1) ;
#79223=TOROIDAL_SURFACE('',#96039,0.2,0.1) ;
#79224=TOROIDAL_SURFACE('',#96050,0.2,0.1) ;
#79225=TOROIDAL_SURFACE('',#96057,0.2,0.1) ;
#79226=TOROIDAL_SURFACE('',#96063,0.2,0.1) ;
#79227=TOROIDAL_SURFACE('',#96066,0.2,0.1) ;
#79228=TOROIDAL_SURFACE('',#96076,0.2,0.1) ;
#79229=TOROIDAL_SURFACE('',#96084,0.2,0.1) ;
#79230=TOROIDAL_SURFACE('',#96098,1.75625,0.1) ;
#79231=TOROIDAL_SURFACE('',#96121,0.2,0.1) ;
#79232=TOROIDAL_SURFACE('',#96123,0.2,0.1) ;
#79233=TOROIDAL_SURFACE('',#96138,0.2,0.1) ;
#79234=TOROIDAL_SURFACE('',#96154,0.2,0.1) ;
#79235=TOROIDAL_SURFACE('',#96156,0.2,0.1) ;
#79236=TOROIDAL_SURFACE('',#96159,0.2,0.1) ;
#79237=TOROIDAL_SURFACE('',#96172,0.2,0.1) ;
#79238=TOROIDAL_SURFACE('',#96192,0.2,0.1) ;
#79239=TOROIDAL_SURFACE('',#96203,0.2,0.1) ;
#79240=TOROIDAL_SURFACE('',#96210,0.2,0.1) ;
#79241=TOROIDAL_SURFACE('',#96216,0.2,0.1) ;
#79242=TOROIDAL_SURFACE('',#96219,0.2,0.1) ;
#79243=TOROIDAL_SURFACE('',#96229,0.2,0.1) ;
#79244=TOROIDAL_SURFACE('',#96237,0.2,0.1) ;
#79245=TOROIDAL_SURFACE('',#96251,1.75625,0.1) ;
#79246=TOROIDAL_SURFACE('',#96274,0.2,0.1) ;
#79247=TOROIDAL_SURFACE('',#96276,0.2,0.1) ;
#79248=TOROIDAL_SURFACE('',#96291,0.2,0.1) ;
#79249=TOROIDAL_SURFACE('',#96307,0.2,0.1) ;
#79250=TOROIDAL_SURFACE('',#96309,0.2,0.1) ;
#79251=TOROIDAL_SURFACE('',#96312,0.2,0.1) ;
#79252=TOROIDAL_SURFACE('',#96325,0.2,0.1) ;
#79253=TOROIDAL_SURFACE('',#96345,0.2,0.1) ;
#79254=TOROIDAL_SURFACE('',#96356,0.2,0.1) ;
#79255=TOROIDAL_SURFACE('',#96363,0.2,0.1) ;
#79256=TOROIDAL_SURFACE('',#96369,0.2,0.1) ;
#79257=TOROIDAL_SURFACE('',#96372,0.2,0.1) ;
#79258=TOROIDAL_SURFACE('',#96382,0.2,0.1) ;
#79259=TOROIDAL_SURFACE('',#96390,0.2,0.1) ;
#79260=TOROIDAL_SURFACE('',#96404,1.75625,0.1) ;
#79261=TOROIDAL_SURFACE('',#96427,0.2,0.1) ;
#79262=TOROIDAL_SURFACE('',#96429,0.2,0.1) ;
#79263=TOROIDAL_SURFACE('',#96444,0.2,0.1) ;
#79264=TOROIDAL_SURFACE('',#96460,0.2,0.1) ;
#79265=TOROIDAL_SURFACE('',#96462,0.2,0.1) ;
#79266=TOROIDAL_SURFACE('',#96465,0.2,0.1) ;
#79267=TOROIDAL_SURFACE('',#96478,0.2,0.1) ;
#79268=TOROIDAL_SURFACE('',#96498,0.2,0.1) ;
#79269=TOROIDAL_SURFACE('',#96509,0.2,0.1) ;
#79270=TOROIDAL_SURFACE('',#96516,0.2,0.1) ;
#79271=TOROIDAL_SURFACE('',#96522,0.2,0.1) ;
#79272=TOROIDAL_SURFACE('',#96525,0.2,0.1) ;
#79273=TOROIDAL_SURFACE('',#96535,0.2,0.1) ;
#79274=TOROIDAL_SURFACE('',#96543,0.2,0.1) ;
#79275=TOROIDAL_SURFACE('',#96557,1.75625,0.1) ;
#79276=TOROIDAL_SURFACE('',#96580,0.2,0.1) ;
#79277=TOROIDAL_SURFACE('',#96582,0.2,0.1) ;
#79278=TOROIDAL_SURFACE('',#96597,0.2,0.1) ;
#79279=TOROIDAL_SURFACE('',#96613,0.2,0.1) ;
#79280=TOROIDAL_SURFACE('',#96615,0.2,0.1) ;
#79281=TOROIDAL_SURFACE('',#96618,0.2,0.1) ;
#79282=TOROIDAL_SURFACE('',#96631,0.2,0.1) ;
#79283=TOROIDAL_SURFACE('',#96651,0.2,0.1) ;
#79284=TOROIDAL_SURFACE('',#96662,0.2,0.1) ;
#79285=TOROIDAL_SURFACE('',#96669,0.2,0.1) ;
#79286=TOROIDAL_SURFACE('',#96675,0.2,0.1) ;
#79287=TOROIDAL_SURFACE('',#96678,0.2,0.1) ;
#79288=TOROIDAL_SURFACE('',#96688,0.2,0.1) ;
#79289=TOROIDAL_SURFACE('',#96696,0.2,0.1) ;
#79290=TOROIDAL_SURFACE('',#96710,1.75625,0.1) ;
#79291=TOROIDAL_SURFACE('',#96733,0.2,0.1) ;
#79292=TOROIDAL_SURFACE('',#96735,0.2,0.1) ;
#79293=TOROIDAL_SURFACE('',#96750,0.2,0.1) ;
#79294=TOROIDAL_SURFACE('',#96766,0.2,0.1) ;
#79295=TOROIDAL_SURFACE('',#96768,0.2,0.1) ;
#79296=TOROIDAL_SURFACE('',#96771,0.2,0.1) ;
#79297=TOROIDAL_SURFACE('',#96784,0.2,0.1) ;
#79298=TOROIDAL_SURFACE('',#96804,0.2,0.1) ;
#79299=TOROIDAL_SURFACE('',#96815,0.2,0.1) ;
#79300=TOROIDAL_SURFACE('',#96822,0.2,0.1) ;
#79301=TOROIDAL_SURFACE('',#96828,0.2,0.1) ;
#79302=TOROIDAL_SURFACE('',#96831,0.2,0.1) ;
#79303=TOROIDAL_SURFACE('',#96841,0.2,0.1) ;
#79304=TOROIDAL_SURFACE('',#96849,0.2,0.1) ;
#79305=TOROIDAL_SURFACE('',#96863,1.75625,0.1) ;
#79306=TOROIDAL_SURFACE('',#96886,0.2,0.1) ;
#79307=TOROIDAL_SURFACE('',#96888,0.2,0.1) ;
#79308=TOROIDAL_SURFACE('',#97755,0.3,0.1) ;
#79309=TOROIDAL_SURFACE('',#97767,0.9,0.1) ;
#79310=TOROIDAL_SURFACE('',#97768,0.9,0.1) ;
#79311=TOROIDAL_SURFACE('',#97780,0.3,0.1) ;
#79312=TOROIDAL_SURFACE('',#97799,0.3,0.1) ;
#79313=TOROIDAL_SURFACE('',#97811,0.9,0.1) ;
#79314=TOROIDAL_SURFACE('',#97812,0.9,0.1) ;
#79315=TOROIDAL_SURFACE('',#97824,0.3,0.1) ;
#79316=TOROIDAL_SURFACE('',#97843,0.3,0.1) ;
#79317=TOROIDAL_SURFACE('',#97855,0.9,0.1) ;
#79318=TOROIDAL_SURFACE('',#97856,0.9,0.1) ;
#79319=TOROIDAL_SURFACE('',#97868,0.3,0.1) ;
#79320=TOROIDAL_SURFACE('',#97887,0.3,0.1) ;
#79321=TOROIDAL_SURFACE('',#97899,0.9,0.1) ;
#79322=TOROIDAL_SURFACE('',#97900,0.9,0.1) ;
#79323=TOROIDAL_SURFACE('',#97912,0.3,0.1) ;
#79324=TOROIDAL_SURFACE('',#97931,0.3,0.1) ;
#79325=TOROIDAL_SURFACE('',#97943,0.9,0.1) ;
#79326=TOROIDAL_SURFACE('',#97944,0.9,0.1) ;
#79327=TOROIDAL_SURFACE('',#97956,0.3,0.1) ;
#79328=TOROIDAL_SURFACE('',#97975,0.3,0.1) ;
#79329=TOROIDAL_SURFACE('',#97987,0.9,0.1) ;
#79330=TOROIDAL_SURFACE('',#97988,0.9,0.1) ;
#79331=TOROIDAL_SURFACE('',#98000,0.3,0.1) ;
#79332=TOROIDAL_SURFACE('',#98019,0.3,0.1) ;
#79333=TOROIDAL_SURFACE('',#98031,0.9,0.1) ;
#79334=TOROIDAL_SURFACE('',#98032,0.9,0.1) ;
#79335=TOROIDAL_SURFACE('',#98044,0.3,0.1) ;
#79336=TOROIDAL_SURFACE('',#98063,0.3,0.1) ;
#79337=TOROIDAL_SURFACE('',#98075,0.9,0.1) ;
#79338=TOROIDAL_SURFACE('',#98076,0.9,0.1) ;
#79339=TOROIDAL_SURFACE('',#98088,0.3,0.1) ;
#79340=TOROIDAL_SURFACE('',#98107,0.3,0.1) ;
#79341=TOROIDAL_SURFACE('',#98119,0.9,0.1) ;
#79342=TOROIDAL_SURFACE('',#98120,0.9,0.1) ;
#79343=TOROIDAL_SURFACE('',#98132,0.3,0.1) ;
#80780=STYLED_ITEM('',(#170169),#86488) ;
#80781=STYLED_ITEM('',(#170169),#86489) ;
#80782=STYLED_ITEM('',(#170169),#86490) ;
#80783=STYLED_ITEM('',(#170169),#86491) ;
#80784=STYLED_ITEM('',(#170169),#86492) ;
#80785=STYLED_ITEM('',(#170169),#86493) ;
#80786=STYLED_ITEM('',(#170169),#86494) ;
#80787=STYLED_ITEM('',(#170169),#86495) ;
#80788=STYLED_ITEM('',(#170169),#86496) ;
#80789=STYLED_ITEM('',(#170169),#86497) ;
#80790=STYLED_ITEM('',(#170169),#86498) ;
#80791=STYLED_ITEM('',(#170169),#86499) ;
#80792=STYLED_ITEM('',(#170169),#86500) ;
#80793=STYLED_ITEM('',(#170169),#86501) ;
#80794=STYLED_ITEM('',(#170169),#86502) ;
#80795=STYLED_ITEM('',(#170169),#86503) ;
#80796=STYLED_ITEM('',(#170169),#86504) ;
#80797=STYLED_ITEM('',(#170169),#86505) ;
#80798=STYLED_ITEM('',(#170169),#86506) ;
#80799=STYLED_ITEM('',(#170169),#86507) ;
#80800=STYLED_ITEM('',(#170169),#86508) ;
#80801=STYLED_ITEM('',(#170169),#86509) ;
#80802=STYLED_ITEM('',(#170169),#86510) ;
#80803=STYLED_ITEM('',(#170169),#86511) ;
#80804=STYLED_ITEM('',(#170169),#86512) ;
#80805=STYLED_ITEM('',(#170169),#86513) ;
#80806=STYLED_ITEM('',(#170169),#86514) ;
#80807=STYLED_ITEM('',(#170169),#86515) ;
#80808=STYLED_ITEM('',(#170169),#86516) ;
#80809=STYLED_ITEM('',(#170169),#86517) ;
#80810=STYLED_ITEM('',(#170169),#86518) ;
#80811=STYLED_ITEM('',(#170169),#86519) ;
#80812=STYLED_ITEM('',(#170169),#86520) ;
#80813=STYLED_ITEM('',(#170169),#86521) ;
#80814=STYLED_ITEM('',(#170169),#86522) ;
#80815=STYLED_ITEM('',(#170169),#86523) ;
#80816=STYLED_ITEM('',(#170169),#86524) ;
#80817=STYLED_ITEM('',(#170169),#86525) ;
#80818=STYLED_ITEM('',(#170169),#86526) ;
#80819=STYLED_ITEM('',(#170169),#86527) ;
#80820=STYLED_ITEM('',(#170169),#86528) ;
#80821=STYLED_ITEM('',(#170169),#86529) ;
#80822=STYLED_ITEM('',(#170169),#86530) ;
#80823=STYLED_ITEM('',(#170169),#86531) ;
#80824=STYLED_ITEM('',(#170169),#86532) ;
#80825=STYLED_ITEM('',(#170169),#86533) ;
#80826=STYLED_ITEM('',(#170169),#86534) ;
#80827=STYLED_ITEM('',(#170169),#86535) ;
#80828=STYLED_ITEM('',(#170169),#86536) ;
#80829=STYLED_ITEM('',(#170169),#86537) ;
#80830=STYLED_ITEM('',(#170169),#86538) ;
#80831=STYLED_ITEM('',(#170169),#86539) ;
#80832=STYLED_ITEM('',(#170169),#86540) ;
#80833=STYLED_ITEM('',(#170169),#86541) ;
#80834=STYLED_ITEM('',(#170169),#86542) ;
#80835=STYLED_ITEM('',(#170169),#86543) ;
#80836=STYLED_ITEM('',(#170169),#86544) ;
#80837=STYLED_ITEM('',(#170169),#86545) ;
#80838=STYLED_ITEM('',(#170169),#86546) ;
#80839=STYLED_ITEM('',(#170169),#86547) ;
#80840=STYLED_ITEM('',(#170169),#86548) ;
#80841=STYLED_ITEM('',(#170169),#86549) ;
#80842=STYLED_ITEM('',(#170169),#86550) ;
#80843=STYLED_ITEM('',(#170169),#86551) ;
#80844=STYLED_ITEM('',(#170169),#86552) ;
#80845=STYLED_ITEM('',(#170169),#86553) ;
#80846=STYLED_ITEM('',(#170169),#86554) ;
#80847=STYLED_ITEM('',(#170169),#86555) ;
#80848=STYLED_ITEM('',(#170169),#86556) ;
#80849=STYLED_ITEM('',(#170169),#86557) ;
#80850=STYLED_ITEM('',(#170169),#86558) ;
#80851=STYLED_ITEM('',(#170169),#86559) ;
#80852=STYLED_ITEM('',(#170169),#86560) ;
#80853=STYLED_ITEM('',(#170169),#86561) ;
#80854=STYLED_ITEM('',(#170169),#86562) ;
#80855=STYLED_ITEM('',(#170169),#86563) ;
#80856=STYLED_ITEM('',(#170169),#86564) ;
#80857=STYLED_ITEM('',(#170169),#86565) ;
#80858=STYLED_ITEM('',(#170169),#86566) ;
#80859=STYLED_ITEM('',(#170169),#86567) ;
#80860=STYLED_ITEM('',(#170169),#86568) ;
#80861=STYLED_ITEM('',(#170169),#86569) ;
#80862=STYLED_ITEM('',(#170169),#86570) ;
#80863=STYLED_ITEM('',(#170169),#86571) ;
#80864=STYLED_ITEM('',(#170169),#86572) ;
#80865=STYLED_ITEM('',(#170169),#86573) ;
#80866=STYLED_ITEM('',(#170169),#86574) ;
#80867=STYLED_ITEM('',(#170169),#86575) ;
#80868=STYLED_ITEM('',(#170169),#86576) ;
#80869=STYLED_ITEM('',(#170169),#86577) ;
#80870=STYLED_ITEM('',(#170169),#86578) ;
#80871=STYLED_ITEM('',(#170169),#86579) ;
#80872=STYLED_ITEM('',(#170169),#86580) ;
#80873=STYLED_ITEM('',(#170169),#86581) ;
#80874=STYLED_ITEM('',(#170169),#86582) ;
#80875=STYLED_ITEM('',(#170169),#86583) ;
#80876=STYLED_ITEM('',(#170169),#86584) ;
#80877=STYLED_ITEM('',(#170169),#86585) ;
#80878=STYLED_ITEM('',(#170169),#86586) ;
#80879=STYLED_ITEM('',(#170169),#86587) ;
#80880=STYLED_ITEM('',(#170169),#86588) ;
#80881=STYLED_ITEM('',(#170169),#86589) ;
#80882=STYLED_ITEM('',(#170169),#86590) ;
#80883=STYLED_ITEM('',(#170169),#86591) ;
#80884=STYLED_ITEM('',(#170169),#86592) ;
#80885=STYLED_ITEM('',(#170169),#86593) ;
#80886=STYLED_ITEM('',(#170169),#86594) ;
#80887=STYLED_ITEM('',(#170169),#86595) ;
#80888=STYLED_ITEM('',(#170169),#86596) ;
#80889=STYLED_ITEM('',(#170169),#86597) ;
#80890=STYLED_ITEM('',(#170169),#86598) ;
#80891=STYLED_ITEM('',(#170169),#86599) ;
#80892=STYLED_ITEM('',(#170169),#86600) ;
#80893=STYLED_ITEM('',(#170169),#86601) ;
#80894=STYLED_ITEM('',(#170169),#86602) ;
#80895=STYLED_ITEM('',(#170169),#86603) ;
#80896=STYLED_ITEM('',(#170169),#86604) ;
#80897=STYLED_ITEM('',(#170169),#86605) ;
#80898=STYLED_ITEM('',(#170169),#86606) ;
#80899=STYLED_ITEM('',(#170169),#86607) ;
#80900=STYLED_ITEM('',(#170169),#86608) ;
#80901=STYLED_ITEM('',(#170169),#86609) ;
#80902=STYLED_ITEM('',(#170169),#86610) ;
#80903=STYLED_ITEM('',(#170169),#86611) ;
#80904=STYLED_ITEM('',(#170169),#86612) ;
#80905=STYLED_ITEM('',(#170169),#86613) ;
#80906=STYLED_ITEM('',(#170169),#86614) ;
#80907=STYLED_ITEM('',(#170169),#86615) ;
#80908=STYLED_ITEM('',(#170169),#86616) ;
#80909=STYLED_ITEM('',(#170169),#86617) ;
#80910=STYLED_ITEM('',(#170169),#86618) ;
#80911=STYLED_ITEM('',(#170169),#86619) ;
#80912=STYLED_ITEM('',(#170169),#86620) ;
#80913=STYLED_ITEM('',(#170169),#86621) ;
#80914=STYLED_ITEM('',(#170169),#86622) ;
#80915=STYLED_ITEM('',(#170169),#86623) ;
#80916=STYLED_ITEM('',(#170169),#86624) ;
#80917=STYLED_ITEM('',(#170169),#86625) ;
#80918=STYLED_ITEM('',(#170169),#86626) ;
#80919=STYLED_ITEM('',(#170169),#86627) ;
#80920=STYLED_ITEM('',(#170169),#86628) ;
#80921=STYLED_ITEM('',(#170169),#86629) ;
#80922=STYLED_ITEM('',(#170169),#86630) ;
#80923=STYLED_ITEM('',(#170169),#86631) ;
#80924=STYLED_ITEM('',(#170169),#86632) ;
#80925=STYLED_ITEM('',(#170169),#86633) ;
#80926=STYLED_ITEM('',(#170169),#86634) ;
#80927=STYLED_ITEM('',(#170169),#86635) ;
#80928=STYLED_ITEM('',(#170169),#86636) ;
#80929=STYLED_ITEM('',(#170169),#86637) ;
#80930=STYLED_ITEM('',(#170169),#86638) ;
#80931=STYLED_ITEM('',(#170169),#86639) ;
#80932=STYLED_ITEM('',(#170169),#86640) ;
#80933=STYLED_ITEM('',(#170169),#86641) ;
#80934=STYLED_ITEM('',(#170169),#86642) ;
#80935=STYLED_ITEM('',(#170169),#86643) ;
#80936=STYLED_ITEM('',(#170169),#86644) ;
#80937=STYLED_ITEM('',(#170169),#86645) ;
#80938=STYLED_ITEM('',(#170169),#86646) ;
#80939=STYLED_ITEM('',(#170169),#86647) ;
#80940=STYLED_ITEM('',(#170169),#86648) ;
#80941=STYLED_ITEM('',(#170169),#86649) ;
#80942=STYLED_ITEM('',(#170169),#86650) ;
#80943=STYLED_ITEM('',(#170169),#86651) ;
#80944=STYLED_ITEM('',(#170169),#86652) ;
#80945=STYLED_ITEM('',(#170169),#86653) ;
#80946=STYLED_ITEM('',(#170169),#86654) ;
#80947=STYLED_ITEM('',(#170169),#86655) ;
#80948=STYLED_ITEM('',(#170169),#86656) ;
#80949=STYLED_ITEM('',(#170169),#86657) ;
#80950=STYLED_ITEM('',(#170169),#86658) ;
#80951=STYLED_ITEM('',(#170169),#86659) ;
#80952=STYLED_ITEM('',(#170169),#86660) ;
#80953=STYLED_ITEM('',(#170169),#86661) ;
#80954=STYLED_ITEM('',(#170169),#86662) ;
#80955=STYLED_ITEM('',(#170169),#86663) ;
#80956=STYLED_ITEM('',(#170169),#86664) ;
#80957=STYLED_ITEM('',(#170169),#86665) ;
#80958=STYLED_ITEM('',(#170169),#86666) ;
#80959=STYLED_ITEM('',(#170169),#86667) ;
#80960=STYLED_ITEM('',(#170169),#86668) ;
#80961=STYLED_ITEM('',(#170169),#86669) ;
#80962=STYLED_ITEM('',(#170169),#86670) ;
#80963=STYLED_ITEM('',(#170169),#86671) ;
#80964=STYLED_ITEM('',(#170169),#86672) ;
#80965=STYLED_ITEM('',(#170169),#86673) ;
#80966=STYLED_ITEM('',(#170169),#86674) ;
#80967=STYLED_ITEM('',(#170169),#86675) ;
#80968=STYLED_ITEM('',(#170169),#86676) ;
#80969=STYLED_ITEM('',(#170169),#86677) ;
#80970=STYLED_ITEM('',(#170169),#86678) ;
#80971=STYLED_ITEM('',(#170169),#86679) ;
#80972=STYLED_ITEM('',(#170169),#86680) ;
#80973=STYLED_ITEM('',(#170169),#86681) ;
#80974=STYLED_ITEM('',(#170169),#86682) ;
#80975=STYLED_ITEM('',(#170169),#86683) ;
#80976=STYLED_ITEM('',(#170169),#86684) ;
#80977=STYLED_ITEM('',(#170169),#86685) ;
#80978=STYLED_ITEM('',(#170169),#86686) ;
#80979=STYLED_ITEM('',(#170169),#86687) ;
#80980=STYLED_ITEM('',(#170169),#86688) ;
#80981=STYLED_ITEM('',(#170169),#86689) ;
#80982=STYLED_ITEM('',(#170169),#86690) ;
#80983=STYLED_ITEM('',(#170169),#86691) ;
#80984=STYLED_ITEM('',(#170169),#86692) ;
#80985=STYLED_ITEM('',(#170169),#86693) ;
#80986=STYLED_ITEM('',(#170169),#86694) ;
#80987=STYLED_ITEM('',(#170169),#86695) ;
#80988=STYLED_ITEM('',(#170169),#86696) ;
#80989=STYLED_ITEM('',(#170169),#86697) ;
#80990=STYLED_ITEM('',(#170169),#86698) ;
#80991=STYLED_ITEM('',(#170169),#86699) ;
#80992=STYLED_ITEM('',(#170169),#86700) ;
#80993=STYLED_ITEM('',(#170169),#86701) ;
#80994=STYLED_ITEM('',(#170169),#86702) ;
#80995=STYLED_ITEM('',(#170169),#86703) ;
#80996=STYLED_ITEM('',(#170169),#86704) ;
#80997=STYLED_ITEM('',(#170169),#86705) ;
#80998=STYLED_ITEM('',(#170169),#86706) ;
#80999=STYLED_ITEM('',(#170169),#86707) ;
#81000=STYLED_ITEM('',(#170169),#86708) ;
#81001=STYLED_ITEM('',(#170169),#86709) ;
#81002=STYLED_ITEM('',(#170169),#86710) ;
#81003=STYLED_ITEM('',(#170169),#86711) ;
#81004=STYLED_ITEM('',(#170169),#86712) ;
#81005=STYLED_ITEM('',(#170169),#86713) ;
#81006=STYLED_ITEM('',(#170169),#86714) ;
#81007=STYLED_ITEM('',(#170169),#86715) ;
#81008=STYLED_ITEM('',(#170169),#86716) ;
#81009=STYLED_ITEM('',(#170169),#86717) ;
#81010=STYLED_ITEM('',(#170169),#86718) ;
#81011=STYLED_ITEM('',(#170169),#86719) ;
#81012=STYLED_ITEM('',(#170169),#86720) ;
#81013=STYLED_ITEM('',(#170169),#86721) ;
#81014=STYLED_ITEM('',(#170169),#86722) ;
#81015=STYLED_ITEM('',(#170169),#86723) ;
#81016=STYLED_ITEM('',(#170169),#86724) ;
#81017=STYLED_ITEM('',(#170169),#86725) ;
#81018=STYLED_ITEM('',(#170169),#86726) ;
#81019=STYLED_ITEM('',(#170169),#86727) ;
#81020=STYLED_ITEM('',(#170169),#86728) ;
#81021=STYLED_ITEM('',(#170169),#86729) ;
#81022=STYLED_ITEM('',(#170169),#86730) ;
#81023=STYLED_ITEM('',(#170169),#86731) ;
#81024=STYLED_ITEM('',(#170169),#86732) ;
#81025=STYLED_ITEM('',(#170169),#86733) ;
#81026=STYLED_ITEM('',(#170169),#86734) ;
#81027=STYLED_ITEM('',(#170169),#86735) ;
#81028=STYLED_ITEM('',(#170169),#86736) ;
#81029=STYLED_ITEM('',(#170169),#86737) ;
#81030=STYLED_ITEM('',(#170169),#86738) ;
#81031=STYLED_ITEM('',(#170169),#86739) ;
#81032=STYLED_ITEM('',(#170169),#86740) ;
#81033=STYLED_ITEM('',(#170169),#86741) ;
#81034=STYLED_ITEM('',(#170169),#86742) ;
#81035=STYLED_ITEM('',(#170169),#86743) ;
#81036=STYLED_ITEM('',(#170169),#86744) ;
#81037=STYLED_ITEM('',(#170169),#86745) ;
#81038=STYLED_ITEM('',(#170169),#86746) ;
#81039=STYLED_ITEM('',(#170169),#86747) ;
#81040=STYLED_ITEM('',(#170169),#86748) ;
#81041=STYLED_ITEM('',(#170169),#86749) ;
#81042=STYLED_ITEM('',(#170169),#86750) ;
#81043=STYLED_ITEM('',(#170169),#86751) ;
#81044=STYLED_ITEM('',(#170169),#86752) ;
#81045=STYLED_ITEM('',(#170169),#86753) ;
#81046=STYLED_ITEM('',(#170169),#86754) ;
#81047=STYLED_ITEM('',(#170169),#86755) ;
#81048=STYLED_ITEM('',(#170169),#86756) ;
#81049=STYLED_ITEM('',(#170169),#86757) ;
#81050=STYLED_ITEM('',(#170169),#86758) ;
#81051=STYLED_ITEM('',(#170169),#86759) ;
#81052=STYLED_ITEM('',(#170169),#86760) ;
#81053=STYLED_ITEM('',(#170169),#86761) ;
#81054=STYLED_ITEM('',(#170169),#86762) ;
#81055=STYLED_ITEM('',(#170169),#86763) ;
#81056=STYLED_ITEM('',(#170169),#86764) ;
#81057=STYLED_ITEM('',(#170169),#86765) ;
#81058=STYLED_ITEM('',(#170169),#86766) ;
#81059=STYLED_ITEM('',(#170169),#86767) ;
#81060=STYLED_ITEM('',(#170169),#86768) ;
#81061=STYLED_ITEM('',(#170169),#86769) ;
#81062=STYLED_ITEM('',(#170169),#86770) ;
#81063=STYLED_ITEM('',(#170169),#86771) ;
#81064=STYLED_ITEM('',(#170169),#86772) ;
#81065=STYLED_ITEM('',(#170169),#86773) ;
#81066=STYLED_ITEM('',(#170169),#86774) ;
#81067=STYLED_ITEM('',(#170169),#86775) ;
#81068=STYLED_ITEM('',(#170169),#86776) ;
#81069=STYLED_ITEM('',(#170169),#86777) ;
#81070=STYLED_ITEM('',(#170169),#86778) ;
#81071=STYLED_ITEM('',(#170169),#86779) ;
#81072=STYLED_ITEM('',(#170169),#86780) ;
#81073=STYLED_ITEM('',(#170169),#86781) ;
#81074=STYLED_ITEM('',(#170169),#86782) ;
#81075=STYLED_ITEM('',(#170171),#86783) ;
#81076=STYLED_ITEM('',(#170171),#86784) ;
#81077=STYLED_ITEM('',(#170171),#86785) ;
#81078=STYLED_ITEM('',(#170171),#86786) ;
#81079=STYLED_ITEM('',(#170171),#86787) ;
#81080=STYLED_ITEM('',(#170171),#86788) ;
#81081=STYLED_ITEM('',(#170171),#86789) ;
#81082=STYLED_ITEM('',(#170171),#86790) ;
#81083=STYLED_ITEM('',(#170171),#86791) ;
#81084=STYLED_ITEM('',(#170171),#86792) ;
#81085=STYLED_ITEM('',(#170171),#86793) ;
#81086=STYLED_ITEM('',(#170171),#86794) ;
#81087=STYLED_ITEM('',(#170171),#86795) ;
#81088=STYLED_ITEM('',(#170171),#86796) ;
#81089=STYLED_ITEM('',(#170171),#86797) ;
#81090=STYLED_ITEM('',(#170171),#86798) ;
#81091=STYLED_ITEM('',(#170171),#86799) ;
#81092=STYLED_ITEM('',(#170171),#86800) ;
#81093=STYLED_ITEM('',(#170171),#86801) ;
#81094=STYLED_ITEM('',(#170171),#86802) ;
#81095=STYLED_ITEM('',(#170171),#86803) ;
#81096=STYLED_ITEM('',(#170171),#86804) ;
#81097=STYLED_ITEM('',(#170171),#86805) ;
#81098=STYLED_ITEM('',(#170171),#86806) ;
#81099=STYLED_ITEM('',(#170171),#86807) ;
#81100=STYLED_ITEM('',(#170171),#86808) ;
#81101=STYLED_ITEM('',(#170171),#86809) ;
#81102=STYLED_ITEM('',(#170171),#86810) ;
#81103=STYLED_ITEM('',(#170171),#86811) ;
#81104=STYLED_ITEM('',(#170171),#86812) ;
#81105=STYLED_ITEM('',(#170171),#86813) ;
#81106=STYLED_ITEM('',(#170171),#86814) ;
#81107=STYLED_ITEM('',(#170171),#86815) ;
#81108=STYLED_ITEM('',(#170171),#86816) ;
#81109=STYLED_ITEM('',(#170171),#86817) ;
#81110=STYLED_ITEM('',(#170171),#86818) ;
#81111=STYLED_ITEM('',(#170171),#86819) ;
#81112=STYLED_ITEM('',(#170171),#86820) ;
#81113=STYLED_ITEM('',(#170171),#86821) ;
#81114=STYLED_ITEM('',(#170171),#86822) ;
#81115=STYLED_ITEM('',(#170171),#86823) ;
#81116=STYLED_ITEM('',(#170171),#86824) ;
#81117=STYLED_ITEM('',(#170171),#86825) ;
#81118=STYLED_ITEM('',(#170171),#86826) ;
#81119=STYLED_ITEM('',(#170171),#86827) ;
#81120=STYLED_ITEM('',(#170171),#86828) ;
#81121=STYLED_ITEM('',(#170171),#86829) ;
#81122=STYLED_ITEM('',(#170171),#86830) ;
#81123=STYLED_ITEM('',(#170171),#86831) ;
#81124=STYLED_ITEM('',(#170171),#86832) ;
#81125=STYLED_ITEM('',(#170171),#86833) ;
#81126=STYLED_ITEM('',(#170171),#86834) ;
#81127=STYLED_ITEM('',(#170171),#86835) ;
#81128=STYLED_ITEM('',(#170171),#86836) ;
#81129=STYLED_ITEM('',(#170171),#86837) ;
#81130=STYLED_ITEM('',(#170171),#86838) ;
#81131=STYLED_ITEM('',(#170171),#86839) ;
#81132=STYLED_ITEM('',(#170171),#86840) ;
#81133=STYLED_ITEM('',(#170171),#86841) ;
#81134=STYLED_ITEM('',(#170171),#86842) ;
#81135=STYLED_ITEM('',(#170171),#86843) ;
#81136=STYLED_ITEM('',(#170171),#86844) ;
#81137=STYLED_ITEM('',(#170171),#86845) ;
#81138=STYLED_ITEM('',(#170171),#86846) ;
#81139=STYLED_ITEM('',(#170171),#86847) ;
#81140=STYLED_ITEM('',(#170171),#86848) ;
#81141=STYLED_ITEM('',(#170171),#86849) ;
#81142=STYLED_ITEM('',(#170171),#86850) ;
#81143=STYLED_ITEM('',(#170171),#86851) ;
#81144=STYLED_ITEM('',(#170171),#86852) ;
#81145=STYLED_ITEM('',(#170171),#86853) ;
#81146=STYLED_ITEM('',(#170171),#86854) ;
#81147=STYLED_ITEM('',(#170169),#86855) ;
#81148=STYLED_ITEM('',(#170169),#86856) ;
#81149=STYLED_ITEM('',(#170169),#86857) ;
#81150=STYLED_ITEM('',(#170169),#86858) ;
#81151=STYLED_ITEM('',(#170169),#86859) ;
#81152=STYLED_ITEM('',(#170169),#86860) ;
#81153=STYLED_ITEM('',(#170169),#86861) ;
#81154=STYLED_ITEM('',(#170169),#86862) ;
#81155=STYLED_ITEM('',(#170169),#86863) ;
#81156=STYLED_ITEM('',(#170169),#86864) ;
#81157=STYLED_ITEM('',(#170169),#86865) ;
#81158=STYLED_ITEM('',(#170169),#86866) ;
#81159=STYLED_ITEM('',(#170169),#86867) ;
#81160=STYLED_ITEM('',(#170169),#86868) ;
#81161=STYLED_ITEM('',(#170169),#86869) ;
#81162=STYLED_ITEM('',(#170169),#86870) ;
#81163=STYLED_ITEM('',(#170169),#86871) ;
#81164=STYLED_ITEM('',(#170169),#86872) ;
#81165=STYLED_ITEM('',(#170169),#86873) ;
#81166=STYLED_ITEM('',(#170169),#86874) ;
#81167=STYLED_ITEM('',(#170169),#86875) ;
#81168=STYLED_ITEM('',(#170169),#86876) ;
#81169=STYLED_ITEM('',(#170169),#86877) ;
#81170=STYLED_ITEM('',(#170169),#86878) ;
#81171=STYLED_ITEM('',(#170169),#86879) ;
#81172=STYLED_ITEM('',(#170169),#86880) ;
#81173=STYLED_ITEM('',(#170169),#86881) ;
#81174=STYLED_ITEM('',(#170169),#86882) ;
#81175=STYLED_ITEM('',(#170169),#86883) ;
#81176=STYLED_ITEM('',(#170169),#86884) ;
#81177=STYLED_ITEM('',(#170169),#86885) ;
#81178=STYLED_ITEM('',(#170169),#86886) ;
#81179=STYLED_ITEM('',(#170169),#86887) ;
#81180=STYLED_ITEM('',(#170169),#86888) ;
#81181=STYLED_ITEM('',(#170169),#86889) ;
#81182=STYLED_ITEM('',(#170169),#86890) ;
#81183=STYLED_ITEM('',(#170169),#86891) ;
#81184=STYLED_ITEM('',(#170169),#86892) ;
#81185=STYLED_ITEM('',(#170169),#86893) ;
#81186=STYLED_ITEM('',(#170169),#86894) ;
#81187=STYLED_ITEM('',(#170169),#86895) ;
#81188=STYLED_ITEM('',(#170169),#86896) ;
#81189=STYLED_ITEM('',(#170169),#86897) ;
#81190=STYLED_ITEM('',(#170169),#86898) ;
#81191=STYLED_ITEM('',(#170169),#86899) ;
#81192=STYLED_ITEM('',(#170169),#86900) ;
#81193=STYLED_ITEM('',(#170169),#86901) ;
#81194=STYLED_ITEM('',(#170169),#86902) ;
#81195=STYLED_ITEM('',(#170169),#86903) ;
#81196=STYLED_ITEM('',(#170169),#86904) ;
#81197=STYLED_ITEM('',(#170169),#86905) ;
#81198=STYLED_ITEM('',(#170169),#86906) ;
#81199=STYLED_ITEM('',(#170169),#86907) ;
#81200=STYLED_ITEM('',(#170169),#86908) ;
#81201=STYLED_ITEM('',(#170169),#86909) ;
#81202=STYLED_ITEM('',(#170169),#86910) ;
#81203=STYLED_ITEM('',(#170169),#86911) ;
#81204=STYLED_ITEM('',(#170169),#86912) ;
#81205=STYLED_ITEM('',(#170169),#86913) ;
#81206=STYLED_ITEM('',(#170169),#86914) ;
#81207=STYLED_ITEM('',(#170169),#86915) ;
#81208=STYLED_ITEM('',(#170169),#86916) ;
#81209=STYLED_ITEM('',(#170169),#86917) ;
#81210=STYLED_ITEM('',(#170169),#86918) ;
#81211=STYLED_ITEM('',(#170169),#86919) ;
#81212=STYLED_ITEM('',(#170169),#86920) ;
#81213=STYLED_ITEM('',(#170169),#86921) ;
#81214=STYLED_ITEM('',(#170169),#86922) ;
#81215=STYLED_ITEM('',(#170169),#86923) ;
#81216=STYLED_ITEM('',(#170169),#86924) ;
#81217=STYLED_ITEM('',(#170169),#86925) ;
#81218=STYLED_ITEM('',(#170169),#86926) ;
#81219=STYLED_ITEM('',(#170169),#86927) ;
#81220=STYLED_ITEM('',(#170169),#86928) ;
#81221=STYLED_ITEM('',(#170169),#86929) ;
#81222=STYLED_ITEM('',(#170169),#86930) ;
#81223=STYLED_ITEM('',(#170169),#86931) ;
#81224=STYLED_ITEM('',(#170169),#86932) ;
#81225=STYLED_ITEM('',(#170169),#86933) ;
#81226=STYLED_ITEM('',(#170169),#86934) ;
#81227=STYLED_ITEM('',(#170169),#86935) ;
#81228=STYLED_ITEM('',(#170169),#86936) ;
#81229=STYLED_ITEM('',(#170169),#86937) ;
#81230=STYLED_ITEM('',(#170169),#86938) ;
#81231=STYLED_ITEM('',(#170169),#86939) ;
#81232=STYLED_ITEM('',(#170169),#86940) ;
#81233=STYLED_ITEM('',(#170169),#86941) ;
#81234=STYLED_ITEM('',(#170169),#86942) ;
#81235=STYLED_ITEM('',(#170169),#86943) ;
#81236=STYLED_ITEM('',(#170169),#86944) ;
#81237=STYLED_ITEM('',(#170169),#86945) ;
#81238=STYLED_ITEM('',(#170169),#86946) ;
#81239=STYLED_ITEM('',(#170169),#86947) ;
#81240=STYLED_ITEM('',(#170169),#86948) ;
#81241=STYLED_ITEM('',(#170169),#86949) ;
#81242=STYLED_ITEM('',(#170169),#86950) ;
#81243=STYLED_ITEM('',(#170169),#86951) ;
#81244=STYLED_ITEM('',(#170169),#86952) ;
#81245=STYLED_ITEM('',(#170169),#86953) ;
#81246=STYLED_ITEM('',(#170169),#86954) ;
#81247=STYLED_ITEM('',(#170169),#86955) ;
#81248=STYLED_ITEM('',(#170169),#86956) ;
#81249=STYLED_ITEM('',(#170169),#86957) ;
#81250=STYLED_ITEM('',(#170169),#86958) ;
#81251=STYLED_ITEM('',(#170169),#86959) ;
#81252=STYLED_ITEM('',(#170169),#86960) ;
#81253=STYLED_ITEM('',(#170169),#86961) ;
#81254=STYLED_ITEM('',(#170169),#86962) ;
#81255=STYLED_ITEM('',(#170169),#86963) ;
#81256=STYLED_ITEM('',(#170169),#86964) ;
#81257=STYLED_ITEM('',(#170169),#86965) ;
#81258=STYLED_ITEM('',(#170169),#86966) ;
#81259=STYLED_ITEM('',(#170169),#86967) ;
#81260=STYLED_ITEM('',(#170169),#86968) ;
#81261=STYLED_ITEM('',(#170169),#86969) ;
#81262=STYLED_ITEM('',(#170169),#86970) ;
#81263=STYLED_ITEM('',(#170169),#86971) ;
#81264=STYLED_ITEM('',(#170169),#86972) ;
#81265=STYLED_ITEM('',(#170169),#86973) ;
#81266=STYLED_ITEM('',(#170169),#86974) ;
#81267=STYLED_ITEM('',(#170169),#86975) ;
#81268=STYLED_ITEM('',(#170169),#86976) ;
#81269=STYLED_ITEM('',(#170169),#86977) ;
#81270=STYLED_ITEM('',(#170169),#86978) ;
#81271=STYLED_ITEM('',(#170169),#86979) ;
#81272=STYLED_ITEM('',(#170169),#86980) ;
#81273=STYLED_ITEM('',(#170169),#86981) ;
#81274=STYLED_ITEM('',(#170169),#86982) ;
#81275=STYLED_ITEM('',(#170169),#86983) ;
#81276=STYLED_ITEM('',(#170169),#86984) ;
#81277=STYLED_ITEM('',(#170169),#86985) ;
#81278=STYLED_ITEM('',(#170169),#86986) ;
#81279=STYLED_ITEM('',(#170169),#86987) ;
#81280=STYLED_ITEM('',(#170169),#86988) ;
#81281=STYLED_ITEM('',(#170169),#86989) ;
#81282=STYLED_ITEM('',(#170169),#86990) ;
#81283=STYLED_ITEM('',(#170169),#86991) ;
#81284=STYLED_ITEM('',(#170169),#86992) ;
#81285=STYLED_ITEM('',(#170169),#86993) ;
#81286=STYLED_ITEM('',(#170169),#86994) ;
#81287=STYLED_ITEM('',(#170169),#86995) ;
#81288=STYLED_ITEM('',(#170169),#86996) ;
#81289=STYLED_ITEM('',(#170169),#86997) ;
#81290=STYLED_ITEM('',(#170169),#86998) ;
#81291=STYLED_ITEM('',(#170169),#86999) ;
#81292=STYLED_ITEM('',(#170169),#87000) ;
#81293=STYLED_ITEM('',(#170169),#87001) ;
#81294=STYLED_ITEM('',(#170169),#87002) ;
#81295=STYLED_ITEM('',(#170169),#87003) ;
#81296=STYLED_ITEM('',(#170169),#87004) ;
#81297=STYLED_ITEM('',(#170169),#87005) ;
#81298=STYLED_ITEM('',(#170169),#87006) ;
#81299=STYLED_ITEM('',(#170169),#87007) ;
#81300=STYLED_ITEM('',(#170169),#87008) ;
#81301=STYLED_ITEM('',(#170169),#87009) ;
#81302=STYLED_ITEM('',(#170169),#87010) ;
#81303=STYLED_ITEM('',(#170169),#87011) ;
#81304=STYLED_ITEM('',(#170169),#87012) ;
#81305=STYLED_ITEM('',(#170169),#87013) ;
#81306=STYLED_ITEM('',(#170169),#87014) ;
#81307=STYLED_ITEM('',(#170169),#87015) ;
#81308=STYLED_ITEM('',(#170169),#87016) ;
#81309=STYLED_ITEM('',(#170169),#87017) ;
#81310=STYLED_ITEM('',(#170169),#87018) ;
#81311=STYLED_ITEM('',(#170169),#87019) ;
#81312=STYLED_ITEM('',(#170169),#87020) ;
#81313=STYLED_ITEM('',(#170169),#87021) ;
#81314=STYLED_ITEM('',(#170169),#87022) ;
#81315=STYLED_ITEM('',(#170169),#87023) ;
#81316=STYLED_ITEM('',(#170169),#87024) ;
#81317=STYLED_ITEM('',(#170169),#87025) ;
#81318=STYLED_ITEM('',(#170169),#87026) ;
#81319=STYLED_ITEM('',(#170169),#87027) ;
#81320=STYLED_ITEM('',(#170169),#87028) ;
#81321=STYLED_ITEM('',(#170169),#87029) ;
#81322=STYLED_ITEM('',(#170169),#87030) ;
#81323=STYLED_ITEM('',(#170169),#87031) ;
#81324=STYLED_ITEM('',(#170169),#87032) ;
#81325=STYLED_ITEM('',(#170169),#87033) ;
#81326=STYLED_ITEM('',(#170169),#87034) ;
#81327=STYLED_ITEM('',(#170169),#87035) ;
#81328=STYLED_ITEM('',(#170169),#87036) ;
#81329=STYLED_ITEM('',(#170169),#87037) ;
#81330=STYLED_ITEM('',(#170169),#87038) ;
#81331=STYLED_ITEM('',(#170169),#87039) ;
#81332=STYLED_ITEM('',(#170169),#87040) ;
#81333=STYLED_ITEM('',(#170169),#87041) ;
#81334=STYLED_ITEM('',(#170169),#87042) ;
#81335=STYLED_ITEM('',(#170169),#87043) ;
#81336=STYLED_ITEM('',(#170169),#87044) ;
#81337=STYLED_ITEM('',(#170169),#87045) ;
#81338=STYLED_ITEM('',(#170169),#87046) ;
#81339=STYLED_ITEM('',(#170169),#87047) ;
#81340=STYLED_ITEM('',(#170169),#87048) ;
#81341=STYLED_ITEM('',(#170169),#87049) ;
#81342=STYLED_ITEM('',(#170169),#87050) ;
#81343=STYLED_ITEM('',(#170169),#87051) ;
#81344=STYLED_ITEM('',(#170169),#87052) ;
#81345=STYLED_ITEM('',(#170169),#87053) ;
#81346=STYLED_ITEM('',(#170169),#87054) ;
#81347=STYLED_ITEM('',(#170169),#87055) ;
#81348=STYLED_ITEM('',(#170169),#87056) ;
#81349=STYLED_ITEM('',(#170169),#87057) ;
#81350=STYLED_ITEM('',(#170169),#87058) ;
#81351=STYLED_ITEM('',(#170169),#87059) ;
#81352=STYLED_ITEM('',(#170169),#87060) ;
#81353=STYLED_ITEM('',(#170169),#87061) ;
#81354=STYLED_ITEM('',(#170169),#87062) ;
#81355=STYLED_ITEM('',(#170169),#87063) ;
#81356=STYLED_ITEM('',(#170169),#87064) ;
#81357=STYLED_ITEM('',(#170169),#87065) ;
#81358=STYLED_ITEM('',(#170169),#87066) ;
#81359=STYLED_ITEM('',(#170169),#87067) ;
#81360=STYLED_ITEM('',(#170169),#87068) ;
#81361=STYLED_ITEM('',(#170169),#87069) ;
#81362=STYLED_ITEM('',(#170169),#87070) ;
#81363=STYLED_ITEM('',(#170169),#87071) ;
#81364=STYLED_ITEM('',(#170169),#87072) ;
#81365=STYLED_ITEM('',(#170169),#87073) ;
#81366=STYLED_ITEM('',(#170169),#87074) ;
#81367=STYLED_ITEM('',(#170169),#87075) ;
#81368=STYLED_ITEM('',(#170169),#87076) ;
#81369=STYLED_ITEM('',(#170169),#87077) ;
#81370=STYLED_ITEM('',(#170169),#87078) ;
#81371=STYLED_ITEM('',(#170169),#87079) ;
#81372=STYLED_ITEM('',(#170169),#87080) ;
#81373=STYLED_ITEM('',(#170169),#87081) ;
#81374=STYLED_ITEM('',(#170169),#87082) ;
#81375=STYLED_ITEM('',(#170169),#87083) ;
#81376=STYLED_ITEM('',(#170169),#87084) ;
#81377=STYLED_ITEM('',(#170169),#87085) ;
#81378=STYLED_ITEM('',(#170169),#87086) ;
#81379=STYLED_ITEM('',(#170169),#87087) ;
#81380=STYLED_ITEM('',(#170169),#87088) ;
#81381=STYLED_ITEM('',(#170169),#87089) ;
#81382=STYLED_ITEM('',(#170169),#87090) ;
#81383=STYLED_ITEM('',(#170169),#87091) ;
#81384=STYLED_ITEM('',(#170169),#87092) ;
#81385=STYLED_ITEM('',(#170169),#87093) ;
#81386=STYLED_ITEM('',(#170169),#87094) ;
#81387=STYLED_ITEM('',(#170169),#87095) ;
#81388=STYLED_ITEM('',(#170169),#87096) ;
#81389=STYLED_ITEM('',(#170169),#87097) ;
#81390=STYLED_ITEM('',(#170169),#87098) ;
#81391=STYLED_ITEM('',(#170169),#87099) ;
#81392=STYLED_ITEM('',(#170169),#87100) ;
#81393=STYLED_ITEM('',(#170169),#87101) ;
#81394=STYLED_ITEM('',(#170169),#87102) ;
#81395=STYLED_ITEM('',(#170169),#87103) ;
#81396=STYLED_ITEM('',(#170169),#87104) ;
#81397=STYLED_ITEM('',(#170169),#87105) ;
#81398=STYLED_ITEM('',(#170169),#87106) ;
#81399=STYLED_ITEM('',(#170169),#87107) ;
#81400=STYLED_ITEM('',(#170169),#87108) ;
#81401=STYLED_ITEM('',(#170169),#87109) ;
#81402=STYLED_ITEM('',(#170169),#87110) ;
#81403=STYLED_ITEM('',(#170169),#87111) ;
#81404=STYLED_ITEM('',(#170169),#87112) ;
#81405=STYLED_ITEM('',(#170169),#87113) ;
#81406=STYLED_ITEM('',(#170169),#87114) ;
#81407=STYLED_ITEM('',(#170169),#87115) ;
#81408=STYLED_ITEM('',(#170169),#87116) ;
#81409=STYLED_ITEM('',(#170169),#87117) ;
#81410=STYLED_ITEM('',(#170169),#87118) ;
#81411=STYLED_ITEM('',(#170169),#87119) ;
#81412=STYLED_ITEM('',(#170169),#87120) ;
#81413=STYLED_ITEM('',(#170169),#87121) ;
#81414=STYLED_ITEM('',(#170169),#87122) ;
#81415=STYLED_ITEM('',(#170169),#87123) ;
#81416=STYLED_ITEM('',(#170169),#87124) ;
#81417=STYLED_ITEM('',(#170169),#87125) ;
#81418=STYLED_ITEM('',(#170169),#87126) ;
#81419=STYLED_ITEM('',(#170169),#87127) ;
#81420=STYLED_ITEM('',(#170169),#87128) ;
#81421=STYLED_ITEM('',(#170169),#87129) ;
#81422=STYLED_ITEM('',(#170169),#87130) ;
#81423=STYLED_ITEM('',(#170169),#87131) ;
#81424=STYLED_ITEM('',(#170169),#87132) ;
#81425=STYLED_ITEM('',(#170169),#87133) ;
#81426=STYLED_ITEM('',(#170169),#87134) ;
#81427=STYLED_ITEM('',(#170169),#87135) ;
#81428=STYLED_ITEM('',(#170169),#87136) ;
#81429=STYLED_ITEM('',(#170169),#87137) ;
#81430=STYLED_ITEM('',(#170169),#87138) ;
#81431=STYLED_ITEM('',(#170169),#87139) ;
#81432=STYLED_ITEM('',(#170169),#87140) ;
#81433=STYLED_ITEM('',(#170169),#87141) ;
#81434=STYLED_ITEM('',(#170169),#87142) ;
#81435=STYLED_ITEM('',(#170169),#87143) ;
#81436=STYLED_ITEM('',(#170169),#87144) ;
#81437=STYLED_ITEM('',(#170169),#87145) ;
#81438=STYLED_ITEM('',(#170169),#87146) ;
#81439=STYLED_ITEM('',(#170169),#87147) ;
#81440=STYLED_ITEM('',(#170169),#87148) ;
#81441=STYLED_ITEM('',(#170169),#87149) ;
#81442=STYLED_ITEM('',(#170169),#87150) ;
#81443=STYLED_ITEM('',(#170169),#87151) ;
#81444=STYLED_ITEM('',(#170169),#87152) ;
#81445=STYLED_ITEM('',(#170169),#87153) ;
#81446=STYLED_ITEM('',(#170169),#87154) ;
#81447=STYLED_ITEM('',(#170169),#87155) ;
#81448=STYLED_ITEM('',(#170169),#87156) ;
#81449=STYLED_ITEM('',(#170169),#87157) ;
#81450=STYLED_ITEM('',(#170169),#87158) ;
#81451=STYLED_ITEM('',(#170169),#87159) ;
#81452=STYLED_ITEM('',(#170169),#87160) ;
#81453=STYLED_ITEM('',(#170169),#87161) ;
#81454=STYLED_ITEM('',(#170169),#87162) ;
#81455=STYLED_ITEM('',(#170169),#87163) ;
#81456=STYLED_ITEM('',(#170169),#87164) ;
#81457=STYLED_ITEM('',(#170169),#87165) ;
#81458=STYLED_ITEM('',(#170169),#87166) ;
#81459=STYLED_ITEM('',(#170169),#87167) ;
#81460=STYLED_ITEM('',(#170169),#87168) ;
#81461=STYLED_ITEM('',(#170169),#87169) ;
#81462=STYLED_ITEM('',(#170169),#87170) ;
#81463=STYLED_ITEM('',(#170169),#87171) ;
#81464=STYLED_ITEM('',(#170169),#87172) ;
#81465=STYLED_ITEM('',(#170169),#87173) ;
#81466=STYLED_ITEM('',(#170169),#87174) ;
#81467=STYLED_ITEM('',(#170169),#87175) ;
#81468=STYLED_ITEM('',(#170169),#87176) ;
#81469=STYLED_ITEM('',(#170169),#87177) ;
#81470=STYLED_ITEM('',(#170169),#87178) ;
#81471=STYLED_ITEM('',(#170169),#87179) ;
#81472=STYLED_ITEM('',(#170169),#87180) ;
#81473=STYLED_ITEM('',(#170169),#87181) ;
#81474=STYLED_ITEM('',(#170169),#87182) ;
#81475=STYLED_ITEM('',(#170169),#87183) ;
#81476=STYLED_ITEM('',(#170169),#87184) ;
#81477=STYLED_ITEM('',(#170169),#87185) ;
#81478=STYLED_ITEM('',(#170169),#87186) ;
#81479=STYLED_ITEM('',(#170169),#87187) ;
#81480=STYLED_ITEM('',(#170169),#87188) ;
#81481=STYLED_ITEM('',(#170169),#87189) ;
#81482=STYLED_ITEM('',(#170169),#87190) ;
#81483=STYLED_ITEM('',(#170169),#87191) ;
#81484=STYLED_ITEM('',(#170169),#87192) ;
#81485=STYLED_ITEM('',(#170169),#87193) ;
#81486=STYLED_ITEM('',(#170169),#87194) ;
#81487=STYLED_ITEM('',(#170169),#87195) ;
#81488=STYLED_ITEM('',(#170169),#87196) ;
#81489=STYLED_ITEM('',(#170169),#87197) ;
#81490=STYLED_ITEM('',(#170169),#87198) ;
#81491=STYLED_ITEM('',(#170169),#87199) ;
#81492=STYLED_ITEM('',(#170169),#87200) ;
#81493=STYLED_ITEM('',(#170169),#87201) ;
#81494=STYLED_ITEM('',(#170169),#87202) ;
#81495=STYLED_ITEM('',(#170169),#87203) ;
#81496=STYLED_ITEM('',(#170169),#87204) ;
#81497=STYLED_ITEM('',(#170169),#87205) ;
#81498=STYLED_ITEM('',(#170169),#87206) ;
#81499=STYLED_ITEM('',(#170169),#87207) ;
#81500=STYLED_ITEM('',(#170169),#87208) ;
#81501=STYLED_ITEM('',(#170169),#87209) ;
#81502=STYLED_ITEM('',(#170169),#87210) ;
#81503=STYLED_ITEM('',(#170169),#87211) ;
#81504=STYLED_ITEM('',(#170169),#87212) ;
#81505=STYLED_ITEM('',(#170169),#87213) ;
#81506=STYLED_ITEM('',(#170169),#87214) ;
#81507=STYLED_ITEM('',(#170169),#87215) ;
#81508=STYLED_ITEM('',(#170169),#87216) ;
#81509=STYLED_ITEM('',(#170169),#87217) ;
#81510=STYLED_ITEM('',(#170169),#87218) ;
#81511=STYLED_ITEM('',(#170169),#87219) ;
#81512=STYLED_ITEM('',(#170169),#87220) ;
#81513=STYLED_ITEM('',(#170169),#87221) ;
#81514=STYLED_ITEM('',(#170169),#87222) ;
#81515=STYLED_ITEM('',(#170169),#87223) ;
#81516=STYLED_ITEM('',(#170169),#87224) ;
#81517=STYLED_ITEM('',(#170169),#87225) ;
#81518=STYLED_ITEM('',(#170169),#87226) ;
#81519=STYLED_ITEM('',(#170169),#87227) ;
#81520=STYLED_ITEM('',(#170169),#87228) ;
#81521=STYLED_ITEM('',(#170169),#87229) ;
#81522=STYLED_ITEM('',(#170169),#87230) ;
#81523=STYLED_ITEM('',(#170169),#87231) ;
#81524=STYLED_ITEM('',(#170169),#87232) ;
#81525=STYLED_ITEM('',(#170169),#87233) ;
#81526=STYLED_ITEM('',(#170169),#87234) ;
#81527=STYLED_ITEM('',(#170169),#87235) ;
#81528=STYLED_ITEM('',(#170169),#87236) ;
#81529=STYLED_ITEM('',(#170169),#87237) ;
#81530=STYLED_ITEM('',(#170169),#87238) ;
#81531=STYLED_ITEM('',(#170169),#87239) ;
#81532=STYLED_ITEM('',(#170169),#87240) ;
#81533=STYLED_ITEM('',(#170169),#87241) ;
#81534=STYLED_ITEM('',(#170169),#87242) ;
#81535=STYLED_ITEM('',(#170169),#87243) ;
#81536=STYLED_ITEM('',(#170169),#87244) ;
#81537=STYLED_ITEM('',(#170169),#87245) ;
#81538=STYLED_ITEM('',(#170169),#87246) ;
#81539=STYLED_ITEM('',(#170169),#87247) ;
#81540=STYLED_ITEM('',(#170169),#87248) ;
#81541=STYLED_ITEM('',(#170169),#87249) ;
#81542=STYLED_ITEM('',(#170169),#87250) ;
#81543=STYLED_ITEM('',(#170169),#87251) ;
#81544=STYLED_ITEM('',(#170169),#87252) ;
#81545=STYLED_ITEM('',(#170169),#87253) ;
#81546=STYLED_ITEM('',(#170169),#87254) ;
#81547=STYLED_ITEM('',(#170169),#87255) ;
#81548=STYLED_ITEM('',(#170169),#87256) ;
#81549=STYLED_ITEM('',(#170169),#87257) ;
#81550=STYLED_ITEM('',(#170169),#87258) ;
#81551=STYLED_ITEM('',(#170169),#87259) ;
#81552=STYLED_ITEM('',(#170169),#87260) ;
#81553=STYLED_ITEM('',(#170169),#87261) ;
#81554=STYLED_ITEM('',(#170169),#87262) ;
#81555=STYLED_ITEM('',(#170169),#87263) ;
#81556=STYLED_ITEM('',(#170169),#87264) ;
#81557=STYLED_ITEM('',(#170169),#87265) ;
#81558=STYLED_ITEM('',(#170169),#87266) ;
#81559=STYLED_ITEM('',(#170169),#87267) ;
#81560=STYLED_ITEM('',(#170169),#87268) ;
#81561=STYLED_ITEM('',(#170169),#87269) ;
#81562=STYLED_ITEM('',(#170169),#87270) ;
#81563=STYLED_ITEM('',(#170169),#87271) ;
#81564=STYLED_ITEM('',(#170169),#87272) ;
#81565=STYLED_ITEM('',(#170169),#87273) ;
#81566=STYLED_ITEM('',(#170169),#87274) ;
#81567=STYLED_ITEM('',(#170169),#87275) ;
#81568=STYLED_ITEM('',(#170169),#87276) ;
#81569=STYLED_ITEM('',(#170169),#87277) ;
#81570=STYLED_ITEM('',(#170169),#87278) ;
#81571=STYLED_ITEM('',(#170169),#87279) ;
#81572=STYLED_ITEM('',(#170169),#87280) ;
#81573=STYLED_ITEM('',(#170169),#87281) ;
#81574=STYLED_ITEM('',(#170169),#87282) ;
#81575=STYLED_ITEM('',(#170169),#87283) ;
#81576=STYLED_ITEM('',(#170169),#87284) ;
#81577=STYLED_ITEM('',(#170169),#87285) ;
#81578=STYLED_ITEM('',(#170169),#87286) ;
#81579=STYLED_ITEM('',(#170169),#87287) ;
#81580=STYLED_ITEM('',(#170169),#87288) ;
#81581=STYLED_ITEM('',(#170169),#87289) ;
#81582=STYLED_ITEM('',(#170169),#87290) ;
#81583=STYLED_ITEM('',(#170169),#87291) ;
#81584=STYLED_ITEM('',(#170169),#87292) ;
#81585=STYLED_ITEM('',(#170169),#87293) ;
#81586=STYLED_ITEM('',(#170169),#87294) ;
#81587=STYLED_ITEM('',(#170169),#87295) ;
#81588=STYLED_ITEM('',(#170169),#87296) ;
#81589=STYLED_ITEM('',(#170169),#87297) ;
#81590=STYLED_ITEM('',(#170169),#87298) ;
#81591=STYLED_ITEM('',(#170169),#87299) ;
#81592=STYLED_ITEM('',(#170169),#87300) ;
#81593=STYLED_ITEM('',(#170169),#87301) ;
#81594=STYLED_ITEM('',(#170169),#87302) ;
#81595=STYLED_ITEM('',(#170169),#87303) ;
#81596=STYLED_ITEM('',(#170169),#87304) ;
#81597=STYLED_ITEM('',(#170169),#87305) ;
#81598=STYLED_ITEM('',(#170169),#87306) ;
#81599=STYLED_ITEM('',(#170169),#87307) ;
#81600=STYLED_ITEM('',(#170169),#87308) ;
#81601=STYLED_ITEM('',(#170169),#87309) ;
#81602=STYLED_ITEM('',(#170169),#87310) ;
#81603=STYLED_ITEM('',(#170169),#87311) ;
#81604=STYLED_ITEM('',(#170169),#87312) ;
#81605=STYLED_ITEM('',(#170169),#87313) ;
#81606=STYLED_ITEM('',(#170169),#87314) ;
#81607=STYLED_ITEM('',(#170169),#87315) ;
#81608=STYLED_ITEM('',(#170169),#87316) ;
#81609=STYLED_ITEM('',(#170169),#87317) ;
#81610=STYLED_ITEM('',(#170169),#87318) ;
#81611=STYLED_ITEM('',(#170169),#87319) ;
#81612=STYLED_ITEM('',(#170169),#87320) ;
#81613=STYLED_ITEM('',(#170169),#87321) ;
#81614=STYLED_ITEM('',(#170169),#87322) ;
#81615=STYLED_ITEM('',(#170169),#87323) ;
#81616=STYLED_ITEM('',(#170169),#87324) ;
#81617=STYLED_ITEM('',(#170169),#87325) ;
#81618=STYLED_ITEM('',(#170169),#87326) ;
#81619=STYLED_ITEM('',(#170169),#87327) ;
#81620=STYLED_ITEM('',(#170169),#87328) ;
#81621=STYLED_ITEM('',(#170169),#87329) ;
#81622=STYLED_ITEM('',(#170169),#87330) ;
#81623=STYLED_ITEM('',(#170169),#87331) ;
#81624=STYLED_ITEM('',(#170169),#87332) ;
#81625=STYLED_ITEM('',(#170169),#87333) ;
#81626=STYLED_ITEM('',(#170169),#87334) ;
#81627=STYLED_ITEM('',(#170169),#87335) ;
#81628=STYLED_ITEM('',(#170169),#87336) ;
#81629=STYLED_ITEM('',(#170169),#87337) ;
#81630=STYLED_ITEM('',(#170169),#87338) ;
#81631=STYLED_ITEM('',(#170169),#87339) ;
#81632=STYLED_ITEM('',(#170169),#87340) ;
#81633=STYLED_ITEM('',(#170169),#87341) ;
#81634=STYLED_ITEM('',(#170169),#87342) ;
#81635=STYLED_ITEM('',(#170169),#87343) ;
#81636=STYLED_ITEM('',(#170169),#87344) ;
#81637=STYLED_ITEM('',(#170169),#87345) ;
#81638=STYLED_ITEM('',(#170169),#87346) ;
#81639=STYLED_ITEM('',(#170169),#87347) ;
#81640=STYLED_ITEM('',(#170169),#87348) ;
#81641=STYLED_ITEM('',(#170169),#87349) ;
#81642=STYLED_ITEM('',(#170169),#87350) ;
#81643=STYLED_ITEM('',(#170169),#87351) ;
#81644=STYLED_ITEM('',(#170169),#87352) ;
#81645=STYLED_ITEM('',(#170169),#87353) ;
#81646=STYLED_ITEM('',(#170169),#87354) ;
#81647=STYLED_ITEM('',(#170169),#87355) ;
#81648=STYLED_ITEM('',(#170169),#87356) ;
#81649=STYLED_ITEM('',(#170169),#87357) ;
#81650=STYLED_ITEM('',(#170169),#87358) ;
#81651=STYLED_ITEM('',(#170169),#87359) ;
#81652=STYLED_ITEM('',(#170169),#87360) ;
#81653=STYLED_ITEM('',(#170169),#87361) ;
#81654=STYLED_ITEM('',(#170169),#87362) ;
#81655=STYLED_ITEM('',(#170169),#87363) ;
#81656=STYLED_ITEM('',(#170169),#87364) ;
#81657=STYLED_ITEM('',(#170169),#87365) ;
#81658=STYLED_ITEM('',(#170169),#87366) ;
#81659=STYLED_ITEM('',(#170169),#87367) ;
#81660=STYLED_ITEM('',(#170169),#87368) ;
#81661=STYLED_ITEM('',(#170169),#87369) ;
#81662=STYLED_ITEM('',(#170169),#87370) ;
#81663=STYLED_ITEM('',(#170169),#87371) ;
#81664=STYLED_ITEM('',(#170169),#87372) ;
#81665=STYLED_ITEM('',(#170169),#87373) ;
#81666=STYLED_ITEM('',(#170169),#87374) ;
#81667=STYLED_ITEM('',(#170169),#87375) ;
#81668=STYLED_ITEM('',(#170169),#87376) ;
#81669=STYLED_ITEM('',(#170169),#87377) ;
#81670=STYLED_ITEM('',(#170169),#87378) ;
#81671=STYLED_ITEM('',(#170169),#87379) ;
#81672=STYLED_ITEM('',(#170169),#87380) ;
#81673=STYLED_ITEM('',(#170169),#87381) ;
#81674=STYLED_ITEM('',(#170169),#87382) ;
#81675=STYLED_ITEM('',(#170169),#87383) ;
#81676=STYLED_ITEM('',(#170169),#87384) ;
#81677=STYLED_ITEM('',(#170169),#87385) ;
#81678=STYLED_ITEM('',(#170169),#87386) ;
#81679=STYLED_ITEM('',(#170169),#87387) ;
#81680=STYLED_ITEM('',(#170169),#87388) ;
#81681=STYLED_ITEM('',(#170169),#87389) ;
#81682=STYLED_ITEM('',(#170169),#87390) ;
#81683=STYLED_ITEM('',(#170169),#87391) ;
#81684=STYLED_ITEM('',(#170169),#87392) ;
#81685=STYLED_ITEM('',(#170169),#87393) ;
#81686=STYLED_ITEM('',(#170169),#87394) ;
#81687=STYLED_ITEM('',(#170169),#87395) ;
#81688=STYLED_ITEM('',(#170169),#87396) ;
#81689=STYLED_ITEM('',(#170169),#87397) ;
#81690=STYLED_ITEM('',(#170169),#87398) ;
#81691=STYLED_ITEM('',(#170169),#87399) ;
#81692=STYLED_ITEM('',(#170169),#87400) ;
#81693=STYLED_ITEM('',(#170169),#87401) ;
#81694=STYLED_ITEM('',(#170169),#87402) ;
#81695=STYLED_ITEM('',(#170169),#87403) ;
#81696=STYLED_ITEM('',(#170169),#87404) ;
#81697=STYLED_ITEM('',(#170169),#87405) ;
#81698=STYLED_ITEM('',(#170169),#87406) ;
#81699=STYLED_ITEM('',(#170169),#87407) ;
#81700=STYLED_ITEM('',(#170169),#87408) ;
#81701=STYLED_ITEM('',(#170169),#87409) ;
#81702=STYLED_ITEM('',(#170169),#87410) ;
#81703=STYLED_ITEM('',(#170169),#87411) ;
#81704=STYLED_ITEM('',(#170169),#87412) ;
#81705=STYLED_ITEM('',(#170169),#87413) ;
#81706=STYLED_ITEM('',(#170169),#87414) ;
#81707=STYLED_ITEM('',(#170169),#87415) ;
#81708=STYLED_ITEM('',(#170169),#87416) ;
#81709=STYLED_ITEM('',(#170169),#87417) ;
#81710=STYLED_ITEM('',(#170169),#87418) ;
#81711=STYLED_ITEM('',(#170169),#87419) ;
#81712=STYLED_ITEM('',(#170169),#87420) ;
#81713=STYLED_ITEM('',(#170169),#87421) ;
#81714=STYLED_ITEM('',(#170169),#87422) ;
#81715=STYLED_ITEM('',(#170169),#87423) ;
#81716=STYLED_ITEM('',(#170169),#87424) ;
#81717=STYLED_ITEM('',(#170169),#87425) ;
#81718=STYLED_ITEM('',(#170169),#87426) ;
#81719=STYLED_ITEM('',(#170169),#87427) ;
#81720=STYLED_ITEM('',(#170169),#87428) ;
#81721=STYLED_ITEM('',(#170169),#87429) ;
#81722=STYLED_ITEM('',(#170169),#87430) ;
#81723=STYLED_ITEM('',(#170169),#87431) ;
#81724=STYLED_ITEM('',(#170169),#87432) ;
#81725=STYLED_ITEM('',(#170169),#87433) ;
#81726=STYLED_ITEM('',(#170169),#87434) ;
#81727=STYLED_ITEM('',(#170169),#87435) ;
#81728=STYLED_ITEM('',(#170169),#87436) ;
#81729=STYLED_ITEM('',(#170169),#87437) ;
#81730=STYLED_ITEM('',(#170169),#87438) ;
#81731=STYLED_ITEM('',(#170169),#87439) ;
#81732=STYLED_ITEM('',(#170169),#87440) ;
#81733=STYLED_ITEM('',(#170169),#87441) ;
#81734=STYLED_ITEM('',(#170169),#87442) ;
#81735=STYLED_ITEM('',(#170169),#87443) ;
#81736=STYLED_ITEM('',(#170169),#87444) ;
#81737=STYLED_ITEM('',(#170169),#87445) ;
#81738=STYLED_ITEM('',(#170169),#87446) ;
#81739=STYLED_ITEM('',(#170169),#87447) ;
#81740=STYLED_ITEM('',(#170169),#87448) ;
#81741=STYLED_ITEM('',(#170169),#87449) ;
#81742=STYLED_ITEM('',(#170169),#87450) ;
#81743=STYLED_ITEM('',(#170169),#87451) ;
#81744=STYLED_ITEM('',(#170169),#87452) ;
#81745=STYLED_ITEM('',(#170169),#87453) ;
#81746=STYLED_ITEM('',(#170169),#87454) ;
#81747=STYLED_ITEM('',(#170169),#87455) ;
#81748=STYLED_ITEM('',(#170169),#87456) ;
#81749=STYLED_ITEM('',(#170169),#87457) ;
#81750=STYLED_ITEM('',(#170169),#87458) ;
#81751=STYLED_ITEM('',(#170169),#87459) ;
#81752=STYLED_ITEM('',(#170169),#87460) ;
#81753=STYLED_ITEM('',(#170169),#87461) ;
#81754=STYLED_ITEM('',(#170169),#87462) ;
#81755=STYLED_ITEM('',(#170169),#87463) ;
#81756=STYLED_ITEM('',(#170169),#87464) ;
#81757=STYLED_ITEM('',(#170169),#87465) ;
#81758=STYLED_ITEM('',(#170169),#87466) ;
#81759=STYLED_ITEM('',(#170169),#87467) ;
#81760=STYLED_ITEM('',(#170169),#87468) ;
#81761=STYLED_ITEM('',(#170169),#87469) ;
#81762=STYLED_ITEM('',(#170169),#87470) ;
#81763=STYLED_ITEM('',(#170169),#87471) ;
#81764=STYLED_ITEM('',(#170169),#87472) ;
#81765=STYLED_ITEM('',(#170169),#87473) ;
#81766=STYLED_ITEM('',(#170169),#87474) ;
#81767=STYLED_ITEM('',(#170169),#87475) ;
#81768=STYLED_ITEM('',(#170169),#87476) ;
#81769=STYLED_ITEM('',(#170169),#87477) ;
#81770=STYLED_ITEM('',(#170169),#87478) ;
#81771=STYLED_ITEM('',(#170169),#87479) ;
#81772=STYLED_ITEM('',(#170169),#87480) ;
#81773=STYLED_ITEM('',(#170169),#87481) ;
#81774=STYLED_ITEM('',(#170169),#87482) ;
#81775=STYLED_ITEM('',(#170169),#87483) ;
#81776=STYLED_ITEM('',(#170169),#87484) ;
#81777=STYLED_ITEM('',(#170169),#87485) ;
#81778=STYLED_ITEM('',(#170169),#87486) ;
#81779=STYLED_ITEM('',(#170169),#87487) ;
#81780=STYLED_ITEM('',(#170169),#87488) ;
#81781=STYLED_ITEM('',(#170169),#87489) ;
#81782=STYLED_ITEM('',(#170169),#87490) ;
#81783=STYLED_ITEM('',(#170169),#87491) ;
#81784=STYLED_ITEM('',(#170169),#87492) ;
#81785=STYLED_ITEM('',(#170169),#87493) ;
#81786=STYLED_ITEM('',(#170169),#87494) ;
#81787=STYLED_ITEM('',(#170169),#87495) ;
#81788=STYLED_ITEM('',(#170169),#87496) ;
#81789=STYLED_ITEM('',(#170169),#87497) ;
#81790=STYLED_ITEM('',(#170169),#87498) ;
#81791=STYLED_ITEM('',(#170169),#87499) ;
#81792=STYLED_ITEM('',(#170169),#87500) ;
#81793=STYLED_ITEM('',(#170169),#87501) ;
#81794=STYLED_ITEM('',(#170169),#87502) ;
#81795=STYLED_ITEM('',(#170169),#87503) ;
#81796=STYLED_ITEM('',(#170169),#87504) ;
#81797=STYLED_ITEM('',(#170169),#87505) ;
#81798=STYLED_ITEM('',(#170169),#87506) ;
#81799=STYLED_ITEM('',(#170169),#87507) ;
#81800=STYLED_ITEM('',(#170169),#87508) ;
#81801=STYLED_ITEM('',(#170169),#87509) ;
#81802=STYLED_ITEM('',(#170169),#87510) ;
#81803=STYLED_ITEM('',(#170169),#87511) ;
#81804=STYLED_ITEM('',(#170169),#87512) ;
#81805=STYLED_ITEM('',(#170169),#87513) ;
#81806=STYLED_ITEM('',(#170169),#87514) ;
#81807=STYLED_ITEM('',(#170169),#87515) ;
#81808=STYLED_ITEM('',(#170169),#87516) ;
#81809=STYLED_ITEM('',(#170169),#87517) ;
#81810=STYLED_ITEM('',(#170169),#87518) ;
#81811=STYLED_ITEM('',(#170169),#87519) ;
#81812=STYLED_ITEM('',(#170169),#87520) ;
#81813=STYLED_ITEM('',(#170169),#87521) ;
#81814=STYLED_ITEM('',(#170169),#87522) ;
#81815=STYLED_ITEM('',(#170169),#87523) ;
#81816=STYLED_ITEM('',(#170169),#87524) ;
#81817=STYLED_ITEM('',(#170169),#87525) ;
#81818=STYLED_ITEM('',(#170169),#87526) ;
#81819=STYLED_ITEM('',(#170169),#87527) ;
#81820=STYLED_ITEM('',(#170169),#87528) ;
#81821=STYLED_ITEM('',(#170169),#87529) ;
#81822=STYLED_ITEM('',(#170169),#87530) ;
#81823=STYLED_ITEM('',(#170169),#87531) ;
#81824=STYLED_ITEM('',(#170169),#87532) ;
#81825=STYLED_ITEM('',(#170169),#87533) ;
#81826=STYLED_ITEM('',(#170169),#87534) ;
#81827=STYLED_ITEM('',(#170169),#87535) ;
#81828=STYLED_ITEM('',(#170169),#87536) ;
#81829=STYLED_ITEM('',(#170169),#87537) ;
#81830=STYLED_ITEM('',(#170169),#87538) ;
#81831=STYLED_ITEM('',(#170169),#87539) ;
#81832=STYLED_ITEM('',(#170169),#87540) ;
#81833=STYLED_ITEM('',(#170169),#87541) ;
#81834=STYLED_ITEM('',(#170169),#87542) ;
#81835=STYLED_ITEM('',(#170169),#87543) ;
#81836=STYLED_ITEM('',(#170169),#87544) ;
#81837=STYLED_ITEM('',(#170169),#87545) ;
#81838=STYLED_ITEM('',(#170169),#87546) ;
#81839=STYLED_ITEM('',(#170169),#87547) ;
#81840=STYLED_ITEM('',(#170169),#87548) ;
#81841=STYLED_ITEM('',(#170169),#87549) ;
#81842=STYLED_ITEM('',(#170169),#87550) ;
#81843=STYLED_ITEM('',(#170169),#87551) ;
#81844=STYLED_ITEM('',(#170169),#87552) ;
#81845=STYLED_ITEM('',(#170169),#87553) ;
#81846=STYLED_ITEM('',(#170169),#87554) ;
#81847=STYLED_ITEM('',(#170169),#87555) ;
#81848=STYLED_ITEM('',(#170169),#87556) ;
#81849=STYLED_ITEM('',(#170169),#87557) ;
#81850=STYLED_ITEM('',(#170169),#87558) ;
#81851=STYLED_ITEM('',(#170169),#87559) ;
#81852=STYLED_ITEM('',(#170169),#87560) ;
#81853=STYLED_ITEM('',(#170169),#87561) ;
#81854=STYLED_ITEM('',(#170169),#87562) ;
#81855=STYLED_ITEM('',(#170169),#87563) ;
#81856=STYLED_ITEM('',(#170169),#87564) ;
#81857=STYLED_ITEM('',(#170169),#87565) ;
#81858=STYLED_ITEM('',(#170169),#87566) ;
#81859=STYLED_ITEM('',(#170169),#87567) ;
#81860=STYLED_ITEM('',(#170169),#87568) ;
#81861=STYLED_ITEM('',(#170169),#87569) ;
#81862=STYLED_ITEM('',(#170169),#87570) ;
#81863=STYLED_ITEM('',(#170169),#87571) ;
#81864=STYLED_ITEM('',(#170169),#87572) ;
#81865=STYLED_ITEM('',(#170169),#87573) ;
#81866=STYLED_ITEM('',(#170169),#87574) ;
#81867=STYLED_ITEM('',(#170169),#87575) ;
#81868=STYLED_ITEM('',(#170169),#87576) ;
#81869=STYLED_ITEM('',(#170169),#87577) ;
#81870=STYLED_ITEM('',(#170169),#87578) ;
#81871=STYLED_ITEM('',(#170169),#87579) ;
#81872=STYLED_ITEM('',(#170169),#87580) ;
#81873=STYLED_ITEM('',(#170169),#87581) ;
#81874=STYLED_ITEM('',(#170169),#87582) ;
#81875=STYLED_ITEM('',(#170169),#87583) ;
#81876=STYLED_ITEM('',(#170169),#87584) ;
#81877=STYLED_ITEM('',(#170169),#87585) ;
#81878=STYLED_ITEM('',(#170169),#87586) ;
#81879=STYLED_ITEM('',(#170169),#87587) ;
#81880=STYLED_ITEM('',(#170169),#87588) ;
#81881=STYLED_ITEM('',(#170169),#87589) ;
#81882=STYLED_ITEM('',(#170169),#87590) ;
#81883=STYLED_ITEM('',(#170169),#87591) ;
#81884=STYLED_ITEM('',(#170169),#87592) ;
#81885=STYLED_ITEM('',(#170169),#87593) ;
#81886=STYLED_ITEM('',(#170169),#87594) ;
#81887=STYLED_ITEM('',(#170169),#87595) ;
#81888=STYLED_ITEM('',(#170169),#87596) ;
#81889=STYLED_ITEM('',(#170169),#87597) ;
#81890=STYLED_ITEM('',(#170169),#87598) ;
#81891=STYLED_ITEM('',(#170169),#87599) ;
#81892=STYLED_ITEM('',(#170169),#87600) ;
#81893=STYLED_ITEM('',(#170169),#87601) ;
#81894=STYLED_ITEM('',(#170169),#87602) ;
#81895=STYLED_ITEM('',(#170169),#87603) ;
#81896=STYLED_ITEM('',(#170169),#87604) ;
#81897=STYLED_ITEM('',(#170169),#87605) ;
#81898=STYLED_ITEM('',(#170169),#87606) ;
#81899=STYLED_ITEM('',(#170169),#87607) ;
#81900=STYLED_ITEM('',(#170169),#87608) ;
#81901=STYLED_ITEM('',(#170169),#87609) ;
#81902=STYLED_ITEM('',(#170169),#87610) ;
#81903=STYLED_ITEM('',(#170169),#87611) ;
#81904=STYLED_ITEM('',(#170169),#87612) ;
#81905=STYLED_ITEM('',(#170169),#87613) ;
#81906=STYLED_ITEM('',(#170169),#87614) ;
#81907=STYLED_ITEM('',(#170169),#87615) ;
#81908=STYLED_ITEM('',(#170169),#87616) ;
#81909=STYLED_ITEM('',(#170169),#87617) ;
#81910=STYLED_ITEM('',(#170169),#87618) ;
#81911=STYLED_ITEM('',(#170169),#87619) ;
#81912=STYLED_ITEM('',(#170169),#87620) ;
#81913=STYLED_ITEM('',(#170169),#87621) ;
#81914=STYLED_ITEM('',(#170169),#87622) ;
#81915=STYLED_ITEM('',(#170169),#87623) ;
#81916=STYLED_ITEM('',(#170169),#87624) ;
#81917=STYLED_ITEM('',(#170169),#87625) ;
#81918=STYLED_ITEM('',(#170169),#87626) ;
#81919=STYLED_ITEM('',(#170169),#87627) ;
#81920=STYLED_ITEM('',(#170169),#87628) ;
#81921=STYLED_ITEM('',(#170169),#87629) ;
#81922=STYLED_ITEM('',(#170169),#87630) ;
#81923=STYLED_ITEM('',(#170169),#87631) ;
#81924=STYLED_ITEM('',(#170169),#87632) ;
#81925=STYLED_ITEM('',(#170169),#87633) ;
#81926=STYLED_ITEM('',(#170169),#87634) ;
#81927=STYLED_ITEM('',(#170169),#87635) ;
#81928=STYLED_ITEM('',(#170169),#87636) ;
#81929=STYLED_ITEM('',(#170169),#87637) ;
#81930=STYLED_ITEM('',(#170169),#87638) ;
#81931=STYLED_ITEM('',(#170169),#87639) ;
#81932=STYLED_ITEM('',(#170169),#87640) ;
#81933=STYLED_ITEM('',(#170169),#87641) ;
#81934=STYLED_ITEM('',(#170169),#87642) ;
#81935=STYLED_ITEM('',(#170169),#87643) ;
#81936=STYLED_ITEM('',(#170169),#87644) ;
#81937=STYLED_ITEM('',(#170169),#87645) ;
#81938=STYLED_ITEM('',(#170169),#87646) ;
#81939=STYLED_ITEM('',(#170169),#87647) ;
#81940=STYLED_ITEM('',(#170169),#87648) ;
#81941=STYLED_ITEM('',(#170169),#87649) ;
#81942=STYLED_ITEM('',(#170169),#87650) ;
#81943=STYLED_ITEM('',(#170169),#87651) ;
#81944=STYLED_ITEM('',(#170169),#87652) ;
#81945=STYLED_ITEM('',(#170169),#87653) ;
#81946=STYLED_ITEM('',(#170169),#87654) ;
#81947=STYLED_ITEM('',(#170169),#87655) ;
#81948=STYLED_ITEM('',(#170169),#87656) ;
#81949=STYLED_ITEM('',(#170169),#87657) ;
#81950=STYLED_ITEM('',(#170169),#87658) ;
#81951=STYLED_ITEM('',(#170169),#87659) ;
#81952=STYLED_ITEM('',(#170169),#87660) ;
#81953=STYLED_ITEM('',(#170169),#87661) ;
#81954=STYLED_ITEM('',(#170169),#87662) ;
#81955=STYLED_ITEM('',(#170169),#87663) ;
#81956=STYLED_ITEM('',(#170169),#87664) ;
#81957=STYLED_ITEM('',(#170169),#87665) ;
#81958=STYLED_ITEM('',(#170169),#87666) ;
#81959=STYLED_ITEM('',(#170169),#87667) ;
#81960=STYLED_ITEM('',(#170169),#87668) ;
#81961=STYLED_ITEM('',(#170169),#87669) ;
#81962=STYLED_ITEM('',(#170169),#87670) ;
#81963=STYLED_ITEM('',(#170169),#87671) ;
#81964=STYLED_ITEM('',(#170169),#87672) ;
#81965=STYLED_ITEM('',(#170169),#87673) ;
#81966=STYLED_ITEM('',(#170169),#87674) ;
#81967=STYLED_ITEM('',(#170169),#87675) ;
#81968=STYLED_ITEM('',(#170169),#87676) ;
#81969=STYLED_ITEM('',(#170169),#87677) ;
#81970=STYLED_ITEM('',(#170169),#87678) ;
#81971=STYLED_ITEM('',(#170169),#87679) ;
#81972=STYLED_ITEM('',(#170169),#87680) ;
#81973=STYLED_ITEM('',(#170169),#87681) ;
#81974=STYLED_ITEM('',(#170169),#87682) ;
#81975=STYLED_ITEM('',(#170169),#87683) ;
#81976=STYLED_ITEM('',(#170169),#87684) ;
#81977=STYLED_ITEM('',(#170169),#87685) ;
#81978=STYLED_ITEM('',(#170169),#87686) ;
#81979=STYLED_ITEM('',(#170169),#87687) ;
#81980=STYLED_ITEM('',(#170169),#87688) ;
#81981=STYLED_ITEM('',(#170169),#87689) ;
#81982=STYLED_ITEM('',(#170169),#87690) ;
#81983=STYLED_ITEM('',(#170169),#87691) ;
#81984=STYLED_ITEM('',(#170169),#87692) ;
#81985=STYLED_ITEM('',(#170169),#87693) ;
#81986=STYLED_ITEM('',(#170169),#87694) ;
#81987=STYLED_ITEM('',(#170169),#87695) ;
#81988=STYLED_ITEM('',(#170169),#87696) ;
#81989=STYLED_ITEM('',(#170169),#87697) ;
#81990=STYLED_ITEM('',(#170169),#87698) ;
#81991=STYLED_ITEM('',(#170169),#87699) ;
#81992=STYLED_ITEM('',(#170169),#87700) ;
#81993=STYLED_ITEM('',(#170169),#87701) ;
#81994=STYLED_ITEM('',(#170169),#87702) ;
#81995=STYLED_ITEM('',(#170169),#87703) ;
#81996=STYLED_ITEM('',(#170169),#87704) ;
#81997=STYLED_ITEM('',(#170169),#87705) ;
#81998=STYLED_ITEM('',(#170169),#87706) ;
#81999=STYLED_ITEM('',(#170169),#87707) ;
#82000=STYLED_ITEM('',(#170169),#87708) ;
#82001=STYLED_ITEM('',(#170169),#87709) ;
#82002=STYLED_ITEM('',(#170169),#87710) ;
#82003=STYLED_ITEM('',(#170169),#87711) ;
#82004=STYLED_ITEM('',(#170169),#87712) ;
#82005=STYLED_ITEM('',(#170169),#87713) ;
#82006=STYLED_ITEM('',(#170169),#87714) ;
#82007=STYLED_ITEM('',(#170169),#87715) ;
#82008=STYLED_ITEM('',(#170169),#87716) ;
#82009=STYLED_ITEM('',(#170169),#87717) ;
#82010=STYLED_ITEM('',(#170169),#87718) ;
#82011=STYLED_ITEM('',(#170169),#87719) ;
#82012=STYLED_ITEM('',(#170169),#87720) ;
#82013=STYLED_ITEM('',(#170169),#87721) ;
#82014=STYLED_ITEM('',(#170169),#87722) ;
#82015=STYLED_ITEM('',(#170169),#87723) ;
#82016=STYLED_ITEM('',(#170169),#87724) ;
#82017=STYLED_ITEM('',(#170169),#87725) ;
#82018=STYLED_ITEM('',(#170169),#87726) ;
#82019=STYLED_ITEM('',(#170169),#87727) ;
#82020=STYLED_ITEM('',(#170169),#87728) ;
#82021=STYLED_ITEM('',(#170169),#87729) ;
#82022=STYLED_ITEM('',(#170169),#87730) ;
#82023=STYLED_ITEM('',(#170169),#87731) ;
#82024=STYLED_ITEM('',(#170169),#87732) ;
#82025=STYLED_ITEM('',(#170169),#87733) ;
#82026=STYLED_ITEM('',(#170169),#87734) ;
#82027=STYLED_ITEM('',(#170169),#87735) ;
#82028=STYLED_ITEM('',(#170169),#87736) ;
#82029=STYLED_ITEM('',(#170169),#87737) ;
#82030=STYLED_ITEM('',(#170169),#87738) ;
#82031=STYLED_ITEM('',(#170169),#87739) ;
#82032=STYLED_ITEM('',(#170169),#87740) ;
#82033=STYLED_ITEM('',(#170169),#87741) ;
#82034=STYLED_ITEM('',(#170169),#87742) ;
#82035=STYLED_ITEM('',(#170169),#87743) ;
#82036=STYLED_ITEM('',(#170169),#87744) ;
#82037=STYLED_ITEM('',(#170169),#87745) ;
#82038=STYLED_ITEM('',(#170169),#87746) ;
#82039=STYLED_ITEM('',(#170169),#87747) ;
#82040=STYLED_ITEM('',(#170169),#87748) ;
#82041=STYLED_ITEM('',(#170169),#87749) ;
#82042=STYLED_ITEM('',(#170169),#87750) ;
#82043=STYLED_ITEM('',(#170169),#87751) ;
#82044=STYLED_ITEM('',(#170169),#87752) ;
#82045=STYLED_ITEM('',(#170169),#87753) ;
#82046=STYLED_ITEM('',(#170169),#87754) ;
#82047=STYLED_ITEM('',(#170169),#87755) ;
#82048=STYLED_ITEM('',(#170169),#87756) ;
#82049=STYLED_ITEM('',(#170169),#87757) ;
#82050=STYLED_ITEM('',(#170169),#87758) ;
#82051=STYLED_ITEM('',(#170169),#87759) ;
#82052=STYLED_ITEM('',(#170169),#87760) ;
#82053=STYLED_ITEM('',(#170169),#87761) ;
#82054=STYLED_ITEM('',(#170169),#87762) ;
#82055=STYLED_ITEM('',(#170169),#87763) ;
#82056=STYLED_ITEM('',(#170169),#87764) ;
#82057=STYLED_ITEM('',(#170169),#87765) ;
#82058=STYLED_ITEM('',(#170169),#87766) ;
#82059=STYLED_ITEM('',(#170169),#87767) ;
#82060=STYLED_ITEM('',(#170169),#87768) ;
#82061=STYLED_ITEM('',(#170169),#87769) ;
#82062=STYLED_ITEM('',(#170169),#87770) ;
#82063=STYLED_ITEM('',(#170169),#87771) ;
#82064=STYLED_ITEM('',(#170169),#87772) ;
#82065=STYLED_ITEM('',(#170169),#87773) ;
#82066=STYLED_ITEM('',(#170169),#87774) ;
#82067=STYLED_ITEM('',(#170169),#87775) ;
#82068=STYLED_ITEM('',(#170169),#87776) ;
#82069=STYLED_ITEM('',(#170169),#87777) ;
#82070=STYLED_ITEM('',(#170169),#87778) ;
#82071=STYLED_ITEM('',(#170169),#87779) ;
#82072=STYLED_ITEM('',(#170169),#87780) ;
#82073=STYLED_ITEM('',(#170169),#87781) ;
#82074=STYLED_ITEM('',(#170169),#87782) ;
#82075=STYLED_ITEM('',(#170169),#87783) ;
#82076=STYLED_ITEM('',(#170169),#87784) ;
#82077=STYLED_ITEM('',(#170169),#87785) ;
#82078=STYLED_ITEM('',(#170169),#87786) ;
#82079=STYLED_ITEM('',(#170169),#87787) ;
#82080=STYLED_ITEM('',(#170169),#87788) ;
#82081=STYLED_ITEM('',(#170169),#87789) ;
#82082=STYLED_ITEM('',(#170169),#87790) ;
#82083=STYLED_ITEM('',(#170169),#87791) ;
#82084=STYLED_ITEM('',(#170169),#87792) ;
#82085=STYLED_ITEM('',(#170169),#87793) ;
#82086=STYLED_ITEM('',(#170169),#87794) ;
#82087=STYLED_ITEM('',(#170169),#87795) ;
#82088=STYLED_ITEM('',(#170169),#87796) ;
#82089=STYLED_ITEM('',(#170169),#87797) ;
#82090=STYLED_ITEM('',(#170169),#87798) ;
#82091=STYLED_ITEM('',(#170169),#87799) ;
#82092=STYLED_ITEM('',(#170169),#87800) ;
#82093=STYLED_ITEM('',(#170169),#87801) ;
#82094=STYLED_ITEM('',(#170169),#87802) ;
#82095=STYLED_ITEM('',(#170169),#87803) ;
#82096=STYLED_ITEM('',(#170169),#87804) ;
#82097=STYLED_ITEM('',(#170169),#87805) ;
#82098=STYLED_ITEM('',(#170169),#87806) ;
#82099=STYLED_ITEM('',(#170169),#87807) ;
#82100=STYLED_ITEM('',(#170169),#87808) ;
#82101=STYLED_ITEM('',(#170169),#87809) ;
#82102=STYLED_ITEM('',(#170169),#87810) ;
#82103=STYLED_ITEM('',(#170169),#87811) ;
#82104=STYLED_ITEM('',(#170169),#87812) ;
#82105=STYLED_ITEM('',(#170169),#87813) ;
#82106=STYLED_ITEM('',(#170169),#87814) ;
#82107=STYLED_ITEM('',(#170169),#87815) ;
#82108=STYLED_ITEM('',(#170169),#87816) ;
#82109=STYLED_ITEM('',(#170169),#87817) ;
#82110=STYLED_ITEM('',(#170169),#87818) ;
#82111=STYLED_ITEM('',(#170169),#87819) ;
#82112=STYLED_ITEM('',(#170169),#87820) ;
#82113=STYLED_ITEM('',(#170169),#87821) ;
#82114=STYLED_ITEM('',(#170169),#87822) ;
#82115=STYLED_ITEM('',(#170169),#87823) ;
#82116=STYLED_ITEM('',(#170169),#87824) ;
#82117=STYLED_ITEM('',(#170169),#87825) ;
#82118=STYLED_ITEM('',(#170169),#87826) ;
#82119=STYLED_ITEM('',(#170169),#87827) ;
#82120=STYLED_ITEM('',(#170169),#87828) ;
#82121=STYLED_ITEM('',(#170169),#87829) ;
#82122=STYLED_ITEM('',(#170169),#87830) ;
#82123=STYLED_ITEM('',(#170169),#87831) ;
#82124=STYLED_ITEM('',(#170169),#87832) ;
#82125=STYLED_ITEM('',(#170169),#87833) ;
#82126=STYLED_ITEM('',(#170169),#87834) ;
#82127=STYLED_ITEM('',(#170169),#87835) ;
#82128=STYLED_ITEM('',(#170169),#87836) ;
#82129=STYLED_ITEM('',(#170169),#87837) ;
#82130=STYLED_ITEM('',(#170169),#87838) ;
#82131=STYLED_ITEM('',(#170169),#87839) ;
#82132=STYLED_ITEM('',(#170169),#87840) ;
#82133=STYLED_ITEM('',(#170169),#87841) ;
#82134=STYLED_ITEM('',(#170169),#87842) ;
#82135=STYLED_ITEM('',(#170169),#87843) ;
#82136=STYLED_ITEM('',(#170169),#87844) ;
#82137=STYLED_ITEM('',(#170169),#87845) ;
#82138=STYLED_ITEM('',(#170169),#87846) ;
#82139=STYLED_ITEM('',(#170169),#87847) ;
#82140=STYLED_ITEM('',(#170169),#87848) ;
#82141=STYLED_ITEM('',(#170169),#87849) ;
#82142=STYLED_ITEM('',(#170169),#87850) ;
#82143=STYLED_ITEM('',(#170169),#87851) ;
#82144=STYLED_ITEM('',(#170169),#87852) ;
#82145=STYLED_ITEM('',(#170169),#87853) ;
#82146=STYLED_ITEM('',(#170169),#87854) ;
#82147=STYLED_ITEM('',(#170169),#87855) ;
#82148=STYLED_ITEM('',(#170169),#87856) ;
#82149=STYLED_ITEM('',(#170169),#87857) ;
#82150=STYLED_ITEM('',(#170169),#87858) ;
#82151=STYLED_ITEM('',(#170169),#87859) ;
#82152=STYLED_ITEM('',(#170169),#87860) ;
#82153=STYLED_ITEM('',(#170169),#87861) ;
#82154=STYLED_ITEM('',(#170169),#87862) ;
#82155=STYLED_ITEM('',(#170169),#87863) ;
#82156=STYLED_ITEM('',(#170169),#87864) ;
#82157=STYLED_ITEM('',(#170169),#87865) ;
#82158=STYLED_ITEM('',(#170169),#87866) ;
#82159=STYLED_ITEM('',(#170169),#87867) ;
#82160=STYLED_ITEM('',(#170169),#87868) ;
#82161=STYLED_ITEM('',(#170169),#87869) ;
#82162=STYLED_ITEM('',(#170169),#87870) ;
#82163=STYLED_ITEM('',(#170169),#87871) ;
#82164=STYLED_ITEM('',(#170169),#87872) ;
#82165=STYLED_ITEM('',(#170169),#87873) ;
#82166=STYLED_ITEM('',(#170169),#87874) ;
#82167=STYLED_ITEM('',(#170169),#87875) ;
#82168=STYLED_ITEM('',(#170169),#87876) ;
#82169=STYLED_ITEM('',(#170169),#87877) ;
#82170=STYLED_ITEM('',(#170169),#87878) ;
#82171=STYLED_ITEM('',(#170169),#87879) ;
#82172=STYLED_ITEM('',(#170169),#87880) ;
#82173=STYLED_ITEM('',(#170169),#87881) ;
#82174=STYLED_ITEM('',(#170169),#87882) ;
#82175=STYLED_ITEM('',(#170169),#87883) ;
#82176=STYLED_ITEM('',(#170169),#87884) ;
#82177=STYLED_ITEM('',(#170169),#87885) ;
#82178=STYLED_ITEM('',(#170169),#87886) ;
#82179=STYLED_ITEM('',(#170169),#87887) ;
#82180=STYLED_ITEM('',(#170169),#87888) ;
#82181=STYLED_ITEM('',(#170169),#87889) ;
#82182=STYLED_ITEM('',(#170169),#87890) ;
#82183=STYLED_ITEM('',(#170169),#87891) ;
#82184=STYLED_ITEM('',(#170169),#87892) ;
#82185=STYLED_ITEM('',(#170169),#87893) ;
#82186=STYLED_ITEM('',(#170169),#87894) ;
#82187=STYLED_ITEM('',(#170169),#87895) ;
#82188=STYLED_ITEM('',(#170169),#87896) ;
#82189=STYLED_ITEM('',(#170169),#87897) ;
#82190=STYLED_ITEM('',(#170169),#87898) ;
#82191=STYLED_ITEM('',(#170169),#87899) ;
#82192=STYLED_ITEM('',(#170169),#87900) ;
#82193=STYLED_ITEM('',(#170169),#87901) ;
#82194=STYLED_ITEM('',(#170169),#87902) ;
#82195=STYLED_ITEM('',(#170169),#87903) ;
#82196=STYLED_ITEM('',(#170169),#87904) ;
#82197=STYLED_ITEM('',(#170169),#87905) ;
#82198=STYLED_ITEM('',(#170169),#87906) ;
#82199=STYLED_ITEM('',(#170169),#87907) ;
#82200=STYLED_ITEM('',(#170169),#87908) ;
#82201=STYLED_ITEM('',(#170169),#87909) ;
#82202=STYLED_ITEM('',(#170169),#87910) ;
#82203=STYLED_ITEM('',(#170169),#87911) ;
#82204=STYLED_ITEM('',(#170169),#87912) ;
#82205=STYLED_ITEM('',(#170169),#87913) ;
#82206=STYLED_ITEM('',(#170169),#87914) ;
#82207=STYLED_ITEM('',(#170169),#87915) ;
#82208=STYLED_ITEM('',(#170169),#87916) ;
#82209=STYLED_ITEM('',(#170169),#87917) ;
#82210=STYLED_ITEM('',(#170169),#87918) ;
#82211=STYLED_ITEM('',(#170169),#87919) ;
#82212=STYLED_ITEM('',(#170169),#87920) ;
#82213=STYLED_ITEM('',(#170169),#87921) ;
#82214=STYLED_ITEM('',(#170169),#87922) ;
#82215=STYLED_ITEM('',(#170169),#87923) ;
#82216=STYLED_ITEM('',(#170169),#87924) ;
#82217=STYLED_ITEM('',(#170169),#87925) ;
#82218=STYLED_ITEM('',(#170169),#87926) ;
#82219=STYLED_ITEM('',(#170169),#87927) ;
#82220=STYLED_ITEM('',(#170169),#87928) ;
#82221=STYLED_ITEM('',(#170169),#87929) ;
#82222=STYLED_ITEM('',(#170169),#87930) ;
#82223=STYLED_ITEM('',(#170169),#87931) ;
#82224=STYLED_ITEM('',(#170169),#87932) ;
#82225=STYLED_ITEM('',(#170169),#87933) ;
#82226=STYLED_ITEM('',(#170169),#87934) ;
#82227=STYLED_ITEM('',(#170169),#87935) ;
#82228=STYLED_ITEM('',(#170169),#87936) ;
#82229=STYLED_ITEM('',(#170169),#87937) ;
#82230=STYLED_ITEM('',(#170169),#87938) ;
#82231=STYLED_ITEM('',(#170169),#87939) ;
#82232=STYLED_ITEM('',(#170169),#87940) ;
#82233=STYLED_ITEM('',(#170169),#87941) ;
#82234=STYLED_ITEM('',(#170169),#87942) ;
#82235=STYLED_ITEM('',(#170169),#87943) ;
#82236=STYLED_ITEM('',(#170169),#87944) ;
#82237=STYLED_ITEM('',(#170169),#87945) ;
#82238=STYLED_ITEM('',(#170169),#87946) ;
#82239=STYLED_ITEM('',(#170169),#87947) ;
#82240=STYLED_ITEM('',(#170169),#87948) ;
#82241=STYLED_ITEM('',(#170169),#87949) ;
#82242=STYLED_ITEM('',(#170169),#87950) ;
#82243=STYLED_ITEM('',(#170169),#87951) ;
#82244=STYLED_ITEM('',(#170169),#87952) ;
#82245=STYLED_ITEM('',(#170169),#87953) ;
#82246=STYLED_ITEM('',(#170169),#87954) ;
#82247=STYLED_ITEM('',(#170169),#87955) ;
#82248=STYLED_ITEM('',(#170169),#87956) ;
#82249=STYLED_ITEM('',(#170169),#87957) ;
#82250=STYLED_ITEM('',(#170169),#87958) ;
#82251=STYLED_ITEM('',(#170169),#87959) ;
#82252=STYLED_ITEM('',(#170169),#87960) ;
#82253=STYLED_ITEM('',(#170169),#87961) ;
#82254=STYLED_ITEM('',(#170169),#87962) ;
#82255=STYLED_ITEM('',(#170169),#87963) ;
#82256=STYLED_ITEM('',(#170169),#87964) ;
#82257=STYLED_ITEM('',(#170169),#87965) ;
#82258=STYLED_ITEM('',(#170169),#87966) ;
#82259=STYLED_ITEM('',(#170169),#87967) ;
#82260=STYLED_ITEM('',(#170169),#87968) ;
#82261=STYLED_ITEM('',(#170169),#87969) ;
#82262=STYLED_ITEM('',(#170169),#87970) ;
#82263=STYLED_ITEM('',(#170169),#87971) ;
#82264=STYLED_ITEM('',(#170169),#87972) ;
#82265=STYLED_ITEM('',(#170169),#87973) ;
#82266=STYLED_ITEM('',(#170169),#87974) ;
#82267=STYLED_ITEM('',(#170169),#87975) ;
#82268=STYLED_ITEM('',(#170169),#87976) ;
#82269=STYLED_ITEM('',(#170169),#87977) ;
#82270=STYLED_ITEM('',(#170169),#87978) ;
#82271=STYLED_ITEM('',(#170169),#87979) ;
#82272=STYLED_ITEM('',(#170169),#87980) ;
#82273=STYLED_ITEM('',(#170169),#87981) ;
#82274=STYLED_ITEM('',(#170169),#87982) ;
#82275=STYLED_ITEM('',(#170169),#87983) ;
#82276=STYLED_ITEM('',(#170169),#87984) ;
#82277=STYLED_ITEM('',(#170169),#87985) ;
#82278=STYLED_ITEM('',(#170169),#87986) ;
#82279=STYLED_ITEM('',(#170169),#87987) ;
#82280=STYLED_ITEM('',(#170169),#87988) ;
#82281=STYLED_ITEM('',(#170169),#87989) ;
#82282=STYLED_ITEM('',(#170169),#87990) ;
#82283=STYLED_ITEM('',(#170169),#87991) ;
#82284=STYLED_ITEM('',(#170169),#87992) ;
#82285=STYLED_ITEM('',(#170169),#87993) ;
#82286=STYLED_ITEM('',(#170169),#87994) ;
#82287=STYLED_ITEM('',(#170169),#87995) ;
#82288=STYLED_ITEM('',(#170169),#87996) ;
#82289=STYLED_ITEM('',(#170169),#87997) ;
#82290=STYLED_ITEM('',(#170169),#87998) ;
#82291=STYLED_ITEM('',(#170169),#87999) ;
#82292=STYLED_ITEM('',(#170169),#88000) ;
#82293=STYLED_ITEM('',(#170169),#88001) ;
#82294=STYLED_ITEM('',(#170169),#88002) ;
#82295=STYLED_ITEM('',(#170169),#88003) ;
#82296=STYLED_ITEM('',(#170169),#88004) ;
#82297=STYLED_ITEM('',(#170169),#88005) ;
#82298=STYLED_ITEM('',(#170169),#88006) ;
#82299=STYLED_ITEM('',(#170169),#88007) ;
#82300=STYLED_ITEM('',(#170169),#88008) ;
#82301=STYLED_ITEM('',(#170169),#88009) ;
#82302=STYLED_ITEM('',(#170169),#88010) ;
#82303=STYLED_ITEM('',(#170169),#88011) ;
#82304=STYLED_ITEM('',(#170169),#88012) ;
#82305=STYLED_ITEM('',(#170169),#88013) ;
#82306=STYLED_ITEM('',(#170169),#88014) ;
#82307=STYLED_ITEM('',(#170169),#88015) ;
#82308=STYLED_ITEM('',(#170169),#88016) ;
#82309=STYLED_ITEM('',(#170169),#88017) ;
#82310=STYLED_ITEM('',(#170169),#88018) ;
#82311=STYLED_ITEM('',(#170169),#88019) ;
#82312=STYLED_ITEM('',(#170169),#88020) ;
#82313=STYLED_ITEM('',(#170169),#88021) ;
#82314=STYLED_ITEM('',(#170169),#88022) ;
#82315=STYLED_ITEM('',(#170169),#88023) ;
#82316=STYLED_ITEM('',(#170169),#88024) ;
#82317=STYLED_ITEM('',(#170169),#88025) ;
#82318=STYLED_ITEM('',(#170169),#88026) ;
#82319=STYLED_ITEM('',(#170169),#88027) ;
#82320=STYLED_ITEM('',(#170169),#88028) ;
#82321=STYLED_ITEM('',(#170169),#88029) ;
#82322=STYLED_ITEM('',(#170169),#88030) ;
#82323=STYLED_ITEM('',(#170169),#88031) ;
#82324=STYLED_ITEM('',(#170169),#88032) ;
#82325=STYLED_ITEM('',(#170169),#88033) ;
#82326=STYLED_ITEM('',(#170169),#88034) ;
#82327=STYLED_ITEM('',(#170169),#88035) ;
#82328=STYLED_ITEM('',(#170169),#88036) ;
#82329=STYLED_ITEM('',(#170169),#88037) ;
#82330=STYLED_ITEM('',(#170169),#88038) ;
#82331=STYLED_ITEM('',(#170169),#88039) ;
#82332=STYLED_ITEM('',(#170169),#88040) ;
#82333=STYLED_ITEM('',(#170169),#88041) ;
#82334=STYLED_ITEM('',(#170169),#88042) ;
#82335=STYLED_ITEM('',(#170169),#88043) ;
#82336=STYLED_ITEM('',(#170169),#88044) ;
#82337=STYLED_ITEM('',(#170169),#88045) ;
#82338=STYLED_ITEM('',(#170169),#88046) ;
#82339=STYLED_ITEM('',(#170169),#88047) ;
#82340=STYLED_ITEM('',(#170169),#88048) ;
#82341=STYLED_ITEM('',(#170169),#88049) ;
#82342=STYLED_ITEM('',(#170169),#88050) ;
#82343=STYLED_ITEM('',(#170169),#88051) ;
#82344=STYLED_ITEM('',(#170169),#88052) ;
#82345=STYLED_ITEM('',(#170169),#88053) ;
#82346=STYLED_ITEM('',(#170169),#88054) ;
#82347=STYLED_ITEM('',(#170169),#88055) ;
#82348=STYLED_ITEM('',(#170169),#88056) ;
#82349=STYLED_ITEM('',(#170169),#88057) ;
#82350=STYLED_ITEM('',(#170169),#88058) ;
#82351=STYLED_ITEM('',(#170169),#88059) ;
#82352=STYLED_ITEM('',(#170169),#88060) ;
#82353=STYLED_ITEM('',(#170169),#88061) ;
#82354=STYLED_ITEM('',(#170169),#88062) ;
#82355=STYLED_ITEM('',(#170169),#88063) ;
#82356=STYLED_ITEM('',(#170169),#88064) ;
#82357=STYLED_ITEM('',(#170169),#88065) ;
#82358=STYLED_ITEM('',(#170169),#88066) ;
#82359=STYLED_ITEM('',(#170169),#88067) ;
#82360=STYLED_ITEM('',(#170169),#88068) ;
#82361=STYLED_ITEM('',(#170169),#88069) ;
#82362=STYLED_ITEM('',(#170171),#88070) ;
#82363=STYLED_ITEM('',(#170171),#88071) ;
#82364=STYLED_ITEM('',(#170171),#88072) ;
#82365=STYLED_ITEM('',(#170171),#88073) ;
#82366=STYLED_ITEM('',(#170171),#88074) ;
#82367=STYLED_ITEM('',(#170171),#88075) ;
#82368=STYLED_ITEM('',(#170171),#88076) ;
#82369=STYLED_ITEM('',(#170171),#88077) ;
#82370=STYLED_ITEM('',(#170171),#88078) ;
#82371=STYLED_ITEM('',(#170171),#88079) ;
#82372=STYLED_ITEM('',(#170171),#88080) ;
#82373=STYLED_ITEM('',(#170171),#88081) ;
#82374=STYLED_ITEM('',(#170171),#88082) ;
#82375=STYLED_ITEM('',(#170171),#88083) ;
#82376=STYLED_ITEM('',(#170171),#88084) ;
#82377=STYLED_ITEM('',(#170171),#88085) ;
#82378=STYLED_ITEM('',(#170171),#88086) ;
#82379=STYLED_ITEM('',(#170171),#88087) ;
#82380=STYLED_ITEM('',(#170171),#88088) ;
#82381=STYLED_ITEM('',(#170171),#88089) ;
#82382=STYLED_ITEM('',(#170171),#88090) ;
#82383=STYLED_ITEM('',(#170171),#88091) ;
#82384=STYLED_ITEM('',(#170171),#88092) ;
#82385=STYLED_ITEM('',(#170171),#88093) ;
#82386=STYLED_ITEM('',(#170171),#88094) ;
#82387=STYLED_ITEM('',(#170171),#88095) ;
#82388=STYLED_ITEM('',(#170171),#88096) ;
#82389=STYLED_ITEM('',(#170171),#88097) ;
#82390=STYLED_ITEM('',(#170171),#88098) ;
#82391=STYLED_ITEM('',(#170171),#88099) ;
#82392=STYLED_ITEM('',(#170171),#88100) ;
#82393=STYLED_ITEM('',(#170171),#88101) ;
#82394=STYLED_ITEM('',(#170171),#88102) ;
#82395=STYLED_ITEM('',(#170171),#88103) ;
#82396=STYLED_ITEM('',(#170171),#88104) ;
#82397=STYLED_ITEM('',(#170171),#88105) ;
#82398=STYLED_ITEM('',(#170171),#88106) ;
#82399=STYLED_ITEM('',(#170171),#88107) ;
#82400=STYLED_ITEM('',(#170171),#88108) ;
#82401=STYLED_ITEM('',(#170171),#88109) ;
#82402=STYLED_ITEM('',(#170171),#88110) ;
#82403=STYLED_ITEM('',(#170171),#88111) ;
#82404=STYLED_ITEM('',(#170171),#88112) ;
#82405=STYLED_ITEM('',(#170171),#88113) ;
#82406=STYLED_ITEM('',(#170171),#88114) ;
#82407=STYLED_ITEM('',(#170171),#88115) ;
#82408=STYLED_ITEM('',(#170171),#88116) ;
#82409=STYLED_ITEM('',(#170171),#88117) ;
#82410=STYLED_ITEM('',(#170171),#88118) ;
#82411=STYLED_ITEM('',(#170171),#88119) ;
#82412=STYLED_ITEM('',(#170171),#88120) ;
#82413=STYLED_ITEM('',(#170171),#88121) ;
#82414=STYLED_ITEM('',(#170171),#88122) ;
#82415=STYLED_ITEM('',(#170171),#88123) ;
#82416=STYLED_ITEM('',(#170171),#88124) ;
#82417=STYLED_ITEM('',(#170171),#88125) ;
#82418=STYLED_ITEM('',(#170171),#88126) ;
#82419=STYLED_ITEM('',(#170171),#88127) ;
#82420=STYLED_ITEM('',(#170171),#88128) ;
#82421=STYLED_ITEM('',(#170171),#88129) ;
#82422=STYLED_ITEM('',(#170171),#88130) ;
#82423=STYLED_ITEM('',(#170171),#88131) ;
#82424=STYLED_ITEM('',(#170171),#88132) ;
#82425=STYLED_ITEM('',(#170171),#88133) ;
#82426=STYLED_ITEM('',(#170171),#88134) ;
#82427=STYLED_ITEM('',(#170171),#88135) ;
#82428=STYLED_ITEM('',(#170171),#88136) ;
#82429=STYLED_ITEM('',(#170171),#88137) ;
#82430=STYLED_ITEM('',(#170171),#88138) ;
#82431=STYLED_ITEM('',(#170171),#88139) ;
#82432=STYLED_ITEM('',(#170171),#88140) ;
#82433=STYLED_ITEM('',(#170171),#88141) ;
#82434=STYLED_ITEM('',(#170171),#88142) ;
#82435=STYLED_ITEM('',(#170171),#88143) ;
#82436=STYLED_ITEM('',(#170171),#88144) ;
#82437=STYLED_ITEM('',(#170171),#88145) ;
#82438=STYLED_ITEM('',(#170171),#88146) ;
#82439=STYLED_ITEM('',(#170171),#88147) ;
#82440=STYLED_ITEM('',(#170171),#88148) ;
#82441=STYLED_ITEM('',(#170171),#88149) ;
#82442=STYLED_ITEM('',(#170171),#88150) ;
#82443=STYLED_ITEM('',(#170171),#88151) ;
#82444=STYLED_ITEM('',(#170171),#88152) ;
#82445=STYLED_ITEM('',(#170171),#88153) ;
#82446=STYLED_ITEM('',(#170171),#88154) ;
#82447=STYLED_ITEM('',(#170171),#88155) ;
#82448=STYLED_ITEM('',(#170171),#88156) ;
#82449=STYLED_ITEM('',(#170171),#88157) ;
#82450=STYLED_ITEM('',(#170171),#88158) ;
#82451=STYLED_ITEM('',(#170171),#88159) ;
#82452=STYLED_ITEM('',(#170171),#88160) ;
#82453=STYLED_ITEM('',(#170171),#88161) ;
#82454=STYLED_ITEM('',(#170171),#88162) ;
#82455=STYLED_ITEM('',(#170171),#88163) ;
#82456=STYLED_ITEM('',(#170171),#88164) ;
#82457=STYLED_ITEM('',(#170171),#88165) ;
#82458=STYLED_ITEM('',(#170171),#88166) ;
#82459=STYLED_ITEM('',(#170171),#88167) ;
#82460=STYLED_ITEM('',(#170171),#88168) ;
#82461=STYLED_ITEM('',(#170171),#88169) ;
#82462=STYLED_ITEM('',(#170171),#88170) ;
#82463=STYLED_ITEM('',(#170171),#88171) ;
#82464=STYLED_ITEM('',(#170171),#88172) ;
#82465=STYLED_ITEM('',(#170171),#88173) ;
#82466=STYLED_ITEM('',(#170171),#88174) ;
#82467=STYLED_ITEM('',(#170171),#88175) ;
#82468=STYLED_ITEM('',(#170171),#88176) ;
#82469=STYLED_ITEM('',(#170171),#88177) ;
#82470=STYLED_ITEM('',(#170171),#88178) ;
#82471=STYLED_ITEM('',(#170171),#88179) ;
#82472=STYLED_ITEM('',(#170171),#88180) ;
#82473=STYLED_ITEM('',(#170171),#88181) ;
#82474=STYLED_ITEM('',(#170171),#88182) ;
#82475=STYLED_ITEM('',(#170171),#88183) ;
#82476=STYLED_ITEM('',(#170171),#88184) ;
#82477=STYLED_ITEM('',(#170171),#88185) ;
#82478=STYLED_ITEM('',(#170171),#88186) ;
#82479=STYLED_ITEM('',(#170171),#88187) ;
#82480=STYLED_ITEM('',(#170171),#88188) ;
#82481=STYLED_ITEM('',(#170171),#88189) ;
#82482=STYLED_ITEM('',(#170171),#88190) ;
#82483=STYLED_ITEM('',(#170171),#88191) ;
#82484=STYLED_ITEM('',(#170171),#88192) ;
#82485=STYLED_ITEM('',(#170171),#88193) ;
#82486=STYLED_ITEM('',(#170171),#88194) ;
#82487=STYLED_ITEM('',(#170171),#88195) ;
#82488=STYLED_ITEM('',(#170171),#88196) ;
#82489=STYLED_ITEM('',(#170171),#88197) ;
#82490=STYLED_ITEM('',(#170171),#88198) ;
#82491=STYLED_ITEM('',(#170171),#88199) ;
#82492=STYLED_ITEM('',(#170171),#88200) ;
#82493=STYLED_ITEM('',(#170171),#88201) ;
#82494=STYLED_ITEM('',(#170171),#88202) ;
#82495=STYLED_ITEM('',(#170171),#88203) ;
#82496=STYLED_ITEM('',(#170171),#88204) ;
#82497=STYLED_ITEM('',(#170171),#88205) ;
#82498=STYLED_ITEM('',(#170171),#88206) ;
#82499=STYLED_ITEM('',(#170171),#88207) ;
#82500=STYLED_ITEM('',(#170171),#88208) ;
#82501=STYLED_ITEM('',(#170171),#88209) ;
#82502=STYLED_ITEM('',(#170171),#88210) ;
#82503=STYLED_ITEM('',(#170171),#88211) ;
#82504=STYLED_ITEM('',(#170171),#88212) ;
#82505=STYLED_ITEM('',(#170171),#88213) ;
#82506=STYLED_ITEM('',(#170171),#88214) ;
#82507=STYLED_ITEM('',(#170171),#88215) ;
#82508=STYLED_ITEM('',(#170171),#88216) ;
#82509=STYLED_ITEM('',(#170171),#88217) ;
#82510=STYLED_ITEM('',(#170171),#88218) ;
#82511=STYLED_ITEM('',(#170171),#88219) ;
#82512=STYLED_ITEM('',(#170171),#88220) ;
#82513=STYLED_ITEM('',(#170171),#88221) ;
#82514=STYLED_ITEM('',(#170171),#88222) ;
#82515=STYLED_ITEM('',(#170171),#88223) ;
#82516=STYLED_ITEM('',(#170171),#88224) ;
#82517=STYLED_ITEM('',(#170171),#88225) ;
#82518=STYLED_ITEM('',(#170171),#88226) ;
#82519=STYLED_ITEM('',(#170171),#88227) ;
#82520=STYLED_ITEM('',(#170171),#88228) ;
#82521=STYLED_ITEM('',(#170171),#88229) ;
#82522=STYLED_ITEM('',(#170171),#88230) ;
#82523=STYLED_ITEM('',(#170171),#88231) ;
#82524=STYLED_ITEM('',(#170171),#88232) ;
#82525=STYLED_ITEM('',(#170171),#88233) ;
#82526=STYLED_ITEM('',(#170171),#88234) ;
#82527=STYLED_ITEM('',(#170171),#88235) ;
#82528=STYLED_ITEM('',(#170171),#88236) ;
#82529=STYLED_ITEM('',(#170171),#88237) ;
#82530=STYLED_ITEM('',(#170171),#88238) ;
#82531=STYLED_ITEM('',(#170171),#88239) ;
#82532=STYLED_ITEM('',(#170171),#88240) ;
#82533=STYLED_ITEM('',(#170171),#88241) ;
#82534=STYLED_ITEM('',(#170171),#88242) ;
#82535=STYLED_ITEM('',(#170171),#88243) ;
#82536=STYLED_ITEM('',(#170171),#88244) ;
#82537=STYLED_ITEM('',(#170171),#88245) ;
#82538=STYLED_ITEM('',(#170171),#88246) ;
#82539=STYLED_ITEM('',(#170171),#88247) ;
#82540=STYLED_ITEM('',(#170171),#88248) ;
#82541=STYLED_ITEM('',(#170171),#88249) ;
#82542=STYLED_ITEM('',(#170171),#88250) ;
#82543=STYLED_ITEM('',(#170171),#88251) ;
#82544=STYLED_ITEM('',(#170171),#88252) ;
#82545=STYLED_ITEM('',(#170171),#88253) ;
#82546=STYLED_ITEM('',(#170171),#88254) ;
#82547=STYLED_ITEM('',(#170171),#88255) ;
#82548=STYLED_ITEM('',(#170171),#88256) ;
#82549=STYLED_ITEM('',(#170171),#88257) ;
#82550=STYLED_ITEM('',(#170171),#88258) ;
#82551=STYLED_ITEM('',(#170171),#88259) ;
#82552=STYLED_ITEM('',(#170171),#88260) ;
#82553=STYLED_ITEM('',(#170171),#88261) ;
#82554=STYLED_ITEM('',(#170171),#88262) ;
#82555=STYLED_ITEM('',(#170171),#88263) ;
#82556=STYLED_ITEM('',(#170171),#88264) ;
#82557=STYLED_ITEM('',(#170171),#88265) ;
#82558=STYLED_ITEM('',(#170171),#88266) ;
#82559=STYLED_ITEM('',(#170171),#88267) ;
#82560=STYLED_ITEM('',(#170171),#88268) ;
#82561=STYLED_ITEM('',(#170171),#88269) ;
#82562=STYLED_ITEM('',(#170171),#88270) ;
#82563=STYLED_ITEM('',(#170171),#88271) ;
#82564=STYLED_ITEM('',(#170171),#88272) ;
#82565=STYLED_ITEM('',(#170171),#88273) ;
#82566=STYLED_ITEM('',(#170171),#88274) ;
#82567=STYLED_ITEM('',(#170171),#88275) ;
#82568=STYLED_ITEM('',(#170171),#88276) ;
#82569=STYLED_ITEM('',(#170171),#88277) ;
#82570=STYLED_ITEM('',(#170171),#88278) ;
#82571=STYLED_ITEM('',(#170171),#88279) ;
#82572=STYLED_ITEM('',(#170171),#88280) ;
#82573=STYLED_ITEM('',(#170171),#88281) ;
#82574=STYLED_ITEM('',(#170171),#88282) ;
#82575=STYLED_ITEM('',(#170171),#88283) ;
#82576=STYLED_ITEM('',(#170171),#88284) ;
#82577=STYLED_ITEM('',(#170171),#88285) ;
#82578=STYLED_ITEM('',(#170171),#88286) ;
#82579=STYLED_ITEM('',(#170171),#88287) ;
#82580=STYLED_ITEM('',(#170171),#88288) ;
#82581=STYLED_ITEM('',(#170171),#88289) ;
#82582=STYLED_ITEM('',(#170171),#88290) ;
#82583=STYLED_ITEM('',(#170171),#88291) ;
#82584=STYLED_ITEM('',(#170171),#88292) ;
#82585=STYLED_ITEM('',(#170171),#88293) ;
#82586=STYLED_ITEM('',(#170171),#88294) ;
#82587=STYLED_ITEM('',(#170171),#88295) ;
#82588=STYLED_ITEM('',(#170171),#88296) ;
#82589=STYLED_ITEM('',(#170171),#88297) ;
#82590=STYLED_ITEM('',(#170171),#88298) ;
#82591=STYLED_ITEM('',(#170171),#88299) ;
#82592=STYLED_ITEM('',(#170171),#88300) ;
#82593=STYLED_ITEM('',(#170171),#88301) ;
#82594=STYLED_ITEM('',(#170171),#88302) ;
#82595=STYLED_ITEM('',(#170171),#88303) ;
#82596=STYLED_ITEM('',(#170171),#88304) ;
#82597=STYLED_ITEM('',(#170171),#88305) ;
#82598=STYLED_ITEM('',(#170171),#88306) ;
#82599=STYLED_ITEM('',(#170171),#88307) ;
#82600=STYLED_ITEM('',(#170171),#88308) ;
#82601=STYLED_ITEM('',(#170171),#88309) ;
#82602=STYLED_ITEM('',(#170171),#88310) ;
#82603=STYLED_ITEM('',(#170171),#88311) ;
#82604=STYLED_ITEM('',(#170171),#88312) ;
#82605=STYLED_ITEM('',(#170171),#88313) ;
#82606=STYLED_ITEM('',(#170171),#88314) ;
#82607=STYLED_ITEM('',(#170171),#88315) ;
#82608=STYLED_ITEM('',(#170171),#88316) ;
#82609=STYLED_ITEM('',(#170171),#88317) ;
#82610=STYLED_ITEM('',(#170171),#88318) ;
#82611=STYLED_ITEM('',(#170171),#88319) ;
#82612=STYLED_ITEM('',(#170171),#88320) ;
#82613=STYLED_ITEM('',(#170171),#88321) ;
#82614=STYLED_ITEM('',(#170171),#88322) ;
#82615=STYLED_ITEM('',(#170171),#88323) ;
#82616=STYLED_ITEM('',(#170171),#88324) ;
#82617=STYLED_ITEM('',(#170171),#88325) ;
#82618=STYLED_ITEM('',(#170171),#88326) ;
#82619=STYLED_ITEM('',(#170171),#88327) ;
#82620=STYLED_ITEM('',(#170171),#88328) ;
#82621=STYLED_ITEM('',(#170171),#88329) ;
#82622=STYLED_ITEM('',(#170171),#88330) ;
#82623=STYLED_ITEM('',(#170171),#88331) ;
#82624=STYLED_ITEM('',(#170171),#88332) ;
#82625=STYLED_ITEM('',(#170171),#88333) ;
#82626=STYLED_ITEM('',(#170171),#88334) ;
#82627=STYLED_ITEM('',(#170171),#88335) ;
#82628=STYLED_ITEM('',(#170171),#88336) ;
#82629=STYLED_ITEM('',(#170171),#88337) ;
#82630=STYLED_ITEM('',(#170171),#88338) ;
#82631=STYLED_ITEM('',(#170171),#88339) ;
#82632=STYLED_ITEM('',(#170171),#88340) ;
#82633=STYLED_ITEM('',(#170171),#88341) ;
#82634=STYLED_ITEM('',(#170171),#88342) ;
#82635=STYLED_ITEM('',(#170171),#88343) ;
#82636=STYLED_ITEM('',(#170171),#88344) ;
#82637=STYLED_ITEM('',(#170171),#88345) ;
#82638=STYLED_ITEM('',(#170171),#88346) ;
#82639=STYLED_ITEM('',(#170171),#88347) ;
#82640=STYLED_ITEM('',(#170171),#88348) ;
#82641=STYLED_ITEM('',(#170171),#88349) ;
#82642=STYLED_ITEM('',(#170171),#88350) ;
#82643=STYLED_ITEM('',(#170171),#88351) ;
#82644=STYLED_ITEM('',(#170171),#88352) ;
#82645=STYLED_ITEM('',(#170171),#88353) ;
#82646=STYLED_ITEM('',(#170171),#88354) ;
#82647=STYLED_ITEM('',(#170171),#88355) ;
#82648=STYLED_ITEM('',(#170171),#88356) ;
#82649=STYLED_ITEM('',(#170171),#88357) ;
#82650=STYLED_ITEM('',(#170171),#88358) ;
#82651=STYLED_ITEM('',(#170171),#88359) ;
#82652=STYLED_ITEM('',(#170171),#88360) ;
#82653=STYLED_ITEM('',(#170171),#88361) ;
#82654=STYLED_ITEM('',(#170171),#88362) ;
#82655=STYLED_ITEM('',(#170171),#88363) ;
#82656=STYLED_ITEM('',(#170171),#88364) ;
#82657=STYLED_ITEM('',(#170171),#88365) ;
#82658=STYLED_ITEM('',(#170171),#88366) ;
#82659=STYLED_ITEM('',(#170171),#88367) ;
#82660=STYLED_ITEM('',(#170171),#88368) ;
#82661=STYLED_ITEM('',(#170171),#88369) ;
#82662=STYLED_ITEM('',(#170171),#88370) ;
#82663=STYLED_ITEM('',(#170171),#88371) ;
#82664=STYLED_ITEM('',(#170171),#88372) ;
#82665=STYLED_ITEM('',(#170171),#88373) ;
#82666=STYLED_ITEM('',(#170171),#88374) ;
#82667=STYLED_ITEM('',(#170171),#88375) ;
#82668=STYLED_ITEM('',(#170171),#88376) ;
#82669=STYLED_ITEM('',(#170171),#88377) ;
#82670=STYLED_ITEM('',(#170171),#88378) ;
#82671=STYLED_ITEM('',(#170171),#88379) ;
#82672=STYLED_ITEM('',(#170171),#88380) ;
#82673=STYLED_ITEM('',(#170171),#88381) ;
#82674=STYLED_ITEM('',(#170171),#88382) ;
#82675=STYLED_ITEM('',(#170171),#88383) ;
#82676=STYLED_ITEM('',(#170171),#88384) ;
#82677=STYLED_ITEM('',(#170171),#88385) ;
#82678=STYLED_ITEM('',(#170171),#88386) ;
#82679=STYLED_ITEM('',(#170171),#88387) ;
#82680=STYLED_ITEM('',(#170171),#88388) ;
#82681=STYLED_ITEM('',(#170171),#88389) ;
#82682=STYLED_ITEM('',(#170171),#88390) ;
#82683=STYLED_ITEM('',(#170171),#88391) ;
#82684=STYLED_ITEM('',(#170171),#88392) ;
#82685=STYLED_ITEM('',(#170171),#88393) ;
#82686=STYLED_ITEM('',(#170171),#88394) ;
#82687=STYLED_ITEM('',(#170171),#88395) ;
#82688=STYLED_ITEM('',(#170171),#88396) ;
#82689=STYLED_ITEM('',(#170171),#88397) ;
#82690=STYLED_ITEM('',(#170171),#88398) ;
#82691=STYLED_ITEM('',(#170171),#88399) ;
#82692=STYLED_ITEM('',(#170171),#88400) ;
#82693=STYLED_ITEM('',(#170171),#88401) ;
#82694=STYLED_ITEM('',(#170171),#88402) ;
#82695=STYLED_ITEM('',(#170171),#88403) ;
#82696=STYLED_ITEM('',(#170171),#88404) ;
#82697=STYLED_ITEM('',(#170171),#88405) ;
#82698=STYLED_ITEM('',(#170171),#88406) ;
#82699=STYLED_ITEM('',(#170171),#88407) ;
#82700=STYLED_ITEM('',(#170171),#88408) ;
#82701=STYLED_ITEM('',(#170171),#88409) ;
#82702=STYLED_ITEM('',(#170171),#88410) ;
#82703=STYLED_ITEM('',(#170171),#88411) ;
#82704=STYLED_ITEM('',(#170171),#88412) ;
#82705=STYLED_ITEM('',(#170171),#88413) ;
#82706=STYLED_ITEM('',(#170171),#88414) ;
#82707=STYLED_ITEM('',(#170171),#88415) ;
#82708=STYLED_ITEM('',(#170171),#88416) ;
#82709=STYLED_ITEM('',(#170171),#88417) ;
#82710=STYLED_ITEM('',(#170171),#88418) ;
#82711=STYLED_ITEM('',(#170171),#88419) ;
#82712=STYLED_ITEM('',(#170171),#88420) ;
#82713=STYLED_ITEM('',(#170171),#88421) ;
#82714=STYLED_ITEM('',(#170171),#88422) ;
#82715=STYLED_ITEM('',(#170171),#88423) ;
#82716=STYLED_ITEM('',(#170171),#88424) ;
#82717=STYLED_ITEM('',(#170171),#88425) ;
#82718=STYLED_ITEM('',(#170171),#88426) ;
#82719=STYLED_ITEM('',(#170171),#88427) ;
#82720=STYLED_ITEM('',(#170171),#88428) ;
#82721=STYLED_ITEM('',(#170171),#88429) ;
#82722=STYLED_ITEM('',(#170171),#88430) ;
#82723=STYLED_ITEM('',(#170171),#88431) ;
#82724=STYLED_ITEM('',(#170171),#88432) ;
#82725=STYLED_ITEM('',(#170171),#88433) ;
#82726=STYLED_ITEM('',(#170171),#88434) ;
#82727=STYLED_ITEM('',(#170171),#88435) ;
#82728=STYLED_ITEM('',(#170171),#88436) ;
#82729=STYLED_ITEM('',(#170171),#88437) ;
#82730=STYLED_ITEM('',(#170171),#88438) ;
#82731=STYLED_ITEM('',(#170171),#88439) ;
#82732=STYLED_ITEM('',(#170171),#88440) ;
#82733=STYLED_ITEM('',(#170171),#88441) ;
#82734=STYLED_ITEM('',(#170171),#88442) ;
#82735=STYLED_ITEM('',(#170171),#88443) ;
#82736=STYLED_ITEM('',(#170171),#88444) ;
#82737=STYLED_ITEM('',(#170171),#88445) ;
#82738=STYLED_ITEM('',(#170171),#88446) ;
#82739=STYLED_ITEM('',(#170171),#88447) ;
#82740=STYLED_ITEM('',(#170171),#88448) ;
#82741=STYLED_ITEM('',(#170171),#88449) ;
#82742=STYLED_ITEM('',(#170171),#88450) ;
#82743=STYLED_ITEM('',(#170171),#88451) ;
#82744=STYLED_ITEM('',(#170171),#88452) ;
#82745=STYLED_ITEM('',(#170171),#88453) ;
#82746=STYLED_ITEM('',(#170171),#88454) ;
#82747=STYLED_ITEM('',(#170171),#88455) ;
#82748=STYLED_ITEM('',(#170171),#88456) ;
#82749=STYLED_ITEM('',(#170171),#88457) ;
#82750=STYLED_ITEM('',(#170171),#88458) ;
#82751=STYLED_ITEM('',(#170171),#88459) ;
#82752=STYLED_ITEM('',(#170171),#88460) ;
#82753=STYLED_ITEM('',(#170171),#88461) ;
#82754=STYLED_ITEM('',(#170171),#88462) ;
#82755=STYLED_ITEM('',(#170171),#88463) ;
#82756=STYLED_ITEM('',(#170171),#88464) ;
#82757=STYLED_ITEM('',(#170171),#88465) ;
#82758=STYLED_ITEM('',(#170171),#88466) ;
#82759=STYLED_ITEM('',(#170171),#88467) ;
#82760=STYLED_ITEM('',(#170171),#88468) ;
#82761=STYLED_ITEM('',(#170171),#88469) ;
#82762=STYLED_ITEM('',(#170171),#88470) ;
#82763=STYLED_ITEM('',(#170171),#88471) ;
#82764=STYLED_ITEM('',(#170171),#88472) ;
#82765=STYLED_ITEM('',(#170171),#88473) ;
#82766=STYLED_ITEM('',(#170171),#88474) ;
#82767=STYLED_ITEM('',(#170171),#88475) ;
#82768=STYLED_ITEM('',(#170171),#88476) ;
#82769=STYLED_ITEM('',(#170171),#88477) ;
#82770=STYLED_ITEM('',(#170171),#88478) ;
#82771=STYLED_ITEM('',(#170171),#88479) ;
#82772=STYLED_ITEM('',(#170171),#88480) ;
#82773=STYLED_ITEM('',(#170171),#88481) ;
#82774=STYLED_ITEM('',(#170171),#88482) ;
#82775=STYLED_ITEM('',(#170171),#88483) ;
#82776=STYLED_ITEM('',(#170171),#88484) ;
#82777=STYLED_ITEM('',(#170171),#88485) ;
#82778=STYLED_ITEM('',(#170171),#88486) ;
#82779=STYLED_ITEM('',(#170171),#88487) ;
#82780=STYLED_ITEM('',(#170171),#88488) ;
#82781=STYLED_ITEM('',(#170171),#88489) ;
#82782=STYLED_ITEM('',(#170171),#88490) ;
#82783=STYLED_ITEM('',(#170171),#88491) ;
#82784=STYLED_ITEM('',(#170171),#88492) ;
#82785=STYLED_ITEM('',(#170171),#88493) ;
#82786=STYLED_ITEM('',(#170171),#88494) ;
#82787=STYLED_ITEM('',(#170171),#88495) ;
#82788=STYLED_ITEM('',(#170171),#88496) ;
#82789=STYLED_ITEM('',(#170171),#88497) ;
#82790=STYLED_ITEM('',(#170171),#88498) ;
#82791=STYLED_ITEM('',(#170171),#88499) ;
#82792=STYLED_ITEM('',(#170171),#88500) ;
#82793=STYLED_ITEM('',(#170171),#88501) ;
#82794=STYLED_ITEM('',(#170171),#88502) ;
#82795=STYLED_ITEM('',(#170171),#88503) ;
#82796=STYLED_ITEM('',(#170171),#88504) ;
#82797=STYLED_ITEM('',(#170171),#88505) ;
#82798=STYLED_ITEM('',(#170171),#88506) ;
#82799=STYLED_ITEM('',(#170171),#88507) ;
#82800=STYLED_ITEM('',(#170171),#88508) ;
#82801=STYLED_ITEM('',(#170171),#88509) ;
#82802=STYLED_ITEM('',(#170171),#88510) ;
#82803=STYLED_ITEM('',(#170171),#88511) ;
#82804=STYLED_ITEM('',(#170171),#88512) ;
#82805=STYLED_ITEM('',(#170171),#88513) ;
#82806=STYLED_ITEM('',(#170171),#88514) ;
#82807=STYLED_ITEM('',(#170171),#88515) ;
#82808=STYLED_ITEM('',(#170171),#88516) ;
#82809=STYLED_ITEM('',(#170171),#88517) ;
#82810=STYLED_ITEM('',(#170171),#88518) ;
#82811=STYLED_ITEM('',(#170171),#88519) ;
#82812=STYLED_ITEM('',(#170171),#88520) ;
#82813=STYLED_ITEM('',(#170171),#88521) ;
#82814=STYLED_ITEM('',(#170171),#88522) ;
#82815=STYLED_ITEM('',(#170171),#88523) ;
#82816=STYLED_ITEM('',(#170171),#88524) ;
#82817=STYLED_ITEM('',(#170171),#88525) ;
#82818=STYLED_ITEM('',(#170171),#88526) ;
#82819=STYLED_ITEM('',(#170171),#88527) ;
#82820=STYLED_ITEM('',(#170171),#88528) ;
#82821=STYLED_ITEM('',(#170171),#88529) ;
#82822=STYLED_ITEM('',(#170171),#88530) ;
#82823=STYLED_ITEM('',(#170171),#88531) ;
#82824=STYLED_ITEM('',(#170171),#88532) ;
#82825=STYLED_ITEM('',(#170171),#88533) ;
#82826=STYLED_ITEM('',(#170171),#88534) ;
#82827=STYLED_ITEM('',(#170171),#88535) ;
#82828=STYLED_ITEM('',(#170171),#88536) ;
#82829=STYLED_ITEM('',(#170171),#88537) ;
#82830=STYLED_ITEM('',(#170171),#88538) ;
#82831=STYLED_ITEM('',(#170171),#88539) ;
#82832=STYLED_ITEM('',(#170171),#88540) ;
#82833=STYLED_ITEM('',(#170171),#88541) ;
#82834=STYLED_ITEM('',(#170171),#88542) ;
#82835=STYLED_ITEM('',(#170171),#88543) ;
#82836=STYLED_ITEM('',(#170171),#88544) ;
#82837=STYLED_ITEM('',(#170171),#88545) ;
#82838=STYLED_ITEM('',(#170171),#88546) ;
#82839=STYLED_ITEM('',(#170171),#88547) ;
#82840=STYLED_ITEM('',(#170171),#88548) ;
#82841=STYLED_ITEM('',(#170171),#88549) ;
#82842=STYLED_ITEM('',(#170171),#88550) ;
#82843=STYLED_ITEM('',(#170171),#88551) ;
#82844=STYLED_ITEM('',(#170171),#88552) ;
#82845=STYLED_ITEM('',(#170171),#88553) ;
#82846=STYLED_ITEM('',(#170171),#88554) ;
#82847=STYLED_ITEM('',(#170171),#88555) ;
#82848=STYLED_ITEM('',(#170171),#88556) ;
#82849=STYLED_ITEM('',(#170171),#88557) ;
#82850=STYLED_ITEM('',(#170171),#88558) ;
#82851=STYLED_ITEM('',(#170171),#88559) ;
#82852=STYLED_ITEM('',(#170171),#88560) ;
#82853=STYLED_ITEM('',(#170171),#88561) ;
#82854=STYLED_ITEM('',(#170171),#88562) ;
#82855=STYLED_ITEM('',(#170171),#88563) ;
#82856=STYLED_ITEM('',(#170171),#88564) ;
#82857=STYLED_ITEM('',(#170171),#88565) ;
#82858=STYLED_ITEM('',(#170171),#88566) ;
#82859=STYLED_ITEM('',(#170171),#88567) ;
#82860=STYLED_ITEM('',(#170171),#88568) ;
#82861=STYLED_ITEM('',(#170171),#88569) ;
#82862=STYLED_ITEM('',(#170171),#88570) ;
#82863=STYLED_ITEM('',(#170171),#88571) ;
#82864=STYLED_ITEM('',(#170171),#88572) ;
#82865=STYLED_ITEM('',(#170171),#88573) ;
#82866=STYLED_ITEM('',(#170171),#88574) ;
#82867=STYLED_ITEM('',(#170171),#88575) ;
#82868=STYLED_ITEM('',(#170171),#88576) ;
#82869=STYLED_ITEM('',(#170171),#88577) ;
#82870=STYLED_ITEM('',(#170171),#88578) ;
#82871=STYLED_ITEM('',(#170171),#88579) ;
#82872=STYLED_ITEM('',(#170171),#88580) ;
#82873=STYLED_ITEM('',(#170171),#88581) ;
#82874=STYLED_ITEM('',(#170171),#88582) ;
#82875=STYLED_ITEM('',(#170171),#88583) ;
#82876=STYLED_ITEM('',(#170171),#88584) ;
#82877=STYLED_ITEM('',(#170171),#88585) ;
#82878=STYLED_ITEM('',(#170171),#88586) ;
#82879=STYLED_ITEM('',(#170171),#88587) ;
#82880=STYLED_ITEM('',(#170171),#88588) ;
#82881=STYLED_ITEM('',(#170171),#88589) ;
#82882=STYLED_ITEM('',(#170171),#88590) ;
#82883=STYLED_ITEM('',(#170171),#88591) ;
#82884=STYLED_ITEM('',(#170171),#88592) ;
#82885=STYLED_ITEM('',(#170171),#88593) ;
#82886=STYLED_ITEM('',(#170171),#88594) ;
#82887=STYLED_ITEM('',(#170171),#88595) ;
#82888=STYLED_ITEM('',(#170171),#88596) ;
#82889=STYLED_ITEM('',(#170171),#88597) ;
#82890=STYLED_ITEM('',(#170171),#88598) ;
#82891=STYLED_ITEM('',(#170171),#88599) ;
#82892=STYLED_ITEM('',(#170171),#88600) ;
#82893=STYLED_ITEM('',(#170171),#88601) ;
#82894=STYLED_ITEM('',(#170171),#88602) ;
#82895=STYLED_ITEM('',(#170171),#88603) ;
#82896=STYLED_ITEM('',(#170171),#88604) ;
#82897=STYLED_ITEM('',(#170171),#88605) ;
#82898=STYLED_ITEM('',(#170171),#88606) ;
#82899=STYLED_ITEM('',(#170171),#88607) ;
#82900=STYLED_ITEM('',(#170171),#88608) ;
#82901=STYLED_ITEM('',(#170171),#88609) ;
#82902=STYLED_ITEM('',(#170171),#88610) ;
#82903=STYLED_ITEM('',(#170171),#88611) ;
#82904=STYLED_ITEM('',(#170171),#88612) ;
#82905=STYLED_ITEM('',(#170171),#88613) ;
#82906=STYLED_ITEM('',(#170171),#88614) ;
#82907=STYLED_ITEM('',(#170171),#88615) ;
#82908=STYLED_ITEM('',(#170171),#88616) ;
#82909=STYLED_ITEM('',(#170171),#88617) ;
#82910=STYLED_ITEM('',(#170171),#88618) ;
#82911=STYLED_ITEM('',(#170171),#88619) ;
#82912=STYLED_ITEM('',(#170171),#88620) ;
#82913=STYLED_ITEM('',(#170171),#88621) ;
#82914=STYLED_ITEM('',(#170171),#88622) ;
#82915=STYLED_ITEM('',(#170171),#88623) ;
#82916=STYLED_ITEM('',(#170171),#88624) ;
#82917=STYLED_ITEM('',(#170171),#88625) ;
#82918=STYLED_ITEM('',(#170171),#88626) ;
#82919=STYLED_ITEM('',(#170171),#88627) ;
#82920=STYLED_ITEM('',(#170171),#88628) ;
#82921=STYLED_ITEM('',(#170171),#88629) ;
#82922=STYLED_ITEM('',(#170171),#88630) ;
#82923=STYLED_ITEM('',(#170171),#88631) ;
#82924=STYLED_ITEM('',(#170171),#88632) ;
#82925=STYLED_ITEM('',(#170171),#88633) ;
#82926=STYLED_ITEM('',(#170171),#88634) ;
#82927=STYLED_ITEM('',(#170171),#88635) ;
#82928=STYLED_ITEM('',(#170171),#88636) ;
#82929=STYLED_ITEM('',(#170171),#88637) ;
#82930=STYLED_ITEM('',(#170171),#88638) ;
#82931=STYLED_ITEM('',(#170171),#88639) ;
#82932=STYLED_ITEM('',(#170171),#88640) ;
#82933=STYLED_ITEM('',(#170171),#88641) ;
#82934=STYLED_ITEM('',(#170171),#88642) ;
#82935=STYLED_ITEM('',(#170171),#88643) ;
#82936=STYLED_ITEM('',(#170171),#88644) ;
#82937=STYLED_ITEM('',(#170171),#88645) ;
#82938=STYLED_ITEM('',(#170171),#88646) ;
#82939=STYLED_ITEM('',(#170171),#88647) ;
#82940=STYLED_ITEM('',(#170171),#88648) ;
#82941=STYLED_ITEM('',(#170171),#88649) ;
#82942=STYLED_ITEM('',(#170171),#88650) ;
#82943=STYLED_ITEM('',(#170171),#88651) ;
#82944=STYLED_ITEM('',(#170171),#88652) ;
#82945=STYLED_ITEM('',(#170171),#88653) ;
#82946=STYLED_ITEM('',(#170171),#88654) ;
#82947=STYLED_ITEM('',(#170171),#88655) ;
#82948=STYLED_ITEM('',(#170171),#88656) ;
#82949=STYLED_ITEM('',(#170171),#88657) ;
#82950=STYLED_ITEM('',(#170171),#88658) ;
#82951=STYLED_ITEM('',(#170171),#88659) ;
#82952=STYLED_ITEM('',(#170171),#88660) ;
#82953=STYLED_ITEM('',(#170171),#88661) ;
#82954=STYLED_ITEM('',(#170171),#88662) ;
#82955=STYLED_ITEM('',(#170171),#88663) ;
#82956=STYLED_ITEM('',(#170171),#88664) ;
#82957=STYLED_ITEM('',(#170171),#88665) ;
#82958=STYLED_ITEM('',(#170171),#88666) ;
#82959=STYLED_ITEM('',(#170171),#88667) ;
#82960=STYLED_ITEM('',(#170171),#88668) ;
#82961=STYLED_ITEM('',(#170171),#88669) ;
#82962=STYLED_ITEM('',(#170171),#88670) ;
#82963=STYLED_ITEM('',(#170171),#88671) ;
#82964=STYLED_ITEM('',(#170171),#88672) ;
#82965=STYLED_ITEM('',(#170171),#88673) ;
#82966=STYLED_ITEM('',(#170171),#88674) ;
#82967=STYLED_ITEM('',(#170171),#88675) ;
#82968=STYLED_ITEM('',(#170171),#88676) ;
#82969=STYLED_ITEM('',(#170171),#88677) ;
#82970=STYLED_ITEM('',(#170171),#88678) ;
#82971=STYLED_ITEM('',(#170171),#88679) ;
#82972=STYLED_ITEM('',(#170171),#88680) ;
#82973=STYLED_ITEM('',(#170171),#88681) ;
#82974=STYLED_ITEM('',(#170171),#88682) ;
#82975=STYLED_ITEM('',(#170171),#88683) ;
#82976=STYLED_ITEM('',(#170171),#88684) ;
#82977=STYLED_ITEM('',(#170171),#88685) ;
#82978=STYLED_ITEM('',(#170171),#88686) ;
#82979=STYLED_ITEM('',(#170171),#88687) ;
#82980=STYLED_ITEM('',(#170171),#88688) ;
#82981=STYLED_ITEM('',(#170171),#88689) ;
#82982=STYLED_ITEM('',(#170171),#88690) ;
#82983=STYLED_ITEM('',(#170171),#88691) ;
#82984=STYLED_ITEM('',(#170171),#88692) ;
#82985=STYLED_ITEM('',(#170171),#88693) ;
#82986=STYLED_ITEM('',(#170171),#88694) ;
#82987=STYLED_ITEM('',(#170171),#88695) ;
#82988=STYLED_ITEM('',(#170171),#88696) ;
#82989=STYLED_ITEM('',(#170171),#88697) ;
#82990=STYLED_ITEM('',(#170171),#88698) ;
#82991=STYLED_ITEM('',(#170171),#88699) ;
#82992=STYLED_ITEM('',(#170171),#88700) ;
#82993=STYLED_ITEM('',(#170171),#88701) ;
#82994=STYLED_ITEM('',(#170171),#88702) ;
#82995=STYLED_ITEM('',(#170171),#88703) ;
#82996=STYLED_ITEM('',(#170171),#88704) ;
#82997=STYLED_ITEM('',(#170171),#88705) ;
#82998=STYLED_ITEM('',(#170171),#88706) ;
#82999=STYLED_ITEM('',(#170171),#88707) ;
#83000=STYLED_ITEM('',(#170171),#88708) ;
#83001=STYLED_ITEM('',(#170171),#88709) ;
#83002=STYLED_ITEM('',(#170171),#88710) ;
#83003=STYLED_ITEM('',(#170171),#88711) ;
#83004=STYLED_ITEM('',(#170171),#88712) ;
#83005=STYLED_ITEM('',(#170171),#88713) ;
#83006=STYLED_ITEM('',(#170171),#88714) ;
#83007=STYLED_ITEM('',(#170171),#88715) ;
#83008=STYLED_ITEM('',(#170171),#88716) ;
#83009=STYLED_ITEM('',(#170171),#88717) ;
#83010=STYLED_ITEM('',(#170168),#32) ;
#86488=ADVANCED_FACE('',(#18168),#79020,.T.) ;
#86489=ADVANCED_FACE('',(#18169),#79021,.F.) ;
#86490=ADVANCED_FACE('',(#18170),#16277,.F.) ;
#86491=ADVANCED_FACE('',(#18171),#14036,.F.) ;
#86492=ADVANCED_FACE('',(#18172),#79022,.T.) ;
#86493=ADVANCED_FACE('',(#18173),#79023,.F.) ;
#86494=ADVANCED_FACE('',(#18174),#16278,.F.) ;
#86495=ADVANCED_FACE('',(#18175),#14037,.F.) ;
#86496=ADVANCED_FACE('',(#18176),#79024,.T.) ;
#86497=ADVANCED_FACE('',(#18177),#79025,.F.) ;
#86498=ADVANCED_FACE('',(#18178),#16279,.F.) ;
#86499=ADVANCED_FACE('',(#18179),#14038,.F.) ;
#86500=ADVANCED_FACE('',(#18180),#79026,.T.) ;
#86501=ADVANCED_FACE('',(#18181),#79027,.F.) ;
#86502=ADVANCED_FACE('',(#18182),#16280,.F.) ;
#86503=ADVANCED_FACE('',(#18183),#14039,.F.) ;
#86504=ADVANCED_FACE('',(#18184),#79028,.T.) ;
#86505=ADVANCED_FACE('',(#18185),#79029,.F.) ;
#86506=ADVANCED_FACE('',(#18186),#16281,.F.) ;
#86507=ADVANCED_FACE('',(#18187),#14040,.F.) ;
#86508=ADVANCED_FACE('',(#18188),#79030,.T.) ;
#86509=ADVANCED_FACE('',(#18189),#79031,.F.) ;
#86510=ADVANCED_FACE('',(#18190),#16282,.F.) ;
#86511=ADVANCED_FACE('',(#18191),#14041,.F.) ;
#86512=ADVANCED_FACE('',(#18192),#79032,.T.) ;
#86513=ADVANCED_FACE('',(#18193),#79033,.F.) ;
#86514=ADVANCED_FACE('',(#18194),#16283,.F.) ;
#86515=ADVANCED_FACE('',(#18195),#14042,.F.) ;
#86516=ADVANCED_FACE('',(#18196),#79034,.T.) ;
#86517=ADVANCED_FACE('',(#18197),#79035,.F.) ;
#86518=ADVANCED_FACE('',(#18198),#16284,.F.) ;
#86519=ADVANCED_FACE('',(#18199),#14043,.F.) ;
#86520=ADVANCED_FACE('',(#18200),#79036,.T.) ;
#86521=ADVANCED_FACE('',(#18201),#79037,.T.) ;
#86522=ADVANCED_FACE('',(#18202),#79038,.T.) ;
#86523=ADVANCED_FACE('',(#18203),#79039,.T.) ;
#86524=ADVANCED_FACE('',(#18204),#79040,.T.) ;
#86525=ADVANCED_FACE('',(#18205),#79041,.T.) ;
#86526=ADVANCED_FACE('',(#18206),#79042,.T.) ;
#86527=ADVANCED_FACE('',(#18207),#79043,.T.) ;
#86528=ADVANCED_FACE('',(#18208),#79044,.T.) ;
#86529=ADVANCED_FACE('',(#18209),#79045,.T.) ;
#86530=ADVANCED_FACE('',(#18210),#79046,.F.) ;
#86531=ADVANCED_FACE('',(#18211),#16285,.F.) ;
#86532=ADVANCED_FACE('',(#18212),#14044,.F.) ;
#86533=ADVANCED_FACE('',(#18213),#14045,.T.) ;
#86534=ADVANCED_FACE('',(#18214),#14046,.T.) ;
#86535=ADVANCED_FACE('',(#18215),#14047,.T.) ;
#86536=ADVANCED_FACE('',(#18216),#14048,.T.) ;
#86537=ADVANCED_FACE('',(#18217),#14049,.T.) ;
#86538=ADVANCED_FACE('',(#18218),#14050,.T.) ;
#86539=ADVANCED_FACE('',(#18219),#14051,.T.) ;
#86540=ADVANCED_FACE('',(#18220),#14052,.T.) ;
#86541=ADVANCED_FACE('',(#18221),#14053,.T.) ;
#86542=ADVANCED_FACE('',(#18222),#14054,.F.) ;
#86543=ADVANCED_FACE('',(#18223),#14055,.F.) ;
#86544=ADVANCED_FACE('',(#18224),#14056,.F.) ;
#86545=ADVANCED_FACE('',(#18225),#14057,.F.) ;
#86546=ADVANCED_FACE('',(#18226),#14058,.F.) ;
#86547=ADVANCED_FACE('',(#18227),#14059,.F.) ;
#86548=ADVANCED_FACE('',(#18228),#14060,.F.) ;
#86549=ADVANCED_FACE('',(#18229),#14061,.F.) ;
#86550=ADVANCED_FACE('',(#18230),#14062,.F.) ;
#86551=ADVANCED_FACE('',(#18231),#79047,.T.) ;
#86552=ADVANCED_FACE('',(#18232),#79048,.T.) ;
#86553=ADVANCED_FACE('',(#18233),#79049,.F.) ;
#86554=ADVANCED_FACE('',(#18234),#16286,.F.) ;
#86555=ADVANCED_FACE('',(#18235),#14063,.F.) ;
#86556=ADVANCED_FACE('',(#18236),#14064,.T.) ;
#86557=ADVANCED_FACE('',(#18237),#14065,.F.) ;
#86558=ADVANCED_FACE('',(#18238),#1083,.T.) ;
#86559=ADVANCED_FACE('',(#18239),#1084,.T.) ;
#86560=ADVANCED_FACE('',(#18240),#1085,.T.) ;
#86561=ADVANCED_FACE('',(#18241),#1086,.T.) ;
#86562=ADVANCED_FACE('',(#18242),#1087,.T.) ;
#86563=ADVANCED_FACE('',(#18243),#1088,.T.) ;
#86564=ADVANCED_FACE('',(#18244),#1089,.T.) ;
#86565=ADVANCED_FACE('',(#18245),#1090,.T.) ;
#86566=ADVANCED_FACE('',(#18246),#1091,.T.) ;
#86567=ADVANCED_FACE('',(#18247),#1092,.F.) ;
#86568=ADVANCED_FACE('',(#18248),#1093,.F.) ;
#86569=ADVANCED_FACE('',(#18249),#1094,.F.) ;
#86570=ADVANCED_FACE('',(#18250),#1095,.F.) ;
#86571=ADVANCED_FACE('',(#18251),#1096,.F.) ;
#86572=ADVANCED_FACE('',(#18252),#1097,.F.) ;
#86573=ADVANCED_FACE('',(#18253),#1098,.F.) ;
#86574=ADVANCED_FACE('',(#18254),#1099,.F.) ;
#86575=ADVANCED_FACE('',(#18255),#1100,.F.) ;
#86576=ADVANCED_FACE('',(#18256),#1101,.F.) ;
#86577=ADVANCED_FACE('',(#18257),#1102,.F.) ;
#86578=ADVANCED_FACE('',(#18258),#1103,.F.) ;
#86579=ADVANCED_FACE('',(#18259),#1104,.F.) ;
#86580=ADVANCED_FACE('',(#18260),#1105,.F.) ;
#86581=ADVANCED_FACE('',(#18261),#1106,.F.) ;
#86582=ADVANCED_FACE('',(#18262),#1107,.F.) ;
#86583=ADVANCED_FACE('',(#18263),#1108,.F.) ;
#86584=ADVANCED_FACE('',(#18264),#1109,.F.) ;
#86585=ADVANCED_FACE('',(#18265),#14066,.T.) ;
#86586=ADVANCED_FACE('',(#18266),#14067,.T.) ;
#86587=ADVANCED_FACE('',(#18267),#14068,.T.) ;
#86588=ADVANCED_FACE('',(#18268),#14069,.T.) ;
#86589=ADVANCED_FACE('',(#18269),#14070,.T.) ;
#86590=ADVANCED_FACE('',(#18270),#14071,.T.) ;
#86591=ADVANCED_FACE('',(#18271),#14072,.T.) ;
#86592=ADVANCED_FACE('',(#18272),#14073,.T.) ;
#86593=ADVANCED_FACE('',(#18273),#14074,.T.) ;
#86594=ADVANCED_FACE('',(#18274),#1110,.T.) ;
#86595=ADVANCED_FACE('',(#18275),#1111,.F.) ;
#86596=ADVANCED_FACE('',(#18276),#1112,.F.) ;
#86597=ADVANCED_FACE('',(#18277),#14075,.T.) ;
#86598=ADVANCED_FACE('',(#18278),#14076,.T.) ;
#86599=ADVANCED_FACE('',(#18279),#1113,.T.) ;
#86600=ADVANCED_FACE('',(#18280),#14077,.T.) ;
#86601=ADVANCED_FACE('',(#18281),#1114,.T.) ;
#86602=ADVANCED_FACE('',(#18282),#14078,.T.) ;
#86603=ADVANCED_FACE('',(#18283),#1115,.T.) ;
#86604=ADVANCED_FACE('',(#18284),#14079,.F.) ;
#86605=ADVANCED_FACE('',(#18285),#1116,.T.) ;
#86606=ADVANCED_FACE('',(#18286),#14080,.T.) ;
#86607=ADVANCED_FACE('',(#18287),#1117,.T.) ;
#86608=ADVANCED_FACE('',(#18288),#14081,.T.) ;
#86609=ADVANCED_FACE('',(#18289),#1118,.T.) ;
#86610=ADVANCED_FACE('',(#18290),#14082,.F.) ;
#86611=ADVANCED_FACE('',(#18291),#1119,.T.) ;
#86612=ADVANCED_FACE('',(#18292),#14083,.T.) ;
#86613=ADVANCED_FACE('',(#18293,#684,#685,#686,#687,#688,#689,#690,#691,
#692,#693),#1120,.T.) ;
#86614=ADVANCED_FACE('',(#18294),#1121,.F.) ;
#86615=ADVANCED_FACE('',(#18295),#1122,.T.) ;
#86616=ADVANCED_FACE('',(#18296),#1123,.T.) ;
#86617=ADVANCED_FACE('',(#18297),#1124,.F.) ;
#86618=ADVANCED_FACE('',(#18298),#1125,.F.) ;
#86619=ADVANCED_FACE('',(#18299),#1126,.F.) ;
#86620=ADVANCED_FACE('',(#18300),#1127,.F.) ;
#86621=ADVANCED_FACE('',(#18301),#1128,.F.) ;
#86622=ADVANCED_FACE('',(#18302),#14084,.T.) ;
#86623=ADVANCED_FACE('',(#18303),#1129,.F.) ;
#86624=ADVANCED_FACE('',(#18304),#14085,.T.) ;
#86625=ADVANCED_FACE('',(#18305),#1130,.F.) ;
#86626=ADVANCED_FACE('',(#18306),#14086,.F.) ;
#86627=ADVANCED_FACE('',(#18307),#1131,.F.) ;
#86628=ADVANCED_FACE('',(#18308),#14087,.F.) ;
#86629=ADVANCED_FACE('',(#18309),#1132,.F.) ;
#86630=ADVANCED_FACE('',(#18310),#1133,.F.) ;
#86631=ADVANCED_FACE('',(#18311),#14088,.F.) ;
#86632=ADVANCED_FACE('',(#18312),#1134,.F.) ;
#86633=ADVANCED_FACE('',(#18313),#14089,.T.) ;
#86634=ADVANCED_FACE('',(#18314),#1135,.F.) ;
#86635=ADVANCED_FACE('',(#18315),#14090,.T.) ;
#86636=ADVANCED_FACE('',(#18316),#1136,.F.) ;
#86637=ADVANCED_FACE('',(#18317),#14091,.F.) ;
#86638=ADVANCED_FACE('',(#18318),#1137,.F.) ;
#86639=ADVANCED_FACE('',(#18319),#14092,.F.) ;
#86640=ADVANCED_FACE('',(#18320),#1138,.F.) ;
#86641=ADVANCED_FACE('',(#18321),#14093,.F.) ;
#86642=ADVANCED_FACE('',(#18322),#14094,.T.) ;
#86643=ADVANCED_FACE('',(#18323),#14095,.F.) ;
#86644=ADVANCED_FACE('',(#18324),#1139,.F.) ;
#86645=ADVANCED_FACE('',(#18325),#14096,.F.) ;
#86646=ADVANCED_FACE('',(#18326),#1140,.F.) ;
#86647=ADVANCED_FACE('',(#18327),#14097,.F.) ;
#86648=ADVANCED_FACE('',(#18328),#1141,.F.) ;
#86649=ADVANCED_FACE('',(#18329,#694),#1142,.F.) ;
#86650=ADVANCED_FACE('',(#18330,#695),#1143,.T.) ;
#86651=ADVANCED_FACE('',(#18331),#14098,.T.) ;
#86652=ADVANCED_FACE('',(#18332),#14099,.F.) ;
#86653=ADVANCED_FACE('',(#18333),#16287,.F.) ;
#86654=ADVANCED_FACE('',(#18334),#16288,.T.) ;
#86655=ADVANCED_FACE('',(#18335),#79050,.T.) ;
#86656=ADVANCED_FACE('',(#18336),#14100,.F.) ;
#86657=ADVANCED_FACE('',(#18337),#14101,.F.) ;
#86658=ADVANCED_FACE('',(#18338),#14102,.T.) ;
#86659=ADVANCED_FACE('',(#18339),#14103,.T.) ;
#86660=ADVANCED_FACE('',(#18340),#14104,.T.) ;
#86661=ADVANCED_FACE('',(#18341),#14105,.F.) ;
#86662=ADVANCED_FACE('',(#18342),#16289,.F.) ;
#86663=ADVANCED_FACE('',(#18343),#79051,.F.) ;
#86664=ADVANCED_FACE('',(#18344),#79052,.F.) ;
#86665=ADVANCED_FACE('',(#18345),#79053,.T.) ;
#86666=ADVANCED_FACE('',(#18346),#14106,.F.) ;
#86667=ADVANCED_FACE('',(#18347),#14107,.F.) ;
#86668=ADVANCED_FACE('',(#18348),#14108,.F.) ;
#86669=ADVANCED_FACE('',(#18349),#14109,.T.) ;
#86670=ADVANCED_FACE('',(#18350),#14110,.T.) ;
#86671=ADVANCED_FACE('',(#18351),#79054,.F.) ;
#86672=ADVANCED_FACE('',(#18352),#16290,.F.) ;
#86673=ADVANCED_FACE('',(#18353),#16291,.T.) ;
#86674=ADVANCED_FACE('',(#18354),#14111,.T.) ;
#86675=ADVANCED_FACE('',(#18355),#16292,.F.) ;
#86676=ADVANCED_FACE('',(#18356),#16293,.T.) ;
#86677=ADVANCED_FACE('',(#18357),#14112,.F.) ;
#86678=ADVANCED_FACE('',(#18358),#14113,.F.) ;
#86679=ADVANCED_FACE('',(#18359),#14114,.T.) ;
#86680=ADVANCED_FACE('',(#18360),#79055,.T.) ;
#86681=ADVANCED_FACE('',(#18361),#14115,.F.) ;
#86682=ADVANCED_FACE('',(#18362),#14116,.T.) ;
#86683=ADVANCED_FACE('',(#18363),#14117,.F.) ;
#86684=ADVANCED_FACE('',(#18364),#16294,.F.) ;
#86685=ADVANCED_FACE('',(#18365),#79056,.T.) ;
#86686=ADVANCED_FACE('',(#18366),#14118,.T.) ;
#86687=ADVANCED_FACE('',(#18367),#16295,.F.) ;
#86688=ADVANCED_FACE('',(#18368),#79057,.F.) ;
#86689=ADVANCED_FACE('',(#18369),#14119,.F.) ;
#86690=ADVANCED_FACE('',(#18370),#14120,.T.) ;
#86691=ADVANCED_FACE('',(#18371),#79058,.T.) ;
#86692=ADVANCED_FACE('',(#18372),#14121,.F.) ;
#86693=ADVANCED_FACE('',(#18373),#79059,.T.) ;
#86694=ADVANCED_FACE('',(#18374),#14122,.T.) ;
#86695=ADVANCED_FACE('',(#18375),#14123,.T.) ;
#86696=ADVANCED_FACE('',(#18376),#16296,.T.) ;
#86697=ADVANCED_FACE('',(#18377),#16297,.T.) ;
#86698=ADVANCED_FACE('',(#18378),#14124,.T.) ;
#86699=ADVANCED_FACE('',(#18379),#14125,.T.) ;
#86700=ADVANCED_FACE('',(#18380),#79060,.T.) ;
#86701=ADVANCED_FACE('',(#18381),#16298,.T.) ;
#86702=ADVANCED_FACE('',(#18382),#14126,.T.) ;
#86703=ADVANCED_FACE('',(#18383),#14127,.T.) ;
#86704=ADVANCED_FACE('',(#18384),#16299,.T.) ;
#86705=ADVANCED_FACE('',(#18385),#79061,.T.) ;
#86706=ADVANCED_FACE('',(#18386),#14128,.T.) ;
#86707=ADVANCED_FACE('',(#18387),#14129,.T.) ;
#86708=ADVANCED_FACE('',(#18388),#16300,.T.) ;
#86709=ADVANCED_FACE('',(#18389),#16301,.T.) ;
#86710=ADVANCED_FACE('',(#18390),#14130,.T.) ;
#86711=ADVANCED_FACE('',(#18391),#14131,.T.) ;
#86712=ADVANCED_FACE('',(#18392),#16302,.T.) ;
#86713=ADVANCED_FACE('',(#18393),#16303,.T.) ;
#86714=ADVANCED_FACE('',(#18394),#14132,.T.) ;
#86715=ADVANCED_FACE('',(#18395),#14133,.T.) ;
#86716=ADVANCED_FACE('',(#18396),#79062,.T.) ;
#86717=ADVANCED_FACE('',(#18397),#16304,.T.) ;
#86718=ADVANCED_FACE('',(#18398),#14134,.T.) ;
#86719=ADVANCED_FACE('',(#18399),#14135,.T.) ;
#86720=ADVANCED_FACE('',(#18400),#16305,.T.) ;
#86721=ADVANCED_FACE('',(#18401),#79063,.T.) ;
#86722=ADVANCED_FACE('',(#18402),#14136,.T.) ;
#86723=ADVANCED_FACE('',(#18403),#14137,.T.) ;
#86724=ADVANCED_FACE('',(#18404),#16306,.T.) ;
#86725=ADVANCED_FACE('',(#18405),#16307,.T.) ;
#86726=ADVANCED_FACE('',(#18406),#14138,.T.) ;
#86727=ADVANCED_FACE('',(#18407),#14139,.T.) ;
#86728=ADVANCED_FACE('',(#18408),#16308,.T.) ;
#86729=ADVANCED_FACE('',(#18409),#14140,.F.) ;
#86730=ADVANCED_FACE('',(#18410),#79064,.F.) ;
#86731=ADVANCED_FACE('',(#18411),#16309,.F.) ;
#86732=ADVANCED_FACE('',(#18412),#14141,.F.) ;
#86733=ADVANCED_FACE('',(#18413),#14142,.F.) ;
#86734=ADVANCED_FACE('',(#18414),#79065,.F.) ;
#86735=ADVANCED_FACE('',(#18415),#16310,.F.) ;
#86736=ADVANCED_FACE('',(#18416),#14143,.F.) ;
#86737=ADVANCED_FACE('',(#18417),#14144,.F.) ;
#86738=ADVANCED_FACE('',(#18418),#16311,.F.) ;
#86739=ADVANCED_FACE('',(#18419),#16312,.F.) ;
#86740=ADVANCED_FACE('',(#18420),#14145,.F.) ;
#86741=ADVANCED_FACE('',(#18421),#79066,.F.) ;
#86742=ADVANCED_FACE('',(#18422),#16313,.F.) ;
#86743=ADVANCED_FACE('',(#18423),#16314,.F.) ;
#86744=ADVANCED_FACE('',(#18424),#14146,.F.) ;
#86745=ADVANCED_FACE('',(#18425),#14147,.F.) ;
#86746=ADVANCED_FACE('',(#18426),#16315,.F.) ;
#86747=ADVANCED_FACE('',(#18427),#14148,.F.) ;
#86748=ADVANCED_FACE('',(#18428),#14149,.F.) ;
#86749=ADVANCED_FACE('',(#18429),#16316,.F.) ;
#86750=ADVANCED_FACE('',(#18430),#16317,.F.) ;
#86751=ADVANCED_FACE('',(#18431),#14150,.F.) ;
#86752=ADVANCED_FACE('',(#18432),#14151,.F.) ;
#86753=ADVANCED_FACE('',(#18433),#79067,.F.) ;
#86754=ADVANCED_FACE('',(#18434),#79068,.F.) ;
#86755=ADVANCED_FACE('',(#18435),#14152,.F.) ;
#86756=ADVANCED_FACE('',(#18436),#14153,.T.) ;
#86757=ADVANCED_FACE('',(#18437),#16318,.T.) ;
#86758=ADVANCED_FACE('',(#18438),#16319,.T.) ;
#86759=ADVANCED_FACE('',(#18439),#14154,.T.) ;
#86760=ADVANCED_FACE('',(#18440),#14155,.T.) ;
#86761=ADVANCED_FACE('',(#18441),#79069,.T.) ;
#86762=ADVANCED_FACE('',(#18442),#79070,.T.) ;
#86763=ADVANCED_FACE('',(#18443),#14156,.T.) ;
#86764=ADVANCED_FACE('',(#18444),#14157,.T.) ;
#86765=ADVANCED_FACE('',(#18445),#79071,.T.) ;
#86766=ADVANCED_FACE('',(#18446),#14158,.T.) ;
#86767=ADVANCED_FACE('',(#18447),#14159,.T.) ;
#86768=ADVANCED_FACE('',(#18448),#79072,.T.) ;
#86769=ADVANCED_FACE('',(#18449),#79073,.T.) ;
#86770=ADVANCED_FACE('',(#18450),#14160,.T.) ;
#86771=ADVANCED_FACE('',(#18451),#79074,.T.) ;
#86772=ADVANCED_FACE('',(#18452),#79075,.T.) ;
#86773=ADVANCED_FACE('',(#18453),#79076,.T.) ;
#86774=ADVANCED_FACE('',(#18454),#14161,.T.) ;
#86775=ADVANCED_FACE('',(#18455),#14162,.T.) ;
#86776=ADVANCED_FACE('',(#18456),#16320,.T.) ;
#86777=ADVANCED_FACE('',(#18457),#79077,.T.) ;
#86778=ADVANCED_FACE('',(#18458),#14163,.T.) ;
#86779=ADVANCED_FACE('',(#18459),#14164,.T.) ;
#86780=ADVANCED_FACE('',(#18460),#16321,.T.) ;
#86781=ADVANCED_FACE('',(#18461),#79078,.T.) ;
#86782=ADVANCED_FACE('',(#18462),#14165,.T.) ;
#86783=ADVANCED_FACE('',(#18463),#1144,.F.) ;
#86784=ADVANCED_FACE('',(#18464),#1145,.F.) ;
#86785=ADVANCED_FACE('',(#18465),#1146,.F.) ;
#86786=ADVANCED_FACE('',(#18466),#1147,.F.) ;
#86787=ADVANCED_FACE('',(#18467),#1148,.F.) ;
#86788=ADVANCED_FACE('',(#18468),#1149,.T.) ;
#86789=ADVANCED_FACE('',(#18469),#1150,.F.) ;
#86790=ADVANCED_FACE('',(#18470),#14166,.T.) ;
#86791=ADVANCED_FACE('',(#18471),#14167,.F.) ;
#86792=ADVANCED_FACE('',(#18472),#1151,.F.) ;
#86793=ADVANCED_FACE('',(#18473),#1152,.F.) ;
#86794=ADVANCED_FACE('',(#18474),#1153,.F.) ;
#86795=ADVANCED_FACE('',(#18475),#1154,.F.) ;
#86796=ADVANCED_FACE('',(#18476),#1155,.F.) ;
#86797=ADVANCED_FACE('',(#18477),#1156,.T.) ;
#86798=ADVANCED_FACE('',(#18478),#1157,.F.) ;
#86799=ADVANCED_FACE('',(#18479),#1158,.F.) ;
#86800=ADVANCED_FACE('',(#18480),#1159,.F.) ;
#86801=ADVANCED_FACE('',(#18481),#1160,.F.) ;
#86802=ADVANCED_FACE('',(#18482),#1161,.F.) ;
#86803=ADVANCED_FACE('',(#18483),#14168,.T.) ;
#86804=ADVANCED_FACE('',(#18484),#14169,.T.) ;
#86805=ADVANCED_FACE('',(#18485),#16322,.T.) ;
#86806=ADVANCED_FACE('',(#18486),#14170,.T.) ;
#86807=ADVANCED_FACE('',(#18487),#14171,.T.) ;
#86808=ADVANCED_FACE('',(#18488),#14172,.T.) ;
#86809=ADVANCED_FACE('',(#18489),#16323,.T.) ;
#86810=ADVANCED_FACE('',(#18490),#16324,.T.) ;
#86811=ADVANCED_FACE('',(#18491),#14173,.T.) ;
#86812=ADVANCED_FACE('',(#18492),#14174,.T.) ;
#86813=ADVANCED_FACE('',(#18493),#14175,.T.) ;
#86814=ADVANCED_FACE('',(#18494),#16325,.T.) ;
#86815=ADVANCED_FACE('',(#18495),#14176,.T.) ;
#86816=ADVANCED_FACE('',(#18496),#14177,.T.) ;
#86817=ADVANCED_FACE('',(#18497),#14178,.T.) ;
#86818=ADVANCED_FACE('',(#18498),#14179,.T.) ;
#86819=ADVANCED_FACE('',(#18499),#16326,.T.) ;
#86820=ADVANCED_FACE('',(#18500),#14180,.T.) ;
#86821=ADVANCED_FACE('',(#18501),#14181,.T.) ;
#86822=ADVANCED_FACE('',(#18502),#14182,.T.) ;
#86823=ADVANCED_FACE('',(#18503),#16327,.T.) ;
#86824=ADVANCED_FACE('',(#18504),#16328,.T.) ;
#86825=ADVANCED_FACE('',(#18505),#14183,.T.) ;
#86826=ADVANCED_FACE('',(#18506),#14184,.T.) ;
#86827=ADVANCED_FACE('',(#18507),#14185,.T.) ;
#86828=ADVANCED_FACE('',(#18508),#16329,.T.) ;
#86829=ADVANCED_FACE('',(#18509),#14186,.T.) ;
#86830=ADVANCED_FACE('',(#18510),#14187,.T.) ;
#86831=ADVANCED_FACE('',(#18511),#79079,.T.) ;
#86832=ADVANCED_FACE('',(#18512),#14188,.T.) ;
#86833=ADVANCED_FACE('',(#18513),#16330,.T.) ;
#86834=ADVANCED_FACE('',(#18514),#14189,.T.) ;
#86835=ADVANCED_FACE('',(#18515),#16331,.T.) ;
#86836=ADVANCED_FACE('',(#18516),#14190,.T.) ;
#86837=ADVANCED_FACE('',(#18517),#79080,.T.) ;
#86838=ADVANCED_FACE('',(#18518),#79081,.T.) ;
#86839=ADVANCED_FACE('',(#18519),#14191,.T.) ;
#86840=ADVANCED_FACE('',(#18520),#16332,.T.) ;
#86841=ADVANCED_FACE('',(#18521),#14192,.T.) ;
#86842=ADVANCED_FACE('',(#18522),#16333,.T.) ;
#86843=ADVANCED_FACE('',(#18523),#14193,.T.) ;
#86844=ADVANCED_FACE('',(#18524),#79082,.T.) ;
#86845=ADVANCED_FACE('',(#18525),#14194,.T.) ;
#86846=ADVANCED_FACE('',(#18526),#16334,.T.) ;
#86847=ADVANCED_FACE('',(#18527),#14195,.T.) ;
#86848=ADVANCED_FACE('',(#18528),#16335,.T.) ;
#86849=ADVANCED_FACE('',(#18529),#14196,.T.) ;
#86850=ADVANCED_FACE('',(#18530),#14197,.T.) ;
#86851=ADVANCED_FACE('',(#18531),#16336,.T.) ;
#86852=ADVANCED_FACE('',(#18532),#14198,.T.) ;
#86853=ADVANCED_FACE('',(#18533),#14199,.T.) ;
#86854=ADVANCED_FACE('',(#18534),#16337,.T.) ;
#86855=ADVANCED_FACE('',(#18535),#1162,.T.) ;
#86856=ADVANCED_FACE('',(#18536),#1163,.T.) ;
#86857=ADVANCED_FACE('',(#18537),#1164,.T.) ;
#86858=ADVANCED_FACE('',(#18538),#1165,.T.) ;
#86859=ADVANCED_FACE('',(#18539),#1166,.T.) ;
#86860=ADVANCED_FACE('',(#18540),#1167,.T.) ;
#86861=ADVANCED_FACE('',(#18541),#1168,.T.) ;
#86862=ADVANCED_FACE('',(#18542),#1169,.T.) ;
#86863=ADVANCED_FACE('',(#18543),#1170,.T.) ;
#86864=ADVANCED_FACE('',(#18544),#1171,.F.) ;
#86865=ADVANCED_FACE('',(#18545),#1172,.F.) ;
#86866=ADVANCED_FACE('',(#18546),#1173,.F.) ;
#86867=ADVANCED_FACE('',(#18547),#1174,.F.) ;
#86868=ADVANCED_FACE('',(#18548),#1175,.F.) ;
#86869=ADVANCED_FACE('',(#18549),#1176,.F.) ;
#86870=ADVANCED_FACE('',(#18550),#1177,.F.) ;
#86871=ADVANCED_FACE('',(#18551),#1178,.F.) ;
#86872=ADVANCED_FACE('',(#18552),#1179,.F.) ;
#86873=ADVANCED_FACE('',(#18553),#1180,.F.) ;
#86874=ADVANCED_FACE('',(#18554),#1181,.F.) ;
#86875=ADVANCED_FACE('',(#18555),#1182,.F.) ;
#86876=ADVANCED_FACE('',(#18556),#1183,.F.) ;
#86877=ADVANCED_FACE('',(#18557),#1184,.F.) ;
#86878=ADVANCED_FACE('',(#18558),#1185,.F.) ;
#86879=ADVANCED_FACE('',(#18559),#1186,.F.) ;
#86880=ADVANCED_FACE('',(#18560),#1187,.F.) ;
#86881=ADVANCED_FACE('',(#18561),#1188,.F.) ;
#86882=ADVANCED_FACE('',(#18562),#1189,.F.) ;
#86883=ADVANCED_FACE('',(#18563),#1190,.F.) ;
#86884=ADVANCED_FACE('',(#18564),#1191,.F.) ;
#86885=ADVANCED_FACE('',(#18565),#1192,.F.) ;
#86886=ADVANCED_FACE('',(#18566),#1193,.F.) ;
#86887=ADVANCED_FACE('',(#18567),#1194,.F.) ;
#86888=ADVANCED_FACE('',(#18568),#1195,.F.) ;
#86889=ADVANCED_FACE('',(#18569),#1196,.F.) ;
#86890=ADVANCED_FACE('',(#18570),#1197,.F.) ;
#86891=ADVANCED_FACE('',(#18571),#1198,.F.) ;
#86892=ADVANCED_FACE('',(#18572),#1199,.F.) ;
#86893=ADVANCED_FACE('',(#18573),#1200,.F.) ;
#86894=ADVANCED_FACE('',(#18574),#1201,.F.) ;
#86895=ADVANCED_FACE('',(#18575),#1202,.F.) ;
#86896=ADVANCED_FACE('',(#18576),#1203,.F.) ;
#86897=ADVANCED_FACE('',(#18577),#1204,.F.) ;
#86898=ADVANCED_FACE('',(#18578),#1205,.F.) ;
#86899=ADVANCED_FACE('',(#18579),#1206,.F.) ;
#86900=ADVANCED_FACE('',(#18580),#1207,.F.) ;
#86901=ADVANCED_FACE('',(#18581),#1208,.F.) ;
#86902=ADVANCED_FACE('',(#18582),#1209,.F.) ;
#86903=ADVANCED_FACE('',(#18583),#1210,.F.) ;
#86904=ADVANCED_FACE('',(#18584),#1211,.F.) ;
#86905=ADVANCED_FACE('',(#18585),#1212,.F.) ;
#86906=ADVANCED_FACE('',(#18586),#1213,.F.) ;
#86907=ADVANCED_FACE('',(#18587),#1214,.F.) ;
#86908=ADVANCED_FACE('',(#18588),#1215,.F.) ;
#86909=ADVANCED_FACE('',(#18589),#14200,.T.) ;
#86910=ADVANCED_FACE('',(#18590),#1216,.F.) ;
#86911=ADVANCED_FACE('',(#18591),#14201,.T.) ;
#86912=ADVANCED_FACE('',(#18592),#1217,.F.) ;
#86913=ADVANCED_FACE('',(#18593),#14202,.F.) ;
#86914=ADVANCED_FACE('',(#18594),#1218,.F.) ;
#86915=ADVANCED_FACE('',(#18595),#14203,.F.) ;
#86916=ADVANCED_FACE('',(#18596),#1219,.F.) ;
#86917=ADVANCED_FACE('',(#18597),#1220,.F.) ;
#86918=ADVANCED_FACE('',(#18598),#14204,.F.) ;
#86919=ADVANCED_FACE('',(#18599),#1221,.F.) ;
#86920=ADVANCED_FACE('',(#18600),#14205,.T.) ;
#86921=ADVANCED_FACE('',(#18601),#1222,.F.) ;
#86922=ADVANCED_FACE('',(#18602),#14206,.T.) ;
#86923=ADVANCED_FACE('',(#18603),#1223,.F.) ;
#86924=ADVANCED_FACE('',(#18604),#14207,.F.) ;
#86925=ADVANCED_FACE('',(#18605),#1224,.F.) ;
#86926=ADVANCED_FACE('',(#18606),#14208,.F.) ;
#86927=ADVANCED_FACE('',(#18607),#1225,.F.) ;
#86928=ADVANCED_FACE('',(#18608),#14209,.F.) ;
#86929=ADVANCED_FACE('',(#18609),#14210,.T.) ;
#86930=ADVANCED_FACE('',(#18610),#14211,.F.) ;
#86931=ADVANCED_FACE('',(#18611),#1226,.F.) ;
#86932=ADVANCED_FACE('',(#18612),#14212,.F.) ;
#86933=ADVANCED_FACE('',(#18613),#1227,.F.) ;
#86934=ADVANCED_FACE('',(#18614),#14213,.F.) ;
#86935=ADVANCED_FACE('',(#18615),#1228,.F.) ;
#86936=ADVANCED_FACE('',(#18616,#696),#1229,.F.) ;
#86937=ADVANCED_FACE('',(#18617),#14214,.T.) ;
#86938=ADVANCED_FACE('',(#18618),#1230,.F.) ;
#86939=ADVANCED_FACE('',(#18619),#14215,.T.) ;
#86940=ADVANCED_FACE('',(#18620),#1231,.F.) ;
#86941=ADVANCED_FACE('',(#18621),#14216,.F.) ;
#86942=ADVANCED_FACE('',(#18622),#1232,.F.) ;
#86943=ADVANCED_FACE('',(#18623),#14217,.F.) ;
#86944=ADVANCED_FACE('',(#18624),#1233,.F.) ;
#86945=ADVANCED_FACE('',(#18625),#1234,.F.) ;
#86946=ADVANCED_FACE('',(#18626),#14218,.F.) ;
#86947=ADVANCED_FACE('',(#18627),#1235,.F.) ;
#86948=ADVANCED_FACE('',(#18628),#14219,.T.) ;
#86949=ADVANCED_FACE('',(#18629),#1236,.F.) ;
#86950=ADVANCED_FACE('',(#18630),#14220,.T.) ;
#86951=ADVANCED_FACE('',(#18631),#1237,.F.) ;
#86952=ADVANCED_FACE('',(#18632),#14221,.F.) ;
#86953=ADVANCED_FACE('',(#18633),#1238,.F.) ;
#86954=ADVANCED_FACE('',(#18634),#14222,.F.) ;
#86955=ADVANCED_FACE('',(#18635),#1239,.F.) ;
#86956=ADVANCED_FACE('',(#18636),#14223,.F.) ;
#86957=ADVANCED_FACE('',(#18637),#14224,.T.) ;
#86958=ADVANCED_FACE('',(#18638),#14225,.F.) ;
#86959=ADVANCED_FACE('',(#18639),#1240,.F.) ;
#86960=ADVANCED_FACE('',(#18640),#14226,.F.) ;
#86961=ADVANCED_FACE('',(#18641),#1241,.F.) ;
#86962=ADVANCED_FACE('',(#18642),#14227,.F.) ;
#86963=ADVANCED_FACE('',(#18643),#1242,.F.) ;
#86964=ADVANCED_FACE('',(#18644,#697),#1243,.F.) ;
#86965=ADVANCED_FACE('',(#18645),#14228,.T.) ;
#86966=ADVANCED_FACE('',(#18646),#1244,.F.) ;
#86967=ADVANCED_FACE('',(#18647),#14229,.T.) ;
#86968=ADVANCED_FACE('',(#18648),#1245,.F.) ;
#86969=ADVANCED_FACE('',(#18649),#14230,.F.) ;
#86970=ADVANCED_FACE('',(#18650),#1246,.F.) ;
#86971=ADVANCED_FACE('',(#18651),#14231,.F.) ;
#86972=ADVANCED_FACE('',(#18652),#1247,.F.) ;
#86973=ADVANCED_FACE('',(#18653),#1248,.F.) ;
#86974=ADVANCED_FACE('',(#18654),#14232,.F.) ;
#86975=ADVANCED_FACE('',(#18655),#1249,.F.) ;
#86976=ADVANCED_FACE('',(#18656),#14233,.T.) ;
#86977=ADVANCED_FACE('',(#18657),#1250,.F.) ;
#86978=ADVANCED_FACE('',(#18658),#14234,.T.) ;
#86979=ADVANCED_FACE('',(#18659),#1251,.F.) ;
#86980=ADVANCED_FACE('',(#18660),#14235,.F.) ;
#86981=ADVANCED_FACE('',(#18661),#1252,.F.) ;
#86982=ADVANCED_FACE('',(#18662),#14236,.F.) ;
#86983=ADVANCED_FACE('',(#18663),#1253,.F.) ;
#86984=ADVANCED_FACE('',(#18664),#14237,.F.) ;
#86985=ADVANCED_FACE('',(#18665),#14238,.T.) ;
#86986=ADVANCED_FACE('',(#18666),#14239,.F.) ;
#86987=ADVANCED_FACE('',(#18667),#1254,.F.) ;
#86988=ADVANCED_FACE('',(#18668),#14240,.F.) ;
#86989=ADVANCED_FACE('',(#18669),#1255,.F.) ;
#86990=ADVANCED_FACE('',(#18670),#14241,.F.) ;
#86991=ADVANCED_FACE('',(#18671),#1256,.F.) ;
#86992=ADVANCED_FACE('',(#18672,#698),#1257,.F.) ;
#86993=ADVANCED_FACE('',(#18673),#14242,.T.) ;
#86994=ADVANCED_FACE('',(#18674),#1258,.F.) ;
#86995=ADVANCED_FACE('',(#18675),#14243,.T.) ;
#86996=ADVANCED_FACE('',(#18676),#1259,.F.) ;
#86997=ADVANCED_FACE('',(#18677),#14244,.F.) ;
#86998=ADVANCED_FACE('',(#18678),#1260,.F.) ;
#86999=ADVANCED_FACE('',(#18679),#14245,.F.) ;
#87000=ADVANCED_FACE('',(#18680),#1261,.F.) ;
#87001=ADVANCED_FACE('',(#18681),#1262,.F.) ;
#87002=ADVANCED_FACE('',(#18682),#14246,.F.) ;
#87003=ADVANCED_FACE('',(#18683),#1263,.F.) ;
#87004=ADVANCED_FACE('',(#18684),#14247,.T.) ;
#87005=ADVANCED_FACE('',(#18685),#1264,.F.) ;
#87006=ADVANCED_FACE('',(#18686),#14248,.T.) ;
#87007=ADVANCED_FACE('',(#18687),#1265,.F.) ;
#87008=ADVANCED_FACE('',(#18688),#14249,.F.) ;
#87009=ADVANCED_FACE('',(#18689),#1266,.F.) ;
#87010=ADVANCED_FACE('',(#18690),#14250,.F.) ;
#87011=ADVANCED_FACE('',(#18691),#1267,.F.) ;
#87012=ADVANCED_FACE('',(#18692),#14251,.F.) ;
#87013=ADVANCED_FACE('',(#18693),#14252,.T.) ;
#87014=ADVANCED_FACE('',(#18694),#14253,.F.) ;
#87015=ADVANCED_FACE('',(#18695),#1268,.F.) ;
#87016=ADVANCED_FACE('',(#18696),#14254,.F.) ;
#87017=ADVANCED_FACE('',(#18697),#1269,.F.) ;
#87018=ADVANCED_FACE('',(#18698),#14255,.F.) ;
#87019=ADVANCED_FACE('',(#18699),#1270,.F.) ;
#87020=ADVANCED_FACE('',(#18700,#699),#1271,.F.) ;
#87021=ADVANCED_FACE('',(#18701),#14256,.T.) ;
#87022=ADVANCED_FACE('',(#18702),#1272,.F.) ;
#87023=ADVANCED_FACE('',(#18703),#14257,.T.) ;
#87024=ADVANCED_FACE('',(#18704),#1273,.F.) ;
#87025=ADVANCED_FACE('',(#18705),#14258,.F.) ;
#87026=ADVANCED_FACE('',(#18706),#1274,.F.) ;
#87027=ADVANCED_FACE('',(#18707),#14259,.F.) ;
#87028=ADVANCED_FACE('',(#18708),#1275,.F.) ;
#87029=ADVANCED_FACE('',(#18709),#1276,.F.) ;
#87030=ADVANCED_FACE('',(#18710),#14260,.F.) ;
#87031=ADVANCED_FACE('',(#18711),#1277,.F.) ;
#87032=ADVANCED_FACE('',(#18712),#14261,.T.) ;
#87033=ADVANCED_FACE('',(#18713),#1278,.F.) ;
#87034=ADVANCED_FACE('',(#18714),#14262,.T.) ;
#87035=ADVANCED_FACE('',(#18715),#1279,.F.) ;
#87036=ADVANCED_FACE('',(#18716),#14263,.F.) ;
#87037=ADVANCED_FACE('',(#18717),#1280,.F.) ;
#87038=ADVANCED_FACE('',(#18718),#14264,.F.) ;
#87039=ADVANCED_FACE('',(#18719),#1281,.F.) ;
#87040=ADVANCED_FACE('',(#18720),#14265,.F.) ;
#87041=ADVANCED_FACE('',(#18721),#14266,.T.) ;
#87042=ADVANCED_FACE('',(#18722),#14267,.F.) ;
#87043=ADVANCED_FACE('',(#18723),#1282,.F.) ;
#87044=ADVANCED_FACE('',(#18724),#14268,.F.) ;
#87045=ADVANCED_FACE('',(#18725),#1283,.F.) ;
#87046=ADVANCED_FACE('',(#18726),#14269,.F.) ;
#87047=ADVANCED_FACE('',(#18727),#1284,.F.) ;
#87048=ADVANCED_FACE('',(#18728,#700),#1285,.F.) ;
#87049=ADVANCED_FACE('',(#18729),#14270,.T.) ;
#87050=ADVANCED_FACE('',(#18730),#1286,.F.) ;
#87051=ADVANCED_FACE('',(#18731),#14271,.T.) ;
#87052=ADVANCED_FACE('',(#18732),#1287,.F.) ;
#87053=ADVANCED_FACE('',(#18733),#14272,.F.) ;
#87054=ADVANCED_FACE('',(#18734),#1288,.F.) ;
#87055=ADVANCED_FACE('',(#18735),#14273,.F.) ;
#87056=ADVANCED_FACE('',(#18736),#1289,.F.) ;
#87057=ADVANCED_FACE('',(#18737),#1290,.F.) ;
#87058=ADVANCED_FACE('',(#18738),#14274,.F.) ;
#87059=ADVANCED_FACE('',(#18739),#1291,.F.) ;
#87060=ADVANCED_FACE('',(#18740),#14275,.T.) ;
#87061=ADVANCED_FACE('',(#18741),#1292,.F.) ;
#87062=ADVANCED_FACE('',(#18742),#14276,.T.) ;
#87063=ADVANCED_FACE('',(#18743),#1293,.F.) ;
#87064=ADVANCED_FACE('',(#18744),#14277,.F.) ;
#87065=ADVANCED_FACE('',(#18745),#1294,.F.) ;
#87066=ADVANCED_FACE('',(#18746),#14278,.F.) ;
#87067=ADVANCED_FACE('',(#18747),#1295,.F.) ;
#87068=ADVANCED_FACE('',(#18748),#14279,.F.) ;
#87069=ADVANCED_FACE('',(#18749),#14280,.T.) ;
#87070=ADVANCED_FACE('',(#18750),#14281,.F.) ;
#87071=ADVANCED_FACE('',(#18751),#1296,.F.) ;
#87072=ADVANCED_FACE('',(#18752),#14282,.F.) ;
#87073=ADVANCED_FACE('',(#18753),#1297,.F.) ;
#87074=ADVANCED_FACE('',(#18754),#14283,.F.) ;
#87075=ADVANCED_FACE('',(#18755),#1298,.F.) ;
#87076=ADVANCED_FACE('',(#18756,#701),#1299,.F.) ;
#87077=ADVANCED_FACE('',(#18757),#14284,.T.) ;
#87078=ADVANCED_FACE('',(#18758),#1300,.F.) ;
#87079=ADVANCED_FACE('',(#18759),#14285,.T.) ;
#87080=ADVANCED_FACE('',(#18760),#1301,.F.) ;
#87081=ADVANCED_FACE('',(#18761),#14286,.F.) ;
#87082=ADVANCED_FACE('',(#18762),#1302,.F.) ;
#87083=ADVANCED_FACE('',(#18763),#14287,.F.) ;
#87084=ADVANCED_FACE('',(#18764),#1303,.F.) ;
#87085=ADVANCED_FACE('',(#18765),#1304,.F.) ;
#87086=ADVANCED_FACE('',(#18766),#14288,.F.) ;
#87087=ADVANCED_FACE('',(#18767),#1305,.F.) ;
#87088=ADVANCED_FACE('',(#18768),#14289,.T.) ;
#87089=ADVANCED_FACE('',(#18769),#1306,.F.) ;
#87090=ADVANCED_FACE('',(#18770),#14290,.T.) ;
#87091=ADVANCED_FACE('',(#18771),#1307,.F.) ;
#87092=ADVANCED_FACE('',(#18772),#14291,.F.) ;
#87093=ADVANCED_FACE('',(#18773),#1308,.F.) ;
#87094=ADVANCED_FACE('',(#18774),#14292,.F.) ;
#87095=ADVANCED_FACE('',(#18775),#1309,.F.) ;
#87096=ADVANCED_FACE('',(#18776),#14293,.F.) ;
#87097=ADVANCED_FACE('',(#18777),#14294,.T.) ;
#87098=ADVANCED_FACE('',(#18778),#14295,.F.) ;
#87099=ADVANCED_FACE('',(#18779),#1310,.F.) ;
#87100=ADVANCED_FACE('',(#18780),#14296,.F.) ;
#87101=ADVANCED_FACE('',(#18781),#1311,.F.) ;
#87102=ADVANCED_FACE('',(#18782),#14297,.F.) ;
#87103=ADVANCED_FACE('',(#18783),#1312,.F.) ;
#87104=ADVANCED_FACE('',(#18784,#702),#1313,.F.) ;
#87105=ADVANCED_FACE('',(#18785),#14298,.T.) ;
#87106=ADVANCED_FACE('',(#18786),#1314,.F.) ;
#87107=ADVANCED_FACE('',(#18787),#14299,.T.) ;
#87108=ADVANCED_FACE('',(#18788),#1315,.F.) ;
#87109=ADVANCED_FACE('',(#18789),#14300,.F.) ;
#87110=ADVANCED_FACE('',(#18790),#1316,.F.) ;
#87111=ADVANCED_FACE('',(#18791),#14301,.F.) ;
#87112=ADVANCED_FACE('',(#18792),#1317,.F.) ;
#87113=ADVANCED_FACE('',(#18793),#1318,.F.) ;
#87114=ADVANCED_FACE('',(#18794),#14302,.F.) ;
#87115=ADVANCED_FACE('',(#18795),#1319,.F.) ;
#87116=ADVANCED_FACE('',(#18796),#14303,.T.) ;
#87117=ADVANCED_FACE('',(#18797),#1320,.F.) ;
#87118=ADVANCED_FACE('',(#18798),#14304,.T.) ;
#87119=ADVANCED_FACE('',(#18799),#1321,.F.) ;
#87120=ADVANCED_FACE('',(#18800),#14305,.F.) ;
#87121=ADVANCED_FACE('',(#18801),#1322,.F.) ;
#87122=ADVANCED_FACE('',(#18802),#14306,.F.) ;
#87123=ADVANCED_FACE('',(#18803),#1323,.F.) ;
#87124=ADVANCED_FACE('',(#18804),#14307,.F.) ;
#87125=ADVANCED_FACE('',(#18805),#14308,.T.) ;
#87126=ADVANCED_FACE('',(#18806),#14309,.F.) ;
#87127=ADVANCED_FACE('',(#18807),#1324,.F.) ;
#87128=ADVANCED_FACE('',(#18808),#14310,.F.) ;
#87129=ADVANCED_FACE('',(#18809),#1325,.F.) ;
#87130=ADVANCED_FACE('',(#18810),#14311,.F.) ;
#87131=ADVANCED_FACE('',(#18811),#1326,.F.) ;
#87132=ADVANCED_FACE('',(#18812,#703),#1327,.F.) ;
#87133=ADVANCED_FACE('',(#18813),#14312,.T.) ;
#87134=ADVANCED_FACE('',(#18814),#1328,.F.) ;
#87135=ADVANCED_FACE('',(#18815),#14313,.T.) ;
#87136=ADVANCED_FACE('',(#18816),#1329,.F.) ;
#87137=ADVANCED_FACE('',(#18817),#14314,.F.) ;
#87138=ADVANCED_FACE('',(#18818),#1330,.F.) ;
#87139=ADVANCED_FACE('',(#18819),#14315,.F.) ;
#87140=ADVANCED_FACE('',(#18820),#1331,.F.) ;
#87141=ADVANCED_FACE('',(#18821),#1332,.F.) ;
#87142=ADVANCED_FACE('',(#18822),#14316,.F.) ;
#87143=ADVANCED_FACE('',(#18823),#1333,.F.) ;
#87144=ADVANCED_FACE('',(#18824),#14317,.T.) ;
#87145=ADVANCED_FACE('',(#18825),#1334,.F.) ;
#87146=ADVANCED_FACE('',(#18826),#14318,.T.) ;
#87147=ADVANCED_FACE('',(#18827),#1335,.F.) ;
#87148=ADVANCED_FACE('',(#18828),#14319,.F.) ;
#87149=ADVANCED_FACE('',(#18829),#1336,.F.) ;
#87150=ADVANCED_FACE('',(#18830),#14320,.F.) ;
#87151=ADVANCED_FACE('',(#18831),#1337,.F.) ;
#87152=ADVANCED_FACE('',(#18832),#14321,.F.) ;
#87153=ADVANCED_FACE('',(#18833),#14322,.T.) ;
#87154=ADVANCED_FACE('',(#18834),#14323,.F.) ;
#87155=ADVANCED_FACE('',(#18835),#1338,.F.) ;
#87156=ADVANCED_FACE('',(#18836),#14324,.F.) ;
#87157=ADVANCED_FACE('',(#18837),#1339,.F.) ;
#87158=ADVANCED_FACE('',(#18838),#14325,.F.) ;
#87159=ADVANCED_FACE('',(#18839),#1340,.F.) ;
#87160=ADVANCED_FACE('',(#18840,#704),#1341,.F.) ;
#87161=ADVANCED_FACE('',(#18841,#705),#1342,.T.) ;
#87162=ADVANCED_FACE('',(#18842,#706),#1343,.T.) ;
#87163=ADVANCED_FACE('',(#18843,#707),#1344,.T.) ;
#87164=ADVANCED_FACE('',(#18844,#708),#1345,.T.) ;
#87165=ADVANCED_FACE('',(#18845,#709),#1346,.T.) ;
#87166=ADVANCED_FACE('',(#18846,#710),#1347,.T.) ;
#87167=ADVANCED_FACE('',(#18847,#711),#1348,.T.) ;
#87168=ADVANCED_FACE('',(#18848,#712),#1349,.T.) ;
#87169=ADVANCED_FACE('',(#18849,#713),#1350,.T.) ;
#87170=ADVANCED_FACE('',(#18850),#14326,.T.) ;
#87171=ADVANCED_FACE('',(#18851),#14327,.F.) ;
#87172=ADVANCED_FACE('',(#18852),#16338,.F.) ;
#87173=ADVANCED_FACE('',(#18853),#16339,.T.) ;
#87174=ADVANCED_FACE('',(#18854),#79083,.T.) ;
#87175=ADVANCED_FACE('',(#18855),#14328,.F.) ;
#87176=ADVANCED_FACE('',(#18856),#14329,.F.) ;
#87177=ADVANCED_FACE('',(#18857),#14330,.T.) ;
#87178=ADVANCED_FACE('',(#18858),#14331,.T.) ;
#87179=ADVANCED_FACE('',(#18859),#14332,.T.) ;
#87180=ADVANCED_FACE('',(#18860),#14333,.F.) ;
#87181=ADVANCED_FACE('',(#18861),#16340,.F.) ;
#87182=ADVANCED_FACE('',(#18862),#79084,.F.) ;
#87183=ADVANCED_FACE('',(#18863),#79085,.F.) ;
#87184=ADVANCED_FACE('',(#18864),#79086,.T.) ;
#87185=ADVANCED_FACE('',(#18865),#14334,.F.) ;
#87186=ADVANCED_FACE('',(#18866),#14335,.F.) ;
#87187=ADVANCED_FACE('',(#18867),#14336,.F.) ;
#87188=ADVANCED_FACE('',(#18868),#14337,.T.) ;
#87189=ADVANCED_FACE('',(#18869),#14338,.T.) ;
#87190=ADVANCED_FACE('',(#18870),#79087,.F.) ;
#87191=ADVANCED_FACE('',(#18871),#16341,.F.) ;
#87192=ADVANCED_FACE('',(#18872),#16342,.T.) ;
#87193=ADVANCED_FACE('',(#18873),#14339,.T.) ;
#87194=ADVANCED_FACE('',(#18874),#16343,.F.) ;
#87195=ADVANCED_FACE('',(#18875),#16344,.T.) ;
#87196=ADVANCED_FACE('',(#18876),#14340,.F.) ;
#87197=ADVANCED_FACE('',(#18877),#14341,.F.) ;
#87198=ADVANCED_FACE('',(#18878),#14342,.T.) ;
#87199=ADVANCED_FACE('',(#18879),#79088,.T.) ;
#87200=ADVANCED_FACE('',(#18880),#14343,.F.) ;
#87201=ADVANCED_FACE('',(#18881),#14344,.T.) ;
#87202=ADVANCED_FACE('',(#18882),#14345,.F.) ;
#87203=ADVANCED_FACE('',(#18883),#16345,.F.) ;
#87204=ADVANCED_FACE('',(#18884),#79089,.T.) ;
#87205=ADVANCED_FACE('',(#18885),#14346,.T.) ;
#87206=ADVANCED_FACE('',(#18886),#16346,.F.) ;
#87207=ADVANCED_FACE('',(#18887),#79090,.F.) ;
#87208=ADVANCED_FACE('',(#18888),#14347,.F.) ;
#87209=ADVANCED_FACE('',(#18889),#14348,.T.) ;
#87210=ADVANCED_FACE('',(#18890),#79091,.T.) ;
#87211=ADVANCED_FACE('',(#18891),#14349,.F.) ;
#87212=ADVANCED_FACE('',(#18892),#79092,.T.) ;
#87213=ADVANCED_FACE('',(#18893),#14350,.T.) ;
#87214=ADVANCED_FACE('',(#18894),#14351,.T.) ;
#87215=ADVANCED_FACE('',(#18895),#16347,.T.) ;
#87216=ADVANCED_FACE('',(#18896),#14352,.F.) ;
#87217=ADVANCED_FACE('',(#18897),#79093,.F.) ;
#87218=ADVANCED_FACE('',(#18898),#16348,.F.) ;
#87219=ADVANCED_FACE('',(#18899),#14353,.F.) ;
#87220=ADVANCED_FACE('',(#18900),#14354,.F.) ;
#87221=ADVANCED_FACE('',(#18901),#79094,.F.) ;
#87222=ADVANCED_FACE('',(#18902),#16349,.F.) ;
#87223=ADVANCED_FACE('',(#18903),#14355,.F.) ;
#87224=ADVANCED_FACE('',(#18904),#14356,.F.) ;
#87225=ADVANCED_FACE('',(#18905),#16350,.F.) ;
#87226=ADVANCED_FACE('',(#18906),#16351,.F.) ;
#87227=ADVANCED_FACE('',(#18907),#14357,.F.) ;
#87228=ADVANCED_FACE('',(#18908),#79095,.F.) ;
#87229=ADVANCED_FACE('',(#18909),#16352,.F.) ;
#87230=ADVANCED_FACE('',(#18910),#16353,.F.) ;
#87231=ADVANCED_FACE('',(#18911),#14358,.F.) ;
#87232=ADVANCED_FACE('',(#18912),#14359,.F.) ;
#87233=ADVANCED_FACE('',(#18913),#16354,.F.) ;
#87234=ADVANCED_FACE('',(#18914),#14360,.F.) ;
#87235=ADVANCED_FACE('',(#18915),#14361,.F.) ;
#87236=ADVANCED_FACE('',(#18916),#16355,.F.) ;
#87237=ADVANCED_FACE('',(#18917),#16356,.F.) ;
#87238=ADVANCED_FACE('',(#18918),#14362,.F.) ;
#87239=ADVANCED_FACE('',(#18919),#14363,.F.) ;
#87240=ADVANCED_FACE('',(#18920),#79096,.F.) ;
#87241=ADVANCED_FACE('',(#18921),#79097,.F.) ;
#87242=ADVANCED_FACE('',(#18922),#14364,.F.) ;
#87243=ADVANCED_FACE('',(#18923),#14365,.T.) ;
#87244=ADVANCED_FACE('',(#18924),#16357,.T.) ;
#87245=ADVANCED_FACE('',(#18925),#16358,.T.) ;
#87246=ADVANCED_FACE('',(#18926),#14366,.T.) ;
#87247=ADVANCED_FACE('',(#18927),#14367,.T.) ;
#87248=ADVANCED_FACE('',(#18928),#79098,.T.) ;
#87249=ADVANCED_FACE('',(#18929),#79099,.T.) ;
#87250=ADVANCED_FACE('',(#18930),#14368,.T.) ;
#87251=ADVANCED_FACE('',(#18931),#14369,.T.) ;
#87252=ADVANCED_FACE('',(#18932),#79100,.T.) ;
#87253=ADVANCED_FACE('',(#18933),#14370,.T.) ;
#87254=ADVANCED_FACE('',(#18934),#14371,.T.) ;
#87255=ADVANCED_FACE('',(#18935),#79101,.T.) ;
#87256=ADVANCED_FACE('',(#18936),#79102,.T.) ;
#87257=ADVANCED_FACE('',(#18937),#14372,.T.) ;
#87258=ADVANCED_FACE('',(#18938),#79103,.T.) ;
#87259=ADVANCED_FACE('',(#18939),#79104,.T.) ;
#87260=ADVANCED_FACE('',(#18940),#79105,.T.) ;
#87261=ADVANCED_FACE('',(#18941),#14373,.T.) ;
#87262=ADVANCED_FACE('',(#18942),#14374,.T.) ;
#87263=ADVANCED_FACE('',(#18943),#16359,.T.) ;
#87264=ADVANCED_FACE('',(#18944),#79106,.T.) ;
#87265=ADVANCED_FACE('',(#18945),#14375,.T.) ;
#87266=ADVANCED_FACE('',(#18946),#14376,.T.) ;
#87267=ADVANCED_FACE('',(#18947),#16360,.T.) ;
#87268=ADVANCED_FACE('',(#18948),#79107,.T.) ;
#87269=ADVANCED_FACE('',(#18949),#14377,.T.) ;
#87270=ADVANCED_FACE('',(#18950),#14378,.T.) ;
#87271=ADVANCED_FACE('',(#18951),#16361,.T.) ;
#87272=ADVANCED_FACE('',(#18952),#16362,.T.) ;
#87273=ADVANCED_FACE('',(#18953),#14379,.T.) ;
#87274=ADVANCED_FACE('',(#18954),#14380,.T.) ;
#87275=ADVANCED_FACE('',(#18955),#79108,.T.) ;
#87276=ADVANCED_FACE('',(#18956),#79109,.T.) ;
#87277=ADVANCED_FACE('',(#18957),#14381,.T.) ;
#87278=ADVANCED_FACE('',(#18958),#14382,.T.) ;
#87279=ADVANCED_FACE('',(#18959),#79110,.T.) ;
#87280=ADVANCED_FACE('',(#18960),#14383,.T.) ;
#87281=ADVANCED_FACE('',(#18961),#14384,.T.) ;
#87282=ADVANCED_FACE('',(#18962),#79111,.T.) ;
#87283=ADVANCED_FACE('',(#18963),#79112,.T.) ;
#87284=ADVANCED_FACE('',(#18964),#14385,.T.) ;
#87285=ADVANCED_FACE('',(#18965),#79113,.T.) ;
#87286=ADVANCED_FACE('',(#18966),#79114,.T.) ;
#87287=ADVANCED_FACE('',(#18967),#79115,.T.) ;
#87288=ADVANCED_FACE('',(#18968),#14386,.T.) ;
#87289=ADVANCED_FACE('',(#18969),#14387,.T.) ;
#87290=ADVANCED_FACE('',(#18970),#16363,.T.) ;
#87291=ADVANCED_FACE('',(#18971),#79116,.T.) ;
#87292=ADVANCED_FACE('',(#18972),#14388,.T.) ;
#87293=ADVANCED_FACE('',(#18973),#14389,.T.) ;
#87294=ADVANCED_FACE('',(#18974),#16364,.T.) ;
#87295=ADVANCED_FACE('',(#18975),#79117,.T.) ;
#87296=ADVANCED_FACE('',(#18976),#14390,.T.) ;
#87297=ADVANCED_FACE('',(#18977),#14391,.T.) ;
#87298=ADVANCED_FACE('',(#18978),#16365,.T.) ;
#87299=ADVANCED_FACE('',(#18979),#16366,.T.) ;
#87300=ADVANCED_FACE('',(#18980),#14392,.T.) ;
#87301=ADVANCED_FACE('',(#18981),#14393,.T.) ;
#87302=ADVANCED_FACE('',(#18982),#79118,.T.) ;
#87303=ADVANCED_FACE('',(#18983),#79119,.T.) ;
#87304=ADVANCED_FACE('',(#18984),#14394,.T.) ;
#87305=ADVANCED_FACE('',(#18985),#14395,.T.) ;
#87306=ADVANCED_FACE('',(#18986),#79120,.T.) ;
#87307=ADVANCED_FACE('',(#18987),#14396,.T.) ;
#87308=ADVANCED_FACE('',(#18988),#14397,.T.) ;
#87309=ADVANCED_FACE('',(#18989),#79121,.T.) ;
#87310=ADVANCED_FACE('',(#18990),#79122,.T.) ;
#87311=ADVANCED_FACE('',(#18991),#14398,.T.) ;
#87312=ADVANCED_FACE('',(#18992),#79123,.T.) ;
#87313=ADVANCED_FACE('',(#18993),#79124,.T.) ;
#87314=ADVANCED_FACE('',(#18994),#79125,.T.) ;
#87315=ADVANCED_FACE('',(#18995),#14399,.T.) ;
#87316=ADVANCED_FACE('',(#18996),#14400,.T.) ;
#87317=ADVANCED_FACE('',(#18997),#16367,.T.) ;
#87318=ADVANCED_FACE('',(#18998),#79126,.T.) ;
#87319=ADVANCED_FACE('',(#18999),#14401,.T.) ;
#87320=ADVANCED_FACE('',(#19000),#14402,.T.) ;
#87321=ADVANCED_FACE('',(#19001),#16368,.T.) ;
#87322=ADVANCED_FACE('',(#19002),#79127,.T.) ;
#87323=ADVANCED_FACE('',(#19003),#14403,.T.) ;
#87324=ADVANCED_FACE('',(#19004),#14404,.T.) ;
#87325=ADVANCED_FACE('',(#19005),#16369,.T.) ;
#87326=ADVANCED_FACE('',(#19006),#16370,.T.) ;
#87327=ADVANCED_FACE('',(#19007),#14405,.T.) ;
#87328=ADVANCED_FACE('',(#19008),#14406,.T.) ;
#87329=ADVANCED_FACE('',(#19009),#79128,.T.) ;
#87330=ADVANCED_FACE('',(#19010),#79129,.T.) ;
#87331=ADVANCED_FACE('',(#19011),#14407,.T.) ;
#87332=ADVANCED_FACE('',(#19012),#14408,.T.) ;
#87333=ADVANCED_FACE('',(#19013),#79130,.T.) ;
#87334=ADVANCED_FACE('',(#19014),#14409,.T.) ;
#87335=ADVANCED_FACE('',(#19015),#14410,.T.) ;
#87336=ADVANCED_FACE('',(#19016),#79131,.T.) ;
#87337=ADVANCED_FACE('',(#19017),#79132,.T.) ;
#87338=ADVANCED_FACE('',(#19018),#14411,.T.) ;
#87339=ADVANCED_FACE('',(#19019),#79133,.T.) ;
#87340=ADVANCED_FACE('',(#19020),#79134,.T.) ;
#87341=ADVANCED_FACE('',(#19021),#79135,.T.) ;
#87342=ADVANCED_FACE('',(#19022),#14412,.T.) ;
#87343=ADVANCED_FACE('',(#19023),#14413,.T.) ;
#87344=ADVANCED_FACE('',(#19024),#16371,.T.) ;
#87345=ADVANCED_FACE('',(#19025),#79136,.T.) ;
#87346=ADVANCED_FACE('',(#19026),#14414,.T.) ;
#87347=ADVANCED_FACE('',(#19027),#14415,.T.) ;
#87348=ADVANCED_FACE('',(#19028),#16372,.T.) ;
#87349=ADVANCED_FACE('',(#19029),#79137,.T.) ;
#87350=ADVANCED_FACE('',(#19030),#14416,.T.) ;
#87351=ADVANCED_FACE('',(#19031),#14417,.T.) ;
#87352=ADVANCED_FACE('',(#19032),#16373,.T.) ;
#87353=ADVANCED_FACE('',(#19033),#16374,.T.) ;
#87354=ADVANCED_FACE('',(#19034),#14418,.T.) ;
#87355=ADVANCED_FACE('',(#19035),#14419,.T.) ;
#87356=ADVANCED_FACE('',(#19036),#79138,.T.) ;
#87357=ADVANCED_FACE('',(#19037),#79139,.T.) ;
#87358=ADVANCED_FACE('',(#19038),#14420,.T.) ;
#87359=ADVANCED_FACE('',(#19039),#14421,.T.) ;
#87360=ADVANCED_FACE('',(#19040),#79140,.T.) ;
#87361=ADVANCED_FACE('',(#19041),#14422,.T.) ;
#87362=ADVANCED_FACE('',(#19042),#14423,.T.) ;
#87363=ADVANCED_FACE('',(#19043),#79141,.T.) ;
#87364=ADVANCED_FACE('',(#19044),#79142,.T.) ;
#87365=ADVANCED_FACE('',(#19045),#14424,.T.) ;
#87366=ADVANCED_FACE('',(#19046),#79143,.T.) ;
#87367=ADVANCED_FACE('',(#19047),#79144,.T.) ;
#87368=ADVANCED_FACE('',(#19048),#79145,.T.) ;
#87369=ADVANCED_FACE('',(#19049),#14425,.T.) ;
#87370=ADVANCED_FACE('',(#19050),#14426,.T.) ;
#87371=ADVANCED_FACE('',(#19051),#16375,.T.) ;
#87372=ADVANCED_FACE('',(#19052),#79146,.T.) ;
#87373=ADVANCED_FACE('',(#19053),#14427,.T.) ;
#87374=ADVANCED_FACE('',(#19054),#14428,.T.) ;
#87375=ADVANCED_FACE('',(#19055),#16376,.T.) ;
#87376=ADVANCED_FACE('',(#19056),#79147,.T.) ;
#87377=ADVANCED_FACE('',(#19057),#14429,.T.) ;
#87378=ADVANCED_FACE('',(#19058),#14430,.T.) ;
#87379=ADVANCED_FACE('',(#19059),#16377,.T.) ;
#87380=ADVANCED_FACE('',(#19060),#16378,.T.) ;
#87381=ADVANCED_FACE('',(#19061),#14431,.T.) ;
#87382=ADVANCED_FACE('',(#19062),#14432,.T.) ;
#87383=ADVANCED_FACE('',(#19063),#79148,.T.) ;
#87384=ADVANCED_FACE('',(#19064),#79149,.T.) ;
#87385=ADVANCED_FACE('',(#19065),#14433,.T.) ;
#87386=ADVANCED_FACE('',(#19066),#14434,.T.) ;
#87387=ADVANCED_FACE('',(#19067),#79150,.T.) ;
#87388=ADVANCED_FACE('',(#19068),#14435,.T.) ;
#87389=ADVANCED_FACE('',(#19069),#14436,.T.) ;
#87390=ADVANCED_FACE('',(#19070),#79151,.T.) ;
#87391=ADVANCED_FACE('',(#19071),#79152,.T.) ;
#87392=ADVANCED_FACE('',(#19072),#14437,.T.) ;
#87393=ADVANCED_FACE('',(#19073),#79153,.T.) ;
#87394=ADVANCED_FACE('',(#19074),#79154,.T.) ;
#87395=ADVANCED_FACE('',(#19075),#79155,.T.) ;
#87396=ADVANCED_FACE('',(#19076),#14438,.T.) ;
#87397=ADVANCED_FACE('',(#19077),#14439,.T.) ;
#87398=ADVANCED_FACE('',(#19078),#16379,.T.) ;
#87399=ADVANCED_FACE('',(#19079),#79156,.T.) ;
#87400=ADVANCED_FACE('',(#19080),#14440,.T.) ;
#87401=ADVANCED_FACE('',(#19081),#14441,.T.) ;
#87402=ADVANCED_FACE('',(#19082),#16380,.T.) ;
#87403=ADVANCED_FACE('',(#19083),#79157,.T.) ;
#87404=ADVANCED_FACE('',(#19084),#14442,.T.) ;
#87405=ADVANCED_FACE('',(#19085),#14443,.T.) ;
#87406=ADVANCED_FACE('',(#19086),#16381,.T.) ;
#87407=ADVANCED_FACE('',(#19087),#16382,.T.) ;
#87408=ADVANCED_FACE('',(#19088),#14444,.T.) ;
#87409=ADVANCED_FACE('',(#19089),#14445,.T.) ;
#87410=ADVANCED_FACE('',(#19090),#79158,.T.) ;
#87411=ADVANCED_FACE('',(#19091),#79159,.T.) ;
#87412=ADVANCED_FACE('',(#19092),#14446,.T.) ;
#87413=ADVANCED_FACE('',(#19093),#14447,.T.) ;
#87414=ADVANCED_FACE('',(#19094),#79160,.T.) ;
#87415=ADVANCED_FACE('',(#19095),#14448,.T.) ;
#87416=ADVANCED_FACE('',(#19096),#14449,.T.) ;
#87417=ADVANCED_FACE('',(#19097),#79161,.T.) ;
#87418=ADVANCED_FACE('',(#19098),#79162,.T.) ;
#87419=ADVANCED_FACE('',(#19099),#14450,.T.) ;
#87420=ADVANCED_FACE('',(#19100),#79163,.T.) ;
#87421=ADVANCED_FACE('',(#19101),#79164,.T.) ;
#87422=ADVANCED_FACE('',(#19102),#79165,.T.) ;
#87423=ADVANCED_FACE('',(#19103),#14451,.T.) ;
#87424=ADVANCED_FACE('',(#19104),#14452,.T.) ;
#87425=ADVANCED_FACE('',(#19105),#16383,.T.) ;
#87426=ADVANCED_FACE('',(#19106),#79166,.T.) ;
#87427=ADVANCED_FACE('',(#19107),#14453,.T.) ;
#87428=ADVANCED_FACE('',(#19108),#14454,.T.) ;
#87429=ADVANCED_FACE('',(#19109),#16384,.T.) ;
#87430=ADVANCED_FACE('',(#19110),#79167,.T.) ;
#87431=ADVANCED_FACE('',(#19111),#14455,.T.) ;
#87432=ADVANCED_FACE('',(#19112),#14456,.T.) ;
#87433=ADVANCED_FACE('',(#19113),#16385,.T.) ;
#87434=ADVANCED_FACE('',(#19114),#16386,.T.) ;
#87435=ADVANCED_FACE('',(#19115),#14457,.T.) ;
#87436=ADVANCED_FACE('',(#19116),#14458,.T.) ;
#87437=ADVANCED_FACE('',(#19117),#79168,.T.) ;
#87438=ADVANCED_FACE('',(#19118),#79169,.T.) ;
#87439=ADVANCED_FACE('',(#19119),#14459,.T.) ;
#87440=ADVANCED_FACE('',(#19120),#14460,.T.) ;
#87441=ADVANCED_FACE('',(#19121),#79170,.T.) ;
#87442=ADVANCED_FACE('',(#19122),#14461,.T.) ;
#87443=ADVANCED_FACE('',(#19123),#14462,.T.) ;
#87444=ADVANCED_FACE('',(#19124),#79171,.T.) ;
#87445=ADVANCED_FACE('',(#19125),#79172,.T.) ;
#87446=ADVANCED_FACE('',(#19126),#14463,.T.) ;
#87447=ADVANCED_FACE('',(#19127),#79173,.T.) ;
#87448=ADVANCED_FACE('',(#19128),#79174,.T.) ;
#87449=ADVANCED_FACE('',(#19129),#79175,.T.) ;
#87450=ADVANCED_FACE('',(#19130),#14464,.T.) ;
#87451=ADVANCED_FACE('',(#19131),#14465,.T.) ;
#87452=ADVANCED_FACE('',(#19132),#16387,.T.) ;
#87453=ADVANCED_FACE('',(#19133),#79176,.T.) ;
#87454=ADVANCED_FACE('',(#19134),#14466,.T.) ;
#87455=ADVANCED_FACE('',(#19135),#14467,.T.) ;
#87456=ADVANCED_FACE('',(#19136),#16388,.T.) ;
#87457=ADVANCED_FACE('',(#19137),#79177,.T.) ;
#87458=ADVANCED_FACE('',(#19138),#14468,.T.) ;
#87459=ADVANCED_FACE('',(#19139),#14469,.T.) ;
#87460=ADVANCED_FACE('',(#19140),#16389,.T.) ;
#87461=ADVANCED_FACE('',(#19141),#16390,.T.) ;
#87462=ADVANCED_FACE('',(#19142),#14470,.T.) ;
#87463=ADVANCED_FACE('',(#19143),#14471,.T.) ;
#87464=ADVANCED_FACE('',(#19144),#79178,.T.) ;
#87465=ADVANCED_FACE('',(#19145),#79179,.T.) ;
#87466=ADVANCED_FACE('',(#19146),#14472,.T.) ;
#87467=ADVANCED_FACE('',(#19147),#14473,.T.) ;
#87468=ADVANCED_FACE('',(#19148),#79180,.T.) ;
#87469=ADVANCED_FACE('',(#19149),#14474,.T.) ;
#87470=ADVANCED_FACE('',(#19150),#14475,.T.) ;
#87471=ADVANCED_FACE('',(#19151),#79181,.T.) ;
#87472=ADVANCED_FACE('',(#19152),#79182,.T.) ;
#87473=ADVANCED_FACE('',(#19153),#14476,.T.) ;
#87474=ADVANCED_FACE('',(#19154),#79183,.T.) ;
#87475=ADVANCED_FACE('',(#19155),#79184,.T.) ;
#87476=ADVANCED_FACE('',(#19156),#79185,.T.) ;
#87477=ADVANCED_FACE('',(#19157),#14477,.T.) ;
#87478=ADVANCED_FACE('',(#19158),#14478,.T.) ;
#87479=ADVANCED_FACE('',(#19159),#16391,.T.) ;
#87480=ADVANCED_FACE('',(#19160),#79186,.T.) ;
#87481=ADVANCED_FACE('',(#19161),#14479,.T.) ;
#87482=ADVANCED_FACE('',(#19162),#14480,.T.) ;
#87483=ADVANCED_FACE('',(#19163),#16392,.T.) ;
#87484=ADVANCED_FACE('',(#19164),#79187,.T.) ;
#87485=ADVANCED_FACE('',(#19165),#14481,.T.) ;
#87486=ADVANCED_FACE('',(#19166),#14482,.T.) ;
#87487=ADVANCED_FACE('',(#19167),#14483,.F.) ;
#87488=ADVANCED_FACE('',(#19168),#16393,.F.) ;
#87489=ADVANCED_FACE('',(#19169),#16394,.T.) ;
#87490=ADVANCED_FACE('',(#19170),#79188,.T.) ;
#87491=ADVANCED_FACE('',(#19171),#14484,.F.) ;
#87492=ADVANCED_FACE('',(#19172),#14485,.F.) ;
#87493=ADVANCED_FACE('',(#19173),#14486,.T.) ;
#87494=ADVANCED_FACE('',(#19174),#14487,.T.) ;
#87495=ADVANCED_FACE('',(#19175),#14488,.T.) ;
#87496=ADVANCED_FACE('',(#19176),#14489,.F.) ;
#87497=ADVANCED_FACE('',(#19177),#16395,.F.) ;
#87498=ADVANCED_FACE('',(#19178),#79189,.F.) ;
#87499=ADVANCED_FACE('',(#19179),#79190,.F.) ;
#87500=ADVANCED_FACE('',(#19180),#79191,.T.) ;
#87501=ADVANCED_FACE('',(#19181),#14490,.F.) ;
#87502=ADVANCED_FACE('',(#19182),#14491,.F.) ;
#87503=ADVANCED_FACE('',(#19183),#14492,.F.) ;
#87504=ADVANCED_FACE('',(#19184),#14493,.T.) ;
#87505=ADVANCED_FACE('',(#19185),#14494,.T.) ;
#87506=ADVANCED_FACE('',(#19186),#79192,.F.) ;
#87507=ADVANCED_FACE('',(#19187),#16396,.F.) ;
#87508=ADVANCED_FACE('',(#19188),#16397,.T.) ;
#87509=ADVANCED_FACE('',(#19189),#14495,.T.) ;
#87510=ADVANCED_FACE('',(#19190),#16398,.F.) ;
#87511=ADVANCED_FACE('',(#19191),#16399,.T.) ;
#87512=ADVANCED_FACE('',(#19192),#14496,.F.) ;
#87513=ADVANCED_FACE('',(#19193),#14497,.F.) ;
#87514=ADVANCED_FACE('',(#19194),#14498,.T.) ;
#87515=ADVANCED_FACE('',(#19195),#79193,.T.) ;
#87516=ADVANCED_FACE('',(#19196),#14499,.F.) ;
#87517=ADVANCED_FACE('',(#19197),#14500,.T.) ;
#87518=ADVANCED_FACE('',(#19198),#14501,.F.) ;
#87519=ADVANCED_FACE('',(#19199),#16400,.F.) ;
#87520=ADVANCED_FACE('',(#19200),#79194,.T.) ;
#87521=ADVANCED_FACE('',(#19201),#14502,.T.) ;
#87522=ADVANCED_FACE('',(#19202),#16401,.F.) ;
#87523=ADVANCED_FACE('',(#19203),#79195,.F.) ;
#87524=ADVANCED_FACE('',(#19204),#14503,.F.) ;
#87525=ADVANCED_FACE('',(#19205),#14504,.T.) ;
#87526=ADVANCED_FACE('',(#19206),#79196,.T.) ;
#87527=ADVANCED_FACE('',(#19207),#14505,.F.) ;
#87528=ADVANCED_FACE('',(#19208),#79197,.T.) ;
#87529=ADVANCED_FACE('',(#19209),#14506,.T.) ;
#87530=ADVANCED_FACE('',(#19210),#14507,.T.) ;
#87531=ADVANCED_FACE('',(#19211),#16402,.T.) ;
#87532=ADVANCED_FACE('',(#19212),#14508,.F.) ;
#87533=ADVANCED_FACE('',(#19213),#79198,.F.) ;
#87534=ADVANCED_FACE('',(#19214),#16403,.F.) ;
#87535=ADVANCED_FACE('',(#19215),#14509,.F.) ;
#87536=ADVANCED_FACE('',(#19216),#14510,.F.) ;
#87537=ADVANCED_FACE('',(#19217),#79199,.F.) ;
#87538=ADVANCED_FACE('',(#19218),#16404,.F.) ;
#87539=ADVANCED_FACE('',(#19219),#14511,.F.) ;
#87540=ADVANCED_FACE('',(#19220),#14512,.F.) ;
#87541=ADVANCED_FACE('',(#19221),#16405,.F.) ;
#87542=ADVANCED_FACE('',(#19222),#16406,.F.) ;
#87543=ADVANCED_FACE('',(#19223),#14513,.F.) ;
#87544=ADVANCED_FACE('',(#19224),#79200,.F.) ;
#87545=ADVANCED_FACE('',(#19225),#16407,.F.) ;
#87546=ADVANCED_FACE('',(#19226),#16408,.F.) ;
#87547=ADVANCED_FACE('',(#19227),#14514,.F.) ;
#87548=ADVANCED_FACE('',(#19228),#14515,.F.) ;
#87549=ADVANCED_FACE('',(#19229),#16409,.F.) ;
#87550=ADVANCED_FACE('',(#19230),#14516,.F.) ;
#87551=ADVANCED_FACE('',(#19231),#14517,.F.) ;
#87552=ADVANCED_FACE('',(#19232),#16410,.F.) ;
#87553=ADVANCED_FACE('',(#19233),#16411,.F.) ;
#87554=ADVANCED_FACE('',(#19234),#14518,.F.) ;
#87555=ADVANCED_FACE('',(#19235),#14519,.F.) ;
#87556=ADVANCED_FACE('',(#19236),#79201,.F.) ;
#87557=ADVANCED_FACE('',(#19237),#79202,.F.) ;
#87558=ADVANCED_FACE('',(#19238),#14520,.F.) ;
#87559=ADVANCED_FACE('',(#19239),#14521,.T.) ;
#87560=ADVANCED_FACE('',(#19240),#14522,.F.) ;
#87561=ADVANCED_FACE('',(#19241),#16412,.F.) ;
#87562=ADVANCED_FACE('',(#19242),#16413,.T.) ;
#87563=ADVANCED_FACE('',(#19243),#79203,.T.) ;
#87564=ADVANCED_FACE('',(#19244),#14523,.F.) ;
#87565=ADVANCED_FACE('',(#19245),#14524,.F.) ;
#87566=ADVANCED_FACE('',(#19246),#14525,.T.) ;
#87567=ADVANCED_FACE('',(#19247),#14526,.T.) ;
#87568=ADVANCED_FACE('',(#19248),#14527,.T.) ;
#87569=ADVANCED_FACE('',(#19249),#14528,.F.) ;
#87570=ADVANCED_FACE('',(#19250),#16414,.F.) ;
#87571=ADVANCED_FACE('',(#19251),#79204,.F.) ;
#87572=ADVANCED_FACE('',(#19252),#79205,.F.) ;
#87573=ADVANCED_FACE('',(#19253),#79206,.T.) ;
#87574=ADVANCED_FACE('',(#19254),#14529,.F.) ;
#87575=ADVANCED_FACE('',(#19255),#14530,.F.) ;
#87576=ADVANCED_FACE('',(#19256),#14531,.F.) ;
#87577=ADVANCED_FACE('',(#19257),#14532,.T.) ;
#87578=ADVANCED_FACE('',(#19258),#14533,.T.) ;
#87579=ADVANCED_FACE('',(#19259),#79207,.F.) ;
#87580=ADVANCED_FACE('',(#19260),#16415,.F.) ;
#87581=ADVANCED_FACE('',(#19261),#16416,.T.) ;
#87582=ADVANCED_FACE('',(#19262),#14534,.T.) ;
#87583=ADVANCED_FACE('',(#19263),#16417,.F.) ;
#87584=ADVANCED_FACE('',(#19264),#16418,.T.) ;
#87585=ADVANCED_FACE('',(#19265),#14535,.F.) ;
#87586=ADVANCED_FACE('',(#19266),#14536,.F.) ;
#87587=ADVANCED_FACE('',(#19267),#14537,.T.) ;
#87588=ADVANCED_FACE('',(#19268),#79208,.T.) ;
#87589=ADVANCED_FACE('',(#19269),#14538,.F.) ;
#87590=ADVANCED_FACE('',(#19270),#14539,.T.) ;
#87591=ADVANCED_FACE('',(#19271),#14540,.F.) ;
#87592=ADVANCED_FACE('',(#19272),#16419,.F.) ;
#87593=ADVANCED_FACE('',(#19273),#79209,.T.) ;
#87594=ADVANCED_FACE('',(#19274),#14541,.T.) ;
#87595=ADVANCED_FACE('',(#19275),#16420,.F.) ;
#87596=ADVANCED_FACE('',(#19276),#79210,.F.) ;
#87597=ADVANCED_FACE('',(#19277),#14542,.F.) ;
#87598=ADVANCED_FACE('',(#19278),#14543,.T.) ;
#87599=ADVANCED_FACE('',(#19279),#79211,.T.) ;
#87600=ADVANCED_FACE('',(#19280),#14544,.F.) ;
#87601=ADVANCED_FACE('',(#19281),#79212,.T.) ;
#87602=ADVANCED_FACE('',(#19282),#14545,.T.) ;
#87603=ADVANCED_FACE('',(#19283),#14546,.T.) ;
#87604=ADVANCED_FACE('',(#19284),#16421,.T.) ;
#87605=ADVANCED_FACE('',(#19285),#14547,.F.) ;
#87606=ADVANCED_FACE('',(#19286),#79213,.F.) ;
#87607=ADVANCED_FACE('',(#19287),#16422,.F.) ;
#87608=ADVANCED_FACE('',(#19288),#14548,.F.) ;
#87609=ADVANCED_FACE('',(#19289),#14549,.F.) ;
#87610=ADVANCED_FACE('',(#19290),#79214,.F.) ;
#87611=ADVANCED_FACE('',(#19291),#16423,.F.) ;
#87612=ADVANCED_FACE('',(#19292),#14550,.F.) ;
#87613=ADVANCED_FACE('',(#19293),#14551,.F.) ;
#87614=ADVANCED_FACE('',(#19294),#16424,.F.) ;
#87615=ADVANCED_FACE('',(#19295),#16425,.F.) ;
#87616=ADVANCED_FACE('',(#19296),#14552,.F.) ;
#87617=ADVANCED_FACE('',(#19297),#79215,.F.) ;
#87618=ADVANCED_FACE('',(#19298),#16426,.F.) ;
#87619=ADVANCED_FACE('',(#19299),#16427,.F.) ;
#87620=ADVANCED_FACE('',(#19300),#14553,.F.) ;
#87621=ADVANCED_FACE('',(#19301),#14554,.F.) ;
#87622=ADVANCED_FACE('',(#19302),#16428,.F.) ;
#87623=ADVANCED_FACE('',(#19303),#14555,.F.) ;
#87624=ADVANCED_FACE('',(#19304),#14556,.F.) ;
#87625=ADVANCED_FACE('',(#19305),#16429,.F.) ;
#87626=ADVANCED_FACE('',(#19306),#16430,.F.) ;
#87627=ADVANCED_FACE('',(#19307),#14557,.F.) ;
#87628=ADVANCED_FACE('',(#19308),#14558,.F.) ;
#87629=ADVANCED_FACE('',(#19309),#79216,.F.) ;
#87630=ADVANCED_FACE('',(#19310),#79217,.F.) ;
#87631=ADVANCED_FACE('',(#19311),#14559,.F.) ;
#87632=ADVANCED_FACE('',(#19312),#14560,.T.) ;
#87633=ADVANCED_FACE('',(#19313),#14561,.F.) ;
#87634=ADVANCED_FACE('',(#19314),#16431,.F.) ;
#87635=ADVANCED_FACE('',(#19315),#16432,.T.) ;
#87636=ADVANCED_FACE('',(#19316),#79218,.T.) ;
#87637=ADVANCED_FACE('',(#19317),#14562,.F.) ;
#87638=ADVANCED_FACE('',(#19318),#14563,.F.) ;
#87639=ADVANCED_FACE('',(#19319),#14564,.T.) ;
#87640=ADVANCED_FACE('',(#19320),#14565,.T.) ;
#87641=ADVANCED_FACE('',(#19321),#14566,.T.) ;
#87642=ADVANCED_FACE('',(#19322),#14567,.F.) ;
#87643=ADVANCED_FACE('',(#19323),#16433,.F.) ;
#87644=ADVANCED_FACE('',(#19324),#79219,.F.) ;
#87645=ADVANCED_FACE('',(#19325),#79220,.F.) ;
#87646=ADVANCED_FACE('',(#19326),#79221,.T.) ;
#87647=ADVANCED_FACE('',(#19327),#14568,.F.) ;
#87648=ADVANCED_FACE('',(#19328),#14569,.F.) ;
#87649=ADVANCED_FACE('',(#19329),#14570,.F.) ;
#87650=ADVANCED_FACE('',(#19330),#14571,.T.) ;
#87651=ADVANCED_FACE('',(#19331),#14572,.T.) ;
#87652=ADVANCED_FACE('',(#19332),#79222,.F.) ;
#87653=ADVANCED_FACE('',(#19333),#16434,.F.) ;
#87654=ADVANCED_FACE('',(#19334),#16435,.T.) ;
#87655=ADVANCED_FACE('',(#19335),#14573,.T.) ;
#87656=ADVANCED_FACE('',(#19336),#16436,.F.) ;
#87657=ADVANCED_FACE('',(#19337),#16437,.T.) ;
#87658=ADVANCED_FACE('',(#19338),#14574,.F.) ;
#87659=ADVANCED_FACE('',(#19339),#14575,.F.) ;
#87660=ADVANCED_FACE('',(#19340),#14576,.T.) ;
#87661=ADVANCED_FACE('',(#19341),#79223,.T.) ;
#87662=ADVANCED_FACE('',(#19342),#14577,.F.) ;
#87663=ADVANCED_FACE('',(#19343),#14578,.T.) ;
#87664=ADVANCED_FACE('',(#19344),#14579,.F.) ;
#87665=ADVANCED_FACE('',(#19345),#16438,.F.) ;
#87666=ADVANCED_FACE('',(#19346),#79224,.T.) ;
#87667=ADVANCED_FACE('',(#19347),#14580,.T.) ;
#87668=ADVANCED_FACE('',(#19348),#16439,.F.) ;
#87669=ADVANCED_FACE('',(#19349),#79225,.F.) ;
#87670=ADVANCED_FACE('',(#19350),#14581,.F.) ;
#87671=ADVANCED_FACE('',(#19351),#14582,.T.) ;
#87672=ADVANCED_FACE('',(#19352),#79226,.T.) ;
#87673=ADVANCED_FACE('',(#19353),#14583,.F.) ;
#87674=ADVANCED_FACE('',(#19354),#79227,.T.) ;
#87675=ADVANCED_FACE('',(#19355),#14584,.T.) ;
#87676=ADVANCED_FACE('',(#19356),#14585,.T.) ;
#87677=ADVANCED_FACE('',(#19357),#16440,.T.) ;
#87678=ADVANCED_FACE('',(#19358),#14586,.F.) ;
#87679=ADVANCED_FACE('',(#19359),#79228,.F.) ;
#87680=ADVANCED_FACE('',(#19360),#16441,.F.) ;
#87681=ADVANCED_FACE('',(#19361),#14587,.F.) ;
#87682=ADVANCED_FACE('',(#19362),#14588,.F.) ;
#87683=ADVANCED_FACE('',(#19363),#79229,.F.) ;
#87684=ADVANCED_FACE('',(#19364),#16442,.F.) ;
#87685=ADVANCED_FACE('',(#19365),#14589,.F.) ;
#87686=ADVANCED_FACE('',(#19366),#14590,.F.) ;
#87687=ADVANCED_FACE('',(#19367),#16443,.F.) ;
#87688=ADVANCED_FACE('',(#19368),#16444,.F.) ;
#87689=ADVANCED_FACE('',(#19369),#14591,.F.) ;
#87690=ADVANCED_FACE('',(#19370),#79230,.F.) ;
#87691=ADVANCED_FACE('',(#19371),#16445,.F.) ;
#87692=ADVANCED_FACE('',(#19372),#16446,.F.) ;
#87693=ADVANCED_FACE('',(#19373),#14592,.F.) ;
#87694=ADVANCED_FACE('',(#19374),#14593,.F.) ;
#87695=ADVANCED_FACE('',(#19375),#16447,.F.) ;
#87696=ADVANCED_FACE('',(#19376),#14594,.F.) ;
#87697=ADVANCED_FACE('',(#19377),#14595,.F.) ;
#87698=ADVANCED_FACE('',(#19378),#16448,.F.) ;
#87699=ADVANCED_FACE('',(#19379),#16449,.F.) ;
#87700=ADVANCED_FACE('',(#19380),#14596,.F.) ;
#87701=ADVANCED_FACE('',(#19381),#14597,.F.) ;
#87702=ADVANCED_FACE('',(#19382),#79231,.F.) ;
#87703=ADVANCED_FACE('',(#19383),#79232,.F.) ;
#87704=ADVANCED_FACE('',(#19384),#14598,.F.) ;
#87705=ADVANCED_FACE('',(#19385),#14599,.T.) ;
#87706=ADVANCED_FACE('',(#19386),#14600,.F.) ;
#87707=ADVANCED_FACE('',(#19387),#16450,.F.) ;
#87708=ADVANCED_FACE('',(#19388),#16451,.T.) ;
#87709=ADVANCED_FACE('',(#19389),#79233,.T.) ;
#87710=ADVANCED_FACE('',(#19390),#14601,.F.) ;
#87711=ADVANCED_FACE('',(#19391),#14602,.F.) ;
#87712=ADVANCED_FACE('',(#19392),#14603,.T.) ;
#87713=ADVANCED_FACE('',(#19393),#14604,.T.) ;
#87714=ADVANCED_FACE('',(#19394),#14605,.T.) ;
#87715=ADVANCED_FACE('',(#19395),#14606,.F.) ;
#87716=ADVANCED_FACE('',(#19396),#16452,.F.) ;
#87717=ADVANCED_FACE('',(#19397),#79234,.F.) ;
#87718=ADVANCED_FACE('',(#19398),#79235,.F.) ;
#87719=ADVANCED_FACE('',(#19399),#79236,.T.) ;
#87720=ADVANCED_FACE('',(#19400),#14607,.F.) ;
#87721=ADVANCED_FACE('',(#19401),#14608,.F.) ;
#87722=ADVANCED_FACE('',(#19402),#14609,.F.) ;
#87723=ADVANCED_FACE('',(#19403),#14610,.T.) ;
#87724=ADVANCED_FACE('',(#19404),#14611,.T.) ;
#87725=ADVANCED_FACE('',(#19405),#79237,.F.) ;
#87726=ADVANCED_FACE('',(#19406),#16453,.F.) ;
#87727=ADVANCED_FACE('',(#19407),#16454,.T.) ;
#87728=ADVANCED_FACE('',(#19408),#14612,.T.) ;
#87729=ADVANCED_FACE('',(#19409),#16455,.F.) ;
#87730=ADVANCED_FACE('',(#19410),#16456,.T.) ;
#87731=ADVANCED_FACE('',(#19411),#14613,.F.) ;
#87732=ADVANCED_FACE('',(#19412),#14614,.F.) ;
#87733=ADVANCED_FACE('',(#19413),#14615,.T.) ;
#87734=ADVANCED_FACE('',(#19414),#79238,.T.) ;
#87735=ADVANCED_FACE('',(#19415),#14616,.F.) ;
#87736=ADVANCED_FACE('',(#19416),#14617,.T.) ;
#87737=ADVANCED_FACE('',(#19417),#14618,.F.) ;
#87738=ADVANCED_FACE('',(#19418),#16457,.F.) ;
#87739=ADVANCED_FACE('',(#19419),#79239,.T.) ;
#87740=ADVANCED_FACE('',(#19420),#14619,.T.) ;
#87741=ADVANCED_FACE('',(#19421),#16458,.F.) ;
#87742=ADVANCED_FACE('',(#19422),#79240,.F.) ;
#87743=ADVANCED_FACE('',(#19423),#14620,.F.) ;
#87744=ADVANCED_FACE('',(#19424),#14621,.T.) ;
#87745=ADVANCED_FACE('',(#19425),#79241,.T.) ;
#87746=ADVANCED_FACE('',(#19426),#14622,.F.) ;
#87747=ADVANCED_FACE('',(#19427),#79242,.T.) ;
#87748=ADVANCED_FACE('',(#19428),#14623,.T.) ;
#87749=ADVANCED_FACE('',(#19429),#14624,.T.) ;
#87750=ADVANCED_FACE('',(#19430),#16459,.T.) ;
#87751=ADVANCED_FACE('',(#19431),#14625,.F.) ;
#87752=ADVANCED_FACE('',(#19432),#79243,.F.) ;
#87753=ADVANCED_FACE('',(#19433),#16460,.F.) ;
#87754=ADVANCED_FACE('',(#19434),#14626,.F.) ;
#87755=ADVANCED_FACE('',(#19435),#14627,.F.) ;
#87756=ADVANCED_FACE('',(#19436),#79244,.F.) ;
#87757=ADVANCED_FACE('',(#19437),#16461,.F.) ;
#87758=ADVANCED_FACE('',(#19438),#14628,.F.) ;
#87759=ADVANCED_FACE('',(#19439),#14629,.F.) ;
#87760=ADVANCED_FACE('',(#19440),#16462,.F.) ;
#87761=ADVANCED_FACE('',(#19441),#16463,.F.) ;
#87762=ADVANCED_FACE('',(#19442),#14630,.F.) ;
#87763=ADVANCED_FACE('',(#19443),#79245,.F.) ;
#87764=ADVANCED_FACE('',(#19444),#16464,.F.) ;
#87765=ADVANCED_FACE('',(#19445),#16465,.F.) ;
#87766=ADVANCED_FACE('',(#19446),#14631,.F.) ;
#87767=ADVANCED_FACE('',(#19447),#14632,.F.) ;
#87768=ADVANCED_FACE('',(#19448),#16466,.F.) ;
#87769=ADVANCED_FACE('',(#19449),#14633,.F.) ;
#87770=ADVANCED_FACE('',(#19450),#14634,.F.) ;
#87771=ADVANCED_FACE('',(#19451),#16467,.F.) ;
#87772=ADVANCED_FACE('',(#19452),#16468,.F.) ;
#87773=ADVANCED_FACE('',(#19453),#14635,.F.) ;
#87774=ADVANCED_FACE('',(#19454),#14636,.F.) ;
#87775=ADVANCED_FACE('',(#19455),#79246,.F.) ;
#87776=ADVANCED_FACE('',(#19456),#79247,.F.) ;
#87777=ADVANCED_FACE('',(#19457),#14637,.F.) ;
#87778=ADVANCED_FACE('',(#19458),#14638,.T.) ;
#87779=ADVANCED_FACE('',(#19459),#14639,.F.) ;
#87780=ADVANCED_FACE('',(#19460),#16469,.F.) ;
#87781=ADVANCED_FACE('',(#19461),#16470,.T.) ;
#87782=ADVANCED_FACE('',(#19462),#79248,.T.) ;
#87783=ADVANCED_FACE('',(#19463),#14640,.F.) ;
#87784=ADVANCED_FACE('',(#19464),#14641,.F.) ;
#87785=ADVANCED_FACE('',(#19465),#14642,.T.) ;
#87786=ADVANCED_FACE('',(#19466),#14643,.T.) ;
#87787=ADVANCED_FACE('',(#19467),#14644,.T.) ;
#87788=ADVANCED_FACE('',(#19468),#14645,.F.) ;
#87789=ADVANCED_FACE('',(#19469),#16471,.F.) ;
#87790=ADVANCED_FACE('',(#19470),#79249,.F.) ;
#87791=ADVANCED_FACE('',(#19471),#79250,.F.) ;
#87792=ADVANCED_FACE('',(#19472),#79251,.T.) ;
#87793=ADVANCED_FACE('',(#19473),#14646,.F.) ;
#87794=ADVANCED_FACE('',(#19474),#14647,.F.) ;
#87795=ADVANCED_FACE('',(#19475),#14648,.F.) ;
#87796=ADVANCED_FACE('',(#19476),#14649,.T.) ;
#87797=ADVANCED_FACE('',(#19477),#14650,.T.) ;
#87798=ADVANCED_FACE('',(#19478),#79252,.F.) ;
#87799=ADVANCED_FACE('',(#19479),#16472,.F.) ;
#87800=ADVANCED_FACE('',(#19480),#16473,.T.) ;
#87801=ADVANCED_FACE('',(#19481),#14651,.T.) ;
#87802=ADVANCED_FACE('',(#19482),#16474,.F.) ;
#87803=ADVANCED_FACE('',(#19483),#16475,.T.) ;
#87804=ADVANCED_FACE('',(#19484),#14652,.F.) ;
#87805=ADVANCED_FACE('',(#19485),#14653,.F.) ;
#87806=ADVANCED_FACE('',(#19486),#14654,.T.) ;
#87807=ADVANCED_FACE('',(#19487),#79253,.T.) ;
#87808=ADVANCED_FACE('',(#19488),#14655,.F.) ;
#87809=ADVANCED_FACE('',(#19489),#14656,.T.) ;
#87810=ADVANCED_FACE('',(#19490),#14657,.F.) ;
#87811=ADVANCED_FACE('',(#19491),#16476,.F.) ;
#87812=ADVANCED_FACE('',(#19492),#79254,.T.) ;
#87813=ADVANCED_FACE('',(#19493),#14658,.T.) ;
#87814=ADVANCED_FACE('',(#19494),#16477,.F.) ;
#87815=ADVANCED_FACE('',(#19495),#79255,.F.) ;
#87816=ADVANCED_FACE('',(#19496),#14659,.F.) ;
#87817=ADVANCED_FACE('',(#19497),#14660,.T.) ;
#87818=ADVANCED_FACE('',(#19498),#79256,.T.) ;
#87819=ADVANCED_FACE('',(#19499),#14661,.F.) ;
#87820=ADVANCED_FACE('',(#19500),#79257,.T.) ;
#87821=ADVANCED_FACE('',(#19501),#14662,.T.) ;
#87822=ADVANCED_FACE('',(#19502),#14663,.T.) ;
#87823=ADVANCED_FACE('',(#19503),#16478,.T.) ;
#87824=ADVANCED_FACE('',(#19504),#14664,.F.) ;
#87825=ADVANCED_FACE('',(#19505),#79258,.F.) ;
#87826=ADVANCED_FACE('',(#19506),#16479,.F.) ;
#87827=ADVANCED_FACE('',(#19507),#14665,.F.) ;
#87828=ADVANCED_FACE('',(#19508),#14666,.F.) ;
#87829=ADVANCED_FACE('',(#19509),#79259,.F.) ;
#87830=ADVANCED_FACE('',(#19510),#16480,.F.) ;
#87831=ADVANCED_FACE('',(#19511),#14667,.F.) ;
#87832=ADVANCED_FACE('',(#19512),#14668,.F.) ;
#87833=ADVANCED_FACE('',(#19513),#16481,.F.) ;
#87834=ADVANCED_FACE('',(#19514),#16482,.F.) ;
#87835=ADVANCED_FACE('',(#19515),#14669,.F.) ;
#87836=ADVANCED_FACE('',(#19516),#79260,.F.) ;
#87837=ADVANCED_FACE('',(#19517),#16483,.F.) ;
#87838=ADVANCED_FACE('',(#19518),#16484,.F.) ;
#87839=ADVANCED_FACE('',(#19519),#14670,.F.) ;
#87840=ADVANCED_FACE('',(#19520),#14671,.F.) ;
#87841=ADVANCED_FACE('',(#19521),#16485,.F.) ;
#87842=ADVANCED_FACE('',(#19522),#14672,.F.) ;
#87843=ADVANCED_FACE('',(#19523),#14673,.F.) ;
#87844=ADVANCED_FACE('',(#19524),#16486,.F.) ;
#87845=ADVANCED_FACE('',(#19525),#16487,.F.) ;
#87846=ADVANCED_FACE('',(#19526),#14674,.F.) ;
#87847=ADVANCED_FACE('',(#19527),#14675,.F.) ;
#87848=ADVANCED_FACE('',(#19528),#79261,.F.) ;
#87849=ADVANCED_FACE('',(#19529),#79262,.F.) ;
#87850=ADVANCED_FACE('',(#19530),#14676,.F.) ;
#87851=ADVANCED_FACE('',(#19531),#14677,.T.) ;
#87852=ADVANCED_FACE('',(#19532),#14678,.F.) ;
#87853=ADVANCED_FACE('',(#19533),#16488,.F.) ;
#87854=ADVANCED_FACE('',(#19534),#16489,.T.) ;
#87855=ADVANCED_FACE('',(#19535),#79263,.T.) ;
#87856=ADVANCED_FACE('',(#19536),#14679,.F.) ;
#87857=ADVANCED_FACE('',(#19537),#14680,.F.) ;
#87858=ADVANCED_FACE('',(#19538),#14681,.T.) ;
#87859=ADVANCED_FACE('',(#19539),#14682,.T.) ;
#87860=ADVANCED_FACE('',(#19540),#14683,.T.) ;
#87861=ADVANCED_FACE('',(#19541),#14684,.F.) ;
#87862=ADVANCED_FACE('',(#19542),#16490,.F.) ;
#87863=ADVANCED_FACE('',(#19543),#79264,.F.) ;
#87864=ADVANCED_FACE('',(#19544),#79265,.F.) ;
#87865=ADVANCED_FACE('',(#19545),#79266,.T.) ;
#87866=ADVANCED_FACE('',(#19546),#14685,.F.) ;
#87867=ADVANCED_FACE('',(#19547),#14686,.F.) ;
#87868=ADVANCED_FACE('',(#19548),#14687,.F.) ;
#87869=ADVANCED_FACE('',(#19549),#14688,.T.) ;
#87870=ADVANCED_FACE('',(#19550),#14689,.T.) ;
#87871=ADVANCED_FACE('',(#19551),#79267,.F.) ;
#87872=ADVANCED_FACE('',(#19552),#16491,.F.) ;
#87873=ADVANCED_FACE('',(#19553),#16492,.T.) ;
#87874=ADVANCED_FACE('',(#19554),#14690,.T.) ;
#87875=ADVANCED_FACE('',(#19555),#16493,.F.) ;
#87876=ADVANCED_FACE('',(#19556),#16494,.T.) ;
#87877=ADVANCED_FACE('',(#19557),#14691,.F.) ;
#87878=ADVANCED_FACE('',(#19558),#14692,.F.) ;
#87879=ADVANCED_FACE('',(#19559),#14693,.T.) ;
#87880=ADVANCED_FACE('',(#19560),#79268,.T.) ;
#87881=ADVANCED_FACE('',(#19561),#14694,.F.) ;
#87882=ADVANCED_FACE('',(#19562),#14695,.T.) ;
#87883=ADVANCED_FACE('',(#19563),#14696,.F.) ;
#87884=ADVANCED_FACE('',(#19564),#16495,.F.) ;
#87885=ADVANCED_FACE('',(#19565),#79269,.T.) ;
#87886=ADVANCED_FACE('',(#19566),#14697,.T.) ;
#87887=ADVANCED_FACE('',(#19567),#16496,.F.) ;
#87888=ADVANCED_FACE('',(#19568),#79270,.F.) ;
#87889=ADVANCED_FACE('',(#19569),#14698,.F.) ;
#87890=ADVANCED_FACE('',(#19570),#14699,.T.) ;
#87891=ADVANCED_FACE('',(#19571),#79271,.T.) ;
#87892=ADVANCED_FACE('',(#19572),#14700,.F.) ;
#87893=ADVANCED_FACE('',(#19573),#79272,.T.) ;
#87894=ADVANCED_FACE('',(#19574),#14701,.T.) ;
#87895=ADVANCED_FACE('',(#19575),#14702,.T.) ;
#87896=ADVANCED_FACE('',(#19576),#16497,.T.) ;
#87897=ADVANCED_FACE('',(#19577),#14703,.F.) ;
#87898=ADVANCED_FACE('',(#19578),#79273,.F.) ;
#87899=ADVANCED_FACE('',(#19579),#16498,.F.) ;
#87900=ADVANCED_FACE('',(#19580),#14704,.F.) ;
#87901=ADVANCED_FACE('',(#19581),#14705,.F.) ;
#87902=ADVANCED_FACE('',(#19582),#79274,.F.) ;
#87903=ADVANCED_FACE('',(#19583),#16499,.F.) ;
#87904=ADVANCED_FACE('',(#19584),#14706,.F.) ;
#87905=ADVANCED_FACE('',(#19585),#14707,.F.) ;
#87906=ADVANCED_FACE('',(#19586),#16500,.F.) ;
#87907=ADVANCED_FACE('',(#19587),#16501,.F.) ;
#87908=ADVANCED_FACE('',(#19588),#14708,.F.) ;
#87909=ADVANCED_FACE('',(#19589),#79275,.F.) ;
#87910=ADVANCED_FACE('',(#19590),#16502,.F.) ;
#87911=ADVANCED_FACE('',(#19591),#16503,.F.) ;
#87912=ADVANCED_FACE('',(#19592),#14709,.F.) ;
#87913=ADVANCED_FACE('',(#19593),#14710,.F.) ;
#87914=ADVANCED_FACE('',(#19594),#16504,.F.) ;
#87915=ADVANCED_FACE('',(#19595),#14711,.F.) ;
#87916=ADVANCED_FACE('',(#19596),#14712,.F.) ;
#87917=ADVANCED_FACE('',(#19597),#16505,.F.) ;
#87918=ADVANCED_FACE('',(#19598),#16506,.F.) ;
#87919=ADVANCED_FACE('',(#19599),#14713,.F.) ;
#87920=ADVANCED_FACE('',(#19600),#14714,.F.) ;
#87921=ADVANCED_FACE('',(#19601),#79276,.F.) ;
#87922=ADVANCED_FACE('',(#19602),#79277,.F.) ;
#87923=ADVANCED_FACE('',(#19603),#14715,.F.) ;
#87924=ADVANCED_FACE('',(#19604),#14716,.T.) ;
#87925=ADVANCED_FACE('',(#19605),#14717,.F.) ;
#87926=ADVANCED_FACE('',(#19606),#16507,.F.) ;
#87927=ADVANCED_FACE('',(#19607),#16508,.T.) ;
#87928=ADVANCED_FACE('',(#19608),#79278,.T.) ;
#87929=ADVANCED_FACE('',(#19609),#14718,.F.) ;
#87930=ADVANCED_FACE('',(#19610),#14719,.F.) ;
#87931=ADVANCED_FACE('',(#19611),#14720,.T.) ;
#87932=ADVANCED_FACE('',(#19612),#14721,.T.) ;
#87933=ADVANCED_FACE('',(#19613),#14722,.T.) ;
#87934=ADVANCED_FACE('',(#19614),#14723,.F.) ;
#87935=ADVANCED_FACE('',(#19615),#16509,.F.) ;
#87936=ADVANCED_FACE('',(#19616),#79279,.F.) ;
#87937=ADVANCED_FACE('',(#19617),#79280,.F.) ;
#87938=ADVANCED_FACE('',(#19618),#79281,.T.) ;
#87939=ADVANCED_FACE('',(#19619),#14724,.F.) ;
#87940=ADVANCED_FACE('',(#19620),#14725,.F.) ;
#87941=ADVANCED_FACE('',(#19621),#14726,.F.) ;
#87942=ADVANCED_FACE('',(#19622),#14727,.T.) ;
#87943=ADVANCED_FACE('',(#19623),#14728,.T.) ;
#87944=ADVANCED_FACE('',(#19624),#79282,.F.) ;
#87945=ADVANCED_FACE('',(#19625),#16510,.F.) ;
#87946=ADVANCED_FACE('',(#19626),#16511,.T.) ;
#87947=ADVANCED_FACE('',(#19627),#14729,.T.) ;
#87948=ADVANCED_FACE('',(#19628),#16512,.F.) ;
#87949=ADVANCED_FACE('',(#19629),#16513,.T.) ;
#87950=ADVANCED_FACE('',(#19630),#14730,.F.) ;
#87951=ADVANCED_FACE('',(#19631),#14731,.F.) ;
#87952=ADVANCED_FACE('',(#19632),#14732,.T.) ;
#87953=ADVANCED_FACE('',(#19633),#79283,.T.) ;
#87954=ADVANCED_FACE('',(#19634),#14733,.F.) ;
#87955=ADVANCED_FACE('',(#19635),#14734,.T.) ;
#87956=ADVANCED_FACE('',(#19636),#14735,.F.) ;
#87957=ADVANCED_FACE('',(#19637),#16514,.F.) ;
#87958=ADVANCED_FACE('',(#19638),#79284,.T.) ;
#87959=ADVANCED_FACE('',(#19639),#14736,.T.) ;
#87960=ADVANCED_FACE('',(#19640),#16515,.F.) ;
#87961=ADVANCED_FACE('',(#19641),#79285,.F.) ;
#87962=ADVANCED_FACE('',(#19642),#14737,.F.) ;
#87963=ADVANCED_FACE('',(#19643),#14738,.T.) ;
#87964=ADVANCED_FACE('',(#19644),#79286,.T.) ;
#87965=ADVANCED_FACE('',(#19645),#14739,.F.) ;
#87966=ADVANCED_FACE('',(#19646),#79287,.T.) ;
#87967=ADVANCED_FACE('',(#19647),#14740,.T.) ;
#87968=ADVANCED_FACE('',(#19648),#14741,.T.) ;
#87969=ADVANCED_FACE('',(#19649),#16516,.T.) ;
#87970=ADVANCED_FACE('',(#19650),#14742,.F.) ;
#87971=ADVANCED_FACE('',(#19651),#79288,.F.) ;
#87972=ADVANCED_FACE('',(#19652),#16517,.F.) ;
#87973=ADVANCED_FACE('',(#19653),#14743,.F.) ;
#87974=ADVANCED_FACE('',(#19654),#14744,.F.) ;
#87975=ADVANCED_FACE('',(#19655),#79289,.F.) ;
#87976=ADVANCED_FACE('',(#19656),#16518,.F.) ;
#87977=ADVANCED_FACE('',(#19657),#14745,.F.) ;
#87978=ADVANCED_FACE('',(#19658),#14746,.F.) ;
#87979=ADVANCED_FACE('',(#19659),#16519,.F.) ;
#87980=ADVANCED_FACE('',(#19660),#16520,.F.) ;
#87981=ADVANCED_FACE('',(#19661),#14747,.F.) ;
#87982=ADVANCED_FACE('',(#19662),#79290,.F.) ;
#87983=ADVANCED_FACE('',(#19663),#16521,.F.) ;
#87984=ADVANCED_FACE('',(#19664),#16522,.F.) ;
#87985=ADVANCED_FACE('',(#19665),#14748,.F.) ;
#87986=ADVANCED_FACE('',(#19666),#14749,.F.) ;
#87987=ADVANCED_FACE('',(#19667),#16523,.F.) ;
#87988=ADVANCED_FACE('',(#19668),#14750,.F.) ;
#87989=ADVANCED_FACE('',(#19669),#14751,.F.) ;
#87990=ADVANCED_FACE('',(#19670),#16524,.F.) ;
#87991=ADVANCED_FACE('',(#19671),#16525,.F.) ;
#87992=ADVANCED_FACE('',(#19672),#14752,.F.) ;
#87993=ADVANCED_FACE('',(#19673),#14753,.F.) ;
#87994=ADVANCED_FACE('',(#19674),#79291,.F.) ;
#87995=ADVANCED_FACE('',(#19675),#79292,.F.) ;
#87996=ADVANCED_FACE('',(#19676),#14754,.F.) ;
#87997=ADVANCED_FACE('',(#19677),#14755,.T.) ;
#87998=ADVANCED_FACE('',(#19678),#14756,.F.) ;
#87999=ADVANCED_FACE('',(#19679),#16526,.F.) ;
#88000=ADVANCED_FACE('',(#19680),#16527,.T.) ;
#88001=ADVANCED_FACE('',(#19681),#79293,.T.) ;
#88002=ADVANCED_FACE('',(#19682),#14757,.F.) ;
#88003=ADVANCED_FACE('',(#19683),#14758,.F.) ;
#88004=ADVANCED_FACE('',(#19684),#14759,.T.) ;
#88005=ADVANCED_FACE('',(#19685),#14760,.T.) ;
#88006=ADVANCED_FACE('',(#19686),#14761,.T.) ;
#88007=ADVANCED_FACE('',(#19687),#14762,.F.) ;
#88008=ADVANCED_FACE('',(#19688),#16528,.F.) ;
#88009=ADVANCED_FACE('',(#19689),#79294,.F.) ;
#88010=ADVANCED_FACE('',(#19690),#79295,.F.) ;
#88011=ADVANCED_FACE('',(#19691),#79296,.T.) ;
#88012=ADVANCED_FACE('',(#19692),#14763,.F.) ;
#88013=ADVANCED_FACE('',(#19693),#14764,.F.) ;
#88014=ADVANCED_FACE('',(#19694),#14765,.F.) ;
#88015=ADVANCED_FACE('',(#19695),#14766,.T.) ;
#88016=ADVANCED_FACE('',(#19696),#14767,.T.) ;
#88017=ADVANCED_FACE('',(#19697),#79297,.F.) ;
#88018=ADVANCED_FACE('',(#19698),#16529,.F.) ;
#88019=ADVANCED_FACE('',(#19699),#16530,.T.) ;
#88020=ADVANCED_FACE('',(#19700),#14768,.T.) ;
#88021=ADVANCED_FACE('',(#19701),#16531,.F.) ;
#88022=ADVANCED_FACE('',(#19702),#16532,.T.) ;
#88023=ADVANCED_FACE('',(#19703),#14769,.F.) ;
#88024=ADVANCED_FACE('',(#19704),#14770,.F.) ;
#88025=ADVANCED_FACE('',(#19705),#14771,.T.) ;
#88026=ADVANCED_FACE('',(#19706),#79298,.T.) ;
#88027=ADVANCED_FACE('',(#19707),#14772,.F.) ;
#88028=ADVANCED_FACE('',(#19708),#14773,.T.) ;
#88029=ADVANCED_FACE('',(#19709),#14774,.F.) ;
#88030=ADVANCED_FACE('',(#19710),#16533,.F.) ;
#88031=ADVANCED_FACE('',(#19711),#79299,.T.) ;
#88032=ADVANCED_FACE('',(#19712),#14775,.T.) ;
#88033=ADVANCED_FACE('',(#19713),#16534,.F.) ;
#88034=ADVANCED_FACE('',(#19714),#79300,.F.) ;
#88035=ADVANCED_FACE('',(#19715),#14776,.F.) ;
#88036=ADVANCED_FACE('',(#19716),#14777,.T.) ;
#88037=ADVANCED_FACE('',(#19717),#79301,.T.) ;
#88038=ADVANCED_FACE('',(#19718),#14778,.F.) ;
#88039=ADVANCED_FACE('',(#19719),#79302,.T.) ;
#88040=ADVANCED_FACE('',(#19720),#14779,.T.) ;
#88041=ADVANCED_FACE('',(#19721),#14780,.T.) ;
#88042=ADVANCED_FACE('',(#19722),#16535,.T.) ;
#88043=ADVANCED_FACE('',(#19723),#14781,.F.) ;
#88044=ADVANCED_FACE('',(#19724),#79303,.F.) ;
#88045=ADVANCED_FACE('',(#19725),#16536,.F.) ;
#88046=ADVANCED_FACE('',(#19726),#14782,.F.) ;
#88047=ADVANCED_FACE('',(#19727),#14783,.F.) ;
#88048=ADVANCED_FACE('',(#19728),#79304,.F.) ;
#88049=ADVANCED_FACE('',(#19729),#16537,.F.) ;
#88050=ADVANCED_FACE('',(#19730),#14784,.F.) ;
#88051=ADVANCED_FACE('',(#19731),#14785,.F.) ;
#88052=ADVANCED_FACE('',(#19732),#16538,.F.) ;
#88053=ADVANCED_FACE('',(#19733),#16539,.F.) ;
#88054=ADVANCED_FACE('',(#19734),#14786,.F.) ;
#88055=ADVANCED_FACE('',(#19735),#79305,.F.) ;
#88056=ADVANCED_FACE('',(#19736),#16540,.F.) ;
#88057=ADVANCED_FACE('',(#19737),#16541,.F.) ;
#88058=ADVANCED_FACE('',(#19738),#14787,.F.) ;
#88059=ADVANCED_FACE('',(#19739),#14788,.F.) ;
#88060=ADVANCED_FACE('',(#19740),#16542,.F.) ;
#88061=ADVANCED_FACE('',(#19741),#14789,.F.) ;
#88062=ADVANCED_FACE('',(#19742),#14790,.F.) ;
#88063=ADVANCED_FACE('',(#19743),#16543,.F.) ;
#88064=ADVANCED_FACE('',(#19744),#16544,.F.) ;
#88065=ADVANCED_FACE('',(#19745),#14791,.F.) ;
#88066=ADVANCED_FACE('',(#19746),#14792,.F.) ;
#88067=ADVANCED_FACE('',(#19747),#79306,.F.) ;
#88068=ADVANCED_FACE('',(#19748),#79307,.F.) ;
#88069=ADVANCED_FACE('',(#19749),#14793,.F.) ;
#88070=ADVANCED_FACE('',(#19750),#1351,.F.) ;
#88071=ADVANCED_FACE('',(#19751),#1352,.F.) ;
#88072=ADVANCED_FACE('',(#19752),#1353,.F.) ;
#88073=ADVANCED_FACE('',(#19753),#1354,.F.) ;
#88074=ADVANCED_FACE('',(#19754),#1355,.F.) ;
#88075=ADVANCED_FACE('',(#19755),#1356,.T.) ;
#88076=ADVANCED_FACE('',(#19756),#1357,.F.) ;
#88077=ADVANCED_FACE('',(#19757),#14794,.T.) ;
#88078=ADVANCED_FACE('',(#19758),#14795,.F.) ;
#88079=ADVANCED_FACE('',(#19759),#1358,.F.) ;
#88080=ADVANCED_FACE('',(#19760),#1359,.F.) ;
#88081=ADVANCED_FACE('',(#19761),#1360,.F.) ;
#88082=ADVANCED_FACE('',(#19762),#1361,.F.) ;
#88083=ADVANCED_FACE('',(#19763),#1362,.F.) ;
#88084=ADVANCED_FACE('',(#19764),#1363,.T.) ;
#88085=ADVANCED_FACE('',(#19765),#1364,.F.) ;
#88086=ADVANCED_FACE('',(#19766),#1365,.F.) ;
#88087=ADVANCED_FACE('',(#19767),#1366,.F.) ;
#88088=ADVANCED_FACE('',(#19768),#1367,.F.) ;
#88089=ADVANCED_FACE('',(#19769),#1368,.F.) ;
#88090=ADVANCED_FACE('',(#19770),#1369,.F.) ;
#88091=ADVANCED_FACE('',(#19771),#1370,.T.) ;
#88092=ADVANCED_FACE('',(#19772),#1371,.F.) ;
#88093=ADVANCED_FACE('',(#19773),#14796,.T.) ;
#88094=ADVANCED_FACE('',(#19774),#14797,.F.) ;
#88095=ADVANCED_FACE('',(#19775),#1372,.F.) ;
#88096=ADVANCED_FACE('',(#19776),#1373,.F.) ;
#88097=ADVANCED_FACE('',(#19777),#1374,.F.) ;
#88098=ADVANCED_FACE('',(#19778),#1375,.F.) ;
#88099=ADVANCED_FACE('',(#19779),#1376,.F.) ;
#88100=ADVANCED_FACE('',(#19780),#1377,.T.) ;
#88101=ADVANCED_FACE('',(#19781),#1378,.F.) ;
#88102=ADVANCED_FACE('',(#19782),#1379,.F.) ;
#88103=ADVANCED_FACE('',(#19783),#1380,.F.) ;
#88104=ADVANCED_FACE('',(#19784),#1381,.F.) ;
#88105=ADVANCED_FACE('',(#19785),#1382,.F.) ;
#88106=ADVANCED_FACE('',(#19786),#1383,.F.) ;
#88107=ADVANCED_FACE('',(#19787),#1384,.T.) ;
#88108=ADVANCED_FACE('',(#19788),#1385,.F.) ;
#88109=ADVANCED_FACE('',(#19789),#14798,.T.) ;
#88110=ADVANCED_FACE('',(#19790),#14799,.F.) ;
#88111=ADVANCED_FACE('',(#19791),#1386,.F.) ;
#88112=ADVANCED_FACE('',(#19792),#1387,.F.) ;
#88113=ADVANCED_FACE('',(#19793),#1388,.F.) ;
#88114=ADVANCED_FACE('',(#19794),#1389,.F.) ;
#88115=ADVANCED_FACE('',(#19795),#1390,.F.) ;
#88116=ADVANCED_FACE('',(#19796),#1391,.T.) ;
#88117=ADVANCED_FACE('',(#19797),#1392,.F.) ;
#88118=ADVANCED_FACE('',(#19798),#1393,.F.) ;
#88119=ADVANCED_FACE('',(#19799),#1394,.F.) ;
#88120=ADVANCED_FACE('',(#19800),#1395,.F.) ;
#88121=ADVANCED_FACE('',(#19801),#1396,.F.) ;
#88122=ADVANCED_FACE('',(#19802),#1397,.F.) ;
#88123=ADVANCED_FACE('',(#19803),#1398,.T.) ;
#88124=ADVANCED_FACE('',(#19804),#1399,.F.) ;
#88125=ADVANCED_FACE('',(#19805),#14800,.T.) ;
#88126=ADVANCED_FACE('',(#19806),#14801,.F.) ;
#88127=ADVANCED_FACE('',(#19807),#1400,.F.) ;
#88128=ADVANCED_FACE('',(#19808),#1401,.F.) ;
#88129=ADVANCED_FACE('',(#19809),#1402,.F.) ;
#88130=ADVANCED_FACE('',(#19810),#1403,.F.) ;
#88131=ADVANCED_FACE('',(#19811),#1404,.F.) ;
#88132=ADVANCED_FACE('',(#19812),#1405,.T.) ;
#88133=ADVANCED_FACE('',(#19813),#1406,.F.) ;
#88134=ADVANCED_FACE('',(#19814),#1407,.F.) ;
#88135=ADVANCED_FACE('',(#19815),#1408,.F.) ;
#88136=ADVANCED_FACE('',(#19816),#1409,.F.) ;
#88137=ADVANCED_FACE('',(#19817),#1410,.F.) ;
#88138=ADVANCED_FACE('',(#19818),#1411,.F.) ;
#88139=ADVANCED_FACE('',(#19819),#1412,.T.) ;
#88140=ADVANCED_FACE('',(#19820),#1413,.F.) ;
#88141=ADVANCED_FACE('',(#19821),#14802,.T.) ;
#88142=ADVANCED_FACE('',(#19822),#14803,.F.) ;
#88143=ADVANCED_FACE('',(#19823),#1414,.F.) ;
#88144=ADVANCED_FACE('',(#19824),#1415,.F.) ;
#88145=ADVANCED_FACE('',(#19825),#1416,.F.) ;
#88146=ADVANCED_FACE('',(#19826),#1417,.F.) ;
#88147=ADVANCED_FACE('',(#19827),#1418,.F.) ;
#88148=ADVANCED_FACE('',(#19828),#1419,.T.) ;
#88149=ADVANCED_FACE('',(#19829),#1420,.F.) ;
#88150=ADVANCED_FACE('',(#19830),#1421,.F.) ;
#88151=ADVANCED_FACE('',(#19831),#1422,.F.) ;
#88152=ADVANCED_FACE('',(#19832),#1423,.F.) ;
#88153=ADVANCED_FACE('',(#19833),#1424,.F.) ;
#88154=ADVANCED_FACE('',(#19834),#1425,.F.) ;
#88155=ADVANCED_FACE('',(#19835),#1426,.T.) ;
#88156=ADVANCED_FACE('',(#19836),#1427,.F.) ;
#88157=ADVANCED_FACE('',(#19837),#14804,.T.) ;
#88158=ADVANCED_FACE('',(#19838),#14805,.F.) ;
#88159=ADVANCED_FACE('',(#19839),#1428,.F.) ;
#88160=ADVANCED_FACE('',(#19840),#1429,.F.) ;
#88161=ADVANCED_FACE('',(#19841),#1430,.F.) ;
#88162=ADVANCED_FACE('',(#19842),#1431,.F.) ;
#88163=ADVANCED_FACE('',(#19843),#1432,.F.) ;
#88164=ADVANCED_FACE('',(#19844),#1433,.T.) ;
#88165=ADVANCED_FACE('',(#19845),#1434,.F.) ;
#88166=ADVANCED_FACE('',(#19846),#1435,.F.) ;
#88167=ADVANCED_FACE('',(#19847),#1436,.F.) ;
#88168=ADVANCED_FACE('',(#19848),#1437,.F.) ;
#88169=ADVANCED_FACE('',(#19849),#1438,.F.) ;
#88170=ADVANCED_FACE('',(#19850),#1439,.F.) ;
#88171=ADVANCED_FACE('',(#19851),#1440,.T.) ;
#88172=ADVANCED_FACE('',(#19852),#1441,.F.) ;
#88173=ADVANCED_FACE('',(#19853),#14806,.T.) ;
#88174=ADVANCED_FACE('',(#19854),#14807,.F.) ;
#88175=ADVANCED_FACE('',(#19855),#1442,.F.) ;
#88176=ADVANCED_FACE('',(#19856),#1443,.F.) ;
#88177=ADVANCED_FACE('',(#19857),#1444,.F.) ;
#88178=ADVANCED_FACE('',(#19858),#1445,.F.) ;
#88179=ADVANCED_FACE('',(#19859),#1446,.F.) ;
#88180=ADVANCED_FACE('',(#19860),#1447,.T.) ;
#88181=ADVANCED_FACE('',(#19861),#1448,.F.) ;
#88182=ADVANCED_FACE('',(#19862),#1449,.F.) ;
#88183=ADVANCED_FACE('',(#19863),#1450,.F.) ;
#88184=ADVANCED_FACE('',(#19864),#1451,.F.) ;
#88185=ADVANCED_FACE('',(#19865),#1452,.F.) ;
#88186=ADVANCED_FACE('',(#19866),#1453,.F.) ;
#88187=ADVANCED_FACE('',(#19867),#1454,.T.) ;
#88188=ADVANCED_FACE('',(#19868),#1455,.F.) ;
#88189=ADVANCED_FACE('',(#19869),#14808,.T.) ;
#88190=ADVANCED_FACE('',(#19870),#14809,.F.) ;
#88191=ADVANCED_FACE('',(#19871),#1456,.F.) ;
#88192=ADVANCED_FACE('',(#19872),#1457,.F.) ;
#88193=ADVANCED_FACE('',(#19873),#1458,.F.) ;
#88194=ADVANCED_FACE('',(#19874),#1459,.F.) ;
#88195=ADVANCED_FACE('',(#19875),#1460,.F.) ;
#88196=ADVANCED_FACE('',(#19876),#1461,.T.) ;
#88197=ADVANCED_FACE('',(#19877),#1462,.F.) ;
#88198=ADVANCED_FACE('',(#19878),#1463,.F.) ;
#88199=ADVANCED_FACE('',(#19879),#1464,.F.) ;
#88200=ADVANCED_FACE('',(#19880),#1465,.F.) ;
#88201=ADVANCED_FACE('',(#19881),#1466,.F.) ;
#88202=ADVANCED_FACE('',(#19882),#1467,.F.) ;
#88203=ADVANCED_FACE('',(#19883),#1468,.T.) ;
#88204=ADVANCED_FACE('',(#19884),#1469,.F.) ;
#88205=ADVANCED_FACE('',(#19885),#14810,.T.) ;
#88206=ADVANCED_FACE('',(#19886),#14811,.F.) ;
#88207=ADVANCED_FACE('',(#19887),#1470,.F.) ;
#88208=ADVANCED_FACE('',(#19888),#1471,.F.) ;
#88209=ADVANCED_FACE('',(#19889),#1472,.F.) ;
#88210=ADVANCED_FACE('',(#19890),#1473,.F.) ;
#88211=ADVANCED_FACE('',(#19891),#1474,.F.) ;
#88212=ADVANCED_FACE('',(#19892),#1475,.T.) ;
#88213=ADVANCED_FACE('',(#19893),#1476,.F.) ;
#88214=ADVANCED_FACE('',(#19894),#1477,.F.) ;
#88215=ADVANCED_FACE('',(#19895),#1478,.F.) ;
#88216=ADVANCED_FACE('',(#19896),#1479,.F.) ;
#88217=ADVANCED_FACE('',(#19897),#1480,.F.) ;
#88218=ADVANCED_FACE('',(#19898),#1481,.F.) ;
#88219=ADVANCED_FACE('',(#19899),#1482,.F.) ;
#88220=ADVANCED_FACE('',(#19900),#1483,.F.) ;
#88221=ADVANCED_FACE('',(#19901),#1484,.F.) ;
#88222=ADVANCED_FACE('',(#19902),#1485,.F.) ;
#88223=ADVANCED_FACE('',(#19903),#1486,.F.) ;
#88224=ADVANCED_FACE('',(#19904),#1487,.F.) ;
#88225=ADVANCED_FACE('',(#19905),#1488,.F.) ;
#88226=ADVANCED_FACE('',(#19906),#1489,.F.) ;
#88227=ADVANCED_FACE('',(#19907),#1490,.F.) ;
#88228=ADVANCED_FACE('',(#19908),#1491,.F.) ;
#88229=ADVANCED_FACE('',(#19909),#1492,.F.) ;
#88230=ADVANCED_FACE('',(#19910),#1493,.F.) ;
#88231=ADVANCED_FACE('',(#19911),#1494,.F.) ;
#88232=ADVANCED_FACE('',(#19912),#1495,.F.) ;
#88233=ADVANCED_FACE('',(#19913),#1496,.F.) ;
#88234=ADVANCED_FACE('',(#19914),#1497,.F.) ;
#88235=ADVANCED_FACE('',(#19915),#1498,.F.) ;
#88236=ADVANCED_FACE('',(#19916),#1499,.F.) ;
#88237=ADVANCED_FACE('',(#19917),#1500,.F.) ;
#88238=ADVANCED_FACE('',(#19918),#1501,.F.) ;
#88239=ADVANCED_FACE('',(#19919),#1502,.F.) ;
#88240=ADVANCED_FACE('',(#19920),#1503,.F.) ;
#88241=ADVANCED_FACE('',(#19921),#1504,.F.) ;
#88242=ADVANCED_FACE('',(#19922),#1505,.F.) ;
#88243=ADVANCED_FACE('',(#19923),#1506,.F.) ;
#88244=ADVANCED_FACE('',(#19924),#1507,.F.) ;
#88245=ADVANCED_FACE('',(#19925),#1508,.F.) ;
#88246=ADVANCED_FACE('',(#19926),#1509,.F.) ;
#88247=ADVANCED_FACE('',(#19927),#1510,.F.) ;
#88248=ADVANCED_FACE('',(#19928),#1511,.F.) ;
#88249=ADVANCED_FACE('',(#19929),#1512,.F.) ;
#88250=ADVANCED_FACE('',(#19930),#14812,.T.) ;
#88251=ADVANCED_FACE('',(#19931),#14813,.T.) ;
#88252=ADVANCED_FACE('',(#19932),#16545,.T.) ;
#88253=ADVANCED_FACE('',(#19933),#14814,.T.) ;
#88254=ADVANCED_FACE('',(#19934),#14815,.T.) ;
#88255=ADVANCED_FACE('',(#19935),#14816,.T.) ;
#88256=ADVANCED_FACE('',(#19936),#16546,.T.) ;
#88257=ADVANCED_FACE('',(#19937),#16547,.T.) ;
#88258=ADVANCED_FACE('',(#19938),#14817,.T.) ;
#88259=ADVANCED_FACE('',(#19939),#14818,.T.) ;
#88260=ADVANCED_FACE('',(#19940),#14819,.T.) ;
#88261=ADVANCED_FACE('',(#19941),#16548,.T.) ;
#88262=ADVANCED_FACE('',(#19942),#14820,.T.) ;
#88263=ADVANCED_FACE('',(#19943),#14821,.T.) ;
#88264=ADVANCED_FACE('',(#19944),#14822,.T.) ;
#88265=ADVANCED_FACE('',(#19945),#14823,.T.) ;
#88266=ADVANCED_FACE('',(#19946),#16549,.T.) ;
#88267=ADVANCED_FACE('',(#19947),#14824,.T.) ;
#88268=ADVANCED_FACE('',(#19948),#14825,.T.) ;
#88269=ADVANCED_FACE('',(#19949),#14826,.T.) ;
#88270=ADVANCED_FACE('',(#19950),#16550,.T.) ;
#88271=ADVANCED_FACE('',(#19951),#16551,.T.) ;
#88272=ADVANCED_FACE('',(#19952),#14827,.T.) ;
#88273=ADVANCED_FACE('',(#19953),#14828,.T.) ;
#88274=ADVANCED_FACE('',(#19954),#14829,.T.) ;
#88275=ADVANCED_FACE('',(#19955),#16552,.T.) ;
#88276=ADVANCED_FACE('',(#19956),#14830,.T.) ;
#88277=ADVANCED_FACE('',(#19957),#14831,.T.) ;
#88278=ADVANCED_FACE('',(#19958),#14832,.T.) ;
#88279=ADVANCED_FACE('',(#19959),#14833,.T.) ;
#88280=ADVANCED_FACE('',(#19960),#16553,.T.) ;
#88281=ADVANCED_FACE('',(#19961),#14834,.T.) ;
#88282=ADVANCED_FACE('',(#19962),#14835,.T.) ;
#88283=ADVANCED_FACE('',(#19963),#14836,.T.) ;
#88284=ADVANCED_FACE('',(#19964),#16554,.T.) ;
#88285=ADVANCED_FACE('',(#19965),#16555,.T.) ;
#88286=ADVANCED_FACE('',(#19966),#14837,.T.) ;
#88287=ADVANCED_FACE('',(#19967),#14838,.T.) ;
#88288=ADVANCED_FACE('',(#19968),#14839,.T.) ;
#88289=ADVANCED_FACE('',(#19969),#16556,.T.) ;
#88290=ADVANCED_FACE('',(#19970),#14840,.T.) ;
#88291=ADVANCED_FACE('',(#19971),#14841,.T.) ;
#88292=ADVANCED_FACE('',(#19972),#14842,.T.) ;
#88293=ADVANCED_FACE('',(#19973),#14843,.T.) ;
#88294=ADVANCED_FACE('',(#19974),#16557,.T.) ;
#88295=ADVANCED_FACE('',(#19975),#14844,.T.) ;
#88296=ADVANCED_FACE('',(#19976),#14845,.T.) ;
#88297=ADVANCED_FACE('',(#19977),#14846,.T.) ;
#88298=ADVANCED_FACE('',(#19978),#16558,.T.) ;
#88299=ADVANCED_FACE('',(#19979),#16559,.T.) ;
#88300=ADVANCED_FACE('',(#19980),#14847,.T.) ;
#88301=ADVANCED_FACE('',(#19981),#14848,.T.) ;
#88302=ADVANCED_FACE('',(#19982),#14849,.T.) ;
#88303=ADVANCED_FACE('',(#19983),#16560,.T.) ;
#88304=ADVANCED_FACE('',(#19984),#14850,.T.) ;
#88305=ADVANCED_FACE('',(#19985),#14851,.T.) ;
#88306=ADVANCED_FACE('',(#19986),#14852,.T.) ;
#88307=ADVANCED_FACE('',(#19987),#14853,.T.) ;
#88308=ADVANCED_FACE('',(#19988),#16561,.T.) ;
#88309=ADVANCED_FACE('',(#19989),#14854,.T.) ;
#88310=ADVANCED_FACE('',(#19990),#14855,.T.) ;
#88311=ADVANCED_FACE('',(#19991),#14856,.T.) ;
#88312=ADVANCED_FACE('',(#19992),#16562,.T.) ;
#88313=ADVANCED_FACE('',(#19993),#16563,.T.) ;
#88314=ADVANCED_FACE('',(#19994),#14857,.T.) ;
#88315=ADVANCED_FACE('',(#19995),#14858,.T.) ;
#88316=ADVANCED_FACE('',(#19996),#14859,.T.) ;
#88317=ADVANCED_FACE('',(#19997),#16564,.T.) ;
#88318=ADVANCED_FACE('',(#19998),#14860,.T.) ;
#88319=ADVANCED_FACE('',(#19999),#14861,.T.) ;
#88320=ADVANCED_FACE('',(#20000),#14862,.T.) ;
#88321=ADVANCED_FACE('',(#20001),#14863,.T.) ;
#88322=ADVANCED_FACE('',(#20002),#16565,.T.) ;
#88323=ADVANCED_FACE('',(#20003),#14864,.T.) ;
#88324=ADVANCED_FACE('',(#20004),#14865,.T.) ;
#88325=ADVANCED_FACE('',(#20005),#14866,.T.) ;
#88326=ADVANCED_FACE('',(#20006),#16566,.T.) ;
#88327=ADVANCED_FACE('',(#20007),#16567,.T.) ;
#88328=ADVANCED_FACE('',(#20008),#14867,.T.) ;
#88329=ADVANCED_FACE('',(#20009),#14868,.T.) ;
#88330=ADVANCED_FACE('',(#20010),#14869,.T.) ;
#88331=ADVANCED_FACE('',(#20011),#16568,.T.) ;
#88332=ADVANCED_FACE('',(#20012),#14870,.T.) ;
#88333=ADVANCED_FACE('',(#20013),#14871,.T.) ;
#88334=ADVANCED_FACE('',(#20014),#14872,.T.) ;
#88335=ADVANCED_FACE('',(#20015),#14873,.T.) ;
#88336=ADVANCED_FACE('',(#20016),#16569,.T.) ;
#88337=ADVANCED_FACE('',(#20017),#14874,.T.) ;
#88338=ADVANCED_FACE('',(#20018),#14875,.T.) ;
#88339=ADVANCED_FACE('',(#20019),#14876,.T.) ;
#88340=ADVANCED_FACE('',(#20020),#16570,.T.) ;
#88341=ADVANCED_FACE('',(#20021),#16571,.T.) ;
#88342=ADVANCED_FACE('',(#20022),#14877,.T.) ;
#88343=ADVANCED_FACE('',(#20023),#14878,.T.) ;
#88344=ADVANCED_FACE('',(#20024),#14879,.T.) ;
#88345=ADVANCED_FACE('',(#20025),#16572,.T.) ;
#88346=ADVANCED_FACE('',(#20026),#14880,.T.) ;
#88347=ADVANCED_FACE('',(#20027),#14881,.T.) ;
#88348=ADVANCED_FACE('',(#20028),#14882,.T.) ;
#88349=ADVANCED_FACE('',(#20029),#14883,.T.) ;
#88350=ADVANCED_FACE('',(#20030),#16573,.T.) ;
#88351=ADVANCED_FACE('',(#20031),#14884,.T.) ;
#88352=ADVANCED_FACE('',(#20032),#14885,.T.) ;
#88353=ADVANCED_FACE('',(#20033),#14886,.T.) ;
#88354=ADVANCED_FACE('',(#20034),#16574,.T.) ;
#88355=ADVANCED_FACE('',(#20035),#16575,.T.) ;
#88356=ADVANCED_FACE('',(#20036),#14887,.T.) ;
#88357=ADVANCED_FACE('',(#20037),#14888,.T.) ;
#88358=ADVANCED_FACE('',(#20038),#14889,.T.) ;
#88359=ADVANCED_FACE('',(#20039),#16576,.T.) ;
#88360=ADVANCED_FACE('',(#20040),#14890,.T.) ;
#88361=ADVANCED_FACE('',(#20041),#14891,.T.) ;
#88362=ADVANCED_FACE('',(#20042),#14892,.T.) ;
#88363=ADVANCED_FACE('',(#20043),#14893,.T.) ;
#88364=ADVANCED_FACE('',(#20044),#16577,.T.) ;
#88365=ADVANCED_FACE('',(#20045),#14894,.T.) ;
#88366=ADVANCED_FACE('',(#20046),#14895,.T.) ;
#88367=ADVANCED_FACE('',(#20047),#14896,.T.) ;
#88368=ADVANCED_FACE('',(#20048),#16578,.T.) ;
#88369=ADVANCED_FACE('',(#20049),#16579,.T.) ;
#88370=ADVANCED_FACE('',(#20050),#14897,.T.) ;
#88371=ADVANCED_FACE('',(#20051),#14898,.T.) ;
#88372=ADVANCED_FACE('',(#20052),#14899,.T.) ;
#88373=ADVANCED_FACE('',(#20053),#16580,.T.) ;
#88374=ADVANCED_FACE('',(#20054),#14900,.T.) ;
#88375=ADVANCED_FACE('',(#20055),#14901,.T.) ;
#88376=ADVANCED_FACE('',(#20056),#14902,.T.) ;
#88377=ADVANCED_FACE('',(#20057),#14903,.T.) ;
#88378=ADVANCED_FACE('',(#20058),#16581,.T.) ;
#88379=ADVANCED_FACE('',(#20059),#14904,.T.) ;
#88380=ADVANCED_FACE('',(#20060),#14905,.T.) ;
#88381=ADVANCED_FACE('',(#20061),#14906,.T.) ;
#88382=ADVANCED_FACE('',(#20062),#16582,.T.) ;
#88383=ADVANCED_FACE('',(#20063),#16583,.T.) ;
#88384=ADVANCED_FACE('',(#20064),#14907,.T.) ;
#88385=ADVANCED_FACE('',(#20065),#14908,.T.) ;
#88386=ADVANCED_FACE('',(#20066),#14909,.T.) ;
#88387=ADVANCED_FACE('',(#20067),#16584,.T.) ;
#88388=ADVANCED_FACE('',(#20068),#14910,.T.) ;
#88389=ADVANCED_FACE('',(#20069),#14911,.T.) ;
#88390=ADVANCED_FACE('',(#20070),#14912,.T.) ;
#88391=ADVANCED_FACE('',(#20071),#14913,.T.) ;
#88392=ADVANCED_FACE('',(#20072),#16585,.T.) ;
#88393=ADVANCED_FACE('',(#20073),#14914,.T.) ;
#88394=ADVANCED_FACE('',(#20074),#14915,.T.) ;
#88395=ADVANCED_FACE('',(#20075),#14916,.T.) ;
#88396=ADVANCED_FACE('',(#20076),#16586,.T.) ;
#88397=ADVANCED_FACE('',(#20077),#16587,.T.) ;
#88398=ADVANCED_FACE('',(#20078),#14917,.T.) ;
#88399=ADVANCED_FACE('',(#20079),#14918,.T.) ;
#88400=ADVANCED_FACE('',(#20080),#14919,.T.) ;
#88401=ADVANCED_FACE('',(#20081),#16588,.T.) ;
#88402=ADVANCED_FACE('',(#20082),#14920,.T.) ;
#88403=ADVANCED_FACE('',(#20083),#14921,.T.) ;
#88404=ADVANCED_FACE('',(#20084),#14922,.T.) ;
#88405=ADVANCED_FACE('',(#20085),#14923,.T.) ;
#88406=ADVANCED_FACE('',(#20086),#16589,.T.) ;
#88407=ADVANCED_FACE('',(#20087),#14924,.T.) ;
#88408=ADVANCED_FACE('',(#20088),#14925,.T.) ;
#88409=ADVANCED_FACE('',(#20089),#14926,.T.) ;
#88410=ADVANCED_FACE('',(#20090),#16590,.T.) ;
#88411=ADVANCED_FACE('',(#20091),#16591,.T.) ;
#88412=ADVANCED_FACE('',(#20092),#14927,.T.) ;
#88413=ADVANCED_FACE('',(#20093),#14928,.T.) ;
#88414=ADVANCED_FACE('',(#20094),#14929,.T.) ;
#88415=ADVANCED_FACE('',(#20095),#16592,.T.) ;
#88416=ADVANCED_FACE('',(#20096),#14930,.T.) ;
#88417=ADVANCED_FACE('',(#20097),#14931,.T.) ;
#88418=ADVANCED_FACE('',(#20098),#14932,.T.) ;
#88419=ADVANCED_FACE('',(#20099),#14933,.T.) ;
#88420=ADVANCED_FACE('',(#20100),#16593,.T.) ;
#88421=ADVANCED_FACE('',(#20101),#14934,.T.) ;
#88422=ADVANCED_FACE('',(#20102),#14935,.T.) ;
#88423=ADVANCED_FACE('',(#20103),#14936,.T.) ;
#88424=ADVANCED_FACE('',(#20104),#16594,.T.) ;
#88425=ADVANCED_FACE('',(#20105),#16595,.T.) ;
#88426=ADVANCED_FACE('',(#20106),#14937,.T.) ;
#88427=ADVANCED_FACE('',(#20107),#14938,.T.) ;
#88428=ADVANCED_FACE('',(#20108),#14939,.T.) ;
#88429=ADVANCED_FACE('',(#20109),#16596,.T.) ;
#88430=ADVANCED_FACE('',(#20110),#14940,.T.) ;
#88431=ADVANCED_FACE('',(#20111),#14941,.T.) ;
#88432=ADVANCED_FACE('',(#20112),#14942,.T.) ;
#88433=ADVANCED_FACE('',(#20113),#14943,.T.) ;
#88434=ADVANCED_FACE('',(#20114),#16597,.T.) ;
#88435=ADVANCED_FACE('',(#20115),#14944,.T.) ;
#88436=ADVANCED_FACE('',(#20116),#14945,.T.) ;
#88437=ADVANCED_FACE('',(#20117),#14946,.T.) ;
#88438=ADVANCED_FACE('',(#20118),#16598,.T.) ;
#88439=ADVANCED_FACE('',(#20119),#16599,.T.) ;
#88440=ADVANCED_FACE('',(#20120),#14947,.T.) ;
#88441=ADVANCED_FACE('',(#20121),#14948,.T.) ;
#88442=ADVANCED_FACE('',(#20122),#14949,.T.) ;
#88443=ADVANCED_FACE('',(#20123),#16600,.T.) ;
#88444=ADVANCED_FACE('',(#20124),#14950,.T.) ;
#88445=ADVANCED_FACE('',(#20125),#14951,.T.) ;
#88446=ADVANCED_FACE('',(#20126),#14952,.T.) ;
#88447=ADVANCED_FACE('',(#20127),#14953,.T.) ;
#88448=ADVANCED_FACE('',(#20128),#16601,.T.) ;
#88449=ADVANCED_FACE('',(#20129),#14954,.T.) ;
#88450=ADVANCED_FACE('',(#20130),#14955,.T.) ;
#88451=ADVANCED_FACE('',(#20131),#14956,.T.) ;
#88452=ADVANCED_FACE('',(#20132),#16602,.T.) ;
#88453=ADVANCED_FACE('',(#20133),#16603,.T.) ;
#88454=ADVANCED_FACE('',(#20134),#14957,.T.) ;
#88455=ADVANCED_FACE('',(#20135),#14958,.T.) ;
#88456=ADVANCED_FACE('',(#20136),#14959,.T.) ;
#88457=ADVANCED_FACE('',(#20137),#16604,.T.) ;
#88458=ADVANCED_FACE('',(#20138),#14960,.T.) ;
#88459=ADVANCED_FACE('',(#20139),#14961,.T.) ;
#88460=ADVANCED_FACE('',(#20140),#14962,.T.) ;
#88461=ADVANCED_FACE('',(#20141),#14963,.T.) ;
#88462=ADVANCED_FACE('',(#20142),#16605,.T.) ;
#88463=ADVANCED_FACE('',(#20143),#14964,.T.) ;
#88464=ADVANCED_FACE('',(#20144),#14965,.T.) ;
#88465=ADVANCED_FACE('',(#20145),#14966,.T.) ;
#88466=ADVANCED_FACE('',(#20146),#16606,.T.) ;
#88467=ADVANCED_FACE('',(#20147),#16607,.T.) ;
#88468=ADVANCED_FACE('',(#20148),#14967,.T.) ;
#88469=ADVANCED_FACE('',(#20149),#14968,.T.) ;
#88470=ADVANCED_FACE('',(#20150),#14969,.T.) ;
#88471=ADVANCED_FACE('',(#20151),#16608,.T.) ;
#88472=ADVANCED_FACE('',(#20152),#14970,.T.) ;
#88473=ADVANCED_FACE('',(#20153),#14971,.T.) ;
#88474=ADVANCED_FACE('',(#20154),#14972,.T.) ;
#88475=ADVANCED_FACE('',(#20155),#14973,.T.) ;
#88476=ADVANCED_FACE('',(#20156),#16609,.T.) ;
#88477=ADVANCED_FACE('',(#20157),#14974,.T.) ;
#88478=ADVANCED_FACE('',(#20158),#14975,.T.) ;
#88479=ADVANCED_FACE('',(#20159),#14976,.T.) ;
#88480=ADVANCED_FACE('',(#20160),#16610,.T.) ;
#88481=ADVANCED_FACE('',(#20161),#16611,.T.) ;
#88482=ADVANCED_FACE('',(#20162),#14977,.T.) ;
#88483=ADVANCED_FACE('',(#20163),#14978,.T.) ;
#88484=ADVANCED_FACE('',(#20164),#14979,.T.) ;
#88485=ADVANCED_FACE('',(#20165),#16612,.T.) ;
#88486=ADVANCED_FACE('',(#20166),#14980,.T.) ;
#88487=ADVANCED_FACE('',(#20167),#14981,.T.) ;
#88488=ADVANCED_FACE('',(#20168),#14982,.T.) ;
#88489=ADVANCED_FACE('',(#20169),#14983,.T.) ;
#88490=ADVANCED_FACE('',(#20170),#16613,.T.) ;
#88491=ADVANCED_FACE('',(#20171),#14984,.T.) ;
#88492=ADVANCED_FACE('',(#20172),#14985,.T.) ;
#88493=ADVANCED_FACE('',(#20173),#14986,.T.) ;
#88494=ADVANCED_FACE('',(#20174),#16614,.T.) ;
#88495=ADVANCED_FACE('',(#20175),#16615,.T.) ;
#88496=ADVANCED_FACE('',(#20176),#14987,.T.) ;
#88497=ADVANCED_FACE('',(#20177),#14988,.T.) ;
#88498=ADVANCED_FACE('',(#20178),#14989,.T.) ;
#88499=ADVANCED_FACE('',(#20179),#16616,.T.) ;
#88500=ADVANCED_FACE('',(#20180),#14990,.T.) ;
#88501=ADVANCED_FACE('',(#20181),#14991,.T.) ;
#88502=ADVANCED_FACE('',(#20182),#79308,.T.) ;
#88503=ADVANCED_FACE('',(#20183),#14992,.T.) ;
#88504=ADVANCED_FACE('',(#20184),#16617,.T.) ;
#88505=ADVANCED_FACE('',(#20185),#14993,.T.) ;
#88506=ADVANCED_FACE('',(#20186),#16618,.T.) ;
#88507=ADVANCED_FACE('',(#20187),#14994,.T.) ;
#88508=ADVANCED_FACE('',(#20188),#79309,.T.) ;
#88509=ADVANCED_FACE('',(#20189),#79310,.T.) ;
#88510=ADVANCED_FACE('',(#20190),#14995,.T.) ;
#88511=ADVANCED_FACE('',(#20191),#16619,.T.) ;
#88512=ADVANCED_FACE('',(#20192),#14996,.T.) ;
#88513=ADVANCED_FACE('',(#20193),#16620,.T.) ;
#88514=ADVANCED_FACE('',(#20194),#14997,.T.) ;
#88515=ADVANCED_FACE('',(#20195),#79311,.T.) ;
#88516=ADVANCED_FACE('',(#20196),#14998,.T.) ;
#88517=ADVANCED_FACE('',(#20197),#16621,.T.) ;
#88518=ADVANCED_FACE('',(#20198),#14999,.T.) ;
#88519=ADVANCED_FACE('',(#20199),#16622,.T.) ;
#88520=ADVANCED_FACE('',(#20200),#15000,.T.) ;
#88521=ADVANCED_FACE('',(#20201),#15001,.T.) ;
#88522=ADVANCED_FACE('',(#20202),#16623,.T.) ;
#88523=ADVANCED_FACE('',(#20203),#15002,.T.) ;
#88524=ADVANCED_FACE('',(#20204),#15003,.T.) ;
#88525=ADVANCED_FACE('',(#20205),#16624,.T.) ;
#88526=ADVANCED_FACE('',(#20206),#79312,.T.) ;
#88527=ADVANCED_FACE('',(#20207),#15004,.T.) ;
#88528=ADVANCED_FACE('',(#20208),#16625,.T.) ;
#88529=ADVANCED_FACE('',(#20209),#15005,.T.) ;
#88530=ADVANCED_FACE('',(#20210),#16626,.T.) ;
#88531=ADVANCED_FACE('',(#20211),#15006,.T.) ;
#88532=ADVANCED_FACE('',(#20212),#79313,.T.) ;
#88533=ADVANCED_FACE('',(#20213),#79314,.T.) ;
#88534=ADVANCED_FACE('',(#20214),#15007,.T.) ;
#88535=ADVANCED_FACE('',(#20215),#16627,.T.) ;
#88536=ADVANCED_FACE('',(#20216),#15008,.T.) ;
#88537=ADVANCED_FACE('',(#20217),#16628,.T.) ;
#88538=ADVANCED_FACE('',(#20218),#15009,.T.) ;
#88539=ADVANCED_FACE('',(#20219),#79315,.T.) ;
#88540=ADVANCED_FACE('',(#20220),#15010,.T.) ;
#88541=ADVANCED_FACE('',(#20221),#16629,.T.) ;
#88542=ADVANCED_FACE('',(#20222),#15011,.T.) ;
#88543=ADVANCED_FACE('',(#20223),#16630,.T.) ;
#88544=ADVANCED_FACE('',(#20224),#15012,.T.) ;
#88545=ADVANCED_FACE('',(#20225),#15013,.T.) ;
#88546=ADVANCED_FACE('',(#20226),#16631,.T.) ;
#88547=ADVANCED_FACE('',(#20227),#15014,.T.) ;
#88548=ADVANCED_FACE('',(#20228),#15015,.T.) ;
#88549=ADVANCED_FACE('',(#20229),#16632,.T.) ;
#88550=ADVANCED_FACE('',(#20230),#79316,.T.) ;
#88551=ADVANCED_FACE('',(#20231),#15016,.T.) ;
#88552=ADVANCED_FACE('',(#20232),#16633,.T.) ;
#88553=ADVANCED_FACE('',(#20233),#15017,.T.) ;
#88554=ADVANCED_FACE('',(#20234),#16634,.T.) ;
#88555=ADVANCED_FACE('',(#20235),#15018,.T.) ;
#88556=ADVANCED_FACE('',(#20236),#79317,.T.) ;
#88557=ADVANCED_FACE('',(#20237),#79318,.T.) ;
#88558=ADVANCED_FACE('',(#20238),#15019,.T.) ;
#88559=ADVANCED_FACE('',(#20239),#16635,.T.) ;
#88560=ADVANCED_FACE('',(#20240),#15020,.T.) ;
#88561=ADVANCED_FACE('',(#20241),#16636,.T.) ;
#88562=ADVANCED_FACE('',(#20242),#15021,.T.) ;
#88563=ADVANCED_FACE('',(#20243),#79319,.T.) ;
#88564=ADVANCED_FACE('',(#20244),#15022,.T.) ;
#88565=ADVANCED_FACE('',(#20245),#16637,.T.) ;
#88566=ADVANCED_FACE('',(#20246),#15023,.T.) ;
#88567=ADVANCED_FACE('',(#20247),#16638,.T.) ;
#88568=ADVANCED_FACE('',(#20248),#15024,.T.) ;
#88569=ADVANCED_FACE('',(#20249),#15025,.T.) ;
#88570=ADVANCED_FACE('',(#20250),#16639,.T.) ;
#88571=ADVANCED_FACE('',(#20251),#15026,.T.) ;
#88572=ADVANCED_FACE('',(#20252),#15027,.T.) ;
#88573=ADVANCED_FACE('',(#20253),#16640,.T.) ;
#88574=ADVANCED_FACE('',(#20254),#79320,.T.) ;
#88575=ADVANCED_FACE('',(#20255),#15028,.T.) ;
#88576=ADVANCED_FACE('',(#20256),#16641,.T.) ;
#88577=ADVANCED_FACE('',(#20257),#15029,.T.) ;
#88578=ADVANCED_FACE('',(#20258),#16642,.T.) ;
#88579=ADVANCED_FACE('',(#20259),#15030,.T.) ;
#88580=ADVANCED_FACE('',(#20260),#79321,.T.) ;
#88581=ADVANCED_FACE('',(#20261),#79322,.T.) ;
#88582=ADVANCED_FACE('',(#20262),#15031,.T.) ;
#88583=ADVANCED_FACE('',(#20263),#16643,.T.) ;
#88584=ADVANCED_FACE('',(#20264),#15032,.T.) ;
#88585=ADVANCED_FACE('',(#20265),#16644,.T.) ;
#88586=ADVANCED_FACE('',(#20266),#15033,.T.) ;
#88587=ADVANCED_FACE('',(#20267),#79323,.T.) ;
#88588=ADVANCED_FACE('',(#20268),#15034,.T.) ;
#88589=ADVANCED_FACE('',(#20269),#16645,.T.) ;
#88590=ADVANCED_FACE('',(#20270),#15035,.T.) ;
#88591=ADVANCED_FACE('',(#20271),#16646,.T.) ;
#88592=ADVANCED_FACE('',(#20272),#15036,.T.) ;
#88593=ADVANCED_FACE('',(#20273),#15037,.T.) ;
#88594=ADVANCED_FACE('',(#20274),#16647,.T.) ;
#88595=ADVANCED_FACE('',(#20275),#15038,.T.) ;
#88596=ADVANCED_FACE('',(#20276),#15039,.T.) ;
#88597=ADVANCED_FACE('',(#20277),#16648,.T.) ;
#88598=ADVANCED_FACE('',(#20278),#79324,.T.) ;
#88599=ADVANCED_FACE('',(#20279),#15040,.T.) ;
#88600=ADVANCED_FACE('',(#20280),#16649,.T.) ;
#88601=ADVANCED_FACE('',(#20281),#15041,.T.) ;
#88602=ADVANCED_FACE('',(#20282),#16650,.T.) ;
#88603=ADVANCED_FACE('',(#20283),#15042,.T.) ;
#88604=ADVANCED_FACE('',(#20284),#79325,.T.) ;
#88605=ADVANCED_FACE('',(#20285),#79326,.T.) ;
#88606=ADVANCED_FACE('',(#20286),#15043,.T.) ;
#88607=ADVANCED_FACE('',(#20287),#16651,.T.) ;
#88608=ADVANCED_FACE('',(#20288),#15044,.T.) ;
#88609=ADVANCED_FACE('',(#20289),#16652,.T.) ;
#88610=ADVANCED_FACE('',(#20290),#15045,.T.) ;
#88611=ADVANCED_FACE('',(#20291),#79327,.T.) ;
#88612=ADVANCED_FACE('',(#20292),#15046,.T.) ;
#88613=ADVANCED_FACE('',(#20293),#16653,.T.) ;
#88614=ADVANCED_FACE('',(#20294),#15047,.T.) ;
#88615=ADVANCED_FACE('',(#20295),#16654,.T.) ;
#88616=ADVANCED_FACE('',(#20296),#15048,.T.) ;
#88617=ADVANCED_FACE('',(#20297),#15049,.T.) ;
#88618=ADVANCED_FACE('',(#20298),#16655,.T.) ;
#88619=ADVANCED_FACE('',(#20299),#15050,.T.) ;
#88620=ADVANCED_FACE('',(#20300),#15051,.T.) ;
#88621=ADVANCED_FACE('',(#20301),#16656,.T.) ;
#88622=ADVANCED_FACE('',(#20302),#79328,.T.) ;
#88623=ADVANCED_FACE('',(#20303),#15052,.T.) ;
#88624=ADVANCED_FACE('',(#20304),#16657,.T.) ;
#88625=ADVANCED_FACE('',(#20305),#15053,.T.) ;
#88626=ADVANCED_FACE('',(#20306),#16658,.T.) ;
#88627=ADVANCED_FACE('',(#20307),#15054,.T.) ;
#88628=ADVANCED_FACE('',(#20308),#79329,.T.) ;
#88629=ADVANCED_FACE('',(#20309),#79330,.T.) ;
#88630=ADVANCED_FACE('',(#20310),#15055,.T.) ;
#88631=ADVANCED_FACE('',(#20311),#16659,.T.) ;
#88632=ADVANCED_FACE('',(#20312),#15056,.T.) ;
#88633=ADVANCED_FACE('',(#20313),#16660,.T.) ;
#88634=ADVANCED_FACE('',(#20314),#15057,.T.) ;
#88635=ADVANCED_FACE('',(#20315),#79331,.T.) ;
#88636=ADVANCED_FACE('',(#20316),#15058,.T.) ;
#88637=ADVANCED_FACE('',(#20317),#16661,.T.) ;
#88638=ADVANCED_FACE('',(#20318),#15059,.T.) ;
#88639=ADVANCED_FACE('',(#20319),#16662,.T.) ;
#88640=ADVANCED_FACE('',(#20320),#15060,.T.) ;
#88641=ADVANCED_FACE('',(#20321),#15061,.T.) ;
#88642=ADVANCED_FACE('',(#20322),#16663,.T.) ;
#88643=ADVANCED_FACE('',(#20323),#15062,.T.) ;
#88644=ADVANCED_FACE('',(#20324),#15063,.T.) ;
#88645=ADVANCED_FACE('',(#20325),#16664,.T.) ;
#88646=ADVANCED_FACE('',(#20326),#79332,.T.) ;
#88647=ADVANCED_FACE('',(#20327),#15064,.T.) ;
#88648=ADVANCED_FACE('',(#20328),#16665,.T.) ;
#88649=ADVANCED_FACE('',(#20329),#15065,.T.) ;
#88650=ADVANCED_FACE('',(#20330),#16666,.T.) ;
#88651=ADVANCED_FACE('',(#20331),#15066,.T.) ;
#88652=ADVANCED_FACE('',(#20332),#79333,.T.) ;
#88653=ADVANCED_FACE('',(#20333),#79334,.T.) ;
#88654=ADVANCED_FACE('',(#20334),#15067,.T.) ;
#88655=ADVANCED_FACE('',(#20335),#16667,.T.) ;
#88656=ADVANCED_FACE('',(#20336),#15068,.T.) ;
#88657=ADVANCED_FACE('',(#20337),#16668,.T.) ;
#88658=ADVANCED_FACE('',(#20338),#15069,.T.) ;
#88659=ADVANCED_FACE('',(#20339),#79335,.T.) ;
#88660=ADVANCED_FACE('',(#20340),#15070,.T.) ;
#88661=ADVANCED_FACE('',(#20341),#16669,.T.) ;
#88662=ADVANCED_FACE('',(#20342),#15071,.T.) ;
#88663=ADVANCED_FACE('',(#20343),#16670,.T.) ;
#88664=ADVANCED_FACE('',(#20344),#15072,.T.) ;
#88665=ADVANCED_FACE('',(#20345),#15073,.T.) ;
#88666=ADVANCED_FACE('',(#20346),#16671,.T.) ;
#88667=ADVANCED_FACE('',(#20347),#15074,.T.) ;
#88668=ADVANCED_FACE('',(#20348),#15075,.T.) ;
#88669=ADVANCED_FACE('',(#20349),#16672,.T.) ;
#88670=ADVANCED_FACE('',(#20350),#79336,.T.) ;
#88671=ADVANCED_FACE('',(#20351),#15076,.T.) ;
#88672=ADVANCED_FACE('',(#20352),#16673,.T.) ;
#88673=ADVANCED_FACE('',(#20353),#15077,.T.) ;
#88674=ADVANCED_FACE('',(#20354),#16674,.T.) ;
#88675=ADVANCED_FACE('',(#20355),#15078,.T.) ;
#88676=ADVANCED_FACE('',(#20356),#79337,.T.) ;
#88677=ADVANCED_FACE('',(#20357),#79338,.T.) ;
#88678=ADVANCED_FACE('',(#20358),#15079,.T.) ;
#88679=ADVANCED_FACE('',(#20359),#16675,.T.) ;
#88680=ADVANCED_FACE('',(#20360),#15080,.T.) ;
#88681=ADVANCED_FACE('',(#20361),#16676,.T.) ;
#88682=ADVANCED_FACE('',(#20362),#15081,.T.) ;
#88683=ADVANCED_FACE('',(#20363),#79339,.T.) ;
#88684=ADVANCED_FACE('',(#20364),#15082,.T.) ;
#88685=ADVANCED_FACE('',(#20365),#16677,.T.) ;
#88686=ADVANCED_FACE('',(#20366),#15083,.T.) ;
#88687=ADVANCED_FACE('',(#20367),#16678,.T.) ;
#88688=ADVANCED_FACE('',(#20368),#15084,.T.) ;
#88689=ADVANCED_FACE('',(#20369),#15085,.T.) ;
#88690=ADVANCED_FACE('',(#20370),#16679,.T.) ;
#88691=ADVANCED_FACE('',(#20371),#15086,.T.) ;
#88692=ADVANCED_FACE('',(#20372),#15087,.T.) ;
#88693=ADVANCED_FACE('',(#20373),#16680,.T.) ;
#88694=ADVANCED_FACE('',(#20374),#79340,.T.) ;
#88695=ADVANCED_FACE('',(#20375),#15088,.T.) ;
#88696=ADVANCED_FACE('',(#20376),#16681,.T.) ;
#88697=ADVANCED_FACE('',(#20377),#15089,.T.) ;
#88698=ADVANCED_FACE('',(#20378),#16682,.T.) ;
#88699=ADVANCED_FACE('',(#20379),#15090,.T.) ;
#88700=ADVANCED_FACE('',(#20380),#79341,.T.) ;
#88701=ADVANCED_FACE('',(#20381),#79342,.T.) ;
#88702=ADVANCED_FACE('',(#20382),#15091,.T.) ;
#88703=ADVANCED_FACE('',(#20383),#16683,.T.) ;
#88704=ADVANCED_FACE('',(#20384),#15092,.T.) ;
#88705=ADVANCED_FACE('',(#20385),#16684,.T.) ;
#88706=ADVANCED_FACE('',(#20386),#15093,.T.) ;
#88707=ADVANCED_FACE('',(#20387),#79343,.T.) ;
#88708=ADVANCED_FACE('',(#20388),#15094,.T.) ;
#88709=ADVANCED_FACE('',(#20389),#16685,.T.) ;
#88710=ADVANCED_FACE('',(#20390),#15095,.T.) ;
#88711=ADVANCED_FACE('',(#20391),#16686,.T.) ;
#88712=ADVANCED_FACE('',(#20392),#15096,.T.) ;
#88713=ADVANCED_FACE('',(#20393),#15097,.T.) ;
#88714=ADVANCED_FACE('',(#20394),#16687,.T.) ;
#88715=ADVANCED_FACE('',(#20395),#15098,.T.) ;
#88716=ADVANCED_FACE('',(#20396),#15099,.T.) ;
#88717=ADVANCED_FACE('',(#20397),#16688,.T.) ;
#91086=CLOSED_SHELL('',(#86488,#86489,#86490,#86491,#86492,#86493,#86494,
#86495,#86496,#86497,#86498,#86499,#86500,#86501,#86502,#86503,#86504,#86505,
#86506,#86507,#86508,#86509,#86510,#86511,#86512,#86513,#86514,#86515,#86516,
#86517,#86518,#86519,#86520,#86521,#86522,#86523,#86524,#86525,#86526,#86527,
#86528,#86529,#86530,#86531,#86532,#86533,#86534,#86535,#86536,#86537,#86538,
#86539,#86540,#86541,#86542,#86543,#86544,#86545,#86546,#86547,#86548,#86549,
#86550,#86551,#86552,#86553,#86554,#86555,#86556,#86557,#86558,#86559,#86560,
#86561,#86562,#86563,#86564,#86565,#86566,#86567,#86568,#86569,#86570,#86571,
#86572,#86573,#86574,#86575,#86576,#86577,#86578,#86579,#86580,#86581,#86582,
#86583,#86584,#86585,#86586,#86587,#86588,#86589,#86590,#86591,#86592,#86593,
#86594,#86595,#86596,#86597,#86598,#86599,#86600,#86601,#86602,#86603,#86604,
#86605,#86606,#86607,#86608,#86609,#86610,#86611,#86612,#86613,#86614,#86615,
#86616,#86617,#86618,#86619,#86620,#86621,#86622,#86623,#86624,#86625,#86626,
#86627,#86628,#86629,#86630,#86631,#86632,#86633,#86634,#86635,#86636,#86637,
#86638,#86639,#86640,#86641,#86642,#86643,#86644,#86645,#86646,#86647,#86648,
#86649,#86650,#86651,#86652,#86653,#86654,#86655,#86656,#86657,#86658,#86659,
#86660,#86661,#86662,#86663,#86664,#86665,#86666,#86667,#86668,#86669,#86670,
#86671,#86672,#86673,#86674,#86675,#86676,#86677,#86678,#86679,#86680,#86681,
#86682,#86683,#86684,#86685,#86686,#86687,#86688,#86689,#86690,#86691,#86692,
#86693,#86694,#86695,#86696,#86697,#86698,#86699,#86700,#86701,#86702,#86703,
#86704,#86705,#86706,#86707,#86708,#86709,#86710,#86711,#86712,#86713,#86714,
#86715,#86716,#86717,#86718,#86719,#86720,#86721,#86722,#86723,#86724,#86725,
#86726,#86727,#86728,#86729,#86730,#86731,#86732,#86733,#86734,#86735,#86736,
#86737,#86738,#86739,#86740,#86741,#86742,#86743,#86744,#86745,#86746,#86747,
#86748,#86749,#86750,#86751,#86752,#86753,#86754,#86755,#86756,#86757,#86758,
#86759,#86760,#86761,#86762,#86763,#86764,#86765,#86766,#86767,#86768,#86769,
#86770,#86771,#86772,#86773,#86774,#86775,#86776,#86777,#86778,#86779,#86780,
#86781,#86782,#86783,#86784,#86785,#86786,#86787,#86788,#86789,#86790,#86791,
#86792,#86793,#86794,#86795,#86796,#86797,#86798,#86799,#86800,#86801,#86802,
#86803,#86804,#86805,#86806,#86807,#86808,#86809,#86810,#86811,#86812,#86813,
#86814,#86815,#86816,#86817,#86818,#86819,#86820,#86821,#86822,#86823,#86824,
#86825,#86826,#86827,#86828,#86829,#86830,#86831,#86832,#86833,#86834,#86835,
#86836,#86837,#86838,#86839,#86840,#86841,#86842,#86843,#86844,#86845,#86846,
#86847,#86848,#86849,#86850,#86851,#86852,#86853,#86854,#86855,#86856,#86857,
#86858,#86859,#86860,#86861,#86862,#86863,#86864,#86865,#86866,#86867,#86868,
#86869,#86870,#86871,#86872,#86873,#86874,#86875,#86876,#86877,#86878,#86879,
#86880,#86881,#86882,#86883,#86884,#86885,#86886,#86887,#86888,#86889,#86890,
#86891,#86892,#86893,#86894,#86895,#86896,#86897,#86898,#86899,#86900,#86901,
#86902,#86903,#86904,#86905,#86906,#86907,#86908,#86909,#86910,#86911,#86912,
#86913,#86914,#86915,#86916,#86917,#86918,#86919,#86920,#86921,#86922,#86923,
#86924,#86925,#86926,#86927,#86928,#86929,#86930,#86931,#86932,#86933,#86934,
#86935,#86936,#86937,#86938,#86939,#86940,#86941,#86942,#86943,#86944,#86945,
#86946,#86947,#86948,#86949,#86950,#86951,#86952,#86953,#86954,#86955,#86956,
#86957,#86958,#86959,#86960,#86961,#86962,#86963,#86964,#86965,#86966,#86967,
#86968,#86969,#86970,#86971,#86972,#86973,#86974,#86975,#86976,#86977,#86978,
#86979,#86980,#86981,#86982,#86983,#86984,#86985,#86986,#86987,#86988,#86989,
#86990,#86991,#86992,#86993,#86994,#86995,#86996,#86997,#86998,#86999,#87000,
#87001,#87002,#87003,#87004,#87005,#87006,#87007,#87008,#87009,#87010,#87011,
#87012,#87013,#87014,#87015,#87016,#87017,#87018,#87019,#87020,#87021,#87022,
#87023,#87024,#87025,#87026,#87027,#87028,#87029,#87030,#87031,#87032,#87033,
#87034,#87035,#87036,#87037,#87038,#87039,#87040,#87041,#87042,#87043,#87044,
#87045,#87046,#87047,#87048,#87049,#87050,#87051,#87052,#87053,#87054,#87055,
#87056,#87057,#87058,#87059,#87060,#87061,#87062,#87063,#87064,#87065,#87066,
#87067,#87068,#87069,#87070,#87071,#87072,#87073,#87074,#87075,#87076,#87077,
#87078,#87079,#87080,#87081,#87082,#87083,#87084,#87085,#87086,#87087,#87088,
#87089,#87090,#87091,#87092,#87093,#87094,#87095,#87096,#87097,#87098,#87099,
#87100,#87101,#87102,#87103,#87104,#87105,#87106,#87107,#87108,#87109,#87110,
#87111,#87112,#87113,#87114,#87115,#87116,#87117,#87118,#87119,#87120,#87121,
#87122,#87123,#87124,#87125,#87126,#87127,#87128,#87129,#87130,#87131,#87132,
#87133,#87134,#87135,#87136,#87137,#87138,#87139,#87140,#87141,#87142,#87143,
#87144,#87145,#87146,#87147,#87148,#87149,#87150,#87151,#87152,#87153,#87154,
#87155,#87156,#87157,#87158,#87159,#87160,#87161,#87162,#87163,#87164,#87165,
#87166,#87167,#87168,#87169,#87170,#87171,#87172,#87173,#87174,#87175,#87176,
#87177,#87178,#87179,#87180,#87181,#87182,#87183,#87184,#87185,#87186,#87187,
#87188,#87189,#87190,#87191,#87192,#87193,#87194,#87195,#87196,#87197,#87198,
#87199,#87200,#87201,#87202,#87203,#87204,#87205,#87206,#87207,#87208,#87209,
#87210,#87211,#87212,#87213,#87214,#87215,#87216,#87217,#87218,#87219,#87220,
#87221,#87222,#87223,#87224,#87225,#87226,#87227,#87228,#87229,#87230,#87231,
#87232,#87233,#87234,#87235,#87236,#87237,#87238,#87239,#87240,#87241,#87242,
#87243,#87244,#87245,#87246,#87247,#87248,#87249,#87250,#87251,#87252,#87253,
#87254,#87255,#87256,#87257,#87258,#87259,#87260,#87261,#87262,#87263,#87264,
#87265,#87266,#87267,#87268,#87269,#87270,#87271,#87272,#87273,#87274,#87275,
#87276,#87277,#87278,#87279,#87280,#87281,#87282,#87283,#87284,#87285,#87286,
#87287,#87288,#87289,#87290,#87291,#87292,#87293,#87294,#87295,#87296,#87297,
#87298,#87299,#87300,#87301,#87302,#87303,#87304,#87305,#87306,#87307,#87308,
#87309,#87310,#87311,#87312,#87313,#87314,#87315,#87316,#87317,#87318,#87319,
#87320,#87321,#87322,#87323,#87324,#87325,#87326,#87327,#87328,#87329,#87330,
#87331,#87332,#87333,#87334,#87335,#87336,#87337,#87338,#87339,#87340,#87341,
#87342,#87343,#87344,#87345,#87346,#87347,#87348,#87349,#87350,#87351,#87352,
#87353,#87354,#87355,#87356,#87357,#87358,#87359,#87360,#87361,#87362,#87363,
#87364,#87365,#87366,#87367,#87368,#87369,#87370,#87371,#87372,#87373,#87374,
#87375,#87376,#87377,#87378,#87379,#87380,#87381,#87382,#87383,#87384,#87385,
#87386,#87387,#87388,#87389,#87390,#87391,#87392,#87393,#87394,#87395,#87396,
#87397,#87398,#87399,#87400,#87401,#87402,#87403,#87404,#87405,#87406,#87407,
#87408,#87409,#87410,#87411,#87412,#87413,#87414,#87415,#87416,#87417,#87418,
#87419,#87420,#87421,#87422,#87423,#87424,#87425,#87426,#87427,#87428,#87429,
#87430,#87431,#87432,#87433,#87434,#87435,#87436,#87437,#87438,#87439,#87440,
#87441,#87442,#87443,#87444,#87445,#87446,#87447,#87448,#87449,#87450,#87451,
#87452,#87453,#87454,#87455,#87456,#87457,#87458,#87459,#87460,#87461,#87462,
#87463,#87464,#87465,#87466,#87467,#87468,#87469,#87470,#87471,#87472,#87473,
#87474,#87475,#87476,#87477,#87478,#87479,#87480,#87481,#87482,#87483,#87484,
#87485,#87486,#87487,#87488,#87489,#87490,#87491,#87492,#87493,#87494,#87495,
#87496,#87497,#87498,#87499,#87500,#87501,#87502,#87503,#87504,#87505,#87506,
#87507,#87508,#87509,#87510,#87511,#87512,#87513,#87514,#87515,#87516,#87517,
#87518,#87519,#87520,#87521,#87522,#87523,#87524,#87525,#87526,#87527,#87528,
#87529,#87530,#87531,#87532,#87533,#87534,#87535,#87536,#87537,#87538,#87539,
#87540,#87541,#87542,#87543,#87544,#87545,#87546,#87547,#87548,#87549,#87550,
#87551,#87552,#87553,#87554,#87555,#87556,#87557,#87558,#87559,#87560,#87561,
#87562,#87563,#87564,#87565,#87566,#87567,#87568,#87569,#87570,#87571,#87572,
#87573,#87574,#87575,#87576,#87577,#87578,#87579,#87580,#87581,#87582,#87583,
#87584,#87585,#87586,#87587,#87588,#87589,#87590,#87591,#87592,#87593,#87594,
#87595,#87596,#87597,#87598,#87599,#87600,#87601,#87602,#87603,#87604,#87605,
#87606,#87607,#87608,#87609,#87610,#87611,#87612,#87613,#87614,#87615,#87616,
#87617,#87618,#87619,#87620,#87621,#87622,#87623,#87624,#87625,#87626,#87627,
#87628,#87629,#87630,#87631,#87632,#87633,#87634,#87635,#87636,#87637,#87638,
#87639,#87640,#87641,#87642,#87643,#87644,#87645,#87646,#87647,#87648,#87649,
#87650,#87651,#87652,#87653,#87654,#87655,#87656,#87657,#87658,#87659,#87660,
#87661,#87662,#87663,#87664,#87665,#87666,#87667,#87668,#87669,#87670,#87671,
#87672,#87673,#87674,#87675,#87676,#87677,#87678,#87679,#87680,#87681,#87682,
#87683,#87684,#87685,#87686,#87687,#87688,#87689,#87690,#87691,#87692,#87693,
#87694,#87695,#87696,#87697,#87698,#87699,#87700,#87701,#87702,#87703,#87704,
#87705,#87706,#87707,#87708,#87709,#87710,#87711,#87712,#87713,#87714,#87715,
#87716,#87717,#87718,#87719,#87720,#87721,#87722,#87723,#87724,#87725,#87726,
#87727,#87728,#87729,#87730,#87731,#87732,#87733,#87734,#87735,#87736,#87737,
#87738,#87739,#87740,#87741,#87742,#87743,#87744,#87745,#87746,#87747,#87748,
#87749,#87750,#87751,#87752,#87753,#87754,#87755,#87756,#87757,#87758,#87759,
#87760,#87761,#87762,#87763,#87764,#87765,#87766,#87767,#87768,#87769,#87770,
#87771,#87772,#87773,#87774,#87775,#87776,#87777,#87778,#87779,#87780,#87781,
#87782,#87783,#87784,#87785,#87786,#87787,#87788,#87789,#87790,#87791,#87792,
#87793,#87794,#87795,#87796,#87797,#87798,#87799,#87800,#87801,#87802,#87803,
#87804,#87805,#87806,#87807,#87808,#87809,#87810,#87811,#87812,#87813,#87814,
#87815,#87816,#87817,#87818,#87819,#87820,#87821,#87822,#87823,#87824,#87825,
#87826,#87827,#87828,#87829,#87830,#87831,#87832,#87833,#87834,#87835,#87836,
#87837,#87838,#87839,#87840,#87841,#87842,#87843,#87844,#87845,#87846,#87847,
#87848,#87849,#87850,#87851,#87852,#87853,#87854,#87855,#87856,#87857,#87858,
#87859,#87860,#87861,#87862,#87863,#87864,#87865,#87866,#87867,#87868,#87869,
#87870,#87871,#87872,#87873,#87874,#87875,#87876,#87877,#87878,#87879,#87880,
#87881,#87882,#87883,#87884,#87885,#87886,#87887,#87888,#87889,#87890,#87891,
#87892,#87893,#87894,#87895,#87896,#87897,#87898,#87899,#87900,#87901,#87902,
#87903,#87904,#87905,#87906,#87907,#87908,#87909,#87910,#87911,#87912,#87913,
#87914,#87915,#87916,#87917,#87918,#87919,#87920,#87921,#87922,#87923,#87924,
#87925,#87926,#87927,#87928,#87929,#87930,#87931,#87932,#87933,#87934,#87935,
#87936,#87937,#87938,#87939,#87940,#87941,#87942,#87943,#87944,#87945,#87946,
#87947,#87948,#87949,#87950,#87951,#87952,#87953,#87954,#87955,#87956,#87957,
#87958,#87959,#87960,#87961,#87962,#87963,#87964,#87965,#87966,#87967,#87968,
#87969,#87970,#87971,#87972,#87973,#87974,#87975,#87976,#87977,#87978,#87979,
#87980,#87981,#87982,#87983,#87984,#87985,#87986,#87987,#87988,#87989,#87990,
#87991,#87992,#87993,#87994,#87995,#87996,#87997,#87998,#87999,#88000,#88001,
#88002,#88003,#88004,#88005,#88006,#88007,#88008,#88009,#88010,#88011,#88012,
#88013,#88014,#88015,#88016,#88017,#88018,#88019,#88020,#88021,#88022,#88023,
#88024,#88025,#88026,#88027,#88028,#88029,#88030,#88031,#88032,#88033,#88034,
#88035,#88036,#88037,#88038,#88039,#88040,#88041,#88042,#88043,#88044,#88045,
#88046,#88047,#88048,#88049,#88050,#88051,#88052,#88053,#88054,#88055,#88056,
#88057,#88058,#88059,#88060,#88061,#88062,#88063,#88064,#88065,#88066,#88067,
#88068,#88069,#88070,#88071,#88072,#88073,#88074,#88075,#88076,#88077,#88078,
#88079,#88080,#88081,#88082,#88083,#88084,#88085,#88086,#88087,#88088,#88089,
#88090,#88091,#88092,#88093,#88094,#88095,#88096,#88097,#88098,#88099,#88100,
#88101,#88102,#88103,#88104,#88105,#88106,#88107,#88108,#88109,#88110,#88111,
#88112,#88113,#88114,#88115,#88116,#88117,#88118,#88119,#88120,#88121,#88122,
#88123,#88124,#88125,#88126,#88127,#88128,#88129,#88130,#88131,#88132,#88133,
#88134,#88135,#88136,#88137,#88138,#88139,#88140,#88141,#88142,#88143,#88144,
#88145,#88146,#88147,#88148,#88149,#88150,#88151,#88152,#88153,#88154,#88155,
#88156,#88157,#88158,#88159,#88160,#88161,#88162,#88163,#88164,#88165,#88166,
#88167,#88168,#88169,#88170,#88171,#88172,#88173,#88174,#88175,#88176,#88177,
#88178,#88179,#88180,#88181,#88182,#88183,#88184,#88185,#88186,#88187,#88188,
#88189,#88190,#88191,#88192,#88193,#88194,#88195,#88196,#88197,#88198,#88199,
#88200,#88201,#88202,#88203,#88204,#88205,#88206,#88207,#88208,#88209,#88210,
#88211,#88212,#88213,#88214,#88215,#88216,#88217,#88218,#88219,#88220,#88221,
#88222,#88223,#88224,#88225,#88226,#88227,#88228,#88229,#88230,#88231,#88232,
#88233,#88234,#88235,#88236,#88237,#88238,#88239,#88240,#88241,#88242,#88243,
#88244,#88245,#88246,#88247,#88248,#88249,#88250,#88251,#88252,#88253,#88254,
#88255,#88256,#88257,#88258,#88259,#88260,#88261,#88262,#88263,#88264,#88265,
#88266,#88267,#88268,#88269,#88270,#88271,#88272,#88273,#88274,#88275,#88276,
#88277,#88278,#88279,#88280,#88281,#88282,#88283,#88284,#88285,#88286,#88287,
#88288,#88289,#88290,#88291,#88292,#88293,#88294,#88295,#88296,#88297,#88298,
#88299,#88300,#88301,#88302,#88303,#88304,#88305,#88306,#88307,#88308,#88309,
#88310,#88311,#88312,#88313,#88314,#88315,#88316,#88317,#88318,#88319,#88320,
#88321,#88322,#88323,#88324,#88325,#88326,#88327,#88328,#88329,#88330,#88331,
#88332,#88333,#88334,#88335,#88336,#88337,#88338,#88339,#88340,#88341,#88342,
#88343,#88344,#88345,#88346,#88347,#88348,#88349,#88350,#88351,#88352,#88353,
#88354,#88355,#88356,#88357,#88358,#88359,#88360,#88361,#88362,#88363,#88364,
#88365,#88366,#88367,#88368,#88369,#88370,#88371,#88372,#88373,#88374,#88375,
#88376,#88377,#88378,#88379,#88380,#88381,#88382,#88383,#88384,#88385,#88386,
#88387,#88388,#88389,#88390,#88391,#88392,#88393,#88394,#88395,#88396,#88397,
#88398,#88399,#88400,#88401,#88402,#88403,#88404,#88405,#88406,#88407,#88408,
#88409,#88410,#88411,#88412,#88413,#88414,#88415,#88416,#88417,#88418,#88419,
#88420,#88421,#88422,#88423,#88424,#88425,#88426,#88427,#88428,#88429,#88430,
#88431,#88432,#88433,#88434,#88435,#88436,#88437,#88438,#88439,#88440,#88441,
#88442,#88443,#88444,#88445,#88446,#88447,#88448,#88449,#88450,#88451,#88452,
#88453,#88454,#88455,#88456,#88457,#88458,#88459,#88460,#88461,#88462,#88463,
#88464,#88465,#88466,#88467,#88468,#88469,#88470,#88471,#88472,#88473,#88474,
#88475,#88476,#88477,#88478,#88479,#88480,#88481,#88482,#88483,#88484,#88485,
#88486,#88487,#88488,#88489,#88490,#88491,#88492,#88493,#88494,#88495,#88496,
#88497,#88498,#88499,#88500,#88501,#88502,#88503,#88504,#88505,#88506,#88507,
#88508,#88509,#88510,#88511,#88512,#88513,#88514,#88515,#88516,#88517,#88518,
#88519,#88520,#88521,#88522,#88523,#88524,#88525,#88526,#88527,#88528,#88529,
#88530,#88531,#88532,#88533,#88534,#88535,#88536,#88537,#88538,#88539,#88540,
#88541,#88542,#88543,#88544,#88545,#88546,#88547,#88548,#88549,#88550,#88551,
#88552,#88553,#88554,#88555,#88556,#88557,#88558,#88559,#88560,#88561,#88562,
#88563,#88564,#88565,#88566,#88567,#88568,#88569,#88570,#88571,#88572,#88573,
#88574,#88575,#88576,#88577,#88578,#88579,#88580,#88581,#88582,#88583,#88584,
#88585,#88586,#88587,#88588,#88589,#88590,#88591,#88592,#88593,#88594,#88595,
#88596,#88597,#88598,#88599,#88600,#88601,#88602,#88603,#88604,#88605,#88606,
#88607,#88608,#88609,#88610,#88611,#88612,#88613,#88614,#88615,#88616,#88617,
#88618,#88619,#88620,#88621,#88622,#88623,#88624,#88625,#88626,#88627,#88628,
#88629,#88630,#88631,#88632,#88633,#88634,#88635,#88636,#88637,#88638,#88639,
#88640,#88641,#88642,#88643,#88644,#88645,#88646,#88647,#88648,#88649,#88650,
#88651,#88652,#88653,#88654,#88655,#88656,#88657,#88658,#88659,#88660,#88661,
#88662,#88663,#88664,#88665,#88666,#88667,#88668,#88669,#88670,#88671,#88672,
#88673,#88674,#88675,#88676,#88677,#88678,#88679,#88680,#88681,#88682,#88683,
#88684,#88685,#88686,#88687,#88688,#88689,#88690,#88691,#88692,#88693,#88694,
#88695,#88696,#88697,#88698,#88699,#88700,#88701,#88702,#88703,#88704,#88705,
#88706,#88707,#88708,#88709,#88710,#88711,#88712,#88713,#88714,#88715,#88716,
#88717)) ;
#93348=AXIS2_PLACEMENT_3D('',#141826,#108731,#108732) ;
#93349=AXIS2_PLACEMENT_3D('',#141827,#108733,#108734) ;
#93350=AXIS2_PLACEMENT_3D('',#141829,#108735,#108736) ;
#93351=AXIS2_PLACEMENT_3D('',#141831,#108737,#108738) ;
#93352=AXIS2_PLACEMENT_3D('',#141833,#108739,#108740) ;
#93353=AXIS2_PLACEMENT_3D('',#141834,#108741,#108742) ;
#93354=AXIS2_PLACEMENT_3D('',#141835,#108743,#108744) ;
#93355=AXIS2_PLACEMENT_3D('',#141837,#108745,#108746) ;
#93356=AXIS2_PLACEMENT_3D('',#141839,#108747,#108748) ;
#93357=AXIS2_PLACEMENT_3D('',#141840,#108749,#108750) ;
#93358=AXIS2_PLACEMENT_3D('',#141841,#108751,#108752) ;
#93359=AXIS2_PLACEMENT_3D('',#141844,#108753,#108754) ;
#93360=AXIS2_PLACEMENT_3D('',#141846,#108755,#108756) ;
#93361=AXIS2_PLACEMENT_3D('',#141847,#108757,#108758) ;
#93362=AXIS2_PLACEMENT_3D('',#141848,#108759,#108760) ;
#93363=AXIS2_PLACEMENT_3D('',#141851,#108761,#108762) ;
#93364=AXIS2_PLACEMENT_3D('',#141853,#108763,#108764) ;
#93365=AXIS2_PLACEMENT_3D('',#141857,#108766,#108767) ;
#93366=AXIS2_PLACEMENT_3D('',#141870,#108770,#108771) ;
#93367=AXIS2_PLACEMENT_3D('',#141872,#108772,#108773) ;
#93368=AXIS2_PLACEMENT_3D('',#141874,#108774,#108775) ;
#93369=AXIS2_PLACEMENT_3D('',#141876,#108776,#108777) ;
#93370=AXIS2_PLACEMENT_3D('',#141877,#108778,#108779) ;
#93371=AXIS2_PLACEMENT_3D('',#141878,#108780,#108781) ;
#93372=AXIS2_PLACEMENT_3D('',#141880,#108782,#108783) ;
#93373=AXIS2_PLACEMENT_3D('',#141882,#108784,#108785) ;
#93374=AXIS2_PLACEMENT_3D('',#141883,#108786,#108787) ;
#93375=AXIS2_PLACEMENT_3D('',#141884,#108788,#108789) ;
#93376=AXIS2_PLACEMENT_3D('',#141887,#108790,#108791) ;
#93377=AXIS2_PLACEMENT_3D('',#141889,#108792,#108793) ;
#93378=AXIS2_PLACEMENT_3D('',#141890,#108794,#108795) ;
#93379=AXIS2_PLACEMENT_3D('',#141891,#108796,#108797) ;
#93380=AXIS2_PLACEMENT_3D('',#141894,#108798,#108799) ;
#93381=AXIS2_PLACEMENT_3D('',#141896,#108800,#108801) ;
#93382=AXIS2_PLACEMENT_3D('',#141900,#108803,#108804) ;
#93383=AXIS2_PLACEMENT_3D('',#141913,#108807,#108808) ;
#93384=AXIS2_PLACEMENT_3D('',#141915,#108809,#108810) ;
#93385=AXIS2_PLACEMENT_3D('',#141917,#108811,#108812) ;
#93386=AXIS2_PLACEMENT_3D('',#141919,#108813,#108814) ;
#93387=AXIS2_PLACEMENT_3D('',#141920,#108815,#108816) ;
#93388=AXIS2_PLACEMENT_3D('',#141921,#108817,#108818) ;
#93389=AXIS2_PLACEMENT_3D('',#141923,#108819,#108820) ;
#93390=AXIS2_PLACEMENT_3D('',#141925,#108821,#108822) ;
#93391=AXIS2_PLACEMENT_3D('',#141926,#108823,#108824) ;
#93392=AXIS2_PLACEMENT_3D('',#141927,#108825,#108826) ;
#93393=AXIS2_PLACEMENT_3D('',#141930,#108827,#108828) ;
#93394=AXIS2_PLACEMENT_3D('',#141932,#108829,#108830) ;
#93395=AXIS2_PLACEMENT_3D('',#141933,#108831,#108832) ;
#93396=AXIS2_PLACEMENT_3D('',#141934,#108833,#108834) ;
#93397=AXIS2_PLACEMENT_3D('',#141937,#108835,#108836) ;
#93398=AXIS2_PLACEMENT_3D('',#141939,#108837,#108838) ;
#93399=AXIS2_PLACEMENT_3D('',#141943,#108840,#108841) ;
#93400=AXIS2_PLACEMENT_3D('',#141956,#108844,#108845) ;
#93401=AXIS2_PLACEMENT_3D('',#141958,#108846,#108847) ;
#93402=AXIS2_PLACEMENT_3D('',#141960,#108848,#108849) ;
#93403=AXIS2_PLACEMENT_3D('',#141962,#108850,#108851) ;
#93404=AXIS2_PLACEMENT_3D('',#141963,#108852,#108853) ;
#93405=AXIS2_PLACEMENT_3D('',#141964,#108854,#108855) ;
#93406=AXIS2_PLACEMENT_3D('',#141966,#108856,#108857) ;
#93407=AXIS2_PLACEMENT_3D('',#141968,#108858,#108859) ;
#93408=AXIS2_PLACEMENT_3D('',#141969,#108860,#108861) ;
#93409=AXIS2_PLACEMENT_3D('',#141970,#108862,#108863) ;
#93410=AXIS2_PLACEMENT_3D('',#141973,#108864,#108865) ;
#93411=AXIS2_PLACEMENT_3D('',#141975,#108866,#108867) ;
#93412=AXIS2_PLACEMENT_3D('',#141976,#108868,#108869) ;
#93413=AXIS2_PLACEMENT_3D('',#141977,#108870,#108871) ;
#93414=AXIS2_PLACEMENT_3D('',#141980,#108872,#108873) ;
#93415=AXIS2_PLACEMENT_3D('',#141982,#108874,#108875) ;
#93416=AXIS2_PLACEMENT_3D('',#141986,#108877,#108878) ;
#93417=AXIS2_PLACEMENT_3D('',#141999,#108881,#108882) ;
#93418=AXIS2_PLACEMENT_3D('',#142001,#108883,#108884) ;
#93419=AXIS2_PLACEMENT_3D('',#142003,#108885,#108886) ;
#93420=AXIS2_PLACEMENT_3D('',#142005,#108887,#108888) ;
#93421=AXIS2_PLACEMENT_3D('',#142006,#108889,#108890) ;
#93422=AXIS2_PLACEMENT_3D('',#142007,#108891,#108892) ;
#93423=AXIS2_PLACEMENT_3D('',#142009,#108893,#108894) ;
#93424=AXIS2_PLACEMENT_3D('',#142011,#108895,#108896) ;
#93425=AXIS2_PLACEMENT_3D('',#142012,#108897,#108898) ;
#93426=AXIS2_PLACEMENT_3D('',#142013,#108899,#108900) ;
#93427=AXIS2_PLACEMENT_3D('',#142016,#108901,#108902) ;
#93428=AXIS2_PLACEMENT_3D('',#142018,#108903,#108904) ;
#93429=AXIS2_PLACEMENT_3D('',#142019,#108905,#108906) ;
#93430=AXIS2_PLACEMENT_3D('',#142020,#108907,#108908) ;
#93431=AXIS2_PLACEMENT_3D('',#142023,#108909,#108910) ;
#93432=AXIS2_PLACEMENT_3D('',#142025,#108911,#108912) ;
#93433=AXIS2_PLACEMENT_3D('',#142029,#108914,#108915) ;
#93434=AXIS2_PLACEMENT_3D('',#142042,#108918,#108919) ;
#93435=AXIS2_PLACEMENT_3D('',#142044,#108920,#108921) ;
#93436=AXIS2_PLACEMENT_3D('',#142046,#108922,#108923) ;
#93437=AXIS2_PLACEMENT_3D('',#142048,#108924,#108925) ;
#93438=AXIS2_PLACEMENT_3D('',#142049,#108926,#108927) ;
#93439=AXIS2_PLACEMENT_3D('',#142050,#108928,#108929) ;
#93440=AXIS2_PLACEMENT_3D('',#142052,#108930,#108931) ;
#93441=AXIS2_PLACEMENT_3D('',#142054,#108932,#108933) ;
#93442=AXIS2_PLACEMENT_3D('',#142055,#108934,#108935) ;
#93443=AXIS2_PLACEMENT_3D('',#142056,#108936,#108937) ;
#93444=AXIS2_PLACEMENT_3D('',#142059,#108938,#108939) ;
#93445=AXIS2_PLACEMENT_3D('',#142061,#108940,#108941) ;
#93446=AXIS2_PLACEMENT_3D('',#142062,#108942,#108943) ;
#93447=AXIS2_PLACEMENT_3D('',#142063,#108944,#108945) ;
#93448=AXIS2_PLACEMENT_3D('',#142066,#108946,#108947) ;
#93449=AXIS2_PLACEMENT_3D('',#142068,#108948,#108949) ;
#93450=AXIS2_PLACEMENT_3D('',#142072,#108951,#108952) ;
#93451=AXIS2_PLACEMENT_3D('',#142085,#108955,#108956) ;
#93452=AXIS2_PLACEMENT_3D('',#142087,#108957,#108958) ;
#93453=AXIS2_PLACEMENT_3D('',#142089,#108959,#108960) ;
#93454=AXIS2_PLACEMENT_3D('',#142091,#108961,#108962) ;
#93455=AXIS2_PLACEMENT_3D('',#142092,#108963,#108964) ;
#93456=AXIS2_PLACEMENT_3D('',#142093,#108965,#108966) ;
#93457=AXIS2_PLACEMENT_3D('',#142095,#108967,#108968) ;
#93458=AXIS2_PLACEMENT_3D('',#142097,#108969,#108970) ;
#93459=AXIS2_PLACEMENT_3D('',#142098,#108971,#108972) ;
#93460=AXIS2_PLACEMENT_3D('',#142099,#108973,#108974) ;
#93461=AXIS2_PLACEMENT_3D('',#142102,#108975,#108976) ;
#93462=AXIS2_PLACEMENT_3D('',#142104,#108977,#108978) ;
#93463=AXIS2_PLACEMENT_3D('',#142105,#108979,#108980) ;
#93464=AXIS2_PLACEMENT_3D('',#142106,#108981,#108982) ;
#93465=AXIS2_PLACEMENT_3D('',#142109,#108983,#108984) ;
#93466=AXIS2_PLACEMENT_3D('',#142111,#108985,#108986) ;
#93467=AXIS2_PLACEMENT_3D('',#142115,#108988,#108989) ;
#93468=AXIS2_PLACEMENT_3D('',#142128,#108992,#108993) ;
#93469=AXIS2_PLACEMENT_3D('',#142130,#108994,#108995) ;
#93470=AXIS2_PLACEMENT_3D('',#142132,#108996,#108997) ;
#93471=AXIS2_PLACEMENT_3D('',#142134,#108998,#108999) ;
#93472=AXIS2_PLACEMENT_3D('',#142135,#109000,#109001) ;
#93473=AXIS2_PLACEMENT_3D('',#142136,#109002,#109003) ;
#93474=AXIS2_PLACEMENT_3D('',#142138,#109004,#109005) ;
#93475=AXIS2_PLACEMENT_3D('',#142140,#109006,#109007) ;
#93476=AXIS2_PLACEMENT_3D('',#142141,#109008,#109009) ;
#93477=AXIS2_PLACEMENT_3D('',#142142,#109010,#109011) ;
#93478=AXIS2_PLACEMENT_3D('',#142145,#109012,#109013) ;
#93479=AXIS2_PLACEMENT_3D('',#142147,#109014,#109015) ;
#93480=AXIS2_PLACEMENT_3D('',#142148,#109016,#109017) ;
#93481=AXIS2_PLACEMENT_3D('',#142149,#109018,#109019) ;
#93482=AXIS2_PLACEMENT_3D('',#142152,#109020,#109021) ;
#93483=AXIS2_PLACEMENT_3D('',#142154,#109022,#109023) ;
#93484=AXIS2_PLACEMENT_3D('',#142158,#109025,#109026) ;
#93485=AXIS2_PLACEMENT_3D('',#142171,#109029,#109030) ;
#93486=AXIS2_PLACEMENT_3D('',#142173,#109031,#109032) ;
#93487=AXIS2_PLACEMENT_3D('',#142175,#109033,#109034) ;
#93488=AXIS2_PLACEMENT_3D('',#142177,#109035,#109036) ;
#93489=AXIS2_PLACEMENT_3D('',#142178,#109037,#109038) ;
#93490=AXIS2_PLACEMENT_3D('',#142179,#109039,#109040) ;
#93491=AXIS2_PLACEMENT_3D('',#142182,#109041,#109042) ;
#93492=AXIS2_PLACEMENT_3D('',#142184,#109043,#109044) ;
#93493=AXIS2_PLACEMENT_3D('',#142186,#109045,#109046) ;
#93494=AXIS2_PLACEMENT_3D('',#142187,#109047,#109048) ;
#93495=AXIS2_PLACEMENT_3D('',#142188,#109049,#109050) ;
#93496=AXIS2_PLACEMENT_3D('',#142191,#109051,#109052) ;
#93497=AXIS2_PLACEMENT_3D('',#142193,#109053,#109054) ;
#93498=AXIS2_PLACEMENT_3D('',#142195,#109055,#109056) ;
#93499=AXIS2_PLACEMENT_3D('',#142196,#109057,#109058) ;
#93500=AXIS2_PLACEMENT_3D('',#142197,#109059,#109060) ;
#93501=AXIS2_PLACEMENT_3D('',#142200,#109061,#109062) ;
#93502=AXIS2_PLACEMENT_3D('',#142202,#109063,#109064) ;
#93503=AXIS2_PLACEMENT_3D('',#142204,#109065,#109066) ;
#93504=AXIS2_PLACEMENT_3D('',#142205,#109067,#109068) ;
#93505=AXIS2_PLACEMENT_3D('',#142206,#109069,#109070) ;
#93506=AXIS2_PLACEMENT_3D('',#142209,#109071,#109072) ;
#93507=AXIS2_PLACEMENT_3D('',#142211,#109073,#109074) ;
#93508=AXIS2_PLACEMENT_3D('',#142213,#109075,#109076) ;
#93509=AXIS2_PLACEMENT_3D('',#142214,#109077,#109078) ;
#93510=AXIS2_PLACEMENT_3D('',#142215,#109079,#109080) ;
#93511=AXIS2_PLACEMENT_3D('',#142218,#109081,#109082) ;
#93512=AXIS2_PLACEMENT_3D('',#142220,#109083,#109084) ;
#93513=AXIS2_PLACEMENT_3D('',#142222,#109085,#109086) ;
#93514=AXIS2_PLACEMENT_3D('',#142223,#109087,#109088) ;
#93515=AXIS2_PLACEMENT_3D('',#142224,#109089,#109090) ;
#93516=AXIS2_PLACEMENT_3D('',#142227,#109091,#109092) ;
#93517=AXIS2_PLACEMENT_3D('',#142229,#109093,#109094) ;
#93518=AXIS2_PLACEMENT_3D('',#142231,#109095,#109096) ;
#93519=AXIS2_PLACEMENT_3D('',#142232,#109097,#109098) ;
#93520=AXIS2_PLACEMENT_3D('',#142233,#109099,#109100) ;
#93521=AXIS2_PLACEMENT_3D('',#142236,#109101,#109102) ;
#93522=AXIS2_PLACEMENT_3D('',#142238,#109103,#109104) ;
#93523=AXIS2_PLACEMENT_3D('',#142240,#109105,#109106) ;
#93524=AXIS2_PLACEMENT_3D('',#142241,#109107,#109108) ;
#93525=AXIS2_PLACEMENT_3D('',#142242,#109109,#109110) ;
#93526=AXIS2_PLACEMENT_3D('',#142245,#109111,#109112) ;
#93527=AXIS2_PLACEMENT_3D('',#142247,#109113,#109114) ;
#93528=AXIS2_PLACEMENT_3D('',#142249,#109115,#109116) ;
#93529=AXIS2_PLACEMENT_3D('',#142250,#109117,#109118) ;
#93530=AXIS2_PLACEMENT_3D('',#142251,#109119,#109120) ;
#93531=AXIS2_PLACEMENT_3D('',#142254,#109121,#109122) ;
#93532=AXIS2_PLACEMENT_3D('',#142256,#109123,#109124) ;
#93533=AXIS2_PLACEMENT_3D('',#142258,#109125,#109126) ;
#93534=AXIS2_PLACEMENT_3D('',#142259,#109127,#109128) ;
#93535=AXIS2_PLACEMENT_3D('',#142260,#109129,#109130) ;
#93536=AXIS2_PLACEMENT_3D('',#142262,#109131,#109132) ;
#93537=AXIS2_PLACEMENT_3D('',#142264,#109133,#109134) ;
#93538=AXIS2_PLACEMENT_3D('',#142265,#109135,#109136) ;
#93539=AXIS2_PLACEMENT_3D('',#142266,#109137,#109138) ;
#93540=AXIS2_PLACEMENT_3D('',#142269,#109139,#109140) ;
#93541=AXIS2_PLACEMENT_3D('',#142271,#109141,#109142) ;
#93542=AXIS2_PLACEMENT_3D('',#142272,#109143,#109144) ;
#93543=AXIS2_PLACEMENT_3D('',#142273,#109145,#109146) ;
#93544=AXIS2_PLACEMENT_3D('',#142276,#109147,#109148) ;
#93545=AXIS2_PLACEMENT_3D('',#142278,#109149,#109150) ;
#93546=AXIS2_PLACEMENT_3D('',#142282,#109152,#109153) ;
#93547=AXIS2_PLACEMENT_3D('',#142295,#109156,#109157) ;
#93548=AXIS2_PLACEMENT_3D('',#142297,#109159,#109160) ;
#93549=AXIS2_PLACEMENT_3D('',#142299,#109162,#109163) ;
#93550=AXIS2_PLACEMENT_3D('',#142301,#109165,#109166) ;
#93551=AXIS2_PLACEMENT_3D('',#142303,#109168,#109169) ;
#93552=AXIS2_PLACEMENT_3D('',#142305,#109171,#109172) ;
#93553=AXIS2_PLACEMENT_3D('',#142307,#109174,#109175) ;
#93554=AXIS2_PLACEMENT_3D('',#142309,#109177,#109178) ;
#93555=AXIS2_PLACEMENT_3D('',#142311,#109180,#109181) ;
#93556=AXIS2_PLACEMENT_3D('',#142313,#109183,#109184) ;
#93557=AXIS2_PLACEMENT_3D('',#142316,#109185,#109186) ;
#93558=AXIS2_PLACEMENT_3D('',#142319,#109189,#109190) ;
#93559=AXIS2_PLACEMENT_3D('',#142322,#109191,#109192) ;
#93560=AXIS2_PLACEMENT_3D('',#142325,#109195,#109196) ;
#93561=AXIS2_PLACEMENT_3D('',#142328,#109197,#109198) ;
#93562=AXIS2_PLACEMENT_3D('',#142331,#109201,#109202) ;
#93563=AXIS2_PLACEMENT_3D('',#142334,#109203,#109204) ;
#93564=AXIS2_PLACEMENT_3D('',#142337,#109207,#109208) ;
#93565=AXIS2_PLACEMENT_3D('',#142340,#109209,#109210) ;
#93566=AXIS2_PLACEMENT_3D('',#142343,#109213,#109214) ;
#93567=AXIS2_PLACEMENT_3D('',#142346,#109215,#109216) ;
#93568=AXIS2_PLACEMENT_3D('',#142349,#109219,#109220) ;
#93569=AXIS2_PLACEMENT_3D('',#142352,#109221,#109222) ;
#93570=AXIS2_PLACEMENT_3D('',#142355,#109225,#109226) ;
#93571=AXIS2_PLACEMENT_3D('',#142358,#109227,#109228) ;
#93572=AXIS2_PLACEMENT_3D('',#142361,#109231,#109232) ;
#93573=AXIS2_PLACEMENT_3D('',#142364,#109233,#109234) ;
#93574=AXIS2_PLACEMENT_3D('',#142367,#109237,#109238) ;
#93575=AXIS2_PLACEMENT_3D('',#142369,#109239,#109240) ;
#93576=AXIS2_PLACEMENT_3D('',#142371,#109241,#109242) ;
#93577=AXIS2_PLACEMENT_3D('',#142373,#109243,#109244) ;
#93578=AXIS2_PLACEMENT_3D('',#142374,#109245,#109246) ;
#93579=AXIS2_PLACEMENT_3D('',#142375,#109247,#109248) ;
#93580=AXIS2_PLACEMENT_3D('',#142378,#109249,#109250) ;
#93581=AXIS2_PLACEMENT_3D('',#142380,#109251,#109252) ;
#93582=AXIS2_PLACEMENT_3D('',#142382,#109253,#109254) ;
#93583=AXIS2_PLACEMENT_3D('',#142383,#109255,#109256) ;
#93584=AXIS2_PLACEMENT_3D('',#142384,#109257,#109258) ;
#93585=AXIS2_PLACEMENT_3D('',#142386,#109259,#109260) ;
#93586=AXIS2_PLACEMENT_3D('',#142388,#109261,#109262) ;
#93587=AXIS2_PLACEMENT_3D('',#142389,#109263,#109264) ;
#93588=AXIS2_PLACEMENT_3D('',#142390,#109265,#109266) ;
#93589=AXIS2_PLACEMENT_3D('',#142393,#109267,#109268) ;
#93590=AXIS2_PLACEMENT_3D('',#142395,#109269,#109270) ;
#93591=AXIS2_PLACEMENT_3D('',#142396,#109271,#109272) ;
#93592=AXIS2_PLACEMENT_3D('',#142397,#109273,#109274) ;
#93593=AXIS2_PLACEMENT_3D('',#142400,#109275,#109276) ;
#93594=AXIS2_PLACEMENT_3D('',#142402,#109277,#109278) ;
#93595=AXIS2_PLACEMENT_3D('',#142406,#109280,#109281) ;
#93596=AXIS2_PLACEMENT_3D('',#142419,#109284,#109285) ;
#93597=AXIS2_PLACEMENT_3D('',#142421,#109287,#109288) ;
#93598=AXIS2_PLACEMENT_3D('',#142424,#109289,#109290) ;
#93599=AXIS2_PLACEMENT_3D('',#142427,#109293,#109294) ;
#93600=AXIS2_PLACEMENT_3D('',#142432,#109296,#109297) ;
#93601=AXIS2_PLACEMENT_3D('',#142435,#109299,#109300) ;
#93602=AXIS2_PLACEMENT_3D('',#142437,#109301,#109302) ;
#93603=AXIS2_PLACEMENT_3D('',#142448,#109308,#109309) ;
#93604=AXIS2_PLACEMENT_3D('',#142449,#109310,#109311) ;
#93605=AXIS2_PLACEMENT_3D('',#142454,#109313,#109314) ;
#93606=AXIS2_PLACEMENT_3D('',#142457,#109316,#109317) ;
#93607=AXIS2_PLACEMENT_3D('',#142459,#109318,#109319) ;
#93608=AXIS2_PLACEMENT_3D('',#142470,#109325,#109326) ;
#93609=AXIS2_PLACEMENT_3D('',#142471,#109327,#109328) ;
#93610=AXIS2_PLACEMENT_3D('',#142476,#109330,#109331) ;
#93611=AXIS2_PLACEMENT_3D('',#142479,#109333,#109334) ;
#93612=AXIS2_PLACEMENT_3D('',#142481,#109335,#109336) ;
#93613=AXIS2_PLACEMENT_3D('',#142492,#109342,#109343) ;
#93614=AXIS2_PLACEMENT_3D('',#142493,#109344,#109345) ;
#93615=AXIS2_PLACEMENT_3D('',#142498,#109347,#109348) ;
#93616=AXIS2_PLACEMENT_3D('',#142501,#109350,#109351) ;
#93617=AXIS2_PLACEMENT_3D('',#142503,#109352,#109353) ;
#93618=AXIS2_PLACEMENT_3D('',#142514,#109359,#109360) ;
#93619=AXIS2_PLACEMENT_3D('',#142515,#109361,#109362) ;
#93620=AXIS2_PLACEMENT_3D('',#142520,#109364,#109365) ;
#93621=AXIS2_PLACEMENT_3D('',#142523,#109367,#109368) ;
#93622=AXIS2_PLACEMENT_3D('',#142525,#109369,#109370) ;
#93623=AXIS2_PLACEMENT_3D('',#142536,#109376,#109377) ;
#93624=AXIS2_PLACEMENT_3D('',#142537,#109378,#109379) ;
#93625=AXIS2_PLACEMENT_3D('',#142542,#109381,#109382) ;
#93626=AXIS2_PLACEMENT_3D('',#142545,#109384,#109385) ;
#93627=AXIS2_PLACEMENT_3D('',#142547,#109386,#109387) ;
#93628=AXIS2_PLACEMENT_3D('',#142558,#109393,#109394) ;
#93629=AXIS2_PLACEMENT_3D('',#142559,#109395,#109396) ;
#93630=AXIS2_PLACEMENT_3D('',#142564,#109398,#109399) ;
#93631=AXIS2_PLACEMENT_3D('',#142567,#109401,#109402) ;
#93632=AXIS2_PLACEMENT_3D('',#142569,#109403,#109404) ;
#93633=AXIS2_PLACEMENT_3D('',#142580,#109410,#109411) ;
#93634=AXIS2_PLACEMENT_3D('',#142581,#109412,#109413) ;
#93635=AXIS2_PLACEMENT_3D('',#142586,#109415,#109416) ;
#93636=AXIS2_PLACEMENT_3D('',#142589,#109418,#109419) ;
#93637=AXIS2_PLACEMENT_3D('',#142591,#109420,#109421) ;
#93638=AXIS2_PLACEMENT_3D('',#142602,#109427,#109428) ;
#93639=AXIS2_PLACEMENT_3D('',#142603,#109429,#109430) ;
#93640=AXIS2_PLACEMENT_3D('',#142608,#109432,#109433) ;
#93641=AXIS2_PLACEMENT_3D('',#142611,#109435,#109436) ;
#93642=AXIS2_PLACEMENT_3D('',#142613,#109437,#109438) ;
#93643=AXIS2_PLACEMENT_3D('',#142624,#109444,#109445) ;
#93644=AXIS2_PLACEMENT_3D('',#142625,#109446,#109447) ;
#93645=AXIS2_PLACEMENT_3D('',#142628,#109448,#109449) ;
#93646=AXIS2_PLACEMENT_3D('',#142636,#109454,#109455) ;
#93647=AXIS2_PLACEMENT_3D('',#142639,#109456,#109457) ;
#93648=AXIS2_PLACEMENT_3D('',#142647,#109462,#109463) ;
#93649=AXIS2_PLACEMENT_3D('',#142650,#109464,#109465) ;
#93650=AXIS2_PLACEMENT_3D('',#142658,#109470,#109471) ;
#93651=AXIS2_PLACEMENT_3D('',#142661,#109472,#109473) ;
#93652=AXIS2_PLACEMENT_3D('',#142669,#109478,#109479) ;
#93653=AXIS2_PLACEMENT_3D('',#142672,#109480,#109481) ;
#93654=AXIS2_PLACEMENT_3D('',#142680,#109486,#109487) ;
#93655=AXIS2_PLACEMENT_3D('',#142683,#109488,#109489) ;
#93656=AXIS2_PLACEMENT_3D('',#142691,#109494,#109495) ;
#93657=AXIS2_PLACEMENT_3D('',#142694,#109496,#109497) ;
#93658=AXIS2_PLACEMENT_3D('',#142702,#109502,#109503) ;
#93659=AXIS2_PLACEMENT_3D('',#142705,#109504,#109505) ;
#93660=AXIS2_PLACEMENT_3D('',#142713,#109510,#109511) ;
#93661=AXIS2_PLACEMENT_3D('',#142716,#109512,#109513) ;
#93662=AXIS2_PLACEMENT_3D('',#142724,#109518,#109519) ;
#93663=AXIS2_PLACEMENT_3D('',#142727,#109520,#109521) ;
#93664=AXIS2_PLACEMENT_3D('',#142735,#109526,#109527) ;
#93665=AXIS2_PLACEMENT_3D('',#142738,#109528,#109529) ;
#93666=AXIS2_PLACEMENT_3D('',#142746,#109534,#109535) ;
#93667=AXIS2_PLACEMENT_3D('',#142749,#109536,#109537) ;
#93668=AXIS2_PLACEMENT_3D('',#142757,#109542,#109543) ;
#93669=AXIS2_PLACEMENT_3D('',#142760,#109544,#109545) ;
#93670=AXIS2_PLACEMENT_3D('',#142768,#109550,#109551) ;
#93671=AXIS2_PLACEMENT_3D('',#142771,#109552,#109553) ;
#93672=AXIS2_PLACEMENT_3D('',#142779,#109558,#109559) ;
#93673=AXIS2_PLACEMENT_3D('',#142782,#109560,#109561) ;
#93674=AXIS2_PLACEMENT_3D('',#142790,#109566,#109567) ;
#93675=AXIS2_PLACEMENT_3D('',#142793,#109568,#109569) ;
#93676=AXIS2_PLACEMENT_3D('',#142801,#109574,#109575) ;
#93677=AXIS2_PLACEMENT_3D('',#142804,#109576,#109577) ;
#93678=AXIS2_PLACEMENT_3D('',#142812,#109582,#109583) ;
#93679=AXIS2_PLACEMENT_3D('',#142815,#109584,#109585) ;
#93680=AXIS2_PLACEMENT_3D('',#142823,#109590,#109591) ;
#93681=AXIS2_PLACEMENT_3D('',#142828,#109593,#109594) ;
#93682=AXIS2_PLACEMENT_3D('',#142831,#109596,#109597) ;
#93683=AXIS2_PLACEMENT_3D('',#142832,#109598,#109599) ;
#93684=AXIS2_PLACEMENT_3D('',#142837,#109601,#109602) ;
#93685=AXIS2_PLACEMENT_3D('',#142840,#109604,#109605) ;
#93686=AXIS2_PLACEMENT_3D('',#142841,#109606,#109607) ;
#93687=AXIS2_PLACEMENT_3D('',#142846,#109609,#109610) ;
#93688=AXIS2_PLACEMENT_3D('',#142849,#109612,#109613) ;
#93689=AXIS2_PLACEMENT_3D('',#142850,#109614,#109615) ;
#93690=AXIS2_PLACEMENT_3D('',#142855,#109617,#109618) ;
#93691=AXIS2_PLACEMENT_3D('',#142858,#109620,#109621) ;
#93692=AXIS2_PLACEMENT_3D('',#142859,#109622,#109623) ;
#93693=AXIS2_PLACEMENT_3D('',#142864,#109625,#109626) ;
#93694=AXIS2_PLACEMENT_3D('',#142867,#109628,#109629) ;
#93695=AXIS2_PLACEMENT_3D('',#142868,#109630,#109631) ;
#93696=AXIS2_PLACEMENT_3D('',#142873,#109633,#109634) ;
#93697=AXIS2_PLACEMENT_3D('',#142876,#109636,#109637) ;
#93698=AXIS2_PLACEMENT_3D('',#142877,#109638,#109639) ;
#93699=AXIS2_PLACEMENT_3D('',#142882,#109641,#109642) ;
#93700=AXIS2_PLACEMENT_3D('',#142885,#109644,#109645) ;
#93701=AXIS2_PLACEMENT_3D('',#142886,#109646,#109647) ;
#93702=AXIS2_PLACEMENT_3D('',#142891,#109649,#109650) ;
#93703=AXIS2_PLACEMENT_3D('',#142894,#109652,#109653) ;
#93704=AXIS2_PLACEMENT_3D('',#142895,#109654,#109655) ;
#93705=AXIS2_PLACEMENT_3D('',#142900,#109657,#109658) ;
#93706=AXIS2_PLACEMENT_3D('',#142903,#109660,#109661) ;
#93707=AXIS2_PLACEMENT_3D('',#142904,#109662,#109663) ;
#93708=AXIS2_PLACEMENT_3D('',#142909,#109665,#109666) ;
#93709=AXIS2_PLACEMENT_3D('',#142912,#109668,#109669) ;
#93710=AXIS2_PLACEMENT_3D('',#142914,#109670,#109671) ;
#93711=AXIS2_PLACEMENT_3D('',#142925,#109677,#109678) ;
#93712=AXIS2_PLACEMENT_3D('',#142926,#109679,#109680) ;
#93713=AXIS2_PLACEMENT_3D('',#142929,#109681,#109682) ;
#93714=AXIS2_PLACEMENT_3D('',#142937,#109687,#109688) ;
#93715=AXIS2_PLACEMENT_3D('',#142940,#109689,#109690) ;
#93716=AXIS2_PLACEMENT_3D('',#142948,#109695,#109696) ;
#93717=AXIS2_PLACEMENT_3D('',#142953,#109698,#109699) ;
#93718=AXIS2_PLACEMENT_3D('',#142956,#109701,#109702) ;
#93719=AXIS2_PLACEMENT_3D('',#142957,#109703,#109704) ;
#93720=AXIS2_PLACEMENT_3D('',#142962,#109706,#109707) ;
#93721=AXIS2_PLACEMENT_3D('',#142965,#109709,#109710) ;
#93722=AXIS2_PLACEMENT_3D('',#142966,#109711,#109712) ;
#93723=AXIS2_PLACEMENT_3D('',#142969,#109713,#109714) ;
#93724=AXIS2_PLACEMENT_3D('',#142979,#109720,#109721) ;
#93725=AXIS2_PLACEMENT_3D('',#142983,#109723,#109724) ;
#93726=AXIS2_PLACEMENT_3D('',#142988,#109727,#109728) ;
#93727=AXIS2_PLACEMENT_3D('',#142992,#109730,#109731) ;
#93728=AXIS2_PLACEMENT_3D('',#142997,#109734,#109735) ;
#93729=AXIS2_PLACEMENT_3D('',#143001,#109737,#109738) ;
#93730=AXIS2_PLACEMENT_3D('',#143006,#109741,#109742) ;
#93731=AXIS2_PLACEMENT_3D('',#143010,#109744,#109745) ;
#93732=AXIS2_PLACEMENT_3D('',#143015,#109748,#109749) ;
#93733=AXIS2_PLACEMENT_3D('',#143019,#109751,#109752) ;
#93734=AXIS2_PLACEMENT_3D('',#143024,#109755,#109756) ;
#93735=AXIS2_PLACEMENT_3D('',#143028,#109758,#109759) ;
#93736=AXIS2_PLACEMENT_3D('',#143033,#109762,#109763) ;
#93737=AXIS2_PLACEMENT_3D('',#143037,#109765,#109766) ;
#93738=AXIS2_PLACEMENT_3D('',#143042,#109769,#109770) ;
#93739=AXIS2_PLACEMENT_3D('',#143046,#109772,#109773) ;
#93740=AXIS2_PLACEMENT_3D('',#143051,#109776,#109777) ;
#93741=AXIS2_PLACEMENT_3D('',#143055,#109779,#109780) ;
#93742=AXIS2_PLACEMENT_3D('',#143060,#109783,#109784) ;
#93743=AXIS2_PLACEMENT_3D('',#143062,#109786,#109787) ;
#93744=AXIS2_PLACEMENT_3D('',#143064,#109788,#109789) ;
#93745=AXIS2_PLACEMENT_3D('',#143067,#109791,#109792) ;
#93746=AXIS2_PLACEMENT_3D('',#143068,#109793,#109794) ;
#93747=AXIS2_PLACEMENT_3D('',#143071,#109795,#109796) ;
#93748=AXIS2_PLACEMENT_3D('',#143076,#109799,#109800) ;
#93749=AXIS2_PLACEMENT_3D('',#143080,#109802,#109803) ;
#93750=AXIS2_PLACEMENT_3D('',#143085,#109806,#109807) ;
#93751=AXIS2_PLACEMENT_3D('',#143089,#109809,#109810) ;
#93752=AXIS2_PLACEMENT_3D('',#143094,#109813,#109814) ;
#93753=AXIS2_PLACEMENT_3D('',#143098,#109816,#109817) ;
#93754=AXIS2_PLACEMENT_3D('',#143103,#109820,#109821) ;
#93755=AXIS2_PLACEMENT_3D('',#143107,#109823,#109824) ;
#93756=AXIS2_PLACEMENT_3D('',#143112,#109827,#109828) ;
#93757=AXIS2_PLACEMENT_3D('',#143116,#109830,#109831) ;
#93758=AXIS2_PLACEMENT_3D('',#143121,#109834,#109835) ;
#93759=AXIS2_PLACEMENT_3D('',#143125,#109837,#109838) ;
#93760=AXIS2_PLACEMENT_3D('',#143130,#109841,#109842) ;
#93761=AXIS2_PLACEMENT_3D('',#143134,#109844,#109845) ;
#93762=AXIS2_PLACEMENT_3D('',#143139,#109848,#109849) ;
#93763=AXIS2_PLACEMENT_3D('',#143143,#109851,#109852) ;
#93764=AXIS2_PLACEMENT_3D('',#143148,#109855,#109856) ;
#93765=AXIS2_PLACEMENT_3D('',#143152,#109858,#109859) ;
#93766=AXIS2_PLACEMENT_3D('',#143162,#109865,#109866) ;
#93767=AXIS2_PLACEMENT_3D('',#143164,#109868,#109869) ;
#93768=AXIS2_PLACEMENT_3D('',#143168,#109871,#109872) ;
#93769=AXIS2_PLACEMENT_3D('',#143169,#109873,#109874) ;
#93770=AXIS2_PLACEMENT_3D('',#143170,#109875,#109876) ;
#93771=AXIS2_PLACEMENT_3D('',#143176,#109880,#109881) ;
#93772=AXIS2_PLACEMENT_3D('',#143180,#109883,#109884) ;
#93773=AXIS2_PLACEMENT_3D('',#143181,#109885,#109886) ;
#93774=AXIS2_PLACEMENT_3D('',#143182,#109887,#109888) ;
#93775=AXIS2_PLACEMENT_3D('',#143188,#109892,#109893) ;
#93776=AXIS2_PLACEMENT_3D('',#143192,#109895,#109896) ;
#93777=AXIS2_PLACEMENT_3D('',#143193,#109897,#109898) ;
#93778=AXIS2_PLACEMENT_3D('',#143194,#109899,#109900) ;
#93779=AXIS2_PLACEMENT_3D('',#143200,#109904,#109905) ;
#93780=AXIS2_PLACEMENT_3D('',#143204,#109907,#109908) ;
#93781=AXIS2_PLACEMENT_3D('',#143205,#109909,#109910) ;
#93782=AXIS2_PLACEMENT_3D('',#143206,#109911,#109912) ;
#93783=AXIS2_PLACEMENT_3D('',#143212,#109916,#109917) ;
#93784=AXIS2_PLACEMENT_3D('',#143216,#109919,#109920) ;
#93785=AXIS2_PLACEMENT_3D('',#143217,#109921,#109922) ;
#93786=AXIS2_PLACEMENT_3D('',#143218,#109923,#109924) ;
#93787=AXIS2_PLACEMENT_3D('',#143224,#109928,#109929) ;
#93788=AXIS2_PLACEMENT_3D('',#143228,#109931,#109932) ;
#93789=AXIS2_PLACEMENT_3D('',#143229,#109933,#109934) ;
#93790=AXIS2_PLACEMENT_3D('',#143230,#109935,#109936) ;
#93791=AXIS2_PLACEMENT_3D('',#143235,#109939,#109940) ;
#93792=AXIS2_PLACEMENT_3D('',#143243,#109944,#109945) ;
#93793=AXIS2_PLACEMENT_3D('',#143247,#109947,#109948) ;
#93794=AXIS2_PLACEMENT_3D('',#143252,#109951,#109952) ;
#93795=AXIS2_PLACEMENT_3D('',#143260,#109956,#109957) ;
#93796=AXIS2_PLACEMENT_3D('',#143264,#109959,#109960) ;
#93797=AXIS2_PLACEMENT_3D('',#143268,#109962,#109963) ;
#93798=AXIS2_PLACEMENT_3D('',#143270,#109964,#109965) ;
#93799=AXIS2_PLACEMENT_3D('',#143272,#109966,#109967) ;
#93800=AXIS2_PLACEMENT_3D('',#143276,#109969,#109970) ;
#93801=AXIS2_PLACEMENT_3D('',#143280,#109972,#109973) ;
#93802=AXIS2_PLACEMENT_3D('',#143288,#109977,#109978) ;
#93803=AXIS2_PLACEMENT_3D('',#143292,#109980,#109981) ;
#93804=AXIS2_PLACEMENT_3D('',#143297,#109984,#109985) ;
#93805=AXIS2_PLACEMENT_3D('',#143305,#109989,#109990) ;
#93806=AXIS2_PLACEMENT_3D('',#143309,#109992,#109993) ;
#93807=AXIS2_PLACEMENT_3D('',#143313,#109995,#109996) ;
#93808=AXIS2_PLACEMENT_3D('',#143315,#109997,#109998) ;
#93809=AXIS2_PLACEMENT_3D('',#143317,#109999,#110000) ;
#93810=AXIS2_PLACEMENT_3D('',#143321,#110002,#110003) ;
#93811=AXIS2_PLACEMENT_3D('',#143325,#110005,#110006) ;
#93812=AXIS2_PLACEMENT_3D('',#143333,#110010,#110011) ;
#93813=AXIS2_PLACEMENT_3D('',#143337,#110013,#110014) ;
#93814=AXIS2_PLACEMENT_3D('',#143342,#110017,#110018) ;
#93815=AXIS2_PLACEMENT_3D('',#143350,#110022,#110023) ;
#93816=AXIS2_PLACEMENT_3D('',#143354,#110025,#110026) ;
#93817=AXIS2_PLACEMENT_3D('',#143358,#110028,#110029) ;
#93818=AXIS2_PLACEMENT_3D('',#143360,#110030,#110031) ;
#93819=AXIS2_PLACEMENT_3D('',#143362,#110032,#110033) ;
#93820=AXIS2_PLACEMENT_3D('',#143366,#110035,#110036) ;
#93821=AXIS2_PLACEMENT_3D('',#143370,#110038,#110039) ;
#93822=AXIS2_PLACEMENT_3D('',#143378,#110043,#110044) ;
#93823=AXIS2_PLACEMENT_3D('',#143382,#110046,#110047) ;
#93824=AXIS2_PLACEMENT_3D('',#143387,#110050,#110051) ;
#93825=AXIS2_PLACEMENT_3D('',#143395,#110055,#110056) ;
#93826=AXIS2_PLACEMENT_3D('',#143399,#110058,#110059) ;
#93827=AXIS2_PLACEMENT_3D('',#143403,#110061,#110062) ;
#93828=AXIS2_PLACEMENT_3D('',#143405,#110063,#110064) ;
#93829=AXIS2_PLACEMENT_3D('',#143407,#110065,#110066) ;
#93830=AXIS2_PLACEMENT_3D('',#143411,#110068,#110069) ;
#93831=AXIS2_PLACEMENT_3D('',#143415,#110071,#110072) ;
#93832=AXIS2_PLACEMENT_3D('',#143423,#110076,#110077) ;
#93833=AXIS2_PLACEMENT_3D('',#143427,#110079,#110080) ;
#93834=AXIS2_PLACEMENT_3D('',#143432,#110083,#110084) ;
#93835=AXIS2_PLACEMENT_3D('',#143440,#110088,#110089) ;
#93836=AXIS2_PLACEMENT_3D('',#143444,#110091,#110092) ;
#93837=AXIS2_PLACEMENT_3D('',#143448,#110094,#110095) ;
#93838=AXIS2_PLACEMENT_3D('',#143450,#110096,#110097) ;
#93839=AXIS2_PLACEMENT_3D('',#143452,#110098,#110099) ;
#93840=AXIS2_PLACEMENT_3D('',#143456,#110101,#110102) ;
#93841=AXIS2_PLACEMENT_3D('',#143460,#110104,#110105) ;
#93842=AXIS2_PLACEMENT_3D('',#143468,#110109,#110110) ;
#93843=AXIS2_PLACEMENT_3D('',#143472,#110112,#110113) ;
#93844=AXIS2_PLACEMENT_3D('',#143477,#110116,#110117) ;
#93845=AXIS2_PLACEMENT_3D('',#143485,#110121,#110122) ;
#93846=AXIS2_PLACEMENT_3D('',#143489,#110124,#110125) ;
#93847=AXIS2_PLACEMENT_3D('',#143493,#110127,#110128) ;
#93848=AXIS2_PLACEMENT_3D('',#143495,#110129,#110130) ;
#93849=AXIS2_PLACEMENT_3D('',#143497,#110131,#110132) ;
#93850=AXIS2_PLACEMENT_3D('',#143501,#110134,#110135) ;
#93851=AXIS2_PLACEMENT_3D('',#143505,#110137,#110138) ;
#93852=AXIS2_PLACEMENT_3D('',#143513,#110142,#110143) ;
#93853=AXIS2_PLACEMENT_3D('',#143517,#110145,#110146) ;
#93854=AXIS2_PLACEMENT_3D('',#143522,#110149,#110150) ;
#93855=AXIS2_PLACEMENT_3D('',#143530,#110154,#110155) ;
#93856=AXIS2_PLACEMENT_3D('',#143534,#110157,#110158) ;
#93857=AXIS2_PLACEMENT_3D('',#143538,#110160,#110161) ;
#93858=AXIS2_PLACEMENT_3D('',#143540,#110162,#110163) ;
#93859=AXIS2_PLACEMENT_3D('',#143542,#110164,#110165) ;
#93860=AXIS2_PLACEMENT_3D('',#143546,#110167,#110168) ;
#93861=AXIS2_PLACEMENT_3D('',#143550,#110170,#110171) ;
#93862=AXIS2_PLACEMENT_3D('',#143558,#110175,#110176) ;
#93863=AXIS2_PLACEMENT_3D('',#143562,#110178,#110179) ;
#93864=AXIS2_PLACEMENT_3D('',#143567,#110182,#110183) ;
#93865=AXIS2_PLACEMENT_3D('',#143575,#110187,#110188) ;
#93866=AXIS2_PLACEMENT_3D('',#143579,#110190,#110191) ;
#93867=AXIS2_PLACEMENT_3D('',#143583,#110193,#110194) ;
#93868=AXIS2_PLACEMENT_3D('',#143585,#110195,#110196) ;
#93869=AXIS2_PLACEMENT_3D('',#143587,#110197,#110198) ;
#93870=AXIS2_PLACEMENT_3D('',#143591,#110200,#110201) ;
#93871=AXIS2_PLACEMENT_3D('',#143595,#110203,#110204) ;
#93872=AXIS2_PLACEMENT_3D('',#143603,#110208,#110209) ;
#93873=AXIS2_PLACEMENT_3D('',#143607,#110211,#110212) ;
#93874=AXIS2_PLACEMENT_3D('',#143612,#110215,#110216) ;
#93875=AXIS2_PLACEMENT_3D('',#143620,#110220,#110221) ;
#93876=AXIS2_PLACEMENT_3D('',#143624,#110223,#110224) ;
#93877=AXIS2_PLACEMENT_3D('',#143628,#110226,#110227) ;
#93878=AXIS2_PLACEMENT_3D('',#143630,#110228,#110229) ;
#93879=AXIS2_PLACEMENT_3D('',#143632,#110230,#110231) ;
#93880=AXIS2_PLACEMENT_3D('',#143636,#110233,#110234) ;
#93881=AXIS2_PLACEMENT_3D('',#143640,#110236,#110237) ;
#93882=AXIS2_PLACEMENT_3D('',#143648,#110241,#110242) ;
#93883=AXIS2_PLACEMENT_3D('',#143652,#110244,#110245) ;
#93884=AXIS2_PLACEMENT_3D('',#143657,#110248,#110249) ;
#93885=AXIS2_PLACEMENT_3D('',#143665,#110253,#110254) ;
#93886=AXIS2_PLACEMENT_3D('',#143669,#110256,#110257) ;
#93887=AXIS2_PLACEMENT_3D('',#143673,#110259,#110260) ;
#93888=AXIS2_PLACEMENT_3D('',#143675,#110261,#110262) ;
#93889=AXIS2_PLACEMENT_3D('',#143677,#110263,#110264) ;
#93890=AXIS2_PLACEMENT_3D('',#143681,#110266,#110267) ;
#93891=AXIS2_PLACEMENT_3D('',#143683,#110269,#110270) ;
#93892=AXIS2_PLACEMENT_3D('',#143694,#110275,#110276) ;
#93893=AXIS2_PLACEMENT_3D('',#143702,#110280,#110281) ;
#93894=AXIS2_PLACEMENT_3D('',#143704,#110283,#110284) ;
#93895=AXIS2_PLACEMENT_3D('',#143715,#110289,#110290) ;
#93896=AXIS2_PLACEMENT_3D('',#143723,#110294,#110295) ;
#93897=AXIS2_PLACEMENT_3D('',#143725,#110297,#110298) ;
#93898=AXIS2_PLACEMENT_3D('',#143740,#110305,#110306) ;
#93899=AXIS2_PLACEMENT_3D('',#143744,#110308,#110309) ;
#93900=AXIS2_PLACEMENT_3D('',#143746,#110311,#110312) ;
#93901=AXIS2_PLACEMENT_3D('',#143755,#110317,#110318) ;
#93902=AXIS2_PLACEMENT_3D('',#143761,#110322,#110323) ;
#93903=AXIS2_PLACEMENT_3D('',#143770,#110328,#110329) ;
#93904=AXIS2_PLACEMENT_3D('',#143779,#110334,#110335) ;
#93905=AXIS2_PLACEMENT_3D('',#143788,#110340,#110341) ;
#93906=AXIS2_PLACEMENT_3D('',#143793,#110343,#110344) ;
#93907=AXIS2_PLACEMENT_3D('',#143796,#110346,#110347) ;
#93908=AXIS2_PLACEMENT_3D('',#143797,#110348,#110349) ;
#93909=AXIS2_PLACEMENT_3D('',#143803,#110353,#110354) ;
#93910=AXIS2_PLACEMENT_3D('',#143805,#110355,#110356) ;
#93911=AXIS2_PLACEMENT_3D('',#143808,#110358,#110359) ;
#93912=AXIS2_PLACEMENT_3D('',#143809,#110360,#110361) ;
#93913=AXIS2_PLACEMENT_3D('',#143815,#110365,#110366) ;
#93914=AXIS2_PLACEMENT_3D('',#143817,#110367,#110368) ;
#93915=AXIS2_PLACEMENT_3D('',#143820,#110370,#110371) ;
#93916=AXIS2_PLACEMENT_3D('',#143821,#110372,#110373) ;
#93917=AXIS2_PLACEMENT_3D('',#143826,#110377,#110378) ;
#93918=AXIS2_PLACEMENT_3D('',#143829,#110380,#110381) ;
#93919=AXIS2_PLACEMENT_3D('',#143830,#110382,#110383) ;
#93920=AXIS2_PLACEMENT_3D('',#143833,#110386,#110387) ;
#93921=AXIS2_PLACEMENT_3D('',#143839,#110391,#110392) ;
#93922=AXIS2_PLACEMENT_3D('',#143841,#110393,#110394) ;
#93923=AXIS2_PLACEMENT_3D('',#143844,#110396,#110397) ;
#93924=AXIS2_PLACEMENT_3D('',#143845,#110398,#110399) ;
#93925=AXIS2_PLACEMENT_3D('',#143851,#110403,#110404) ;
#93926=AXIS2_PLACEMENT_3D('',#143853,#110405,#110406) ;
#93927=AXIS2_PLACEMENT_3D('',#143856,#110408,#110409) ;
#93928=AXIS2_PLACEMENT_3D('',#143857,#110410,#110411) ;
#93929=AXIS2_PLACEMENT_3D('',#143863,#110415,#110416) ;
#93930=AXIS2_PLACEMENT_3D('',#143865,#110417,#110418) ;
#93931=AXIS2_PLACEMENT_3D('',#143868,#110420,#110421) ;
#93932=AXIS2_PLACEMENT_3D('',#143869,#110422,#110423) ;
#93933=AXIS2_PLACEMENT_3D('',#143875,#110427,#110428) ;
#93934=AXIS2_PLACEMENT_3D('',#143877,#110429,#110430) ;
#93935=AXIS2_PLACEMENT_3D('',#143880,#110432,#110433) ;
#93936=AXIS2_PLACEMENT_3D('',#143881,#110434,#110435) ;
#93937=AXIS2_PLACEMENT_3D('',#143887,#110439,#110440) ;
#93938=AXIS2_PLACEMENT_3D('',#143889,#110441,#110442) ;
#93939=AXIS2_PLACEMENT_3D('',#143892,#110444,#110445) ;
#93940=AXIS2_PLACEMENT_3D('',#143893,#110446,#110447) ;
#93941=AXIS2_PLACEMENT_3D('',#143899,#110451,#110452) ;
#93942=AXIS2_PLACEMENT_3D('',#143901,#110453,#110454) ;
#93943=AXIS2_PLACEMENT_3D('',#143904,#110456,#110457) ;
#93944=AXIS2_PLACEMENT_3D('',#143905,#110458,#110459) ;
#93945=AXIS2_PLACEMENT_3D('',#143907,#110460,#110461) ;
#93946=AXIS2_PLACEMENT_3D('',#143910,#110463,#110464) ;
#93947=AXIS2_PLACEMENT_3D('',#143911,#110465,#110466) ;
#93948=AXIS2_PLACEMENT_3D('',#143913,#110467,#110468) ;
#93949=AXIS2_PLACEMENT_3D('',#143916,#110470,#110471) ;
#93950=AXIS2_PLACEMENT_3D('',#143917,#110472,#110473) ;
#93951=AXIS2_PLACEMENT_3D('',#143923,#110477,#110478) ;
#93952=AXIS2_PLACEMENT_3D('',#143925,#110479,#110480) ;
#93953=AXIS2_PLACEMENT_3D('',#143928,#110482,#110483) ;
#93954=AXIS2_PLACEMENT_3D('',#143929,#110484,#110485) ;
#93955=AXIS2_PLACEMENT_3D('',#143935,#110489,#110490) ;
#93956=AXIS2_PLACEMENT_3D('',#143937,#110491,#110492) ;
#93957=AXIS2_PLACEMENT_3D('',#143940,#110494,#110495) ;
#93958=AXIS2_PLACEMENT_3D('',#143941,#110496,#110497) ;
#93959=AXIS2_PLACEMENT_3D('',#143944,#110500,#110501) ;
#93960=AXIS2_PLACEMENT_3D('',#143947,#110502,#110503) ;
#93961=AXIS2_PLACEMENT_3D('',#143951,#110505,#110506) ;
#93962=AXIS2_PLACEMENT_3D('',#143959,#110510,#110511) ;
#93963=AXIS2_PLACEMENT_3D('',#143967,#110515,#110516) ;
#93964=AXIS2_PLACEMENT_3D('',#143971,#110518,#110519) ;
#93965=AXIS2_PLACEMENT_3D('',#143980,#110525,#110526) ;
#93966=AXIS2_PLACEMENT_3D('',#143985,#110528,#110529) ;
#93967=AXIS2_PLACEMENT_3D('',#143989,#110531,#110532) ;
#93968=AXIS2_PLACEMENT_3D('',#143993,#110534,#110535) ;
#93969=AXIS2_PLACEMENT_3D('',#143996,#110537,#110538) ;
#93970=AXIS2_PLACEMENT_3D('',#143997,#110539,#110540) ;
#93971=AXIS2_PLACEMENT_3D('',#143998,#110541,#110542) ;
#93972=AXIS2_PLACEMENT_3D('',#143999,#110543,#110544) ;
#93973=AXIS2_PLACEMENT_3D('',#144000,#110545,#110546) ;
#93974=AXIS2_PLACEMENT_3D('',#144001,#110547,#110548) ;
#93975=AXIS2_PLACEMENT_3D('',#144002,#110549,#110550) ;
#93976=AXIS2_PLACEMENT_3D('',#144003,#110551,#110552) ;
#93977=AXIS2_PLACEMENT_3D('',#144005,#110553,#110554) ;
#93978=AXIS2_PLACEMENT_3D('',#144006,#110555,#110556) ;
#93979=AXIS2_PLACEMENT_3D('',#144007,#110557,#110558) ;
#93980=AXIS2_PLACEMENT_3D('',#144008,#110559,#110560) ;
#93981=AXIS2_PLACEMENT_3D('',#144009,#110561,#110562) ;
#93982=AXIS2_PLACEMENT_3D('',#144010,#110563,#110564) ;
#93983=AXIS2_PLACEMENT_3D('',#144011,#110565,#110566) ;
#93984=AXIS2_PLACEMENT_3D('',#144012,#110567,#110568) ;
#93985=AXIS2_PLACEMENT_3D('',#144013,#110569,#110570) ;
#93986=AXIS2_PLACEMENT_3D('',#144024,#110572,#110573) ;
#93987=AXIS2_PLACEMENT_3D('',#144081,#110575,#110576) ;
#93988=AXIS2_PLACEMENT_3D('',#144082,#110577,#110578) ;
#93989=AXIS2_PLACEMENT_3D('',#144083,#110579,#110580) ;
#93990=AXIS2_PLACEMENT_3D('',#144084,#110581,#110582) ;
#93991=AXIS2_PLACEMENT_3D('',#144085,#110583,#110584) ;
#93992=AXIS2_PLACEMENT_3D('',#144086,#110585,#110586) ;
#93993=AXIS2_PLACEMENT_3D('',#144087,#110587,#110588) ;
#93994=AXIS2_PLACEMENT_3D('',#144088,#110589,#110590) ;
#93995=AXIS2_PLACEMENT_3D('',#144089,#110591,#110592) ;
#93996=AXIS2_PLACEMENT_3D('',#144090,#110593,#110594) ;
#93997=AXIS2_PLACEMENT_3D('',#144091,#110595,#110596) ;
#93998=AXIS2_PLACEMENT_3D('',#144092,#110597,#110598) ;
#93999=AXIS2_PLACEMENT_3D('',#144093,#110599,#110600) ;
#94000=AXIS2_PLACEMENT_3D('',#144094,#110601,#110602) ;
#94001=AXIS2_PLACEMENT_3D('',#144095,#110603,#110604) ;
#94002=AXIS2_PLACEMENT_3D('',#144096,#110605,#110606) ;
#94003=AXIS2_PLACEMENT_3D('',#144097,#110607,#110608) ;
#94004=AXIS2_PLACEMENT_3D('',#144098,#110609,#110610) ;
#94005=AXIS2_PLACEMENT_3D('',#144099,#110611,#110612) ;
#94006=AXIS2_PLACEMENT_3D('',#144100,#110613,#110614) ;
#94007=AXIS2_PLACEMENT_3D('',#144101,#110615,#110616) ;
#94008=AXIS2_PLACEMENT_3D('',#144102,#110617,#110618) ;
#94009=AXIS2_PLACEMENT_3D('',#144103,#110619,#110620) ;
#94010=AXIS2_PLACEMENT_3D('',#144106,#110622,#110623) ;
#94011=AXIS2_PLACEMENT_3D('',#144107,#110624,#110625) ;
#94012=AXIS2_PLACEMENT_3D('',#144108,#110626,#110627) ;
#94013=AXIS2_PLACEMENT_3D('',#144109,#110628,#110629) ;
#94014=AXIS2_PLACEMENT_3D('',#144110,#110630,#110631) ;
#94015=AXIS2_PLACEMENT_3D('',#144111,#110632,#110633) ;
#94016=AXIS2_PLACEMENT_3D('',#144112,#110634,#110635) ;
#94017=AXIS2_PLACEMENT_3D('',#144113,#110636,#110637) ;
#94018=AXIS2_PLACEMENT_3D('',#144114,#110638,#110639) ;
#94019=AXIS2_PLACEMENT_3D('',#144115,#110640,#110641) ;
#94020=AXIS2_PLACEMENT_3D('',#144116,#110642,#110643) ;
#94021=AXIS2_PLACEMENT_3D('',#144117,#110644,#110645) ;
#94022=AXIS2_PLACEMENT_3D('',#144118,#110646,#110647) ;
#94023=AXIS2_PLACEMENT_3D('',#144119,#110648,#110649) ;
#94024=AXIS2_PLACEMENT_3D('',#144120,#110650,#110651) ;
#94025=AXIS2_PLACEMENT_3D('',#144121,#110652,#110653) ;
#94026=AXIS2_PLACEMENT_3D('',#144123,#110654,#110655) ;
#94027=AXIS2_PLACEMENT_3D('',#144124,#110656,#110657) ;
#94028=AXIS2_PLACEMENT_3D('',#144125,#110658,#110659) ;
#94029=AXIS2_PLACEMENT_3D('',#144126,#110660,#110661) ;
#94030=AXIS2_PLACEMENT_3D('',#144127,#110662,#110663) ;
#94031=AXIS2_PLACEMENT_3D('',#144128,#110664,#110665) ;
#94032=AXIS2_PLACEMENT_3D('',#144129,#110666,#110667) ;
#94033=AXIS2_PLACEMENT_3D('',#144130,#110668,#110669) ;
#94034=AXIS2_PLACEMENT_3D('',#144131,#110670,#110671) ;
#94035=AXIS2_PLACEMENT_3D('',#144132,#110672,#110673) ;
#94036=AXIS2_PLACEMENT_3D('',#144133,#110674,#110675) ;
#94037=AXIS2_PLACEMENT_3D('',#144134,#110676,#110677) ;
#94038=AXIS2_PLACEMENT_3D('',#144135,#110678,#110679) ;
#94039=AXIS2_PLACEMENT_3D('',#144138,#110681,#110682) ;
#94040=AXIS2_PLACEMENT_3D('',#144139,#110683,#110684) ;
#94041=AXIS2_PLACEMENT_3D('',#144140,#110685,#110686) ;
#94042=AXIS2_PLACEMENT_3D('',#144141,#110687,#110688) ;
#94043=AXIS2_PLACEMENT_3D('',#144142,#110689,#110690) ;
#94044=AXIS2_PLACEMENT_3D('',#144143,#110691,#110692) ;
#94045=AXIS2_PLACEMENT_3D('',#144144,#110693,#110694) ;
#94046=AXIS2_PLACEMENT_3D('',#144145,#110695,#110696) ;
#94047=AXIS2_PLACEMENT_3D('',#144146,#110697,#110698) ;
#94048=AXIS2_PLACEMENT_3D('',#144147,#110699,#110700) ;
#94049=AXIS2_PLACEMENT_3D('',#144148,#110701,#110702) ;
#94050=AXIS2_PLACEMENT_3D('',#144149,#110703,#110704) ;
#94051=AXIS2_PLACEMENT_3D('',#144150,#110705,#110706) ;
#94052=AXIS2_PLACEMENT_3D('',#144152,#110707,#110708) ;
#94053=AXIS2_PLACEMENT_3D('',#144153,#110709,#110710) ;
#94054=AXIS2_PLACEMENT_3D('',#144154,#110711,#110712) ;
#94055=AXIS2_PLACEMENT_3D('',#144155,#110713,#110714) ;
#94056=AXIS2_PLACEMENT_3D('',#144156,#110715,#110716) ;
#94057=AXIS2_PLACEMENT_3D('',#144157,#110717,#110718) ;
#94058=AXIS2_PLACEMENT_3D('',#144158,#110719,#110720) ;
#94059=AXIS2_PLACEMENT_3D('',#144159,#110721,#110722) ;
#94060=AXIS2_PLACEMENT_3D('',#144160,#110723,#110724) ;
#94061=AXIS2_PLACEMENT_3D('',#144161,#110725,#110726) ;
#94062=AXIS2_PLACEMENT_3D('',#144162,#110727,#110728) ;
#94063=AXIS2_PLACEMENT_3D('',#144164,#110730,#110731) ;
#94064=AXIS2_PLACEMENT_3D('',#144165,#110732,#110733) ;
#94065=AXIS2_PLACEMENT_3D('',#144166,#110734,#110735) ;
#94066=AXIS2_PLACEMENT_3D('',#144167,#110736,#110737) ;
#94067=AXIS2_PLACEMENT_3D('',#144168,#110738,#110739) ;
#94068=AXIS2_PLACEMENT_3D('',#144169,#110740,#110741) ;
#94069=AXIS2_PLACEMENT_3D('',#144170,#110742,#110743) ;
#94070=AXIS2_PLACEMENT_3D('',#144171,#110744,#110745) ;
#94071=AXIS2_PLACEMENT_3D('',#144172,#110746,#110747) ;
#94072=AXIS2_PLACEMENT_3D('',#144173,#110748,#110749) ;
#94073=AXIS2_PLACEMENT_3D('',#144174,#110750,#110751) ;
#94074=AXIS2_PLACEMENT_3D('',#144175,#110752,#110753) ;
#94075=AXIS2_PLACEMENT_3D('',#144176,#110754,#110755) ;
#94076=AXIS2_PLACEMENT_3D('',#144177,#110756,#110757) ;
#94077=AXIS2_PLACEMENT_3D('',#144178,#110758,#110759) ;
#94078=AXIS2_PLACEMENT_3D('',#144179,#110760,#110761) ;
#94079=AXIS2_PLACEMENT_3D('',#144180,#110762,#110763) ;
#94080=AXIS2_PLACEMENT_3D('',#144181,#110764,#110765) ;
#94081=AXIS2_PLACEMENT_3D('',#144182,#110766,#110767) ;
#94082=AXIS2_PLACEMENT_3D('',#144183,#110768,#110769) ;
#94083=AXIS2_PLACEMENT_3D('',#144184,#110770,#110771) ;
#94084=AXIS2_PLACEMENT_3D('',#144185,#110772,#110773) ;
#94085=AXIS2_PLACEMENT_3D('',#144186,#110774,#110775) ;
#94086=AXIS2_PLACEMENT_3D('',#144187,#110776,#110777) ;
#94087=AXIS2_PLACEMENT_3D('',#144188,#110778,#110779) ;
#94088=AXIS2_PLACEMENT_3D('',#144189,#110780,#110781) ;
#94089=AXIS2_PLACEMENT_3D('',#144190,#110782,#110783) ;
#94090=AXIS2_PLACEMENT_3D('',#144191,#110784,#110785) ;
#94091=AXIS2_PLACEMENT_3D('',#144192,#110786,#110787) ;
#94092=AXIS2_PLACEMENT_3D('',#144193,#110788,#110789) ;
#94093=AXIS2_PLACEMENT_3D('',#144194,#110790,#110791) ;
#94094=AXIS2_PLACEMENT_3D('',#144195,#110792,#110793) ;
#94095=AXIS2_PLACEMENT_3D('',#144196,#110794,#110795) ;
#94096=AXIS2_PLACEMENT_3D('',#144197,#110796,#110797) ;
#94097=AXIS2_PLACEMENT_3D('',#144198,#110798,#110799) ;
#94098=AXIS2_PLACEMENT_3D('',#144199,#110800,#110801) ;
#94099=AXIS2_PLACEMENT_3D('',#144200,#110802,#110803) ;
#94100=AXIS2_PLACEMENT_3D('',#144201,#110804,#110805) ;
#94101=AXIS2_PLACEMENT_3D('',#144202,#110806,#110807) ;
#94102=AXIS2_PLACEMENT_3D('',#144203,#110808,#110809) ;
#94103=AXIS2_PLACEMENT_3D('',#144204,#110810,#110811) ;
#94104=AXIS2_PLACEMENT_3D('',#144205,#110812,#110813) ;
#94105=AXIS2_PLACEMENT_3D('',#144206,#110814,#110815) ;
#94106=AXIS2_PLACEMENT_3D('',#144207,#110816,#110817) ;
#94107=AXIS2_PLACEMENT_3D('',#144208,#110818,#110819) ;
#94108=AXIS2_PLACEMENT_3D('',#144209,#110820,#110821) ;
#94109=AXIS2_PLACEMENT_3D('',#144210,#110822,#110823) ;
#94110=AXIS2_PLACEMENT_3D('',#144211,#110824,#110825) ;
#94111=AXIS2_PLACEMENT_3D('',#144212,#110826,#110827) ;
#94112=AXIS2_PLACEMENT_3D('',#144213,#110828,#110829) ;
#94113=AXIS2_PLACEMENT_3D('',#144214,#110830,#110831) ;
#94114=AXIS2_PLACEMENT_3D('',#144215,#110832,#110833) ;
#94115=AXIS2_PLACEMENT_3D('',#144216,#110834,#110835) ;
#94116=AXIS2_PLACEMENT_3D('',#144217,#110836,#110837) ;
#94117=AXIS2_PLACEMENT_3D('',#144218,#110838,#110839) ;
#94118=AXIS2_PLACEMENT_3D('',#144219,#110840,#110841) ;
#94119=AXIS2_PLACEMENT_3D('',#144220,#110842,#110843) ;
#94120=AXIS2_PLACEMENT_3D('',#144221,#110844,#110845) ;
#94121=AXIS2_PLACEMENT_3D('',#144222,#110846,#110847) ;
#94122=AXIS2_PLACEMENT_3D('',#144223,#110848,#110849) ;
#94123=AXIS2_PLACEMENT_3D('',#144224,#110850,#110851) ;
#94124=AXIS2_PLACEMENT_3D('',#144225,#110852,#110853) ;
#94125=AXIS2_PLACEMENT_3D('',#144226,#110854,#110855) ;
#94126=AXIS2_PLACEMENT_3D('',#144227,#110856,#110857) ;
#94127=AXIS2_PLACEMENT_3D('',#144228,#110858,#110859) ;
#94128=AXIS2_PLACEMENT_3D('',#144229,#110860,#110861) ;
#94129=AXIS2_PLACEMENT_3D('',#144230,#110862,#110863) ;
#94130=AXIS2_PLACEMENT_3D('',#144231,#110864,#110865) ;
#94131=AXIS2_PLACEMENT_3D('',#144232,#110866,#110867) ;
#94132=AXIS2_PLACEMENT_3D('',#144233,#110868,#110869) ;
#94133=AXIS2_PLACEMENT_3D('',#144234,#110870,#110871) ;
#94134=AXIS2_PLACEMENT_3D('',#144235,#110872,#110873) ;
#94135=AXIS2_PLACEMENT_3D('',#144236,#110874,#110875) ;
#94136=AXIS2_PLACEMENT_3D('',#144237,#110876,#110877) ;
#94137=AXIS2_PLACEMENT_3D('',#144238,#110878,#110879) ;
#94138=AXIS2_PLACEMENT_3D('',#144239,#110880,#110881) ;
#94139=AXIS2_PLACEMENT_3D('',#144240,#110882,#110883) ;
#94140=AXIS2_PLACEMENT_3D('',#144241,#110884,#110885) ;
#94141=AXIS2_PLACEMENT_3D('',#144242,#110886,#110887) ;
#94142=AXIS2_PLACEMENT_3D('',#144243,#110888,#110889) ;
#94143=AXIS2_PLACEMENT_3D('',#144244,#110890,#110891) ;
#94144=AXIS2_PLACEMENT_3D('',#144245,#110892,#110893) ;
#94145=AXIS2_PLACEMENT_3D('',#144246,#110894,#110895) ;
#94146=AXIS2_PLACEMENT_3D('',#144247,#110896,#110897) ;
#94147=AXIS2_PLACEMENT_3D('',#144248,#110898,#110899) ;
#94148=AXIS2_PLACEMENT_3D('',#144249,#110900,#110901) ;
#94149=AXIS2_PLACEMENT_3D('',#144250,#110902,#110903) ;
#94150=AXIS2_PLACEMENT_3D('',#144251,#110904,#110905) ;
#94151=AXIS2_PLACEMENT_3D('',#144252,#110906,#110907) ;
#94152=AXIS2_PLACEMENT_3D('',#144253,#110908,#110909) ;
#94153=AXIS2_PLACEMENT_3D('',#144254,#110910,#110911) ;
#94154=AXIS2_PLACEMENT_3D('',#144255,#110912,#110913) ;
#94155=AXIS2_PLACEMENT_3D('',#144256,#110914,#110915) ;
#94156=AXIS2_PLACEMENT_3D('',#144257,#110916,#110917) ;
#94157=AXIS2_PLACEMENT_3D('',#144258,#110918,#110919) ;
#94158=AXIS2_PLACEMENT_3D('',#144259,#110920,#110921) ;
#94159=AXIS2_PLACEMENT_3D('',#144260,#110922,#110923) ;
#94160=AXIS2_PLACEMENT_3D('',#144261,#110924,#110925) ;
#94161=AXIS2_PLACEMENT_3D('',#144262,#110926,#110927) ;
#94162=AXIS2_PLACEMENT_3D('',#144263,#110928,#110929) ;
#94163=AXIS2_PLACEMENT_3D('',#144264,#110930,#110931) ;
#94164=AXIS2_PLACEMENT_3D('',#144265,#110932,#110933) ;
#94165=AXIS2_PLACEMENT_3D('',#144266,#110934,#110935) ;
#94166=AXIS2_PLACEMENT_3D('',#144267,#110936,#110937) ;
#94167=AXIS2_PLACEMENT_3D('',#144268,#110938,#110939) ;
#94168=AXIS2_PLACEMENT_3D('',#144269,#110940,#110941) ;
#94169=AXIS2_PLACEMENT_3D('',#144270,#110942,#110943) ;
#94170=AXIS2_PLACEMENT_3D('',#144271,#110944,#110945) ;
#94171=AXIS2_PLACEMENT_3D('',#144272,#110946,#110947) ;
#94172=AXIS2_PLACEMENT_3D('',#144273,#110948,#110949) ;
#94173=AXIS2_PLACEMENT_3D('',#144274,#110950,#110951) ;
#94174=AXIS2_PLACEMENT_3D('',#144275,#110952,#110953) ;
#94175=AXIS2_PLACEMENT_3D('',#144276,#110954,#110955) ;
#94176=AXIS2_PLACEMENT_3D('',#144277,#110956,#110957) ;
#94177=AXIS2_PLACEMENT_3D('',#144278,#110958,#110959) ;
#94178=AXIS2_PLACEMENT_3D('',#144279,#110960,#110961) ;
#94179=AXIS2_PLACEMENT_3D('',#144280,#110962,#110963) ;
#94180=AXIS2_PLACEMENT_3D('',#144281,#110964,#110965) ;
#94181=AXIS2_PLACEMENT_3D('',#144282,#110966,#110967) ;
#94182=AXIS2_PLACEMENT_3D('',#144283,#110968,#110969) ;
#94183=AXIS2_PLACEMENT_3D('',#144284,#110970,#110971) ;
#94184=AXIS2_PLACEMENT_3D('',#144285,#110972,#110973) ;
#94185=AXIS2_PLACEMENT_3D('',#144286,#110974,#110975) ;
#94186=AXIS2_PLACEMENT_3D('',#144287,#110976,#110977) ;
#94187=AXIS2_PLACEMENT_3D('',#144288,#110978,#110979) ;
#94188=AXIS2_PLACEMENT_3D('',#144289,#110980,#110981) ;
#94189=AXIS2_PLACEMENT_3D('',#144290,#110982,#110983) ;
#94190=AXIS2_PLACEMENT_3D('',#144291,#110984,#110985) ;
#94191=AXIS2_PLACEMENT_3D('',#144292,#110986,#110987) ;
#94192=AXIS2_PLACEMENT_3D('',#144293,#110988,#110989) ;
#94193=AXIS2_PLACEMENT_3D('',#144294,#110990,#110991) ;
#94194=AXIS2_PLACEMENT_3D('',#144295,#110992,#110993) ;
#94195=AXIS2_PLACEMENT_3D('',#144296,#110994,#110995) ;
#94196=AXIS2_PLACEMENT_3D('',#144297,#110996,#110997) ;
#94197=AXIS2_PLACEMENT_3D('',#144298,#110998,#110999) ;
#94198=AXIS2_PLACEMENT_3D('',#144299,#111000,#111001) ;
#94199=AXIS2_PLACEMENT_3D('',#144300,#111002,#111003) ;
#94200=AXIS2_PLACEMENT_3D('',#144301,#111004,#111005) ;
#94201=AXIS2_PLACEMENT_3D('',#144302,#111006,#111007) ;
#94202=AXIS2_PLACEMENT_3D('',#144303,#111008,#111009) ;
#94203=AXIS2_PLACEMENT_3D('',#144304,#111010,#111011) ;
#94204=AXIS2_PLACEMENT_3D('',#144305,#111012,#111013) ;
#94205=AXIS2_PLACEMENT_3D('',#144306,#111014,#111015) ;
#94206=AXIS2_PLACEMENT_3D('',#144307,#111016,#111017) ;
#94207=AXIS2_PLACEMENT_3D('',#144308,#111018,#111019) ;
#94208=AXIS2_PLACEMENT_3D('',#144309,#111020,#111021) ;
#94209=AXIS2_PLACEMENT_3D('',#144310,#111022,#111023) ;
#94210=AXIS2_PLACEMENT_3D('',#144311,#111024,#111025) ;
#94211=AXIS2_PLACEMENT_3D('',#144312,#111026,#111027) ;
#94212=AXIS2_PLACEMENT_3D('',#144313,#111028,#111029) ;
#94213=AXIS2_PLACEMENT_3D('',#144314,#111030,#111031) ;
#94214=AXIS2_PLACEMENT_3D('',#144315,#111032,#111033) ;
#94215=AXIS2_PLACEMENT_3D('',#144316,#111034,#111035) ;
#94216=AXIS2_PLACEMENT_3D('',#144317,#111036,#111037) ;
#94217=AXIS2_PLACEMENT_3D('',#144318,#111038,#111039) ;
#94218=AXIS2_PLACEMENT_3D('',#144319,#111040,#111041) ;
#94219=AXIS2_PLACEMENT_3D('',#144320,#111042,#111043) ;
#94220=AXIS2_PLACEMENT_3D('',#144321,#111044,#111045) ;
#94221=AXIS2_PLACEMENT_3D('',#144322,#111046,#111047) ;
#94222=AXIS2_PLACEMENT_3D('',#144323,#111048,#111049) ;
#94223=AXIS2_PLACEMENT_3D('',#144324,#111050,#111051) ;
#94224=AXIS2_PLACEMENT_3D('',#144325,#111052,#111053) ;
#94225=AXIS2_PLACEMENT_3D('',#144326,#111054,#111055) ;
#94226=AXIS2_PLACEMENT_3D('',#144327,#111056,#111057) ;
#94227=AXIS2_PLACEMENT_3D('',#144328,#111058,#111059) ;
#94228=AXIS2_PLACEMENT_3D('',#144329,#111060,#111061) ;
#94229=AXIS2_PLACEMENT_3D('',#144330,#111062,#111063) ;
#94230=AXIS2_PLACEMENT_3D('',#144331,#111064,#111065) ;
#94231=AXIS2_PLACEMENT_3D('',#144332,#111066,#111067) ;
#94232=AXIS2_PLACEMENT_3D('',#144333,#111068,#111069) ;
#94233=AXIS2_PLACEMENT_3D('',#144334,#111070,#111071) ;
#94234=AXIS2_PLACEMENT_3D('',#144335,#111072,#111073) ;
#94235=AXIS2_PLACEMENT_3D('',#144336,#111074,#111075) ;
#94236=AXIS2_PLACEMENT_3D('',#144337,#111076,#111077) ;
#94237=AXIS2_PLACEMENT_3D('',#144338,#111078,#111079) ;
#94238=AXIS2_PLACEMENT_3D('',#144339,#111080,#111081) ;
#94239=AXIS2_PLACEMENT_3D('',#144340,#111082,#111083) ;
#94240=AXIS2_PLACEMENT_3D('',#144341,#111084,#111085) ;
#94241=AXIS2_PLACEMENT_3D('',#144350,#111090,#111091) ;
#94242=AXIS2_PLACEMENT_3D('',#144359,#111096,#111097) ;
#94243=AXIS2_PLACEMENT_3D('',#144368,#111102,#111103) ;
#94244=AXIS2_PLACEMENT_3D('',#144377,#111108,#111109) ;
#94245=AXIS2_PLACEMENT_3D('',#144386,#111114,#111115) ;
#94246=AXIS2_PLACEMENT_3D('',#144390,#111117,#111118) ;
#94247=AXIS2_PLACEMENT_3D('',#144392,#111119,#111120) ;
#94248=AXIS2_PLACEMENT_3D('',#144396,#111123,#111124) ;
#94249=AXIS2_PLACEMENT_3D('',#144400,#111126,#111127) ;
#94250=AXIS2_PLACEMENT_3D('',#144402,#111128,#111129) ;
#94251=AXIS2_PLACEMENT_3D('',#144406,#111132,#111133) ;
#94252=AXIS2_PLACEMENT_3D('',#144407,#111134,#111135) ;
#94253=AXIS2_PLACEMENT_3D('',#144408,#111136,#111137) ;
#94254=AXIS2_PLACEMENT_3D('',#144409,#111138,#111139) ;
#94255=AXIS2_PLACEMENT_3D('',#144410,#111140,#111141) ;
#94256=AXIS2_PLACEMENT_3D('',#144411,#111142,#111143) ;
#94257=AXIS2_PLACEMENT_3D('',#144412,#111144,#111145) ;
#94258=AXIS2_PLACEMENT_3D('',#144421,#111150,#111151) ;
#94259=AXIS2_PLACEMENT_3D('',#144427,#111155,#111156) ;
#94260=AXIS2_PLACEMENT_3D('',#144433,#111160,#111161) ;
#94261=AXIS2_PLACEMENT_3D('',#144442,#111166,#111167) ;
#94262=AXIS2_PLACEMENT_3D('',#144451,#111172,#111173) ;
#94263=AXIS2_PLACEMENT_3D('',#144457,#111177,#111178) ;
#94264=AXIS2_PLACEMENT_3D('',#144463,#111182,#111183) ;
#94265=AXIS2_PLACEMENT_3D('',#144472,#111188,#111189) ;
#94266=AXIS2_PLACEMENT_3D('',#144481,#111194,#111195) ;
#94267=AXIS2_PLACEMENT_3D('',#144490,#111200,#111201) ;
#94268=AXIS2_PLACEMENT_3D('',#144499,#111206,#111207) ;
#94269=AXIS2_PLACEMENT_3D('',#144500,#111208,#111209) ;
#94270=AXIS2_PLACEMENT_3D('',#144501,#111210,#111211) ;
#94271=AXIS2_PLACEMENT_3D('',#144502,#111212,#111213) ;
#94272=AXIS2_PLACEMENT_3D('',#144503,#111214,#111215) ;
#94273=AXIS2_PLACEMENT_3D('',#144504,#111216,#111217) ;
#94274=AXIS2_PLACEMENT_3D('',#144505,#111218,#111219) ;
#94275=AXIS2_PLACEMENT_3D('',#144506,#111220,#111221) ;
#94276=AXIS2_PLACEMENT_3D('',#144507,#111222,#111223) ;
#94277=AXIS2_PLACEMENT_3D('',#144508,#111224,#111225) ;
#94278=AXIS2_PLACEMENT_3D('',#144509,#111226,#111227) ;
#94279=AXIS2_PLACEMENT_3D('',#144510,#111228,#111229) ;
#94280=AXIS2_PLACEMENT_3D('',#144511,#111230,#111231) ;
#94281=AXIS2_PLACEMENT_3D('',#144512,#111232,#111233) ;
#94282=AXIS2_PLACEMENT_3D('',#144513,#111234,#111235) ;
#94283=AXIS2_PLACEMENT_3D('',#144514,#111236,#111237) ;
#94284=AXIS2_PLACEMENT_3D('',#144515,#111238,#111239) ;
#94285=AXIS2_PLACEMENT_3D('',#144516,#111240,#111241) ;
#94286=AXIS2_PLACEMENT_3D('',#144517,#111242,#111243) ;
#94287=AXIS2_PLACEMENT_3D('',#144518,#111244,#111245) ;
#94288=AXIS2_PLACEMENT_3D('',#144519,#111246,#111247) ;
#94289=AXIS2_PLACEMENT_3D('',#144520,#111248,#111249) ;
#94290=AXIS2_PLACEMENT_3D('',#144521,#111250,#111251) ;
#94291=AXIS2_PLACEMENT_3D('',#144522,#111252,#111253) ;
#94292=AXIS2_PLACEMENT_3D('',#144523,#111254,#111255) ;
#94293=AXIS2_PLACEMENT_3D('',#144524,#111256,#111257) ;
#94294=AXIS2_PLACEMENT_3D('',#144525,#111258,#111259) ;
#94295=AXIS2_PLACEMENT_3D('',#144526,#111260,#111261) ;
#94296=AXIS2_PLACEMENT_3D('',#144527,#111262,#111263) ;
#94297=AXIS2_PLACEMENT_3D('',#144528,#111264,#111265) ;
#94298=AXIS2_PLACEMENT_3D('',#144529,#111266,#111267) ;
#94299=AXIS2_PLACEMENT_3D('',#144530,#111268,#111269) ;
#94300=AXIS2_PLACEMENT_3D('',#144531,#111270,#111271) ;
#94301=AXIS2_PLACEMENT_3D('',#144532,#111272,#111273) ;
#94302=AXIS2_PLACEMENT_3D('',#144533,#111274,#111275) ;
#94303=AXIS2_PLACEMENT_3D('',#144534,#111276,#111277) ;
#94304=AXIS2_PLACEMENT_3D('',#144535,#111278,#111279) ;
#94305=AXIS2_PLACEMENT_3D('',#144536,#111280,#111281) ;
#94306=AXIS2_PLACEMENT_3D('',#144537,#111282,#111283) ;
#94307=AXIS2_PLACEMENT_3D('',#144538,#111284,#111285) ;
#94308=AXIS2_PLACEMENT_3D('',#144539,#111286,#111287) ;
#94309=AXIS2_PLACEMENT_3D('',#144540,#111288,#111289) ;
#94310=AXIS2_PLACEMENT_3D('',#144541,#111290,#111291) ;
#94311=AXIS2_PLACEMENT_3D('',#144542,#111292,#111293) ;
#94312=AXIS2_PLACEMENT_3D('',#144543,#111294,#111295) ;
#94313=AXIS2_PLACEMENT_3D('',#144544,#111296,#111297) ;
#94314=AXIS2_PLACEMENT_3D('',#144545,#111298,#111299) ;
#94315=AXIS2_PLACEMENT_3D('',#144546,#111300,#111301) ;
#94316=AXIS2_PLACEMENT_3D('',#144547,#111302,#111303) ;
#94317=AXIS2_PLACEMENT_3D('',#144548,#111304,#111305) ;
#94318=AXIS2_PLACEMENT_3D('',#144549,#111306,#111307) ;
#94319=AXIS2_PLACEMENT_3D('',#144550,#111308,#111309) ;
#94320=AXIS2_PLACEMENT_3D('',#144551,#111310,#111311) ;
#94321=AXIS2_PLACEMENT_3D('',#144552,#111312,#111313) ;
#94322=AXIS2_PLACEMENT_3D('',#144553,#111314,#111315) ;
#94323=AXIS2_PLACEMENT_3D('',#144554,#111316,#111317) ;
#94324=AXIS2_PLACEMENT_3D('',#144555,#111318,#111319) ;
#94325=AXIS2_PLACEMENT_3D('',#144556,#111320,#111321) ;
#94326=AXIS2_PLACEMENT_3D('',#144557,#111322,#111323) ;
#94327=AXIS2_PLACEMENT_3D('',#144558,#111324,#111325) ;
#94328=AXIS2_PLACEMENT_3D('',#144559,#111326,#111327) ;
#94329=AXIS2_PLACEMENT_3D('',#144560,#111328,#111329) ;
#94330=AXIS2_PLACEMENT_3D('',#144561,#111330,#111331) ;
#94331=AXIS2_PLACEMENT_3D('',#144562,#111332,#111333) ;
#94332=AXIS2_PLACEMENT_3D('',#144563,#111334,#111335) ;
#94333=AXIS2_PLACEMENT_3D('',#144564,#111336,#111337) ;
#94334=AXIS2_PLACEMENT_3D('',#144565,#111338,#111339) ;
#94335=AXIS2_PLACEMENT_3D('',#144566,#111340,#111341) ;
#94336=AXIS2_PLACEMENT_3D('',#144567,#111342,#111343) ;
#94337=AXIS2_PLACEMENT_3D('',#144568,#111344,#111345) ;
#94338=AXIS2_PLACEMENT_3D('',#144569,#111346,#111347) ;
#94339=AXIS2_PLACEMENT_3D('',#144570,#111348,#111349) ;
#94340=AXIS2_PLACEMENT_3D('',#144571,#111350,#111351) ;
#94341=AXIS2_PLACEMENT_3D('',#144572,#111352,#111353) ;
#94342=AXIS2_PLACEMENT_3D('',#144573,#111354,#111355) ;
#94343=AXIS2_PLACEMENT_3D('',#144574,#111356,#111357) ;
#94344=AXIS2_PLACEMENT_3D('',#144575,#111358,#111359) ;
#94345=AXIS2_PLACEMENT_3D('',#144576,#111360,#111361) ;
#94346=AXIS2_PLACEMENT_3D('',#144577,#111362,#111363) ;
#94347=AXIS2_PLACEMENT_3D('',#144578,#111364,#111365) ;
#94348=AXIS2_PLACEMENT_3D('',#144579,#111366,#111367) ;
#94349=AXIS2_PLACEMENT_3D('',#144580,#111368,#111369) ;
#94350=AXIS2_PLACEMENT_3D('',#144581,#111370,#111371) ;
#94351=AXIS2_PLACEMENT_3D('',#144582,#111372,#111373) ;
#94352=AXIS2_PLACEMENT_3D('',#144583,#111374,#111375) ;
#94353=AXIS2_PLACEMENT_3D('',#144584,#111376,#111377) ;
#94354=AXIS2_PLACEMENT_3D('',#144585,#111378,#111379) ;
#94355=AXIS2_PLACEMENT_3D('',#144586,#111380,#111381) ;
#94356=AXIS2_PLACEMENT_3D('',#144587,#111382,#111383) ;
#94357=AXIS2_PLACEMENT_3D('',#144588,#111384,#111385) ;
#94358=AXIS2_PLACEMENT_3D('',#144589,#111386,#111387) ;
#94359=AXIS2_PLACEMENT_3D('',#144590,#111388,#111389) ;
#94360=AXIS2_PLACEMENT_3D('',#144591,#111390,#111391) ;
#94361=AXIS2_PLACEMENT_3D('',#144592,#111392,#111393) ;
#94362=AXIS2_PLACEMENT_3D('',#144593,#111394,#111395) ;
#94363=AXIS2_PLACEMENT_3D('',#144594,#111396,#111397) ;
#94364=AXIS2_PLACEMENT_3D('',#144595,#111398,#111399) ;
#94365=AXIS2_PLACEMENT_3D('',#144596,#111400,#111401) ;
#94366=AXIS2_PLACEMENT_3D('',#144597,#111402,#111403) ;
#94367=AXIS2_PLACEMENT_3D('',#144598,#111404,#111405) ;
#94368=AXIS2_PLACEMENT_3D('',#144599,#111406,#111407) ;
#94369=AXIS2_PLACEMENT_3D('',#144600,#111408,#111409) ;
#94370=AXIS2_PLACEMENT_3D('',#144601,#111410,#111411) ;
#94371=AXIS2_PLACEMENT_3D('',#144602,#111412,#111413) ;
#94372=AXIS2_PLACEMENT_3D('',#144603,#111414,#111415) ;
#94373=AXIS2_PLACEMENT_3D('',#144604,#111416,#111417) ;
#94374=AXIS2_PLACEMENT_3D('',#144605,#111418,#111419) ;
#94375=AXIS2_PLACEMENT_3D('',#144606,#111420,#111421) ;
#94376=AXIS2_PLACEMENT_3D('',#144607,#111422,#111423) ;
#94377=AXIS2_PLACEMENT_3D('',#144608,#111424,#111425) ;
#94378=AXIS2_PLACEMENT_3D('',#144609,#111426,#111427) ;
#94379=AXIS2_PLACEMENT_3D('',#144610,#111428,#111429) ;
#94380=AXIS2_PLACEMENT_3D('',#144611,#111430,#111431) ;
#94381=AXIS2_PLACEMENT_3D('',#144626,#111438,#111439) ;
#94382=AXIS2_PLACEMENT_3D('',#144630,#111441,#111442) ;
#94383=AXIS2_PLACEMENT_3D('',#144632,#111444,#111445) ;
#94384=AXIS2_PLACEMENT_3D('',#144647,#111452,#111453) ;
#94385=AXIS2_PLACEMENT_3D('',#144651,#111455,#111456) ;
#94386=AXIS2_PLACEMENT_3D('',#144653,#111458,#111459) ;
#94387=AXIS2_PLACEMENT_3D('',#144668,#111466,#111467) ;
#94388=AXIS2_PLACEMENT_3D('',#144672,#111469,#111470) ;
#94389=AXIS2_PLACEMENT_3D('',#144674,#111472,#111473) ;
#94390=AXIS2_PLACEMENT_3D('',#144689,#111480,#111481) ;
#94391=AXIS2_PLACEMENT_3D('',#144693,#111483,#111484) ;
#94392=AXIS2_PLACEMENT_3D('',#144695,#111486,#111487) ;
#94393=AXIS2_PLACEMENT_3D('',#144710,#111494,#111495) ;
#94394=AXIS2_PLACEMENT_3D('',#144714,#111497,#111498) ;
#94395=AXIS2_PLACEMENT_3D('',#144716,#111500,#111501) ;
#94396=AXIS2_PLACEMENT_3D('',#144731,#111508,#111509) ;
#94397=AXIS2_PLACEMENT_3D('',#144735,#111511,#111512) ;
#94398=AXIS2_PLACEMENT_3D('',#144737,#111514,#111515) ;
#94399=AXIS2_PLACEMENT_3D('',#144752,#111522,#111523) ;
#94400=AXIS2_PLACEMENT_3D('',#144756,#111525,#111526) ;
#94401=AXIS2_PLACEMENT_3D('',#144758,#111528,#111529) ;
#94402=AXIS2_PLACEMENT_3D('',#144773,#111536,#111537) ;
#94403=AXIS2_PLACEMENT_3D('',#144777,#111539,#111540) ;
#94404=AXIS2_PLACEMENT_3D('',#144779,#111542,#111543) ;
#94405=AXIS2_PLACEMENT_3D('',#144794,#111550,#111551) ;
#94406=AXIS2_PLACEMENT_3D('',#144798,#111553,#111554) ;
#94407=AXIS2_PLACEMENT_3D('',#144800,#111556,#111557) ;
#94408=AXIS2_PLACEMENT_3D('',#144809,#111562,#111563) ;
#94409=AXIS2_PLACEMENT_3D('',#144815,#111567,#111568) ;
#94410=AXIS2_PLACEMENT_3D('',#144824,#111573,#111574) ;
#94411=AXIS2_PLACEMENT_3D('',#144833,#111579,#111580) ;
#94412=AXIS2_PLACEMENT_3D('',#144842,#111585,#111586) ;
#94413=AXIS2_PLACEMENT_3D('',#144851,#111591,#111592) ;
#94414=AXIS2_PLACEMENT_3D('',#144857,#111596,#111597) ;
#94415=AXIS2_PLACEMENT_3D('',#144866,#111602,#111603) ;
#94416=AXIS2_PLACEMENT_3D('',#144875,#111608,#111609) ;
#94417=AXIS2_PLACEMENT_3D('',#144884,#111614,#111615) ;
#94418=AXIS2_PLACEMENT_3D('',#144893,#111620,#111621) ;
#94419=AXIS2_PLACEMENT_3D('',#144899,#111625,#111626) ;
#94420=AXIS2_PLACEMENT_3D('',#144908,#111631,#111632) ;
#94421=AXIS2_PLACEMENT_3D('',#144917,#111637,#111638) ;
#94422=AXIS2_PLACEMENT_3D('',#144926,#111643,#111644) ;
#94423=AXIS2_PLACEMENT_3D('',#144935,#111649,#111650) ;
#94424=AXIS2_PLACEMENT_3D('',#144941,#111654,#111655) ;
#94425=AXIS2_PLACEMENT_3D('',#144950,#111660,#111661) ;
#94426=AXIS2_PLACEMENT_3D('',#144959,#111666,#111667) ;
#94427=AXIS2_PLACEMENT_3D('',#144968,#111672,#111673) ;
#94428=AXIS2_PLACEMENT_3D('',#144977,#111678,#111679) ;
#94429=AXIS2_PLACEMENT_3D('',#144983,#111683,#111684) ;
#94430=AXIS2_PLACEMENT_3D('',#144992,#111689,#111690) ;
#94431=AXIS2_PLACEMENT_3D('',#145001,#111695,#111696) ;
#94432=AXIS2_PLACEMENT_3D('',#145010,#111701,#111702) ;
#94433=AXIS2_PLACEMENT_3D('',#145019,#111707,#111708) ;
#94434=AXIS2_PLACEMENT_3D('',#145025,#111712,#111713) ;
#94435=AXIS2_PLACEMENT_3D('',#145034,#111718,#111719) ;
#94436=AXIS2_PLACEMENT_3D('',#145043,#111724,#111725) ;
#94437=AXIS2_PLACEMENT_3D('',#145052,#111730,#111731) ;
#94438=AXIS2_PLACEMENT_3D('',#145061,#111736,#111737) ;
#94439=AXIS2_PLACEMENT_3D('',#145067,#111741,#111742) ;
#94440=AXIS2_PLACEMENT_3D('',#145076,#111747,#111748) ;
#94441=AXIS2_PLACEMENT_3D('',#145085,#111753,#111754) ;
#94442=AXIS2_PLACEMENT_3D('',#145094,#111759,#111760) ;
#94443=AXIS2_PLACEMENT_3D('',#145103,#111765,#111766) ;
#94444=AXIS2_PLACEMENT_3D('',#145109,#111770,#111771) ;
#94445=AXIS2_PLACEMENT_3D('',#145118,#111776,#111777) ;
#94446=AXIS2_PLACEMENT_3D('',#145127,#111782,#111783) ;
#94447=AXIS2_PLACEMENT_3D('',#145136,#111788,#111789) ;
#94448=AXIS2_PLACEMENT_3D('',#145145,#111794,#111795) ;
#94449=AXIS2_PLACEMENT_3D('',#145151,#111799,#111800) ;
#94450=AXIS2_PLACEMENT_3D('',#145160,#111805,#111806) ;
#94451=AXIS2_PLACEMENT_3D('',#145169,#111811,#111812) ;
#94452=AXIS2_PLACEMENT_3D('',#145178,#111817,#111818) ;
#94453=AXIS2_PLACEMENT_3D('',#145183,#111820,#111821) ;
#94454=AXIS2_PLACEMENT_3D('',#145186,#111823,#111824) ;
#94455=AXIS2_PLACEMENT_3D('',#145187,#111825,#111826) ;
#94456=AXIS2_PLACEMENT_3D('',#145193,#111830,#111831) ;
#94457=AXIS2_PLACEMENT_3D('',#145195,#111832,#111833) ;
#94458=AXIS2_PLACEMENT_3D('',#145198,#111835,#111836) ;
#94459=AXIS2_PLACEMENT_3D('',#145199,#111837,#111838) ;
#94460=AXIS2_PLACEMENT_3D('',#145205,#111842,#111843) ;
#94461=AXIS2_PLACEMENT_3D('',#145207,#111844,#111845) ;
#94462=AXIS2_PLACEMENT_3D('',#145210,#111847,#111848) ;
#94463=AXIS2_PLACEMENT_3D('',#145211,#111849,#111850) ;
#94464=AXIS2_PLACEMENT_3D('',#145216,#111854,#111855) ;
#94465=AXIS2_PLACEMENT_3D('',#145219,#111857,#111858) ;
#94466=AXIS2_PLACEMENT_3D('',#145220,#111859,#111860) ;
#94467=AXIS2_PLACEMENT_3D('',#145223,#111863,#111864) ;
#94468=AXIS2_PLACEMENT_3D('',#145229,#111868,#111869) ;
#94469=AXIS2_PLACEMENT_3D('',#145231,#111870,#111871) ;
#94470=AXIS2_PLACEMENT_3D('',#145234,#111873,#111874) ;
#94471=AXIS2_PLACEMENT_3D('',#145235,#111875,#111876) ;
#94472=AXIS2_PLACEMENT_3D('',#145241,#111880,#111881) ;
#94473=AXIS2_PLACEMENT_3D('',#145243,#111882,#111883) ;
#94474=AXIS2_PLACEMENT_3D('',#145246,#111885,#111886) ;
#94475=AXIS2_PLACEMENT_3D('',#145247,#111887,#111888) ;
#94476=AXIS2_PLACEMENT_3D('',#145253,#111892,#111893) ;
#94477=AXIS2_PLACEMENT_3D('',#145255,#111894,#111895) ;
#94478=AXIS2_PLACEMENT_3D('',#145258,#111897,#111898) ;
#94479=AXIS2_PLACEMENT_3D('',#145259,#111899,#111900) ;
#94480=AXIS2_PLACEMENT_3D('',#145265,#111904,#111905) ;
#94481=AXIS2_PLACEMENT_3D('',#145267,#111906,#111907) ;
#94482=AXIS2_PLACEMENT_3D('',#145270,#111909,#111910) ;
#94483=AXIS2_PLACEMENT_3D('',#145271,#111911,#111912) ;
#94484=AXIS2_PLACEMENT_3D('',#145277,#111916,#111917) ;
#94485=AXIS2_PLACEMENT_3D('',#145279,#111918,#111919) ;
#94486=AXIS2_PLACEMENT_3D('',#145282,#111921,#111922) ;
#94487=AXIS2_PLACEMENT_3D('',#145283,#111923,#111924) ;
#94488=AXIS2_PLACEMENT_3D('',#145289,#111928,#111929) ;
#94489=AXIS2_PLACEMENT_3D('',#145291,#111930,#111931) ;
#94490=AXIS2_PLACEMENT_3D('',#145294,#111933,#111934) ;
#94491=AXIS2_PLACEMENT_3D('',#145295,#111935,#111936) ;
#94492=AXIS2_PLACEMENT_3D('',#145297,#111937,#111938) ;
#94493=AXIS2_PLACEMENT_3D('',#145300,#111940,#111941) ;
#94494=AXIS2_PLACEMENT_3D('',#145301,#111942,#111943) ;
#94495=AXIS2_PLACEMENT_3D('',#145303,#111944,#111945) ;
#94496=AXIS2_PLACEMENT_3D('',#145306,#111947,#111948) ;
#94497=AXIS2_PLACEMENT_3D('',#145307,#111949,#111950) ;
#94498=AXIS2_PLACEMENT_3D('',#145313,#111954,#111955) ;
#94499=AXIS2_PLACEMENT_3D('',#145315,#111956,#111957) ;
#94500=AXIS2_PLACEMENT_3D('',#145318,#111959,#111960) ;
#94501=AXIS2_PLACEMENT_3D('',#145319,#111961,#111962) ;
#94502=AXIS2_PLACEMENT_3D('',#145325,#111966,#111967) ;
#94503=AXIS2_PLACEMENT_3D('',#145327,#111968,#111969) ;
#94504=AXIS2_PLACEMENT_3D('',#145330,#111971,#111972) ;
#94505=AXIS2_PLACEMENT_3D('',#145331,#111973,#111974) ;
#94506=AXIS2_PLACEMENT_3D('',#145334,#111977,#111978) ;
#94507=AXIS2_PLACEMENT_3D('',#145337,#111979,#111980) ;
#94508=AXIS2_PLACEMENT_3D('',#145341,#111982,#111983) ;
#94509=AXIS2_PLACEMENT_3D('',#145349,#111987,#111988) ;
#94510=AXIS2_PLACEMENT_3D('',#145357,#111992,#111993) ;
#94511=AXIS2_PLACEMENT_3D('',#145361,#111995,#111996) ;
#94512=AXIS2_PLACEMENT_3D('',#145370,#112002,#112003) ;
#94513=AXIS2_PLACEMENT_3D('',#145375,#112005,#112006) ;
#94514=AXIS2_PLACEMENT_3D('',#145378,#112008,#112009) ;
#94515=AXIS2_PLACEMENT_3D('',#145379,#112010,#112011) ;
#94516=AXIS2_PLACEMENT_3D('',#145385,#112015,#112016) ;
#94517=AXIS2_PLACEMENT_3D('',#145387,#112017,#112018) ;
#94518=AXIS2_PLACEMENT_3D('',#145390,#112020,#112021) ;
#94519=AXIS2_PLACEMENT_3D('',#145391,#112022,#112023) ;
#94520=AXIS2_PLACEMENT_3D('',#145397,#112027,#112028) ;
#94521=AXIS2_PLACEMENT_3D('',#145399,#112029,#112030) ;
#94522=AXIS2_PLACEMENT_3D('',#145402,#112032,#112033) ;
#94523=AXIS2_PLACEMENT_3D('',#145403,#112034,#112035) ;
#94524=AXIS2_PLACEMENT_3D('',#145408,#112039,#112040) ;
#94525=AXIS2_PLACEMENT_3D('',#145411,#112042,#112043) ;
#94526=AXIS2_PLACEMENT_3D('',#145412,#112044,#112045) ;
#94527=AXIS2_PLACEMENT_3D('',#145415,#112048,#112049) ;
#94528=AXIS2_PLACEMENT_3D('',#145421,#112053,#112054) ;
#94529=AXIS2_PLACEMENT_3D('',#145423,#112055,#112056) ;
#94530=AXIS2_PLACEMENT_3D('',#145426,#112058,#112059) ;
#94531=AXIS2_PLACEMENT_3D('',#145427,#112060,#112061) ;
#94532=AXIS2_PLACEMENT_3D('',#145433,#112065,#112066) ;
#94533=AXIS2_PLACEMENT_3D('',#145435,#112067,#112068) ;
#94534=AXIS2_PLACEMENT_3D('',#145438,#112070,#112071) ;
#94535=AXIS2_PLACEMENT_3D('',#145439,#112072,#112073) ;
#94536=AXIS2_PLACEMENT_3D('',#145445,#112077,#112078) ;
#94537=AXIS2_PLACEMENT_3D('',#145447,#112079,#112080) ;
#94538=AXIS2_PLACEMENT_3D('',#145450,#112082,#112083) ;
#94539=AXIS2_PLACEMENT_3D('',#145451,#112084,#112085) ;
#94540=AXIS2_PLACEMENT_3D('',#145457,#112089,#112090) ;
#94541=AXIS2_PLACEMENT_3D('',#145459,#112091,#112092) ;
#94542=AXIS2_PLACEMENT_3D('',#145462,#112094,#112095) ;
#94543=AXIS2_PLACEMENT_3D('',#145463,#112096,#112097) ;
#94544=AXIS2_PLACEMENT_3D('',#145469,#112101,#112102) ;
#94545=AXIS2_PLACEMENT_3D('',#145471,#112103,#112104) ;
#94546=AXIS2_PLACEMENT_3D('',#145474,#112106,#112107) ;
#94547=AXIS2_PLACEMENT_3D('',#145475,#112108,#112109) ;
#94548=AXIS2_PLACEMENT_3D('',#145481,#112113,#112114) ;
#94549=AXIS2_PLACEMENT_3D('',#145483,#112115,#112116) ;
#94550=AXIS2_PLACEMENT_3D('',#145486,#112118,#112119) ;
#94551=AXIS2_PLACEMENT_3D('',#145487,#112120,#112121) ;
#94552=AXIS2_PLACEMENT_3D('',#145489,#112122,#112123) ;
#94553=AXIS2_PLACEMENT_3D('',#145492,#112125,#112126) ;
#94554=AXIS2_PLACEMENT_3D('',#145493,#112127,#112128) ;
#94555=AXIS2_PLACEMENT_3D('',#145495,#112129,#112130) ;
#94556=AXIS2_PLACEMENT_3D('',#145498,#112132,#112133) ;
#94557=AXIS2_PLACEMENT_3D('',#145499,#112134,#112135) ;
#94558=AXIS2_PLACEMENT_3D('',#145505,#112139,#112140) ;
#94559=AXIS2_PLACEMENT_3D('',#145507,#112141,#112142) ;
#94560=AXIS2_PLACEMENT_3D('',#145510,#112144,#112145) ;
#94561=AXIS2_PLACEMENT_3D('',#145511,#112146,#112147) ;
#94562=AXIS2_PLACEMENT_3D('',#145517,#112151,#112152) ;
#94563=AXIS2_PLACEMENT_3D('',#145519,#112153,#112154) ;
#94564=AXIS2_PLACEMENT_3D('',#145522,#112156,#112157) ;
#94565=AXIS2_PLACEMENT_3D('',#145523,#112158,#112159) ;
#94566=AXIS2_PLACEMENT_3D('',#145526,#112162,#112163) ;
#94567=AXIS2_PLACEMENT_3D('',#145529,#112164,#112165) ;
#94568=AXIS2_PLACEMENT_3D('',#145533,#112167,#112168) ;
#94569=AXIS2_PLACEMENT_3D('',#145541,#112172,#112173) ;
#94570=AXIS2_PLACEMENT_3D('',#145549,#112177,#112178) ;
#94571=AXIS2_PLACEMENT_3D('',#145553,#112180,#112181) ;
#94572=AXIS2_PLACEMENT_3D('',#145562,#112187,#112188) ;
#94573=AXIS2_PLACEMENT_3D('',#145567,#112190,#112191) ;
#94574=AXIS2_PLACEMENT_3D('',#145570,#112193,#112194) ;
#94575=AXIS2_PLACEMENT_3D('',#145571,#112195,#112196) ;
#94576=AXIS2_PLACEMENT_3D('',#145577,#112200,#112201) ;
#94577=AXIS2_PLACEMENT_3D('',#145579,#112202,#112203) ;
#94578=AXIS2_PLACEMENT_3D('',#145582,#112205,#112206) ;
#94579=AXIS2_PLACEMENT_3D('',#145583,#112207,#112208) ;
#94580=AXIS2_PLACEMENT_3D('',#145589,#112212,#112213) ;
#94581=AXIS2_PLACEMENT_3D('',#145591,#112214,#112215) ;
#94582=AXIS2_PLACEMENT_3D('',#145594,#112217,#112218) ;
#94583=AXIS2_PLACEMENT_3D('',#145595,#112219,#112220) ;
#94584=AXIS2_PLACEMENT_3D('',#145600,#112224,#112225) ;
#94585=AXIS2_PLACEMENT_3D('',#145603,#112227,#112228) ;
#94586=AXIS2_PLACEMENT_3D('',#145604,#112229,#112230) ;
#94587=AXIS2_PLACEMENT_3D('',#145607,#112233,#112234) ;
#94588=AXIS2_PLACEMENT_3D('',#145613,#112238,#112239) ;
#94589=AXIS2_PLACEMENT_3D('',#145615,#112240,#112241) ;
#94590=AXIS2_PLACEMENT_3D('',#145618,#112243,#112244) ;
#94591=AXIS2_PLACEMENT_3D('',#145619,#112245,#112246) ;
#94592=AXIS2_PLACEMENT_3D('',#145625,#112250,#112251) ;
#94593=AXIS2_PLACEMENT_3D('',#145627,#112252,#112253) ;
#94594=AXIS2_PLACEMENT_3D('',#145630,#112255,#112256) ;
#94595=AXIS2_PLACEMENT_3D('',#145631,#112257,#112258) ;
#94596=AXIS2_PLACEMENT_3D('',#145637,#112262,#112263) ;
#94597=AXIS2_PLACEMENT_3D('',#145639,#112264,#112265) ;
#94598=AXIS2_PLACEMENT_3D('',#145642,#112267,#112268) ;
#94599=AXIS2_PLACEMENT_3D('',#145643,#112269,#112270) ;
#94600=AXIS2_PLACEMENT_3D('',#145649,#112274,#112275) ;
#94601=AXIS2_PLACEMENT_3D('',#145651,#112276,#112277) ;
#94602=AXIS2_PLACEMENT_3D('',#145654,#112279,#112280) ;
#94603=AXIS2_PLACEMENT_3D('',#145655,#112281,#112282) ;
#94604=AXIS2_PLACEMENT_3D('',#145661,#112286,#112287) ;
#94605=AXIS2_PLACEMENT_3D('',#145663,#112288,#112289) ;
#94606=AXIS2_PLACEMENT_3D('',#145666,#112291,#112292) ;
#94607=AXIS2_PLACEMENT_3D('',#145667,#112293,#112294) ;
#94608=AXIS2_PLACEMENT_3D('',#145673,#112298,#112299) ;
#94609=AXIS2_PLACEMENT_3D('',#145675,#112300,#112301) ;
#94610=AXIS2_PLACEMENT_3D('',#145678,#112303,#112304) ;
#94611=AXIS2_PLACEMENT_3D('',#145679,#112305,#112306) ;
#94612=AXIS2_PLACEMENT_3D('',#145681,#112307,#112308) ;
#94613=AXIS2_PLACEMENT_3D('',#145684,#112310,#112311) ;
#94614=AXIS2_PLACEMENT_3D('',#145685,#112312,#112313) ;
#94615=AXIS2_PLACEMENT_3D('',#145687,#112314,#112315) ;
#94616=AXIS2_PLACEMENT_3D('',#145690,#112317,#112318) ;
#94617=AXIS2_PLACEMENT_3D('',#145691,#112319,#112320) ;
#94618=AXIS2_PLACEMENT_3D('',#145697,#112324,#112325) ;
#94619=AXIS2_PLACEMENT_3D('',#145699,#112326,#112327) ;
#94620=AXIS2_PLACEMENT_3D('',#145702,#112329,#112330) ;
#94621=AXIS2_PLACEMENT_3D('',#145703,#112331,#112332) ;
#94622=AXIS2_PLACEMENT_3D('',#145709,#112336,#112337) ;
#94623=AXIS2_PLACEMENT_3D('',#145711,#112338,#112339) ;
#94624=AXIS2_PLACEMENT_3D('',#145714,#112341,#112342) ;
#94625=AXIS2_PLACEMENT_3D('',#145715,#112343,#112344) ;
#94626=AXIS2_PLACEMENT_3D('',#145718,#112347,#112348) ;
#94627=AXIS2_PLACEMENT_3D('',#145721,#112349,#112350) ;
#94628=AXIS2_PLACEMENT_3D('',#145725,#112352,#112353) ;
#94629=AXIS2_PLACEMENT_3D('',#145733,#112357,#112358) ;
#94630=AXIS2_PLACEMENT_3D('',#145741,#112362,#112363) ;
#94631=AXIS2_PLACEMENT_3D('',#145745,#112365,#112366) ;
#94632=AXIS2_PLACEMENT_3D('',#145754,#112372,#112373) ;
#94633=AXIS2_PLACEMENT_3D('',#145759,#112375,#112376) ;
#94634=AXIS2_PLACEMENT_3D('',#145762,#112378,#112379) ;
#94635=AXIS2_PLACEMENT_3D('',#145763,#112380,#112381) ;
#94636=AXIS2_PLACEMENT_3D('',#145769,#112385,#112386) ;
#94637=AXIS2_PLACEMENT_3D('',#145771,#112387,#112388) ;
#94638=AXIS2_PLACEMENT_3D('',#145774,#112390,#112391) ;
#94639=AXIS2_PLACEMENT_3D('',#145775,#112392,#112393) ;
#94640=AXIS2_PLACEMENT_3D('',#145781,#112397,#112398) ;
#94641=AXIS2_PLACEMENT_3D('',#145783,#112399,#112400) ;
#94642=AXIS2_PLACEMENT_3D('',#145786,#112402,#112403) ;
#94643=AXIS2_PLACEMENT_3D('',#145787,#112404,#112405) ;
#94644=AXIS2_PLACEMENT_3D('',#145792,#112409,#112410) ;
#94645=AXIS2_PLACEMENT_3D('',#145795,#112412,#112413) ;
#94646=AXIS2_PLACEMENT_3D('',#145796,#112414,#112415) ;
#94647=AXIS2_PLACEMENT_3D('',#145799,#112418,#112419) ;
#94648=AXIS2_PLACEMENT_3D('',#145805,#112423,#112424) ;
#94649=AXIS2_PLACEMENT_3D('',#145807,#112425,#112426) ;
#94650=AXIS2_PLACEMENT_3D('',#145810,#112428,#112429) ;
#94651=AXIS2_PLACEMENT_3D('',#145811,#112430,#112431) ;
#94652=AXIS2_PLACEMENT_3D('',#145817,#112435,#112436) ;
#94653=AXIS2_PLACEMENT_3D('',#145819,#112437,#112438) ;
#94654=AXIS2_PLACEMENT_3D('',#145822,#112440,#112441) ;
#94655=AXIS2_PLACEMENT_3D('',#145823,#112442,#112443) ;
#94656=AXIS2_PLACEMENT_3D('',#145829,#112447,#112448) ;
#94657=AXIS2_PLACEMENT_3D('',#145831,#112449,#112450) ;
#94658=AXIS2_PLACEMENT_3D('',#145834,#112452,#112453) ;
#94659=AXIS2_PLACEMENT_3D('',#145835,#112454,#112455) ;
#94660=AXIS2_PLACEMENT_3D('',#145841,#112459,#112460) ;
#94661=AXIS2_PLACEMENT_3D('',#145843,#112461,#112462) ;
#94662=AXIS2_PLACEMENT_3D('',#145846,#112464,#112465) ;
#94663=AXIS2_PLACEMENT_3D('',#145847,#112466,#112467) ;
#94664=AXIS2_PLACEMENT_3D('',#145853,#112471,#112472) ;
#94665=AXIS2_PLACEMENT_3D('',#145855,#112473,#112474) ;
#94666=AXIS2_PLACEMENT_3D('',#145858,#112476,#112477) ;
#94667=AXIS2_PLACEMENT_3D('',#145859,#112478,#112479) ;
#94668=AXIS2_PLACEMENT_3D('',#145865,#112483,#112484) ;
#94669=AXIS2_PLACEMENT_3D('',#145867,#112485,#112486) ;
#94670=AXIS2_PLACEMENT_3D('',#145870,#112488,#112489) ;
#94671=AXIS2_PLACEMENT_3D('',#145871,#112490,#112491) ;
#94672=AXIS2_PLACEMENT_3D('',#145873,#112492,#112493) ;
#94673=AXIS2_PLACEMENT_3D('',#145876,#112495,#112496) ;
#94674=AXIS2_PLACEMENT_3D('',#145877,#112497,#112498) ;
#94675=AXIS2_PLACEMENT_3D('',#145879,#112499,#112500) ;
#94676=AXIS2_PLACEMENT_3D('',#145882,#112502,#112503) ;
#94677=AXIS2_PLACEMENT_3D('',#145883,#112504,#112505) ;
#94678=AXIS2_PLACEMENT_3D('',#145889,#112509,#112510) ;
#94679=AXIS2_PLACEMENT_3D('',#145891,#112511,#112512) ;
#94680=AXIS2_PLACEMENT_3D('',#145894,#112514,#112515) ;
#94681=AXIS2_PLACEMENT_3D('',#145895,#112516,#112517) ;
#94682=AXIS2_PLACEMENT_3D('',#145901,#112521,#112522) ;
#94683=AXIS2_PLACEMENT_3D('',#145903,#112523,#112524) ;
#94684=AXIS2_PLACEMENT_3D('',#145906,#112526,#112527) ;
#94685=AXIS2_PLACEMENT_3D('',#145907,#112528,#112529) ;
#94686=AXIS2_PLACEMENT_3D('',#145910,#112532,#112533) ;
#94687=AXIS2_PLACEMENT_3D('',#145913,#112534,#112535) ;
#94688=AXIS2_PLACEMENT_3D('',#145917,#112537,#112538) ;
#94689=AXIS2_PLACEMENT_3D('',#145925,#112542,#112543) ;
#94690=AXIS2_PLACEMENT_3D('',#145933,#112547,#112548) ;
#94691=AXIS2_PLACEMENT_3D('',#145937,#112550,#112551) ;
#94692=AXIS2_PLACEMENT_3D('',#145946,#112557,#112558) ;
#94693=AXIS2_PLACEMENT_3D('',#145951,#112560,#112561) ;
#94694=AXIS2_PLACEMENT_3D('',#145954,#112563,#112564) ;
#94695=AXIS2_PLACEMENT_3D('',#145955,#112565,#112566) ;
#94696=AXIS2_PLACEMENT_3D('',#145961,#112570,#112571) ;
#94697=AXIS2_PLACEMENT_3D('',#145963,#112572,#112573) ;
#94698=AXIS2_PLACEMENT_3D('',#145966,#112575,#112576) ;
#94699=AXIS2_PLACEMENT_3D('',#145967,#112577,#112578) ;
#94700=AXIS2_PLACEMENT_3D('',#145973,#112582,#112583) ;
#94701=AXIS2_PLACEMENT_3D('',#145975,#112584,#112585) ;
#94702=AXIS2_PLACEMENT_3D('',#145978,#112587,#112588) ;
#94703=AXIS2_PLACEMENT_3D('',#145979,#112589,#112590) ;
#94704=AXIS2_PLACEMENT_3D('',#145984,#112594,#112595) ;
#94705=AXIS2_PLACEMENT_3D('',#145987,#112597,#112598) ;
#94706=AXIS2_PLACEMENT_3D('',#145988,#112599,#112600) ;
#94707=AXIS2_PLACEMENT_3D('',#145991,#112603,#112604) ;
#94708=AXIS2_PLACEMENT_3D('',#145997,#112608,#112609) ;
#94709=AXIS2_PLACEMENT_3D('',#145999,#112610,#112611) ;
#94710=AXIS2_PLACEMENT_3D('',#146002,#112613,#112614) ;
#94711=AXIS2_PLACEMENT_3D('',#146003,#112615,#112616) ;
#94712=AXIS2_PLACEMENT_3D('',#146009,#112620,#112621) ;
#94713=AXIS2_PLACEMENT_3D('',#146011,#112622,#112623) ;
#94714=AXIS2_PLACEMENT_3D('',#146014,#112625,#112626) ;
#94715=AXIS2_PLACEMENT_3D('',#146015,#112627,#112628) ;
#94716=AXIS2_PLACEMENT_3D('',#146021,#112632,#112633) ;
#94717=AXIS2_PLACEMENT_3D('',#146023,#112634,#112635) ;
#94718=AXIS2_PLACEMENT_3D('',#146026,#112637,#112638) ;
#94719=AXIS2_PLACEMENT_3D('',#146027,#112639,#112640) ;
#94720=AXIS2_PLACEMENT_3D('',#146033,#112644,#112645) ;
#94721=AXIS2_PLACEMENT_3D('',#146035,#112646,#112647) ;
#94722=AXIS2_PLACEMENT_3D('',#146038,#112649,#112650) ;
#94723=AXIS2_PLACEMENT_3D('',#146039,#112651,#112652) ;
#94724=AXIS2_PLACEMENT_3D('',#146045,#112656,#112657) ;
#94725=AXIS2_PLACEMENT_3D('',#146047,#112658,#112659) ;
#94726=AXIS2_PLACEMENT_3D('',#146050,#112661,#112662) ;
#94727=AXIS2_PLACEMENT_3D('',#146051,#112663,#112664) ;
#94728=AXIS2_PLACEMENT_3D('',#146057,#112668,#112669) ;
#94729=AXIS2_PLACEMENT_3D('',#146059,#112670,#112671) ;
#94730=AXIS2_PLACEMENT_3D('',#146062,#112673,#112674) ;
#94731=AXIS2_PLACEMENT_3D('',#146063,#112675,#112676) ;
#94732=AXIS2_PLACEMENT_3D('',#146065,#112677,#112678) ;
#94733=AXIS2_PLACEMENT_3D('',#146068,#112680,#112681) ;
#94734=AXIS2_PLACEMENT_3D('',#146069,#112682,#112683) ;
#94735=AXIS2_PLACEMENT_3D('',#146071,#112684,#112685) ;
#94736=AXIS2_PLACEMENT_3D('',#146074,#112687,#112688) ;
#94737=AXIS2_PLACEMENT_3D('',#146075,#112689,#112690) ;
#94738=AXIS2_PLACEMENT_3D('',#146081,#112694,#112695) ;
#94739=AXIS2_PLACEMENT_3D('',#146083,#112696,#112697) ;
#94740=AXIS2_PLACEMENT_3D('',#146086,#112699,#112700) ;
#94741=AXIS2_PLACEMENT_3D('',#146087,#112701,#112702) ;
#94742=AXIS2_PLACEMENT_3D('',#146093,#112706,#112707) ;
#94743=AXIS2_PLACEMENT_3D('',#146095,#112708,#112709) ;
#94744=AXIS2_PLACEMENT_3D('',#146098,#112711,#112712) ;
#94745=AXIS2_PLACEMENT_3D('',#146099,#112713,#112714) ;
#94746=AXIS2_PLACEMENT_3D('',#146102,#112717,#112718) ;
#94747=AXIS2_PLACEMENT_3D('',#146105,#112719,#112720) ;
#94748=AXIS2_PLACEMENT_3D('',#146109,#112722,#112723) ;
#94749=AXIS2_PLACEMENT_3D('',#146117,#112727,#112728) ;
#94750=AXIS2_PLACEMENT_3D('',#146125,#112732,#112733) ;
#94751=AXIS2_PLACEMENT_3D('',#146129,#112735,#112736) ;
#94752=AXIS2_PLACEMENT_3D('',#146138,#112742,#112743) ;
#94753=AXIS2_PLACEMENT_3D('',#146143,#112745,#112746) ;
#94754=AXIS2_PLACEMENT_3D('',#146146,#112748,#112749) ;
#94755=AXIS2_PLACEMENT_3D('',#146147,#112750,#112751) ;
#94756=AXIS2_PLACEMENT_3D('',#146153,#112755,#112756) ;
#94757=AXIS2_PLACEMENT_3D('',#146155,#112757,#112758) ;
#94758=AXIS2_PLACEMENT_3D('',#146158,#112760,#112761) ;
#94759=AXIS2_PLACEMENT_3D('',#146159,#112762,#112763) ;
#94760=AXIS2_PLACEMENT_3D('',#146165,#112767,#112768) ;
#94761=AXIS2_PLACEMENT_3D('',#146167,#112769,#112770) ;
#94762=AXIS2_PLACEMENT_3D('',#146170,#112772,#112773) ;
#94763=AXIS2_PLACEMENT_3D('',#146171,#112774,#112775) ;
#94764=AXIS2_PLACEMENT_3D('',#146176,#112779,#112780) ;
#94765=AXIS2_PLACEMENT_3D('',#146179,#112782,#112783) ;
#94766=AXIS2_PLACEMENT_3D('',#146180,#112784,#112785) ;
#94767=AXIS2_PLACEMENT_3D('',#146183,#112788,#112789) ;
#94768=AXIS2_PLACEMENT_3D('',#146189,#112793,#112794) ;
#94769=AXIS2_PLACEMENT_3D('',#146191,#112795,#112796) ;
#94770=AXIS2_PLACEMENT_3D('',#146194,#112798,#112799) ;
#94771=AXIS2_PLACEMENT_3D('',#146195,#112800,#112801) ;
#94772=AXIS2_PLACEMENT_3D('',#146201,#112805,#112806) ;
#94773=AXIS2_PLACEMENT_3D('',#146203,#112807,#112808) ;
#94774=AXIS2_PLACEMENT_3D('',#146206,#112810,#112811) ;
#94775=AXIS2_PLACEMENT_3D('',#146207,#112812,#112813) ;
#94776=AXIS2_PLACEMENT_3D('',#146213,#112817,#112818) ;
#94777=AXIS2_PLACEMENT_3D('',#146215,#112819,#112820) ;
#94778=AXIS2_PLACEMENT_3D('',#146218,#112822,#112823) ;
#94779=AXIS2_PLACEMENT_3D('',#146219,#112824,#112825) ;
#94780=AXIS2_PLACEMENT_3D('',#146225,#112829,#112830) ;
#94781=AXIS2_PLACEMENT_3D('',#146227,#112831,#112832) ;
#94782=AXIS2_PLACEMENT_3D('',#146230,#112834,#112835) ;
#94783=AXIS2_PLACEMENT_3D('',#146231,#112836,#112837) ;
#94784=AXIS2_PLACEMENT_3D('',#146237,#112841,#112842) ;
#94785=AXIS2_PLACEMENT_3D('',#146239,#112843,#112844) ;
#94786=AXIS2_PLACEMENT_3D('',#146242,#112846,#112847) ;
#94787=AXIS2_PLACEMENT_3D('',#146243,#112848,#112849) ;
#94788=AXIS2_PLACEMENT_3D('',#146249,#112853,#112854) ;
#94789=AXIS2_PLACEMENT_3D('',#146251,#112855,#112856) ;
#94790=AXIS2_PLACEMENT_3D('',#146254,#112858,#112859) ;
#94791=AXIS2_PLACEMENT_3D('',#146255,#112860,#112861) ;
#94792=AXIS2_PLACEMENT_3D('',#146257,#112862,#112863) ;
#94793=AXIS2_PLACEMENT_3D('',#146260,#112865,#112866) ;
#94794=AXIS2_PLACEMENT_3D('',#146261,#112867,#112868) ;
#94795=AXIS2_PLACEMENT_3D('',#146263,#112869,#112870) ;
#94796=AXIS2_PLACEMENT_3D('',#146266,#112872,#112873) ;
#94797=AXIS2_PLACEMENT_3D('',#146267,#112874,#112875) ;
#94798=AXIS2_PLACEMENT_3D('',#146273,#112879,#112880) ;
#94799=AXIS2_PLACEMENT_3D('',#146275,#112881,#112882) ;
#94800=AXIS2_PLACEMENT_3D('',#146278,#112884,#112885) ;
#94801=AXIS2_PLACEMENT_3D('',#146279,#112886,#112887) ;
#94802=AXIS2_PLACEMENT_3D('',#146285,#112891,#112892) ;
#94803=AXIS2_PLACEMENT_3D('',#146287,#112893,#112894) ;
#94804=AXIS2_PLACEMENT_3D('',#146290,#112896,#112897) ;
#94805=AXIS2_PLACEMENT_3D('',#146291,#112898,#112899) ;
#94806=AXIS2_PLACEMENT_3D('',#146294,#112902,#112903) ;
#94807=AXIS2_PLACEMENT_3D('',#146297,#112904,#112905) ;
#94808=AXIS2_PLACEMENT_3D('',#146301,#112907,#112908) ;
#94809=AXIS2_PLACEMENT_3D('',#146309,#112912,#112913) ;
#94810=AXIS2_PLACEMENT_3D('',#146317,#112917,#112918) ;
#94811=AXIS2_PLACEMENT_3D('',#146321,#112920,#112921) ;
#94812=AXIS2_PLACEMENT_3D('',#146330,#112927,#112928) ;
#94813=AXIS2_PLACEMENT_3D('',#146335,#112930,#112931) ;
#94814=AXIS2_PLACEMENT_3D('',#146338,#112933,#112934) ;
#94815=AXIS2_PLACEMENT_3D('',#146339,#112935,#112936) ;
#94816=AXIS2_PLACEMENT_3D('',#146345,#112940,#112941) ;
#94817=AXIS2_PLACEMENT_3D('',#146347,#112942,#112943) ;
#94818=AXIS2_PLACEMENT_3D('',#146350,#112945,#112946) ;
#94819=AXIS2_PLACEMENT_3D('',#146351,#112947,#112948) ;
#94820=AXIS2_PLACEMENT_3D('',#146357,#112952,#112953) ;
#94821=AXIS2_PLACEMENT_3D('',#146359,#112954,#112955) ;
#94822=AXIS2_PLACEMENT_3D('',#146362,#112957,#112958) ;
#94823=AXIS2_PLACEMENT_3D('',#146363,#112959,#112960) ;
#94824=AXIS2_PLACEMENT_3D('',#146368,#112964,#112965) ;
#94825=AXIS2_PLACEMENT_3D('',#146371,#112967,#112968) ;
#94826=AXIS2_PLACEMENT_3D('',#146372,#112969,#112970) ;
#94827=AXIS2_PLACEMENT_3D('',#146375,#112973,#112974) ;
#94828=AXIS2_PLACEMENT_3D('',#146381,#112978,#112979) ;
#94829=AXIS2_PLACEMENT_3D('',#146383,#112980,#112981) ;
#94830=AXIS2_PLACEMENT_3D('',#146386,#112983,#112984) ;
#94831=AXIS2_PLACEMENT_3D('',#146387,#112985,#112986) ;
#94832=AXIS2_PLACEMENT_3D('',#146393,#112990,#112991) ;
#94833=AXIS2_PLACEMENT_3D('',#146395,#112992,#112993) ;
#94834=AXIS2_PLACEMENT_3D('',#146398,#112995,#112996) ;
#94835=AXIS2_PLACEMENT_3D('',#146399,#112997,#112998) ;
#94836=AXIS2_PLACEMENT_3D('',#146405,#113002,#113003) ;
#94837=AXIS2_PLACEMENT_3D('',#146407,#113004,#113005) ;
#94838=AXIS2_PLACEMENT_3D('',#146410,#113007,#113008) ;
#94839=AXIS2_PLACEMENT_3D('',#146411,#113009,#113010) ;
#94840=AXIS2_PLACEMENT_3D('',#146417,#113014,#113015) ;
#94841=AXIS2_PLACEMENT_3D('',#146419,#113016,#113017) ;
#94842=AXIS2_PLACEMENT_3D('',#146422,#113019,#113020) ;
#94843=AXIS2_PLACEMENT_3D('',#146423,#113021,#113022) ;
#94844=AXIS2_PLACEMENT_3D('',#146429,#113026,#113027) ;
#94845=AXIS2_PLACEMENT_3D('',#146431,#113028,#113029) ;
#94846=AXIS2_PLACEMENT_3D('',#146434,#113031,#113032) ;
#94847=AXIS2_PLACEMENT_3D('',#146435,#113033,#113034) ;
#94848=AXIS2_PLACEMENT_3D('',#146441,#113038,#113039) ;
#94849=AXIS2_PLACEMENT_3D('',#146443,#113040,#113041) ;
#94850=AXIS2_PLACEMENT_3D('',#146446,#113043,#113044) ;
#94851=AXIS2_PLACEMENT_3D('',#146447,#113045,#113046) ;
#94852=AXIS2_PLACEMENT_3D('',#146449,#113047,#113048) ;
#94853=AXIS2_PLACEMENT_3D('',#146452,#113050,#113051) ;
#94854=AXIS2_PLACEMENT_3D('',#146453,#113052,#113053) ;
#94855=AXIS2_PLACEMENT_3D('',#146455,#113054,#113055) ;
#94856=AXIS2_PLACEMENT_3D('',#146458,#113057,#113058) ;
#94857=AXIS2_PLACEMENT_3D('',#146459,#113059,#113060) ;
#94858=AXIS2_PLACEMENT_3D('',#146465,#113064,#113065) ;
#94859=AXIS2_PLACEMENT_3D('',#146467,#113066,#113067) ;
#94860=AXIS2_PLACEMENT_3D('',#146470,#113069,#113070) ;
#94861=AXIS2_PLACEMENT_3D('',#146471,#113071,#113072) ;
#94862=AXIS2_PLACEMENT_3D('',#146477,#113076,#113077) ;
#94863=AXIS2_PLACEMENT_3D('',#146479,#113078,#113079) ;
#94864=AXIS2_PLACEMENT_3D('',#146482,#113081,#113082) ;
#94865=AXIS2_PLACEMENT_3D('',#146483,#113083,#113084) ;
#94866=AXIS2_PLACEMENT_3D('',#146486,#113087,#113088) ;
#94867=AXIS2_PLACEMENT_3D('',#146489,#113089,#113090) ;
#94868=AXIS2_PLACEMENT_3D('',#146493,#113092,#113093) ;
#94869=AXIS2_PLACEMENT_3D('',#146501,#113097,#113098) ;
#94870=AXIS2_PLACEMENT_3D('',#146509,#113102,#113103) ;
#94871=AXIS2_PLACEMENT_3D('',#146513,#113105,#113106) ;
#94872=AXIS2_PLACEMENT_3D('',#146522,#113112,#113113) ;
#94873=AXIS2_PLACEMENT_3D('',#146527,#113115,#113116) ;
#94874=AXIS2_PLACEMENT_3D('',#146530,#113118,#113119) ;
#94875=AXIS2_PLACEMENT_3D('',#146531,#113120,#113121) ;
#94876=AXIS2_PLACEMENT_3D('',#146537,#113125,#113126) ;
#94877=AXIS2_PLACEMENT_3D('',#146539,#113127,#113128) ;
#94878=AXIS2_PLACEMENT_3D('',#146542,#113130,#113131) ;
#94879=AXIS2_PLACEMENT_3D('',#146543,#113132,#113133) ;
#94880=AXIS2_PLACEMENT_3D('',#146549,#113137,#113138) ;
#94881=AXIS2_PLACEMENT_3D('',#146551,#113139,#113140) ;
#94882=AXIS2_PLACEMENT_3D('',#146554,#113142,#113143) ;
#94883=AXIS2_PLACEMENT_3D('',#146555,#113144,#113145) ;
#94884=AXIS2_PLACEMENT_3D('',#146560,#113149,#113150) ;
#94885=AXIS2_PLACEMENT_3D('',#146563,#113152,#113153) ;
#94886=AXIS2_PLACEMENT_3D('',#146564,#113154,#113155) ;
#94887=AXIS2_PLACEMENT_3D('',#146567,#113158,#113159) ;
#94888=AXIS2_PLACEMENT_3D('',#146573,#113163,#113164) ;
#94889=AXIS2_PLACEMENT_3D('',#146575,#113165,#113166) ;
#94890=AXIS2_PLACEMENT_3D('',#146578,#113168,#113169) ;
#94891=AXIS2_PLACEMENT_3D('',#146579,#113170,#113171) ;
#94892=AXIS2_PLACEMENT_3D('',#146585,#113175,#113176) ;
#94893=AXIS2_PLACEMENT_3D('',#146587,#113177,#113178) ;
#94894=AXIS2_PLACEMENT_3D('',#146590,#113180,#113181) ;
#94895=AXIS2_PLACEMENT_3D('',#146591,#113182,#113183) ;
#94896=AXIS2_PLACEMENT_3D('',#146597,#113187,#113188) ;
#94897=AXIS2_PLACEMENT_3D('',#146599,#113189,#113190) ;
#94898=AXIS2_PLACEMENT_3D('',#146602,#113192,#113193) ;
#94899=AXIS2_PLACEMENT_3D('',#146603,#113194,#113195) ;
#94900=AXIS2_PLACEMENT_3D('',#146609,#113199,#113200) ;
#94901=AXIS2_PLACEMENT_3D('',#146611,#113201,#113202) ;
#94902=AXIS2_PLACEMENT_3D('',#146614,#113204,#113205) ;
#94903=AXIS2_PLACEMENT_3D('',#146615,#113206,#113207) ;
#94904=AXIS2_PLACEMENT_3D('',#146621,#113211,#113212) ;
#94905=AXIS2_PLACEMENT_3D('',#146623,#113213,#113214) ;
#94906=AXIS2_PLACEMENT_3D('',#146626,#113216,#113217) ;
#94907=AXIS2_PLACEMENT_3D('',#146627,#113218,#113219) ;
#94908=AXIS2_PLACEMENT_3D('',#146633,#113223,#113224) ;
#94909=AXIS2_PLACEMENT_3D('',#146635,#113225,#113226) ;
#94910=AXIS2_PLACEMENT_3D('',#146638,#113228,#113229) ;
#94911=AXIS2_PLACEMENT_3D('',#146639,#113230,#113231) ;
#94912=AXIS2_PLACEMENT_3D('',#146641,#113232,#113233) ;
#94913=AXIS2_PLACEMENT_3D('',#146644,#113235,#113236) ;
#94914=AXIS2_PLACEMENT_3D('',#146645,#113237,#113238) ;
#94915=AXIS2_PLACEMENT_3D('',#146647,#113239,#113240) ;
#94916=AXIS2_PLACEMENT_3D('',#146650,#113242,#113243) ;
#94917=AXIS2_PLACEMENT_3D('',#146651,#113244,#113245) ;
#94918=AXIS2_PLACEMENT_3D('',#146657,#113249,#113250) ;
#94919=AXIS2_PLACEMENT_3D('',#146659,#113251,#113252) ;
#94920=AXIS2_PLACEMENT_3D('',#146662,#113254,#113255) ;
#94921=AXIS2_PLACEMENT_3D('',#146663,#113256,#113257) ;
#94922=AXIS2_PLACEMENT_3D('',#146669,#113261,#113262) ;
#94923=AXIS2_PLACEMENT_3D('',#146671,#113263,#113264) ;
#94924=AXIS2_PLACEMENT_3D('',#146674,#113266,#113267) ;
#94925=AXIS2_PLACEMENT_3D('',#146675,#113268,#113269) ;
#94926=AXIS2_PLACEMENT_3D('',#146678,#113272,#113273) ;
#94927=AXIS2_PLACEMENT_3D('',#146681,#113274,#113275) ;
#94928=AXIS2_PLACEMENT_3D('',#146685,#113277,#113278) ;
#94929=AXIS2_PLACEMENT_3D('',#146693,#113282,#113283) ;
#94930=AXIS2_PLACEMENT_3D('',#146701,#113287,#113288) ;
#94931=AXIS2_PLACEMENT_3D('',#146705,#113290,#113291) ;
#94932=AXIS2_PLACEMENT_3D('',#146714,#113297,#113298) ;
#94933=AXIS2_PLACEMENT_3D('',#146719,#113300,#113301) ;
#94934=AXIS2_PLACEMENT_3D('',#146722,#113303,#113304) ;
#94935=AXIS2_PLACEMENT_3D('',#146723,#113305,#113306) ;
#94936=AXIS2_PLACEMENT_3D('',#146729,#113310,#113311) ;
#94937=AXIS2_PLACEMENT_3D('',#146731,#113312,#113313) ;
#94938=AXIS2_PLACEMENT_3D('',#146734,#113315,#113316) ;
#94939=AXIS2_PLACEMENT_3D('',#146735,#113317,#113318) ;
#94940=AXIS2_PLACEMENT_3D('',#146741,#113322,#113323) ;
#94941=AXIS2_PLACEMENT_3D('',#146743,#113324,#113325) ;
#94942=AXIS2_PLACEMENT_3D('',#146746,#113327,#113328) ;
#94943=AXIS2_PLACEMENT_3D('',#146747,#113329,#113330) ;
#94944=AXIS2_PLACEMENT_3D('',#146752,#113334,#113335) ;
#94945=AXIS2_PLACEMENT_3D('',#146755,#113337,#113338) ;
#94946=AXIS2_PLACEMENT_3D('',#146756,#113339,#113340) ;
#94947=AXIS2_PLACEMENT_3D('',#146759,#113343,#113344) ;
#94948=AXIS2_PLACEMENT_3D('',#146765,#113348,#113349) ;
#94949=AXIS2_PLACEMENT_3D('',#146767,#113350,#113351) ;
#94950=AXIS2_PLACEMENT_3D('',#146770,#113353,#113354) ;
#94951=AXIS2_PLACEMENT_3D('',#146771,#113355,#113356) ;
#94952=AXIS2_PLACEMENT_3D('',#146777,#113360,#113361) ;
#94953=AXIS2_PLACEMENT_3D('',#146779,#113362,#113363) ;
#94954=AXIS2_PLACEMENT_3D('',#146782,#113365,#113366) ;
#94955=AXIS2_PLACEMENT_3D('',#146783,#113367,#113368) ;
#94956=AXIS2_PLACEMENT_3D('',#146789,#113372,#113373) ;
#94957=AXIS2_PLACEMENT_3D('',#146791,#113374,#113375) ;
#94958=AXIS2_PLACEMENT_3D('',#146794,#113377,#113378) ;
#94959=AXIS2_PLACEMENT_3D('',#146795,#113379,#113380) ;
#94960=AXIS2_PLACEMENT_3D('',#146801,#113384,#113385) ;
#94961=AXIS2_PLACEMENT_3D('',#146803,#113386,#113387) ;
#94962=AXIS2_PLACEMENT_3D('',#146806,#113389,#113390) ;
#94963=AXIS2_PLACEMENT_3D('',#146807,#113391,#113392) ;
#94964=AXIS2_PLACEMENT_3D('',#146813,#113396,#113397) ;
#94965=AXIS2_PLACEMENT_3D('',#146815,#113398,#113399) ;
#94966=AXIS2_PLACEMENT_3D('',#146818,#113401,#113402) ;
#94967=AXIS2_PLACEMENT_3D('',#146819,#113403,#113404) ;
#94968=AXIS2_PLACEMENT_3D('',#146825,#113408,#113409) ;
#94969=AXIS2_PLACEMENT_3D('',#146827,#113410,#113411) ;
#94970=AXIS2_PLACEMENT_3D('',#146830,#113413,#113414) ;
#94971=AXIS2_PLACEMENT_3D('',#146831,#113415,#113416) ;
#94972=AXIS2_PLACEMENT_3D('',#146833,#113417,#113418) ;
#94973=AXIS2_PLACEMENT_3D('',#146836,#113420,#113421) ;
#94974=AXIS2_PLACEMENT_3D('',#146837,#113422,#113423) ;
#94975=AXIS2_PLACEMENT_3D('',#146839,#113424,#113425) ;
#94976=AXIS2_PLACEMENT_3D('',#146842,#113427,#113428) ;
#94977=AXIS2_PLACEMENT_3D('',#146843,#113429,#113430) ;
#94978=AXIS2_PLACEMENT_3D('',#146849,#113434,#113435) ;
#94979=AXIS2_PLACEMENT_3D('',#146851,#113436,#113437) ;
#94980=AXIS2_PLACEMENT_3D('',#146854,#113439,#113440) ;
#94981=AXIS2_PLACEMENT_3D('',#146855,#113441,#113442) ;
#94982=AXIS2_PLACEMENT_3D('',#146861,#113446,#113447) ;
#94983=AXIS2_PLACEMENT_3D('',#146863,#113448,#113449) ;
#94984=AXIS2_PLACEMENT_3D('',#146866,#113451,#113452) ;
#94985=AXIS2_PLACEMENT_3D('',#146867,#113453,#113454) ;
#94986=AXIS2_PLACEMENT_3D('',#146870,#113457,#113458) ;
#94987=AXIS2_PLACEMENT_3D('',#146873,#113459,#113460) ;
#94988=AXIS2_PLACEMENT_3D('',#146877,#113462,#113463) ;
#94989=AXIS2_PLACEMENT_3D('',#146885,#113467,#113468) ;
#94990=AXIS2_PLACEMENT_3D('',#146893,#113472,#113473) ;
#94991=AXIS2_PLACEMENT_3D('',#146897,#113475,#113476) ;
#94992=AXIS2_PLACEMENT_3D('',#146906,#113482,#113483) ;
#94993=AXIS2_PLACEMENT_3D('',#146911,#113485,#113486) ;
#94994=AXIS2_PLACEMENT_3D('',#146915,#113488,#113489) ;
#94995=AXIS2_PLACEMENT_3D('',#146919,#113491,#113492) ;
#94996=AXIS2_PLACEMENT_3D('',#146922,#113494,#113495) ;
#94997=AXIS2_PLACEMENT_3D('',#146923,#113496,#113497) ;
#94998=AXIS2_PLACEMENT_3D('',#146928,#113499,#113500) ;
#94999=AXIS2_PLACEMENT_3D('',#146932,#113502,#113503) ;
#95000=AXIS2_PLACEMENT_3D('',#146936,#113505,#113506) ;
#95001=AXIS2_PLACEMENT_3D('',#146939,#113508,#113509) ;
#95002=AXIS2_PLACEMENT_3D('',#146940,#113510,#113511) ;
#95003=AXIS2_PLACEMENT_3D('',#146945,#113513,#113514) ;
#95004=AXIS2_PLACEMENT_3D('',#146949,#113516,#113517) ;
#95005=AXIS2_PLACEMENT_3D('',#146953,#113519,#113520) ;
#95006=AXIS2_PLACEMENT_3D('',#146956,#113522,#113523) ;
#95007=AXIS2_PLACEMENT_3D('',#146957,#113524,#113525) ;
#95008=AXIS2_PLACEMENT_3D('',#146962,#113527,#113528) ;
#95009=AXIS2_PLACEMENT_3D('',#146966,#113530,#113531) ;
#95010=AXIS2_PLACEMENT_3D('',#146970,#113533,#113534) ;
#95011=AXIS2_PLACEMENT_3D('',#146973,#113536,#113537) ;
#95012=AXIS2_PLACEMENT_3D('',#146974,#113538,#113539) ;
#95013=AXIS2_PLACEMENT_3D('',#146979,#113541,#113542) ;
#95014=AXIS2_PLACEMENT_3D('',#146983,#113544,#113545) ;
#95015=AXIS2_PLACEMENT_3D('',#146987,#113547,#113548) ;
#95016=AXIS2_PLACEMENT_3D('',#146990,#113550,#113551) ;
#95017=AXIS2_PLACEMENT_3D('',#146991,#113552,#113553) ;
#95018=AXIS2_PLACEMENT_3D('',#146996,#113555,#113556) ;
#95019=AXIS2_PLACEMENT_3D('',#147000,#113558,#113559) ;
#95020=AXIS2_PLACEMENT_3D('',#147004,#113561,#113562) ;
#95021=AXIS2_PLACEMENT_3D('',#147007,#113564,#113565) ;
#95022=AXIS2_PLACEMENT_3D('',#147008,#113566,#113567) ;
#95023=AXIS2_PLACEMENT_3D('',#147013,#113569,#113570) ;
#95024=AXIS2_PLACEMENT_3D('',#147017,#113572,#113573) ;
#95025=AXIS2_PLACEMENT_3D('',#147021,#113575,#113576) ;
#95026=AXIS2_PLACEMENT_3D('',#147024,#113578,#113579) ;
#95027=AXIS2_PLACEMENT_3D('',#147025,#113580,#113581) ;
#95028=AXIS2_PLACEMENT_3D('',#147030,#113583,#113584) ;
#95029=AXIS2_PLACEMENT_3D('',#147034,#113586,#113587) ;
#95030=AXIS2_PLACEMENT_3D('',#147038,#113589,#113590) ;
#95031=AXIS2_PLACEMENT_3D('',#147041,#113592,#113593) ;
#95032=AXIS2_PLACEMENT_3D('',#147042,#113594,#113595) ;
#95033=AXIS2_PLACEMENT_3D('',#147047,#113597,#113598) ;
#95034=AXIS2_PLACEMENT_3D('',#147051,#113600,#113601) ;
#95035=AXIS2_PLACEMENT_3D('',#147055,#113603,#113604) ;
#95036=AXIS2_PLACEMENT_3D('',#147058,#113606,#113607) ;
#95037=AXIS2_PLACEMENT_3D('',#147059,#113608,#113609) ;
#95038=AXIS2_PLACEMENT_3D('',#147060,#113610,#113611) ;
#95039=AXIS2_PLACEMENT_3D('',#147061,#113612,#113613) ;
#95040=AXIS2_PLACEMENT_3D('',#147062,#113614,#113615) ;
#95041=AXIS2_PLACEMENT_3D('',#147063,#113616,#113617) ;
#95042=AXIS2_PLACEMENT_3D('',#147064,#113618,#113619) ;
#95043=AXIS2_PLACEMENT_3D('',#147065,#113620,#113621) ;
#95044=AXIS2_PLACEMENT_3D('',#147067,#113622,#113623) ;
#95045=AXIS2_PLACEMENT_3D('',#147068,#113624,#113625) ;
#95046=AXIS2_PLACEMENT_3D('',#147069,#113626,#113627) ;
#95047=AXIS2_PLACEMENT_3D('',#147070,#113628,#113629) ;
#95048=AXIS2_PLACEMENT_3D('',#147071,#113630,#113631) ;
#95049=AXIS2_PLACEMENT_3D('',#147072,#113632,#113633) ;
#95050=AXIS2_PLACEMENT_3D('',#147073,#113634,#113635) ;
#95051=AXIS2_PLACEMENT_3D('',#147074,#113636,#113637) ;
#95052=AXIS2_PLACEMENT_3D('',#147075,#113638,#113639) ;
#95053=AXIS2_PLACEMENT_3D('',#147086,#113641,#113642) ;
#95054=AXIS2_PLACEMENT_3D('',#147143,#113644,#113645) ;
#95055=AXIS2_PLACEMENT_3D('',#147144,#113646,#113647) ;
#95056=AXIS2_PLACEMENT_3D('',#147145,#113648,#113649) ;
#95057=AXIS2_PLACEMENT_3D('',#147146,#113650,#113651) ;
#95058=AXIS2_PLACEMENT_3D('',#147147,#113652,#113653) ;
#95059=AXIS2_PLACEMENT_3D('',#147148,#113654,#113655) ;
#95060=AXIS2_PLACEMENT_3D('',#147149,#113656,#113657) ;
#95061=AXIS2_PLACEMENT_3D('',#147150,#113658,#113659) ;
#95062=AXIS2_PLACEMENT_3D('',#147151,#113660,#113661) ;
#95063=AXIS2_PLACEMENT_3D('',#147152,#113662,#113663) ;
#95064=AXIS2_PLACEMENT_3D('',#147153,#113664,#113665) ;
#95065=AXIS2_PLACEMENT_3D('',#147154,#113666,#113667) ;
#95066=AXIS2_PLACEMENT_3D('',#147155,#113668,#113669) ;
#95067=AXIS2_PLACEMENT_3D('',#147156,#113670,#113671) ;
#95068=AXIS2_PLACEMENT_3D('',#147157,#113672,#113673) ;
#95069=AXIS2_PLACEMENT_3D('',#147158,#113674,#113675) ;
#95070=AXIS2_PLACEMENT_3D('',#147159,#113676,#113677) ;
#95071=AXIS2_PLACEMENT_3D('',#147160,#113678,#113679) ;
#95072=AXIS2_PLACEMENT_3D('',#147161,#113680,#113681) ;
#95073=AXIS2_PLACEMENT_3D('',#147162,#113682,#113683) ;
#95074=AXIS2_PLACEMENT_3D('',#147163,#113684,#113685) ;
#95075=AXIS2_PLACEMENT_3D('',#147164,#113686,#113687) ;
#95076=AXIS2_PLACEMENT_3D('',#147165,#113688,#113689) ;
#95077=AXIS2_PLACEMENT_3D('',#147168,#113691,#113692) ;
#95078=AXIS2_PLACEMENT_3D('',#147169,#113693,#113694) ;
#95079=AXIS2_PLACEMENT_3D('',#147170,#113695,#113696) ;
#95080=AXIS2_PLACEMENT_3D('',#147171,#113697,#113698) ;
#95081=AXIS2_PLACEMENT_3D('',#147172,#113699,#113700) ;
#95082=AXIS2_PLACEMENT_3D('',#147173,#113701,#113702) ;
#95083=AXIS2_PLACEMENT_3D('',#147174,#113703,#113704) ;
#95084=AXIS2_PLACEMENT_3D('',#147175,#113705,#113706) ;
#95085=AXIS2_PLACEMENT_3D('',#147176,#113707,#113708) ;
#95086=AXIS2_PLACEMENT_3D('',#147177,#113709,#113710) ;
#95087=AXIS2_PLACEMENT_3D('',#147178,#113711,#113712) ;
#95088=AXIS2_PLACEMENT_3D('',#147179,#113713,#113714) ;
#95089=AXIS2_PLACEMENT_3D('',#147180,#113715,#113716) ;
#95090=AXIS2_PLACEMENT_3D('',#147181,#113717,#113718) ;
#95091=AXIS2_PLACEMENT_3D('',#147182,#113719,#113720) ;
#95092=AXIS2_PLACEMENT_3D('',#147183,#113721,#113722) ;
#95093=AXIS2_PLACEMENT_3D('',#147185,#113723,#113724) ;
#95094=AXIS2_PLACEMENT_3D('',#147186,#113725,#113726) ;
#95095=AXIS2_PLACEMENT_3D('',#147187,#113727,#113728) ;
#95096=AXIS2_PLACEMENT_3D('',#147188,#113729,#113730) ;
#95097=AXIS2_PLACEMENT_3D('',#147189,#113731,#113732) ;
#95098=AXIS2_PLACEMENT_3D('',#147190,#113733,#113734) ;
#95099=AXIS2_PLACEMENT_3D('',#147191,#113735,#113736) ;
#95100=AXIS2_PLACEMENT_3D('',#147192,#113737,#113738) ;
#95101=AXIS2_PLACEMENT_3D('',#147193,#113739,#113740) ;
#95102=AXIS2_PLACEMENT_3D('',#147194,#113741,#113742) ;
#95103=AXIS2_PLACEMENT_3D('',#147195,#113743,#113744) ;
#95104=AXIS2_PLACEMENT_3D('',#147196,#113745,#113746) ;
#95105=AXIS2_PLACEMENT_3D('',#147197,#113747,#113748) ;
#95106=AXIS2_PLACEMENT_3D('',#147200,#113750,#113751) ;
#95107=AXIS2_PLACEMENT_3D('',#147201,#113752,#113753) ;
#95108=AXIS2_PLACEMENT_3D('',#147202,#113754,#113755) ;
#95109=AXIS2_PLACEMENT_3D('',#147203,#113756,#113757) ;
#95110=AXIS2_PLACEMENT_3D('',#147204,#113758,#113759) ;
#95111=AXIS2_PLACEMENT_3D('',#147205,#113760,#113761) ;
#95112=AXIS2_PLACEMENT_3D('',#147206,#113762,#113763) ;
#95113=AXIS2_PLACEMENT_3D('',#147207,#113764,#113765) ;
#95114=AXIS2_PLACEMENT_3D('',#147208,#113766,#113767) ;
#95115=AXIS2_PLACEMENT_3D('',#147209,#113768,#113769) ;
#95116=AXIS2_PLACEMENT_3D('',#147210,#113770,#113771) ;
#95117=AXIS2_PLACEMENT_3D('',#147211,#113772,#113773) ;
#95118=AXIS2_PLACEMENT_3D('',#147212,#113774,#113775) ;
#95119=AXIS2_PLACEMENT_3D('',#147214,#113776,#113777) ;
#95120=AXIS2_PLACEMENT_3D('',#147215,#113778,#113779) ;
#95121=AXIS2_PLACEMENT_3D('',#147216,#113780,#113781) ;
#95122=AXIS2_PLACEMENT_3D('',#147217,#113782,#113783) ;
#95123=AXIS2_PLACEMENT_3D('',#147218,#113784,#113785) ;
#95124=AXIS2_PLACEMENT_3D('',#147219,#113786,#113787) ;
#95125=AXIS2_PLACEMENT_3D('',#147220,#113788,#113789) ;
#95126=AXIS2_PLACEMENT_3D('',#147221,#113790,#113791) ;
#95127=AXIS2_PLACEMENT_3D('',#147222,#113792,#113793) ;
#95128=AXIS2_PLACEMENT_3D('',#147223,#113794,#113795) ;
#95129=AXIS2_PLACEMENT_3D('',#147224,#113796,#113797) ;
#95130=AXIS2_PLACEMENT_3D('',#147226,#113799,#113800) ;
#95131=AXIS2_PLACEMENT_3D('',#147227,#113801,#113802) ;
#95132=AXIS2_PLACEMENT_3D('',#147228,#113803,#113804) ;
#95133=AXIS2_PLACEMENT_3D('',#147229,#113805,#113806) ;
#95134=AXIS2_PLACEMENT_3D('',#147230,#113807,#113808) ;
#95135=AXIS2_PLACEMENT_3D('',#147231,#113809,#113810) ;
#95136=AXIS2_PLACEMENT_3D('',#147232,#113811,#113812) ;
#95137=AXIS2_PLACEMENT_3D('',#147233,#113813,#113814) ;
#95138=AXIS2_PLACEMENT_3D('',#147234,#113815,#113816) ;
#95139=AXIS2_PLACEMENT_3D('',#147235,#113817,#113818) ;
#95140=AXIS2_PLACEMENT_3D('',#147236,#113819,#113820) ;
#95141=AXIS2_PLACEMENT_3D('',#147237,#113821,#113822) ;
#95142=AXIS2_PLACEMENT_3D('',#147238,#113823,#113824) ;
#95143=AXIS2_PLACEMENT_3D('',#147239,#113825,#113826) ;
#95144=AXIS2_PLACEMENT_3D('',#147240,#113827,#113828) ;
#95145=AXIS2_PLACEMENT_3D('',#147241,#113829,#113830) ;
#95146=AXIS2_PLACEMENT_3D('',#147242,#113831,#113832) ;
#95147=AXIS2_PLACEMENT_3D('',#147243,#113833,#113834) ;
#95148=AXIS2_PLACEMENT_3D('',#147244,#113835,#113836) ;
#95149=AXIS2_PLACEMENT_3D('',#147245,#113837,#113838) ;
#95150=AXIS2_PLACEMENT_3D('',#147246,#113839,#113840) ;
#95151=AXIS2_PLACEMENT_3D('',#147247,#113841,#113842) ;
#95152=AXIS2_PLACEMENT_3D('',#147248,#113843,#113844) ;
#95153=AXIS2_PLACEMENT_3D('',#147249,#113845,#113846) ;
#95154=AXIS2_PLACEMENT_3D('',#147250,#113847,#113848) ;
#95155=AXIS2_PLACEMENT_3D('',#147251,#113849,#113850) ;
#95156=AXIS2_PLACEMENT_3D('',#147252,#113851,#113852) ;
#95157=AXIS2_PLACEMENT_3D('',#147253,#113853,#113854) ;
#95158=AXIS2_PLACEMENT_3D('',#147254,#113855,#113856) ;
#95159=AXIS2_PLACEMENT_3D('',#147255,#113857,#113858) ;
#95160=AXIS2_PLACEMENT_3D('',#147256,#113859,#113860) ;
#95161=AXIS2_PLACEMENT_3D('',#147257,#113861,#113862) ;
#95162=AXIS2_PLACEMENT_3D('',#147258,#113863,#113864) ;
#95163=AXIS2_PLACEMENT_3D('',#147259,#113865,#113866) ;
#95164=AXIS2_PLACEMENT_3D('',#147260,#113867,#113868) ;
#95165=AXIS2_PLACEMENT_3D('',#147261,#113869,#113870) ;
#95166=AXIS2_PLACEMENT_3D('',#147262,#113871,#113872) ;
#95167=AXIS2_PLACEMENT_3D('',#147263,#113873,#113874) ;
#95168=AXIS2_PLACEMENT_3D('',#147264,#113875,#113876) ;
#95169=AXIS2_PLACEMENT_3D('',#147265,#113877,#113878) ;
#95170=AXIS2_PLACEMENT_3D('',#147266,#113879,#113880) ;
#95171=AXIS2_PLACEMENT_3D('',#147267,#113881,#113882) ;
#95172=AXIS2_PLACEMENT_3D('',#147268,#113883,#113884) ;
#95173=AXIS2_PLACEMENT_3D('',#147269,#113885,#113886) ;
#95174=AXIS2_PLACEMENT_3D('',#147270,#113887,#113888) ;
#95175=AXIS2_PLACEMENT_3D('',#147271,#113889,#113890) ;
#95176=AXIS2_PLACEMENT_3D('',#147272,#113891,#113892) ;
#95177=AXIS2_PLACEMENT_3D('',#147273,#113893,#113894) ;
#95178=AXIS2_PLACEMENT_3D('',#147274,#113895,#113896) ;
#95179=AXIS2_PLACEMENT_3D('',#147275,#113897,#113898) ;
#95180=AXIS2_PLACEMENT_3D('',#147276,#113899,#113900) ;
#95181=AXIS2_PLACEMENT_3D('',#147277,#113901,#113902) ;
#95182=AXIS2_PLACEMENT_3D('',#147278,#113903,#113904) ;
#95183=AXIS2_PLACEMENT_3D('',#147279,#113905,#113906) ;
#95184=AXIS2_PLACEMENT_3D('',#147280,#113907,#113908) ;
#95185=AXIS2_PLACEMENT_3D('',#147281,#113909,#113910) ;
#95186=AXIS2_PLACEMENT_3D('',#147282,#113911,#113912) ;
#95187=AXIS2_PLACEMENT_3D('',#147283,#113913,#113914) ;
#95188=AXIS2_PLACEMENT_3D('',#147284,#113915,#113916) ;
#95189=AXIS2_PLACEMENT_3D('',#147285,#113917,#113918) ;
#95190=AXIS2_PLACEMENT_3D('',#147286,#113919,#113920) ;
#95191=AXIS2_PLACEMENT_3D('',#147287,#113921,#113922) ;
#95192=AXIS2_PLACEMENT_3D('',#147288,#113923,#113924) ;
#95193=AXIS2_PLACEMENT_3D('',#147289,#113925,#113926) ;
#95194=AXIS2_PLACEMENT_3D('',#147290,#113927,#113928) ;
#95195=AXIS2_PLACEMENT_3D('',#147291,#113929,#113930) ;
#95196=AXIS2_PLACEMENT_3D('',#147292,#113931,#113932) ;
#95197=AXIS2_PLACEMENT_3D('',#147293,#113933,#113934) ;
#95198=AXIS2_PLACEMENT_3D('',#147294,#113935,#113936) ;
#95199=AXIS2_PLACEMENT_3D('',#147295,#113937,#113938) ;
#95200=AXIS2_PLACEMENT_3D('',#147296,#113939,#113940) ;
#95201=AXIS2_PLACEMENT_3D('',#147297,#113941,#113942) ;
#95202=AXIS2_PLACEMENT_3D('',#147298,#113943,#113944) ;
#95203=AXIS2_PLACEMENT_3D('',#147299,#113945,#113946) ;
#95204=AXIS2_PLACEMENT_3D('',#147300,#113947,#113948) ;
#95205=AXIS2_PLACEMENT_3D('',#147301,#113949,#113950) ;
#95206=AXIS2_PLACEMENT_3D('',#147302,#113951,#113952) ;
#95207=AXIS2_PLACEMENT_3D('',#147303,#113953,#113954) ;
#95208=AXIS2_PLACEMENT_3D('',#147304,#113955,#113956) ;
#95209=AXIS2_PLACEMENT_3D('',#147305,#113957,#113958) ;
#95210=AXIS2_PLACEMENT_3D('',#147306,#113959,#113960) ;
#95211=AXIS2_PLACEMENT_3D('',#147307,#113961,#113962) ;
#95212=AXIS2_PLACEMENT_3D('',#147308,#113963,#113964) ;
#95213=AXIS2_PLACEMENT_3D('',#147309,#113965,#113966) ;
#95214=AXIS2_PLACEMENT_3D('',#147310,#113967,#113968) ;
#95215=AXIS2_PLACEMENT_3D('',#147311,#113969,#113970) ;
#95216=AXIS2_PLACEMENT_3D('',#147312,#113971,#113972) ;
#95217=AXIS2_PLACEMENT_3D('',#147313,#113973,#113974) ;
#95218=AXIS2_PLACEMENT_3D('',#147314,#113975,#113976) ;
#95219=AXIS2_PLACEMENT_3D('',#147315,#113977,#113978) ;
#95220=AXIS2_PLACEMENT_3D('',#147316,#113979,#113980) ;
#95221=AXIS2_PLACEMENT_3D('',#147317,#113981,#113982) ;
#95222=AXIS2_PLACEMENT_3D('',#147318,#113983,#113984) ;
#95223=AXIS2_PLACEMENT_3D('',#147319,#113985,#113986) ;
#95224=AXIS2_PLACEMENT_3D('',#147320,#113987,#113988) ;
#95225=AXIS2_PLACEMENT_3D('',#147321,#113989,#113990) ;
#95226=AXIS2_PLACEMENT_3D('',#147322,#113991,#113992) ;
#95227=AXIS2_PLACEMENT_3D('',#147323,#113993,#113994) ;
#95228=AXIS2_PLACEMENT_3D('',#147324,#113995,#113996) ;
#95229=AXIS2_PLACEMENT_3D('',#147325,#113997,#113998) ;
#95230=AXIS2_PLACEMENT_3D('',#147326,#113999,#114000) ;
#95231=AXIS2_PLACEMENT_3D('',#147327,#114001,#114002) ;
#95232=AXIS2_PLACEMENT_3D('',#147328,#114003,#114004) ;
#95233=AXIS2_PLACEMENT_3D('',#147329,#114005,#114006) ;
#95234=AXIS2_PLACEMENT_3D('',#147330,#114007,#114008) ;
#95235=AXIS2_PLACEMENT_3D('',#147331,#114009,#114010) ;
#95236=AXIS2_PLACEMENT_3D('',#147332,#114011,#114012) ;
#95237=AXIS2_PLACEMENT_3D('',#147333,#114013,#114014) ;
#95238=AXIS2_PLACEMENT_3D('',#147334,#114015,#114016) ;
#95239=AXIS2_PLACEMENT_3D('',#147335,#114017,#114018) ;
#95240=AXIS2_PLACEMENT_3D('',#147336,#114019,#114020) ;
#95241=AXIS2_PLACEMENT_3D('',#147337,#114021,#114022) ;
#95242=AXIS2_PLACEMENT_3D('',#147338,#114023,#114024) ;
#95243=AXIS2_PLACEMENT_3D('',#147339,#114025,#114026) ;
#95244=AXIS2_PLACEMENT_3D('',#147340,#114027,#114028) ;
#95245=AXIS2_PLACEMENT_3D('',#147341,#114029,#114030) ;
#95246=AXIS2_PLACEMENT_3D('',#147342,#114031,#114032) ;
#95247=AXIS2_PLACEMENT_3D('',#147343,#114033,#114034) ;
#95248=AXIS2_PLACEMENT_3D('',#147344,#114035,#114036) ;
#95249=AXIS2_PLACEMENT_3D('',#147345,#114037,#114038) ;
#95250=AXIS2_PLACEMENT_3D('',#147346,#114039,#114040) ;
#95251=AXIS2_PLACEMENT_3D('',#147347,#114041,#114042) ;
#95252=AXIS2_PLACEMENT_3D('',#147348,#114043,#114044) ;
#95253=AXIS2_PLACEMENT_3D('',#147349,#114045,#114046) ;
#95254=AXIS2_PLACEMENT_3D('',#147350,#114047,#114048) ;
#95255=AXIS2_PLACEMENT_3D('',#147351,#114049,#114050) ;
#95256=AXIS2_PLACEMENT_3D('',#147352,#114051,#114052) ;
#95257=AXIS2_PLACEMENT_3D('',#147353,#114053,#114054) ;
#95258=AXIS2_PLACEMENT_3D('',#147354,#114055,#114056) ;
#95259=AXIS2_PLACEMENT_3D('',#147355,#114057,#114058) ;
#95260=AXIS2_PLACEMENT_3D('',#147356,#114059,#114060) ;
#95261=AXIS2_PLACEMENT_3D('',#147357,#114061,#114062) ;
#95262=AXIS2_PLACEMENT_3D('',#147358,#114063,#114064) ;
#95263=AXIS2_PLACEMENT_3D('',#147359,#114065,#114066) ;
#95264=AXIS2_PLACEMENT_3D('',#147360,#114067,#114068) ;
#95265=AXIS2_PLACEMENT_3D('',#147361,#114069,#114070) ;
#95266=AXIS2_PLACEMENT_3D('',#147362,#114071,#114072) ;
#95267=AXIS2_PLACEMENT_3D('',#147363,#114073,#114074) ;
#95268=AXIS2_PLACEMENT_3D('',#147364,#114075,#114076) ;
#95269=AXIS2_PLACEMENT_3D('',#147365,#114077,#114078) ;
#95270=AXIS2_PLACEMENT_3D('',#147366,#114079,#114080) ;
#95271=AXIS2_PLACEMENT_3D('',#147367,#114081,#114082) ;
#95272=AXIS2_PLACEMENT_3D('',#147368,#114083,#114084) ;
#95273=AXIS2_PLACEMENT_3D('',#147369,#114085,#114086) ;
#95274=AXIS2_PLACEMENT_3D('',#147370,#114087,#114088) ;
#95275=AXIS2_PLACEMENT_3D('',#147371,#114089,#114090) ;
#95276=AXIS2_PLACEMENT_3D('',#147372,#114091,#114092) ;
#95277=AXIS2_PLACEMENT_3D('',#147373,#114093,#114094) ;
#95278=AXIS2_PLACEMENT_3D('',#147374,#114095,#114096) ;
#95279=AXIS2_PLACEMENT_3D('',#147375,#114097,#114098) ;
#95280=AXIS2_PLACEMENT_3D('',#147376,#114099,#114100) ;
#95281=AXIS2_PLACEMENT_3D('',#147377,#114101,#114102) ;
#95282=AXIS2_PLACEMENT_3D('',#147378,#114103,#114104) ;
#95283=AXIS2_PLACEMENT_3D('',#147379,#114105,#114106) ;
#95284=AXIS2_PLACEMENT_3D('',#147380,#114107,#114108) ;
#95285=AXIS2_PLACEMENT_3D('',#147381,#114109,#114110) ;
#95286=AXIS2_PLACEMENT_3D('',#147382,#114111,#114112) ;
#95287=AXIS2_PLACEMENT_3D('',#147383,#114113,#114114) ;
#95288=AXIS2_PLACEMENT_3D('',#147384,#114115,#114116) ;
#95289=AXIS2_PLACEMENT_3D('',#147385,#114117,#114118) ;
#95290=AXIS2_PLACEMENT_3D('',#147386,#114119,#114120) ;
#95291=AXIS2_PLACEMENT_3D('',#147387,#114121,#114122) ;
#95292=AXIS2_PLACEMENT_3D('',#147388,#114123,#114124) ;
#95293=AXIS2_PLACEMENT_3D('',#147389,#114125,#114126) ;
#95294=AXIS2_PLACEMENT_3D('',#147390,#114127,#114128) ;
#95295=AXIS2_PLACEMENT_3D('',#147391,#114129,#114130) ;
#95296=AXIS2_PLACEMENT_3D('',#147392,#114131,#114132) ;
#95297=AXIS2_PLACEMENT_3D('',#147393,#114133,#114134) ;
#95298=AXIS2_PLACEMENT_3D('',#147394,#114135,#114136) ;
#95299=AXIS2_PLACEMENT_3D('',#147395,#114137,#114138) ;
#95300=AXIS2_PLACEMENT_3D('',#147396,#114139,#114140) ;
#95301=AXIS2_PLACEMENT_3D('',#147397,#114141,#114142) ;
#95302=AXIS2_PLACEMENT_3D('',#147398,#114143,#114144) ;
#95303=AXIS2_PLACEMENT_3D('',#147399,#114145,#114146) ;
#95304=AXIS2_PLACEMENT_3D('',#147400,#114147,#114148) ;
#95305=AXIS2_PLACEMENT_3D('',#147401,#114149,#114150) ;
#95306=AXIS2_PLACEMENT_3D('',#147402,#114151,#114152) ;
#95307=AXIS2_PLACEMENT_3D('',#147403,#114153,#114154) ;
#95308=AXIS2_PLACEMENT_3D('',#147404,#114155,#114156) ;
#95309=AXIS2_PLACEMENT_3D('',#147405,#114157,#114158) ;
#95310=AXIS2_PLACEMENT_3D('',#147406,#114159,#114160) ;
#95311=AXIS2_PLACEMENT_3D('',#147407,#114161,#114162) ;
#95312=AXIS2_PLACEMENT_3D('',#147408,#114163,#114164) ;
#95313=AXIS2_PLACEMENT_3D('',#147409,#114165,#114166) ;
#95314=AXIS2_PLACEMENT_3D('',#147410,#114167,#114168) ;
#95315=AXIS2_PLACEMENT_3D('',#147411,#114169,#114170) ;
#95316=AXIS2_PLACEMENT_3D('',#147412,#114171,#114172) ;
#95317=AXIS2_PLACEMENT_3D('',#147413,#114173,#114174) ;
#95318=AXIS2_PLACEMENT_3D('',#147414,#114175,#114176) ;
#95319=AXIS2_PLACEMENT_3D('',#147415,#114177,#114178) ;
#95320=AXIS2_PLACEMENT_3D('',#147416,#114179,#114180) ;
#95321=AXIS2_PLACEMENT_3D('',#147417,#114181,#114182) ;
#95322=AXIS2_PLACEMENT_3D('',#147418,#114183,#114184) ;
#95323=AXIS2_PLACEMENT_3D('',#147419,#114185,#114186) ;
#95324=AXIS2_PLACEMENT_3D('',#147420,#114187,#114188) ;
#95325=AXIS2_PLACEMENT_3D('',#147421,#114189,#114190) ;
#95326=AXIS2_PLACEMENT_3D('',#147422,#114191,#114192) ;
#95327=AXIS2_PLACEMENT_3D('',#147423,#114193,#114194) ;
#95328=AXIS2_PLACEMENT_3D('',#147424,#114195,#114196) ;
#95329=AXIS2_PLACEMENT_3D('',#147425,#114197,#114198) ;
#95330=AXIS2_PLACEMENT_3D('',#147426,#114199,#114200) ;
#95331=AXIS2_PLACEMENT_3D('',#147427,#114201,#114202) ;
#95332=AXIS2_PLACEMENT_3D('',#147428,#114203,#114204) ;
#95333=AXIS2_PLACEMENT_3D('',#147429,#114205,#114206) ;
#95334=AXIS2_PLACEMENT_3D('',#147430,#114207,#114208) ;
#95335=AXIS2_PLACEMENT_3D('',#147431,#114209,#114210) ;
#95336=AXIS2_PLACEMENT_3D('',#147432,#114211,#114212) ;
#95337=AXIS2_PLACEMENT_3D('',#147433,#114213,#114214) ;
#95338=AXIS2_PLACEMENT_3D('',#147434,#114215,#114216) ;
#95339=AXIS2_PLACEMENT_3D('',#147435,#114217,#114218) ;
#95340=AXIS2_PLACEMENT_3D('',#147436,#114219,#114220) ;
#95341=AXIS2_PLACEMENT_3D('',#147437,#114221,#114222) ;
#95342=AXIS2_PLACEMENT_3D('',#147438,#114223,#114224) ;
#95343=AXIS2_PLACEMENT_3D('',#147439,#114225,#114226) ;
#95344=AXIS2_PLACEMENT_3D('',#147440,#114227,#114228) ;
#95345=AXIS2_PLACEMENT_3D('',#147441,#114229,#114230) ;
#95346=AXIS2_PLACEMENT_3D('',#147442,#114231,#114232) ;
#95347=AXIS2_PLACEMENT_3D('',#147443,#114233,#114234) ;
#95348=AXIS2_PLACEMENT_3D('',#147444,#114235,#114236) ;
#95349=AXIS2_PLACEMENT_3D('',#147445,#114237,#114238) ;
#95350=AXIS2_PLACEMENT_3D('',#147446,#114239,#114240) ;
#95351=AXIS2_PLACEMENT_3D('',#147447,#114241,#114242) ;
#95352=AXIS2_PLACEMENT_3D('',#147448,#114243,#114244) ;
#95353=AXIS2_PLACEMENT_3D('',#147449,#114245,#114246) ;
#95354=AXIS2_PLACEMENT_3D('',#147450,#114247,#114248) ;
#95355=AXIS2_PLACEMENT_3D('',#147451,#114249,#114250) ;
#95356=AXIS2_PLACEMENT_3D('',#147452,#114251,#114252) ;
#95357=AXIS2_PLACEMENT_3D('',#147453,#114253,#114254) ;
#95358=AXIS2_PLACEMENT_3D('',#147454,#114255,#114256) ;
#95359=AXIS2_PLACEMENT_3D('',#147455,#114257,#114258) ;
#95360=AXIS2_PLACEMENT_3D('',#147456,#114259,#114260) ;
#95361=AXIS2_PLACEMENT_3D('',#147457,#114261,#114262) ;
#95362=AXIS2_PLACEMENT_3D('',#147458,#114263,#114264) ;
#95363=AXIS2_PLACEMENT_3D('',#147459,#114265,#114266) ;
#95364=AXIS2_PLACEMENT_3D('',#147460,#114267,#114268) ;
#95365=AXIS2_PLACEMENT_3D('',#147461,#114269,#114270) ;
#95366=AXIS2_PLACEMENT_3D('',#147462,#114271,#114272) ;
#95367=AXIS2_PLACEMENT_3D('',#147463,#114273,#114274) ;
#95368=AXIS2_PLACEMENT_3D('',#147464,#114275,#114276) ;
#95369=AXIS2_PLACEMENT_3D('',#147465,#114277,#114278) ;
#95370=AXIS2_PLACEMENT_3D('',#147466,#114279,#114280) ;
#95371=AXIS2_PLACEMENT_3D('',#147467,#114281,#114282) ;
#95372=AXIS2_PLACEMENT_3D('',#147468,#114283,#114284) ;
#95373=AXIS2_PLACEMENT_3D('',#147469,#114285,#114286) ;
#95374=AXIS2_PLACEMENT_3D('',#147470,#114287,#114288) ;
#95375=AXIS2_PLACEMENT_3D('',#147471,#114289,#114290) ;
#95376=AXIS2_PLACEMENT_3D('',#147472,#114291,#114292) ;
#95377=AXIS2_PLACEMENT_3D('',#147473,#114293,#114294) ;
#95378=AXIS2_PLACEMENT_3D('',#147474,#114295,#114296) ;
#95379=AXIS2_PLACEMENT_3D('',#147475,#114297,#114298) ;
#95380=AXIS2_PLACEMENT_3D('',#147476,#114299,#114300) ;
#95381=AXIS2_PLACEMENT_3D('',#147477,#114301,#114302) ;
#95382=AXIS2_PLACEMENT_3D('',#147478,#114303,#114304) ;
#95383=AXIS2_PLACEMENT_3D('',#147479,#114305,#114306) ;
#95384=AXIS2_PLACEMENT_3D('',#147480,#114307,#114308) ;
#95385=AXIS2_PLACEMENT_3D('',#147481,#114309,#114310) ;
#95386=AXIS2_PLACEMENT_3D('',#147482,#114311,#114312) ;
#95387=AXIS2_PLACEMENT_3D('',#147483,#114313,#114314) ;
#95388=AXIS2_PLACEMENT_3D('',#147484,#114315,#114316) ;
#95389=AXIS2_PLACEMENT_3D('',#147485,#114317,#114318) ;
#95390=AXIS2_PLACEMENT_3D('',#147486,#114319,#114320) ;
#95391=AXIS2_PLACEMENT_3D('',#147487,#114321,#114322) ;
#95392=AXIS2_PLACEMENT_3D('',#147488,#114323,#114324) ;
#95393=AXIS2_PLACEMENT_3D('',#147489,#114325,#114326) ;
#95394=AXIS2_PLACEMENT_3D('',#147490,#114327,#114328) ;
#95395=AXIS2_PLACEMENT_3D('',#147491,#114329,#114330) ;
#95396=AXIS2_PLACEMENT_3D('',#147492,#114331,#114332) ;
#95397=AXIS2_PLACEMENT_3D('',#147493,#114333,#114334) ;
#95398=AXIS2_PLACEMENT_3D('',#147494,#114335,#114336) ;
#95399=AXIS2_PLACEMENT_3D('',#147495,#114337,#114338) ;
#95400=AXIS2_PLACEMENT_3D('',#147496,#114339,#114340) ;
#95401=AXIS2_PLACEMENT_3D('',#147497,#114341,#114342) ;
#95402=AXIS2_PLACEMENT_3D('',#147498,#114343,#114344) ;
#95403=AXIS2_PLACEMENT_3D('',#147499,#114345,#114346) ;
#95404=AXIS2_PLACEMENT_3D('',#147500,#114347,#114348) ;
#95405=AXIS2_PLACEMENT_3D('',#147501,#114349,#114350) ;
#95406=AXIS2_PLACEMENT_3D('',#147502,#114351,#114352) ;
#95407=AXIS2_PLACEMENT_3D('',#147503,#114353,#114354) ;
#95408=AXIS2_PLACEMENT_3D('',#147504,#114355,#114356) ;
#95409=AXIS2_PLACEMENT_3D('',#147505,#114357,#114358) ;
#95410=AXIS2_PLACEMENT_3D('',#147506,#114359,#114360) ;
#95411=AXIS2_PLACEMENT_3D('',#147507,#114361,#114362) ;
#95412=AXIS2_PLACEMENT_3D('',#147508,#114363,#114364) ;
#95413=AXIS2_PLACEMENT_3D('',#147509,#114365,#114366) ;
#95414=AXIS2_PLACEMENT_3D('',#147510,#114367,#114368) ;
#95415=AXIS2_PLACEMENT_3D('',#147511,#114369,#114370) ;
#95416=AXIS2_PLACEMENT_3D('',#147512,#114371,#114372) ;
#95417=AXIS2_PLACEMENT_3D('',#147513,#114373,#114374) ;
#95418=AXIS2_PLACEMENT_3D('',#147514,#114375,#114376) ;
#95419=AXIS2_PLACEMENT_3D('',#147515,#114377,#114378) ;
#95420=AXIS2_PLACEMENT_3D('',#147516,#114379,#114380) ;
#95421=AXIS2_PLACEMENT_3D('',#147517,#114381,#114382) ;
#95422=AXIS2_PLACEMENT_3D('',#147518,#114383,#114384) ;
#95423=AXIS2_PLACEMENT_3D('',#147519,#114385,#114386) ;
#95424=AXIS2_PLACEMENT_3D('',#147520,#114387,#114388) ;
#95425=AXIS2_PLACEMENT_3D('',#147521,#114389,#114390) ;
#95426=AXIS2_PLACEMENT_3D('',#147522,#114391,#114392) ;
#95427=AXIS2_PLACEMENT_3D('',#147523,#114393,#114394) ;
#95428=AXIS2_PLACEMENT_3D('',#147524,#114395,#114396) ;
#95429=AXIS2_PLACEMENT_3D('',#147525,#114397,#114398) ;
#95430=AXIS2_PLACEMENT_3D('',#147526,#114399,#114400) ;
#95431=AXIS2_PLACEMENT_3D('',#147527,#114401,#114402) ;
#95432=AXIS2_PLACEMENT_3D('',#147528,#114403,#114404) ;
#95433=AXIS2_PLACEMENT_3D('',#147529,#114405,#114406) ;
#95434=AXIS2_PLACEMENT_3D('',#147530,#114407,#114408) ;
#95435=AXIS2_PLACEMENT_3D('',#147531,#114409,#114410) ;
#95436=AXIS2_PLACEMENT_3D('',#147532,#114411,#114412) ;
#95437=AXIS2_PLACEMENT_3D('',#147533,#114413,#114414) ;
#95438=AXIS2_PLACEMENT_3D('',#147534,#114415,#114416) ;
#95439=AXIS2_PLACEMENT_3D('',#147535,#114417,#114418) ;
#95440=AXIS2_PLACEMENT_3D('',#147536,#114419,#114420) ;
#95441=AXIS2_PLACEMENT_3D('',#147537,#114421,#114422) ;
#95442=AXIS2_PLACEMENT_3D('',#147538,#114423,#114424) ;
#95443=AXIS2_PLACEMENT_3D('',#147539,#114425,#114426) ;
#95444=AXIS2_PLACEMENT_3D('',#147540,#114427,#114428) ;
#95445=AXIS2_PLACEMENT_3D('',#147541,#114429,#114430) ;
#95446=AXIS2_PLACEMENT_3D('',#147542,#114431,#114432) ;
#95447=AXIS2_PLACEMENT_3D('',#147543,#114433,#114434) ;
#95448=AXIS2_PLACEMENT_3D('',#147544,#114435,#114436) ;
#95449=AXIS2_PLACEMENT_3D('',#147545,#114437,#114438) ;
#95450=AXIS2_PLACEMENT_3D('',#147546,#114439,#114440) ;
#95451=AXIS2_PLACEMENT_3D('',#147547,#114441,#114442) ;
#95452=AXIS2_PLACEMENT_3D('',#147548,#114443,#114444) ;
#95453=AXIS2_PLACEMENT_3D('',#147549,#114445,#114446) ;
#95454=AXIS2_PLACEMENT_3D('',#147550,#114447,#114448) ;
#95455=AXIS2_PLACEMENT_3D('',#147551,#114449,#114450) ;
#95456=AXIS2_PLACEMENT_3D('',#147552,#114451,#114452) ;
#95457=AXIS2_PLACEMENT_3D('',#147553,#114453,#114454) ;
#95458=AXIS2_PLACEMENT_3D('',#147554,#114455,#114456) ;
#95459=AXIS2_PLACEMENT_3D('',#147555,#114457,#114458) ;
#95460=AXIS2_PLACEMENT_3D('',#147556,#114459,#114460) ;
#95461=AXIS2_PLACEMENT_3D('',#147557,#114461,#114462) ;
#95462=AXIS2_PLACEMENT_3D('',#147558,#114463,#114464) ;
#95463=AXIS2_PLACEMENT_3D('',#147559,#114465,#114466) ;
#95464=AXIS2_PLACEMENT_3D('',#147560,#114467,#114468) ;
#95465=AXIS2_PLACEMENT_3D('',#147561,#114469,#114470) ;
#95466=AXIS2_PLACEMENT_3D('',#147562,#114471,#114472) ;
#95467=AXIS2_PLACEMENT_3D('',#147563,#114473,#114474) ;
#95468=AXIS2_PLACEMENT_3D('',#147564,#114475,#114476) ;
#95469=AXIS2_PLACEMENT_3D('',#147565,#114477,#114478) ;
#95470=AXIS2_PLACEMENT_3D('',#147566,#114479,#114480) ;
#95471=AXIS2_PLACEMENT_3D('',#147567,#114481,#114482) ;
#95472=AXIS2_PLACEMENT_3D('',#147568,#114483,#114484) ;
#95473=AXIS2_PLACEMENT_3D('',#147569,#114485,#114486) ;
#95474=AXIS2_PLACEMENT_3D('',#147570,#114487,#114488) ;
#95475=AXIS2_PLACEMENT_3D('',#147571,#114489,#114490) ;
#95476=AXIS2_PLACEMENT_3D('',#147572,#114491,#114492) ;
#95477=AXIS2_PLACEMENT_3D('',#147573,#114493,#114494) ;
#95478=AXIS2_PLACEMENT_3D('',#147574,#114495,#114496) ;
#95479=AXIS2_PLACEMENT_3D('',#147575,#114497,#114498) ;
#95480=AXIS2_PLACEMENT_3D('',#147576,#114499,#114500) ;
#95481=AXIS2_PLACEMENT_3D('',#147577,#114501,#114502) ;
#95482=AXIS2_PLACEMENT_3D('',#147578,#114503,#114504) ;
#95483=AXIS2_PLACEMENT_3D('',#147579,#114505,#114506) ;
#95484=AXIS2_PLACEMENT_3D('',#147580,#114507,#114508) ;
#95485=AXIS2_PLACEMENT_3D('',#147581,#114509,#114510) ;
#95486=AXIS2_PLACEMENT_3D('',#147582,#114511,#114512) ;
#95487=AXIS2_PLACEMENT_3D('',#147583,#114513,#114514) ;
#95488=AXIS2_PLACEMENT_3D('',#147584,#114515,#114516) ;
#95489=AXIS2_PLACEMENT_3D('',#147585,#114517,#114518) ;
#95490=AXIS2_PLACEMENT_3D('',#147586,#114519,#114520) ;
#95491=AXIS2_PLACEMENT_3D('',#147587,#114521,#114522) ;
#95492=AXIS2_PLACEMENT_3D('',#147588,#114523,#114524) ;
#95493=AXIS2_PLACEMENT_3D('',#147589,#114525,#114526) ;
#95494=AXIS2_PLACEMENT_3D('',#147590,#114527,#114528) ;
#95495=AXIS2_PLACEMENT_3D('',#147591,#114529,#114530) ;
#95496=AXIS2_PLACEMENT_3D('',#147592,#114531,#114532) ;
#95497=AXIS2_PLACEMENT_3D('',#147593,#114533,#114534) ;
#95498=AXIS2_PLACEMENT_3D('',#147594,#114535,#114536) ;
#95499=AXIS2_PLACEMENT_3D('',#147595,#114537,#114538) ;
#95500=AXIS2_PLACEMENT_3D('',#147596,#114539,#114540) ;
#95501=AXIS2_PLACEMENT_3D('',#147597,#114541,#114542) ;
#95502=AXIS2_PLACEMENT_3D('',#147598,#114543,#114544) ;
#95503=AXIS2_PLACEMENT_3D('',#147599,#114545,#114546) ;
#95504=AXIS2_PLACEMENT_3D('',#147600,#114547,#114548) ;
#95505=AXIS2_PLACEMENT_3D('',#147601,#114549,#114550) ;
#95506=AXIS2_PLACEMENT_3D('',#147602,#114551,#114552) ;
#95507=AXIS2_PLACEMENT_3D('',#147603,#114553,#114554) ;
#95508=AXIS2_PLACEMENT_3D('',#147604,#114555,#114556) ;
#95509=AXIS2_PLACEMENT_3D('',#147605,#114557,#114558) ;
#95510=AXIS2_PLACEMENT_3D('',#147606,#114559,#114560) ;
#95511=AXIS2_PLACEMENT_3D('',#147607,#114561,#114562) ;
#95512=AXIS2_PLACEMENT_3D('',#147608,#114563,#114564) ;
#95513=AXIS2_PLACEMENT_3D('',#147609,#114565,#114566) ;
#95514=AXIS2_PLACEMENT_3D('',#147610,#114567,#114568) ;
#95515=AXIS2_PLACEMENT_3D('',#147611,#114569,#114570) ;
#95516=AXIS2_PLACEMENT_3D('',#147612,#114571,#114572) ;
#95517=AXIS2_PLACEMENT_3D('',#147613,#114573,#114574) ;
#95518=AXIS2_PLACEMENT_3D('',#147614,#114575,#114576) ;
#95519=AXIS2_PLACEMENT_3D('',#147615,#114577,#114578) ;
#95520=AXIS2_PLACEMENT_3D('',#147616,#114579,#114580) ;
#95521=AXIS2_PLACEMENT_3D('',#147617,#114581,#114582) ;
#95522=AXIS2_PLACEMENT_3D('',#147618,#114583,#114584) ;
#95523=AXIS2_PLACEMENT_3D('',#147619,#114585,#114586) ;
#95524=AXIS2_PLACEMENT_3D('',#147620,#114587,#114588) ;
#95525=AXIS2_PLACEMENT_3D('',#147621,#114589,#114590) ;
#95526=AXIS2_PLACEMENT_3D('',#147622,#114591,#114592) ;
#95527=AXIS2_PLACEMENT_3D('',#147623,#114593,#114594) ;
#95528=AXIS2_PLACEMENT_3D('',#147624,#114595,#114596) ;
#95529=AXIS2_PLACEMENT_3D('',#147625,#114597,#114598) ;
#95530=AXIS2_PLACEMENT_3D('',#147626,#114599,#114600) ;
#95531=AXIS2_PLACEMENT_3D('',#147627,#114601,#114602) ;
#95532=AXIS2_PLACEMENT_3D('',#147628,#114603,#114604) ;
#95533=AXIS2_PLACEMENT_3D('',#147629,#114605,#114606) ;
#95534=AXIS2_PLACEMENT_3D('',#147630,#114607,#114608) ;
#95535=AXIS2_PLACEMENT_3D('',#147631,#114609,#114610) ;
#95536=AXIS2_PLACEMENT_3D('',#147632,#114611,#114612) ;
#95537=AXIS2_PLACEMENT_3D('',#147633,#114613,#114614) ;
#95538=AXIS2_PLACEMENT_3D('',#147634,#114615,#114616) ;
#95539=AXIS2_PLACEMENT_3D('',#147635,#114617,#114618) ;
#95540=AXIS2_PLACEMENT_3D('',#147636,#114619,#114620) ;
#95541=AXIS2_PLACEMENT_3D('',#147637,#114621,#114622) ;
#95542=AXIS2_PLACEMENT_3D('',#147638,#114623,#114624) ;
#95543=AXIS2_PLACEMENT_3D('',#147639,#114625,#114626) ;
#95544=AXIS2_PLACEMENT_3D('',#147640,#114627,#114628) ;
#95545=AXIS2_PLACEMENT_3D('',#147641,#114629,#114630) ;
#95546=AXIS2_PLACEMENT_3D('',#147642,#114631,#114632) ;
#95547=AXIS2_PLACEMENT_3D('',#147643,#114633,#114634) ;
#95548=AXIS2_PLACEMENT_3D('',#147644,#114635,#114636) ;
#95549=AXIS2_PLACEMENT_3D('',#147645,#114637,#114638) ;
#95550=AXIS2_PLACEMENT_3D('',#147646,#114639,#114640) ;
#95551=AXIS2_PLACEMENT_3D('',#147647,#114641,#114642) ;
#95552=AXIS2_PLACEMENT_3D('',#147648,#114643,#114644) ;
#95553=AXIS2_PLACEMENT_3D('',#147649,#114645,#114646) ;
#95554=AXIS2_PLACEMENT_3D('',#147650,#114647,#114648) ;
#95555=AXIS2_PLACEMENT_3D('',#147651,#114649,#114650) ;
#95556=AXIS2_PLACEMENT_3D('',#147652,#114651,#114652) ;
#95557=AXIS2_PLACEMENT_3D('',#147653,#114653,#114654) ;
#95558=AXIS2_PLACEMENT_3D('',#147654,#114655,#114656) ;
#95559=AXIS2_PLACEMENT_3D('',#147655,#114657,#114658) ;
#95560=AXIS2_PLACEMENT_3D('',#147656,#114659,#114660) ;
#95561=AXIS2_PLACEMENT_3D('',#147657,#114661,#114662) ;
#95562=AXIS2_PLACEMENT_3D('',#147658,#114663,#114664) ;
#95563=AXIS2_PLACEMENT_3D('',#147659,#114665,#114666) ;
#95564=AXIS2_PLACEMENT_3D('',#147660,#114667,#114668) ;
#95565=AXIS2_PLACEMENT_3D('',#147661,#114669,#114670) ;
#95566=AXIS2_PLACEMENT_3D('',#147662,#114671,#114672) ;
#95567=AXIS2_PLACEMENT_3D('',#147663,#114673,#114674) ;
#95568=AXIS2_PLACEMENT_3D('',#147664,#114675,#114676) ;
#95569=AXIS2_PLACEMENT_3D('',#147665,#114677,#114678) ;
#95570=AXIS2_PLACEMENT_3D('',#147666,#114679,#114680) ;
#95571=AXIS2_PLACEMENT_3D('',#147667,#114681,#114682) ;
#95572=AXIS2_PLACEMENT_3D('',#147668,#114683,#114684) ;
#95573=AXIS2_PLACEMENT_3D('',#147669,#114685,#114686) ;
#95574=AXIS2_PLACEMENT_3D('',#147670,#114687,#114688) ;
#95575=AXIS2_PLACEMENT_3D('',#147671,#114689,#114690) ;
#95576=AXIS2_PLACEMENT_3D('',#147672,#114691,#114692) ;
#95577=AXIS2_PLACEMENT_3D('',#147673,#114693,#114694) ;
#95578=AXIS2_PLACEMENT_3D('',#147674,#114695,#114696) ;
#95579=AXIS2_PLACEMENT_3D('',#147675,#114697,#114698) ;
#95580=AXIS2_PLACEMENT_3D('',#147676,#114699,#114700) ;
#95581=AXIS2_PLACEMENT_3D('',#147677,#114701,#114702) ;
#95582=AXIS2_PLACEMENT_3D('',#147678,#114703,#114704) ;
#95583=AXIS2_PLACEMENT_3D('',#147679,#114705,#114706) ;
#95584=AXIS2_PLACEMENT_3D('',#147680,#114707,#114708) ;
#95585=AXIS2_PLACEMENT_3D('',#147681,#114709,#114710) ;
#95586=AXIS2_PLACEMENT_3D('',#147682,#114711,#114712) ;
#95587=AXIS2_PLACEMENT_3D('',#147683,#114713,#114714) ;
#95588=AXIS2_PLACEMENT_3D('',#147684,#114715,#114716) ;
#95589=AXIS2_PLACEMENT_3D('',#147685,#114717,#114718) ;
#95590=AXIS2_PLACEMENT_3D('',#147686,#114719,#114720) ;
#95591=AXIS2_PLACEMENT_3D('',#147687,#114721,#114722) ;
#95592=AXIS2_PLACEMENT_3D('',#147688,#114723,#114724) ;
#95593=AXIS2_PLACEMENT_3D('',#147689,#114725,#114726) ;
#95594=AXIS2_PLACEMENT_3D('',#147690,#114727,#114728) ;
#95595=AXIS2_PLACEMENT_3D('',#147691,#114729,#114730) ;
#95596=AXIS2_PLACEMENT_3D('',#147692,#114731,#114732) ;
#95597=AXIS2_PLACEMENT_3D('',#147693,#114733,#114734) ;
#95598=AXIS2_PLACEMENT_3D('',#147694,#114735,#114736) ;
#95599=AXIS2_PLACEMENT_3D('',#147695,#114737,#114738) ;
#95600=AXIS2_PLACEMENT_3D('',#147696,#114739,#114740) ;
#95601=AXIS2_PLACEMENT_3D('',#147697,#114741,#114742) ;
#95602=AXIS2_PLACEMENT_3D('',#147698,#114743,#114744) ;
#95603=AXIS2_PLACEMENT_3D('',#147699,#114745,#114746) ;
#95604=AXIS2_PLACEMENT_3D('',#147700,#114747,#114748) ;
#95605=AXIS2_PLACEMENT_3D('',#147701,#114749,#114750) ;
#95606=AXIS2_PLACEMENT_3D('',#147702,#114751,#114752) ;
#95607=AXIS2_PLACEMENT_3D('',#147703,#114753,#114754) ;
#95608=AXIS2_PLACEMENT_3D('',#147704,#114755,#114756) ;
#95609=AXIS2_PLACEMENT_3D('',#147705,#114757,#114758) ;
#95610=AXIS2_PLACEMENT_3D('',#147706,#114759,#114760) ;
#95611=AXIS2_PLACEMENT_3D('',#147707,#114761,#114762) ;
#95612=AXIS2_PLACEMENT_3D('',#147708,#114763,#114764) ;
#95613=AXIS2_PLACEMENT_3D('',#147709,#114765,#114766) ;
#95614=AXIS2_PLACEMENT_3D('',#147710,#114767,#114768) ;
#95615=AXIS2_PLACEMENT_3D('',#147711,#114769,#114770) ;
#95616=AXIS2_PLACEMENT_3D('',#147712,#114771,#114772) ;
#95617=AXIS2_PLACEMENT_3D('',#147713,#114773,#114774) ;
#95618=AXIS2_PLACEMENT_3D('',#147714,#114775,#114776) ;
#95619=AXIS2_PLACEMENT_3D('',#147715,#114777,#114778) ;
#95620=AXIS2_PLACEMENT_3D('',#147716,#114779,#114780) ;
#95621=AXIS2_PLACEMENT_3D('',#147717,#114781,#114782) ;
#95622=AXIS2_PLACEMENT_3D('',#147718,#114783,#114784) ;
#95623=AXIS2_PLACEMENT_3D('',#147719,#114785,#114786) ;
#95624=AXIS2_PLACEMENT_3D('',#147720,#114787,#114788) ;
#95625=AXIS2_PLACEMENT_3D('',#147721,#114789,#114790) ;
#95626=AXIS2_PLACEMENT_3D('',#147722,#114791,#114792) ;
#95627=AXIS2_PLACEMENT_3D('',#147723,#114793,#114794) ;
#95628=AXIS2_PLACEMENT_3D('',#147724,#114795,#114796) ;
#95629=AXIS2_PLACEMENT_3D('',#147725,#114797,#114798) ;
#95630=AXIS2_PLACEMENT_3D('',#147726,#114799,#114800) ;
#95631=AXIS2_PLACEMENT_3D('',#147727,#114801,#114802) ;
#95632=AXIS2_PLACEMENT_3D('',#147728,#114803,#114804) ;
#95633=AXIS2_PLACEMENT_3D('',#147729,#114805,#114806) ;
#95634=AXIS2_PLACEMENT_3D('',#147730,#114807,#114808) ;
#95635=AXIS2_PLACEMENT_3D('',#147731,#114809,#114810) ;
#95636=AXIS2_PLACEMENT_3D('',#147732,#114811,#114812) ;
#95637=AXIS2_PLACEMENT_3D('',#147733,#114813,#114814) ;
#95638=AXIS2_PLACEMENT_3D('',#147734,#114815,#114816) ;
#95639=AXIS2_PLACEMENT_3D('',#147735,#114817,#114818) ;
#95640=AXIS2_PLACEMENT_3D('',#147736,#114819,#114820) ;
#95641=AXIS2_PLACEMENT_3D('',#147737,#114821,#114822) ;
#95642=AXIS2_PLACEMENT_3D('',#147738,#114823,#114824) ;
#95643=AXIS2_PLACEMENT_3D('',#147739,#114825,#114826) ;
#95644=AXIS2_PLACEMENT_3D('',#147740,#114827,#114828) ;
#95645=AXIS2_PLACEMENT_3D('',#147741,#114829,#114830) ;
#95646=AXIS2_PLACEMENT_3D('',#147742,#114831,#114832) ;
#95647=AXIS2_PLACEMENT_3D('',#147743,#114833,#114834) ;
#95648=AXIS2_PLACEMENT_3D('',#147744,#114835,#114836) ;
#95649=AXIS2_PLACEMENT_3D('',#147745,#114837,#114838) ;
#95650=AXIS2_PLACEMENT_3D('',#147746,#114839,#114840) ;
#95651=AXIS2_PLACEMENT_3D('',#147747,#114841,#114842) ;
#95652=AXIS2_PLACEMENT_3D('',#147748,#114843,#114844) ;
#95653=AXIS2_PLACEMENT_3D('',#147749,#114845,#114846) ;
#95654=AXIS2_PLACEMENT_3D('',#147750,#114847,#114848) ;
#95655=AXIS2_PLACEMENT_3D('',#147751,#114849,#114850) ;
#95656=AXIS2_PLACEMENT_3D('',#147752,#114851,#114852) ;
#95657=AXIS2_PLACEMENT_3D('',#147753,#114853,#114854) ;
#95658=AXIS2_PLACEMENT_3D('',#147754,#114855,#114856) ;
#95659=AXIS2_PLACEMENT_3D('',#147755,#114857,#114858) ;
#95660=AXIS2_PLACEMENT_3D('',#147756,#114859,#114860) ;
#95661=AXIS2_PLACEMENT_3D('',#147757,#114861,#114862) ;
#95662=AXIS2_PLACEMENT_3D('',#147758,#114863,#114864) ;
#95663=AXIS2_PLACEMENT_3D('',#147759,#114865,#114866) ;
#95664=AXIS2_PLACEMENT_3D('',#147760,#114867,#114868) ;
#95665=AXIS2_PLACEMENT_3D('',#147761,#114869,#114870) ;
#95666=AXIS2_PLACEMENT_3D('',#147762,#114871,#114872) ;
#95667=AXIS2_PLACEMENT_3D('',#147763,#114873,#114874) ;
#95668=AXIS2_PLACEMENT_3D('',#147764,#114875,#114876) ;
#95669=AXIS2_PLACEMENT_3D('',#147765,#114877,#114878) ;
#95670=AXIS2_PLACEMENT_3D('',#147766,#114879,#114880) ;
#95671=AXIS2_PLACEMENT_3D('',#147767,#114881,#114882) ;
#95672=AXIS2_PLACEMENT_3D('',#147768,#114883,#114884) ;
#95673=AXIS2_PLACEMENT_3D('',#147769,#114885,#114886) ;
#95674=AXIS2_PLACEMENT_3D('',#147771,#114887,#114888) ;
#95675=AXIS2_PLACEMENT_3D('',#147772,#114889,#114890) ;
#95676=AXIS2_PLACEMENT_3D('',#147773,#114891,#114892) ;
#95677=AXIS2_PLACEMENT_3D('',#147774,#114893,#114894) ;
#95678=AXIS2_PLACEMENT_3D('',#147775,#114895,#114896) ;
#95679=AXIS2_PLACEMENT_3D('',#147776,#114897,#114898) ;
#95680=AXIS2_PLACEMENT_3D('',#147777,#114899,#114900) ;
#95681=AXIS2_PLACEMENT_3D('',#147778,#114901,#114902) ;
#95682=AXIS2_PLACEMENT_3D('',#147779,#114903,#114904) ;
#95683=AXIS2_PLACEMENT_3D('',#147790,#114906,#114907) ;
#95684=AXIS2_PLACEMENT_3D('',#147847,#114909,#114910) ;
#95685=AXIS2_PLACEMENT_3D('',#147848,#114911,#114912) ;
#95686=AXIS2_PLACEMENT_3D('',#147849,#114913,#114914) ;
#95687=AXIS2_PLACEMENT_3D('',#147850,#114915,#114916) ;
#95688=AXIS2_PLACEMENT_3D('',#147851,#114917,#114918) ;
#95689=AXIS2_PLACEMENT_3D('',#147852,#114919,#114920) ;
#95690=AXIS2_PLACEMENT_3D('',#147853,#114921,#114922) ;
#95691=AXIS2_PLACEMENT_3D('',#147854,#114923,#114924) ;
#95692=AXIS2_PLACEMENT_3D('',#147855,#114925,#114926) ;
#95693=AXIS2_PLACEMENT_3D('',#147856,#114927,#114928) ;
#95694=AXIS2_PLACEMENT_3D('',#147857,#114929,#114930) ;
#95695=AXIS2_PLACEMENT_3D('',#147858,#114931,#114932) ;
#95696=AXIS2_PLACEMENT_3D('',#147859,#114933,#114934) ;
#95697=AXIS2_PLACEMENT_3D('',#147860,#114935,#114936) ;
#95698=AXIS2_PLACEMENT_3D('',#147861,#114937,#114938) ;
#95699=AXIS2_PLACEMENT_3D('',#147862,#114939,#114940) ;
#95700=AXIS2_PLACEMENT_3D('',#147863,#114941,#114942) ;
#95701=AXIS2_PLACEMENT_3D('',#147864,#114943,#114944) ;
#95702=AXIS2_PLACEMENT_3D('',#147865,#114945,#114946) ;
#95703=AXIS2_PLACEMENT_3D('',#147866,#114947,#114948) ;
#95704=AXIS2_PLACEMENT_3D('',#147867,#114949,#114950) ;
#95705=AXIS2_PLACEMENT_3D('',#147868,#114951,#114952) ;
#95706=AXIS2_PLACEMENT_3D('',#147869,#114953,#114954) ;
#95707=AXIS2_PLACEMENT_3D('',#147872,#114956,#114957) ;
#95708=AXIS2_PLACEMENT_3D('',#147873,#114958,#114959) ;
#95709=AXIS2_PLACEMENT_3D('',#147874,#114960,#114961) ;
#95710=AXIS2_PLACEMENT_3D('',#147875,#114962,#114963) ;
#95711=AXIS2_PLACEMENT_3D('',#147876,#114964,#114965) ;
#95712=AXIS2_PLACEMENT_3D('',#147877,#114966,#114967) ;
#95713=AXIS2_PLACEMENT_3D('',#147878,#114968,#114969) ;
#95714=AXIS2_PLACEMENT_3D('',#147879,#114970,#114971) ;
#95715=AXIS2_PLACEMENT_3D('',#147880,#114972,#114973) ;
#95716=AXIS2_PLACEMENT_3D('',#147881,#114974,#114975) ;
#95717=AXIS2_PLACEMENT_3D('',#147882,#114976,#114977) ;
#95718=AXIS2_PLACEMENT_3D('',#147883,#114978,#114979) ;
#95719=AXIS2_PLACEMENT_3D('',#147884,#114980,#114981) ;
#95720=AXIS2_PLACEMENT_3D('',#147885,#114982,#114983) ;
#95721=AXIS2_PLACEMENT_3D('',#147886,#114984,#114985) ;
#95722=AXIS2_PLACEMENT_3D('',#147887,#114986,#114987) ;
#95723=AXIS2_PLACEMENT_3D('',#147889,#114988,#114989) ;
#95724=AXIS2_PLACEMENT_3D('',#147890,#114990,#114991) ;
#95725=AXIS2_PLACEMENT_3D('',#147891,#114992,#114993) ;
#95726=AXIS2_PLACEMENT_3D('',#147892,#114994,#114995) ;
#95727=AXIS2_PLACEMENT_3D('',#147893,#114996,#114997) ;
#95728=AXIS2_PLACEMENT_3D('',#147894,#114998,#114999) ;
#95729=AXIS2_PLACEMENT_3D('',#147895,#115000,#115001) ;
#95730=AXIS2_PLACEMENT_3D('',#147896,#115002,#115003) ;
#95731=AXIS2_PLACEMENT_3D('',#147897,#115004,#115005) ;
#95732=AXIS2_PLACEMENT_3D('',#147898,#115006,#115007) ;
#95733=AXIS2_PLACEMENT_3D('',#147899,#115008,#115009) ;
#95734=AXIS2_PLACEMENT_3D('',#147900,#115010,#115011) ;
#95735=AXIS2_PLACEMENT_3D('',#147901,#115012,#115013) ;
#95736=AXIS2_PLACEMENT_3D('',#147904,#115015,#115016) ;
#95737=AXIS2_PLACEMENT_3D('',#147905,#115017,#115018) ;
#95738=AXIS2_PLACEMENT_3D('',#147906,#115019,#115020) ;
#95739=AXIS2_PLACEMENT_3D('',#147907,#115021,#115022) ;
#95740=AXIS2_PLACEMENT_3D('',#147908,#115023,#115024) ;
#95741=AXIS2_PLACEMENT_3D('',#147909,#115025,#115026) ;
#95742=AXIS2_PLACEMENT_3D('',#147910,#115027,#115028) ;
#95743=AXIS2_PLACEMENT_3D('',#147911,#115029,#115030) ;
#95744=AXIS2_PLACEMENT_3D('',#147912,#115031,#115032) ;
#95745=AXIS2_PLACEMENT_3D('',#147913,#115033,#115034) ;
#95746=AXIS2_PLACEMENT_3D('',#147914,#115035,#115036) ;
#95747=AXIS2_PLACEMENT_3D('',#147915,#115037,#115038) ;
#95748=AXIS2_PLACEMENT_3D('',#147916,#115039,#115040) ;
#95749=AXIS2_PLACEMENT_3D('',#147918,#115041,#115042) ;
#95750=AXIS2_PLACEMENT_3D('',#147919,#115043,#115044) ;
#95751=AXIS2_PLACEMENT_3D('',#147920,#115045,#115046) ;
#95752=AXIS2_PLACEMENT_3D('',#147921,#115047,#115048) ;
#95753=AXIS2_PLACEMENT_3D('',#147922,#115049,#115050) ;
#95754=AXIS2_PLACEMENT_3D('',#147923,#115051,#115052) ;
#95755=AXIS2_PLACEMENT_3D('',#147924,#115053,#115054) ;
#95756=AXIS2_PLACEMENT_3D('',#147925,#115055,#115056) ;
#95757=AXIS2_PLACEMENT_3D('',#147926,#115057,#115058) ;
#95758=AXIS2_PLACEMENT_3D('',#147927,#115059,#115060) ;
#95759=AXIS2_PLACEMENT_3D('',#147928,#115061,#115062) ;
#95760=AXIS2_PLACEMENT_3D('',#147930,#115064,#115065) ;
#95761=AXIS2_PLACEMENT_3D('',#147931,#115066,#115067) ;
#95762=AXIS2_PLACEMENT_3D('',#147932,#115068,#115069) ;
#95763=AXIS2_PLACEMENT_3D('',#147933,#115070,#115071) ;
#95764=AXIS2_PLACEMENT_3D('',#147934,#115072,#115073) ;
#95765=AXIS2_PLACEMENT_3D('',#147935,#115074,#115075) ;
#95766=AXIS2_PLACEMENT_3D('',#147936,#115076,#115077) ;
#95767=AXIS2_PLACEMENT_3D('',#147937,#115078,#115079) ;
#95768=AXIS2_PLACEMENT_3D('',#147938,#115080,#115081) ;
#95769=AXIS2_PLACEMENT_3D('',#147939,#115082,#115083) ;
#95770=AXIS2_PLACEMENT_3D('',#147940,#115084,#115085) ;
#95771=AXIS2_PLACEMENT_3D('',#147941,#115086,#115087) ;
#95772=AXIS2_PLACEMENT_3D('',#147942,#115088,#115089) ;
#95773=AXIS2_PLACEMENT_3D('',#147943,#115090,#115091) ;
#95774=AXIS2_PLACEMENT_3D('',#147944,#115092,#115093) ;
#95775=AXIS2_PLACEMENT_3D('',#147945,#115094,#115095) ;
#95776=AXIS2_PLACEMENT_3D('',#147946,#115096,#115097) ;
#95777=AXIS2_PLACEMENT_3D('',#147947,#115098,#115099) ;
#95778=AXIS2_PLACEMENT_3D('',#147948,#115100,#115101) ;
#95779=AXIS2_PLACEMENT_3D('',#147949,#115102,#115103) ;
#95780=AXIS2_PLACEMENT_3D('',#147950,#115104,#115105) ;
#95781=AXIS2_PLACEMENT_3D('',#147951,#115106,#115107) ;
#95782=AXIS2_PLACEMENT_3D('',#147952,#115108,#115109) ;
#95783=AXIS2_PLACEMENT_3D('',#147953,#115110,#115111) ;
#95784=AXIS2_PLACEMENT_3D('',#147954,#115112,#115113) ;
#95785=AXIS2_PLACEMENT_3D('',#147955,#115114,#115115) ;
#95786=AXIS2_PLACEMENT_3D('',#147956,#115116,#115117) ;
#95787=AXIS2_PLACEMENT_3D('',#147957,#115118,#115119) ;
#95788=AXIS2_PLACEMENT_3D('',#147958,#115120,#115121) ;
#95789=AXIS2_PLACEMENT_3D('',#147959,#115122,#115123) ;
#95790=AXIS2_PLACEMENT_3D('',#147960,#115124,#115125) ;
#95791=AXIS2_PLACEMENT_3D('',#147961,#115126,#115127) ;
#95792=AXIS2_PLACEMENT_3D('',#147962,#115128,#115129) ;
#95793=AXIS2_PLACEMENT_3D('',#147963,#115130,#115131) ;
#95794=AXIS2_PLACEMENT_3D('',#147964,#115132,#115133) ;
#95795=AXIS2_PLACEMENT_3D('',#147965,#115134,#115135) ;
#95796=AXIS2_PLACEMENT_3D('',#147966,#115136,#115137) ;
#95797=AXIS2_PLACEMENT_3D('',#147967,#115138,#115139) ;
#95798=AXIS2_PLACEMENT_3D('',#147968,#115140,#115141) ;
#95799=AXIS2_PLACEMENT_3D('',#147969,#115142,#115143) ;
#95800=AXIS2_PLACEMENT_3D('',#147970,#115144,#115145) ;
#95801=AXIS2_PLACEMENT_3D('',#147971,#115146,#115147) ;
#95802=AXIS2_PLACEMENT_3D('',#147972,#115148,#115149) ;
#95803=AXIS2_PLACEMENT_3D('',#147973,#115150,#115151) ;
#95804=AXIS2_PLACEMENT_3D('',#147974,#115152,#115153) ;
#95805=AXIS2_PLACEMENT_3D('',#147975,#115154,#115155) ;
#95806=AXIS2_PLACEMENT_3D('',#147976,#115156,#115157) ;
#95807=AXIS2_PLACEMENT_3D('',#147977,#115158,#115159) ;
#95808=AXIS2_PLACEMENT_3D('',#147978,#115160,#115161) ;
#95809=AXIS2_PLACEMENT_3D('',#147979,#115162,#115163) ;
#95810=AXIS2_PLACEMENT_3D('',#147980,#115164,#115165) ;
#95811=AXIS2_PLACEMENT_3D('',#147981,#115166,#115167) ;
#95812=AXIS2_PLACEMENT_3D('',#147982,#115168,#115169) ;
#95813=AXIS2_PLACEMENT_3D('',#147983,#115170,#115171) ;
#95814=AXIS2_PLACEMENT_3D('',#147984,#115172,#115173) ;
#95815=AXIS2_PLACEMENT_3D('',#147985,#115174,#115175) ;
#95816=AXIS2_PLACEMENT_3D('',#147986,#115176,#115177) ;
#95817=AXIS2_PLACEMENT_3D('',#147987,#115178,#115179) ;
#95818=AXIS2_PLACEMENT_3D('',#147988,#115180,#115181) ;
#95819=AXIS2_PLACEMENT_3D('',#147989,#115182,#115183) ;
#95820=AXIS2_PLACEMENT_3D('',#147990,#115184,#115185) ;
#95821=AXIS2_PLACEMENT_3D('',#147991,#115186,#115187) ;
#95822=AXIS2_PLACEMENT_3D('',#147992,#115188,#115189) ;
#95823=AXIS2_PLACEMENT_3D('',#147993,#115190,#115191) ;
#95824=AXIS2_PLACEMENT_3D('',#147994,#115192,#115193) ;
#95825=AXIS2_PLACEMENT_3D('',#147995,#115194,#115195) ;
#95826=AXIS2_PLACEMENT_3D('',#147996,#115196,#115197) ;
#95827=AXIS2_PLACEMENT_3D('',#147998,#115198,#115199) ;
#95828=AXIS2_PLACEMENT_3D('',#147999,#115200,#115201) ;
#95829=AXIS2_PLACEMENT_3D('',#148000,#115202,#115203) ;
#95830=AXIS2_PLACEMENT_3D('',#148001,#115204,#115205) ;
#95831=AXIS2_PLACEMENT_3D('',#148002,#115206,#115207) ;
#95832=AXIS2_PLACEMENT_3D('',#148003,#115208,#115209) ;
#95833=AXIS2_PLACEMENT_3D('',#148004,#115210,#115211) ;
#95834=AXIS2_PLACEMENT_3D('',#148005,#115212,#115213) ;
#95835=AXIS2_PLACEMENT_3D('',#148006,#115214,#115215) ;
#95836=AXIS2_PLACEMENT_3D('',#148017,#115217,#115218) ;
#95837=AXIS2_PLACEMENT_3D('',#148074,#115220,#115221) ;
#95838=AXIS2_PLACEMENT_3D('',#148075,#115222,#115223) ;
#95839=AXIS2_PLACEMENT_3D('',#148076,#115224,#115225) ;
#95840=AXIS2_PLACEMENT_3D('',#148077,#115226,#115227) ;
#95841=AXIS2_PLACEMENT_3D('',#148078,#115228,#115229) ;
#95842=AXIS2_PLACEMENT_3D('',#148079,#115230,#115231) ;
#95843=AXIS2_PLACEMENT_3D('',#148080,#115232,#115233) ;
#95844=AXIS2_PLACEMENT_3D('',#148081,#115234,#115235) ;
#95845=AXIS2_PLACEMENT_3D('',#148082,#115236,#115237) ;
#95846=AXIS2_PLACEMENT_3D('',#148083,#115238,#115239) ;
#95847=AXIS2_PLACEMENT_3D('',#148084,#115240,#115241) ;
#95848=AXIS2_PLACEMENT_3D('',#148085,#115242,#115243) ;
#95849=AXIS2_PLACEMENT_3D('',#148086,#115244,#115245) ;
#95850=AXIS2_PLACEMENT_3D('',#148087,#115246,#115247) ;
#95851=AXIS2_PLACEMENT_3D('',#148088,#115248,#115249) ;
#95852=AXIS2_PLACEMENT_3D('',#148089,#115250,#115251) ;
#95853=AXIS2_PLACEMENT_3D('',#148090,#115252,#115253) ;
#95854=AXIS2_PLACEMENT_3D('',#148091,#115254,#115255) ;
#95855=AXIS2_PLACEMENT_3D('',#148092,#115256,#115257) ;
#95856=AXIS2_PLACEMENT_3D('',#148093,#115258,#115259) ;
#95857=AXIS2_PLACEMENT_3D('',#148094,#115260,#115261) ;
#95858=AXIS2_PLACEMENT_3D('',#148095,#115262,#115263) ;
#95859=AXIS2_PLACEMENT_3D('',#148096,#115264,#115265) ;
#95860=AXIS2_PLACEMENT_3D('',#148099,#115267,#115268) ;
#95861=AXIS2_PLACEMENT_3D('',#148100,#115269,#115270) ;
#95862=AXIS2_PLACEMENT_3D('',#148101,#115271,#115272) ;
#95863=AXIS2_PLACEMENT_3D('',#148102,#115273,#115274) ;
#95864=AXIS2_PLACEMENT_3D('',#148103,#115275,#115276) ;
#95865=AXIS2_PLACEMENT_3D('',#148104,#115277,#115278) ;
#95866=AXIS2_PLACEMENT_3D('',#148105,#115279,#115280) ;
#95867=AXIS2_PLACEMENT_3D('',#148106,#115281,#115282) ;
#95868=AXIS2_PLACEMENT_3D('',#148107,#115283,#115284) ;
#95869=AXIS2_PLACEMENT_3D('',#148108,#115285,#115286) ;
#95870=AXIS2_PLACEMENT_3D('',#148109,#115287,#115288) ;
#95871=AXIS2_PLACEMENT_3D('',#148110,#115289,#115290) ;
#95872=AXIS2_PLACEMENT_3D('',#148111,#115291,#115292) ;
#95873=AXIS2_PLACEMENT_3D('',#148112,#115293,#115294) ;
#95874=AXIS2_PLACEMENT_3D('',#148113,#115295,#115296) ;
#95875=AXIS2_PLACEMENT_3D('',#148114,#115297,#115298) ;
#95876=AXIS2_PLACEMENT_3D('',#148116,#115299,#115300) ;
#95877=AXIS2_PLACEMENT_3D('',#148117,#115301,#115302) ;
#95878=AXIS2_PLACEMENT_3D('',#148118,#115303,#115304) ;
#95879=AXIS2_PLACEMENT_3D('',#148119,#115305,#115306) ;
#95880=AXIS2_PLACEMENT_3D('',#148120,#115307,#115308) ;
#95881=AXIS2_PLACEMENT_3D('',#148121,#115309,#115310) ;
#95882=AXIS2_PLACEMENT_3D('',#148122,#115311,#115312) ;
#95883=AXIS2_PLACEMENT_3D('',#148123,#115313,#115314) ;
#95884=AXIS2_PLACEMENT_3D('',#148124,#115315,#115316) ;
#95885=AXIS2_PLACEMENT_3D('',#148125,#115317,#115318) ;
#95886=AXIS2_PLACEMENT_3D('',#148126,#115319,#115320) ;
#95887=AXIS2_PLACEMENT_3D('',#148127,#115321,#115322) ;
#95888=AXIS2_PLACEMENT_3D('',#148128,#115323,#115324) ;
#95889=AXIS2_PLACEMENT_3D('',#148131,#115326,#115327) ;
#95890=AXIS2_PLACEMENT_3D('',#148132,#115328,#115329) ;
#95891=AXIS2_PLACEMENT_3D('',#148133,#115330,#115331) ;
#95892=AXIS2_PLACEMENT_3D('',#148134,#115332,#115333) ;
#95893=AXIS2_PLACEMENT_3D('',#148135,#115334,#115335) ;
#95894=AXIS2_PLACEMENT_3D('',#148136,#115336,#115337) ;
#95895=AXIS2_PLACEMENT_3D('',#148137,#115338,#115339) ;
#95896=AXIS2_PLACEMENT_3D('',#148138,#115340,#115341) ;
#95897=AXIS2_PLACEMENT_3D('',#148139,#115342,#115343) ;
#95898=AXIS2_PLACEMENT_3D('',#148140,#115344,#115345) ;
#95899=AXIS2_PLACEMENT_3D('',#148141,#115346,#115347) ;
#95900=AXIS2_PLACEMENT_3D('',#148142,#115348,#115349) ;
#95901=AXIS2_PLACEMENT_3D('',#148143,#115350,#115351) ;
#95902=AXIS2_PLACEMENT_3D('',#148145,#115352,#115353) ;
#95903=AXIS2_PLACEMENT_3D('',#148146,#115354,#115355) ;
#95904=AXIS2_PLACEMENT_3D('',#148147,#115356,#115357) ;
#95905=AXIS2_PLACEMENT_3D('',#148148,#115358,#115359) ;
#95906=AXIS2_PLACEMENT_3D('',#148149,#115360,#115361) ;
#95907=AXIS2_PLACEMENT_3D('',#148150,#115362,#115363) ;
#95908=AXIS2_PLACEMENT_3D('',#148151,#115364,#115365) ;
#95909=AXIS2_PLACEMENT_3D('',#148152,#115366,#115367) ;
#95910=AXIS2_PLACEMENT_3D('',#148153,#115368,#115369) ;
#95911=AXIS2_PLACEMENT_3D('',#148154,#115370,#115371) ;
#95912=AXIS2_PLACEMENT_3D('',#148155,#115372,#115373) ;
#95913=AXIS2_PLACEMENT_3D('',#148157,#115375,#115376) ;
#95914=AXIS2_PLACEMENT_3D('',#148158,#115377,#115378) ;
#95915=AXIS2_PLACEMENT_3D('',#148159,#115379,#115380) ;
#95916=AXIS2_PLACEMENT_3D('',#148160,#115381,#115382) ;
#95917=AXIS2_PLACEMENT_3D('',#148161,#115383,#115384) ;
#95918=AXIS2_PLACEMENT_3D('',#148162,#115385,#115386) ;
#95919=AXIS2_PLACEMENT_3D('',#148163,#115387,#115388) ;
#95920=AXIS2_PLACEMENT_3D('',#148164,#115389,#115390) ;
#95921=AXIS2_PLACEMENT_3D('',#148165,#115391,#115392) ;
#95922=AXIS2_PLACEMENT_3D('',#148166,#115393,#115394) ;
#95923=AXIS2_PLACEMENT_3D('',#148167,#115395,#115396) ;
#95924=AXIS2_PLACEMENT_3D('',#148168,#115397,#115398) ;
#95925=AXIS2_PLACEMENT_3D('',#148169,#115399,#115400) ;
#95926=AXIS2_PLACEMENT_3D('',#148170,#115401,#115402) ;
#95927=AXIS2_PLACEMENT_3D('',#148171,#115403,#115404) ;
#95928=AXIS2_PLACEMENT_3D('',#148172,#115405,#115406) ;
#95929=AXIS2_PLACEMENT_3D('',#148173,#115407,#115408) ;
#95930=AXIS2_PLACEMENT_3D('',#148174,#115409,#115410) ;
#95931=AXIS2_PLACEMENT_3D('',#148175,#115411,#115412) ;
#95932=AXIS2_PLACEMENT_3D('',#148176,#115413,#115414) ;
#95933=AXIS2_PLACEMENT_3D('',#148177,#115415,#115416) ;
#95934=AXIS2_PLACEMENT_3D('',#148178,#115417,#115418) ;
#95935=AXIS2_PLACEMENT_3D('',#148179,#115419,#115420) ;
#95936=AXIS2_PLACEMENT_3D('',#148180,#115421,#115422) ;
#95937=AXIS2_PLACEMENT_3D('',#148181,#115423,#115424) ;
#95938=AXIS2_PLACEMENT_3D('',#148182,#115425,#115426) ;
#95939=AXIS2_PLACEMENT_3D('',#148183,#115427,#115428) ;
#95940=AXIS2_PLACEMENT_3D('',#148184,#115429,#115430) ;
#95941=AXIS2_PLACEMENT_3D('',#148185,#115431,#115432) ;
#95942=AXIS2_PLACEMENT_3D('',#148186,#115433,#115434) ;
#95943=AXIS2_PLACEMENT_3D('',#148187,#115435,#115436) ;
#95944=AXIS2_PLACEMENT_3D('',#148188,#115437,#115438) ;
#95945=AXIS2_PLACEMENT_3D('',#148189,#115439,#115440) ;
#95946=AXIS2_PLACEMENT_3D('',#148190,#115441,#115442) ;
#95947=AXIS2_PLACEMENT_3D('',#148191,#115443,#115444) ;
#95948=AXIS2_PLACEMENT_3D('',#148192,#115445,#115446) ;
#95949=AXIS2_PLACEMENT_3D('',#148193,#115447,#115448) ;
#95950=AXIS2_PLACEMENT_3D('',#148194,#115449,#115450) ;
#95951=AXIS2_PLACEMENT_3D('',#148195,#115451,#115452) ;
#95952=AXIS2_PLACEMENT_3D('',#148196,#115453,#115454) ;
#95953=AXIS2_PLACEMENT_3D('',#148197,#115455,#115456) ;
#95954=AXIS2_PLACEMENT_3D('',#148198,#115457,#115458) ;
#95955=AXIS2_PLACEMENT_3D('',#148199,#115459,#115460) ;
#95956=AXIS2_PLACEMENT_3D('',#148200,#115461,#115462) ;
#95957=AXIS2_PLACEMENT_3D('',#148201,#115463,#115464) ;
#95958=AXIS2_PLACEMENT_3D('',#148202,#115465,#115466) ;
#95959=AXIS2_PLACEMENT_3D('',#148203,#115467,#115468) ;
#95960=AXIS2_PLACEMENT_3D('',#148204,#115469,#115470) ;
#95961=AXIS2_PLACEMENT_3D('',#148205,#115471,#115472) ;
#95962=AXIS2_PLACEMENT_3D('',#148206,#115473,#115474) ;
#95963=AXIS2_PLACEMENT_3D('',#148207,#115475,#115476) ;
#95964=AXIS2_PLACEMENT_3D('',#148208,#115477,#115478) ;
#95965=AXIS2_PLACEMENT_3D('',#148209,#115479,#115480) ;
#95966=AXIS2_PLACEMENT_3D('',#148210,#115481,#115482) ;
#95967=AXIS2_PLACEMENT_3D('',#148211,#115483,#115484) ;
#95968=AXIS2_PLACEMENT_3D('',#148212,#115485,#115486) ;
#95969=AXIS2_PLACEMENT_3D('',#148213,#115487,#115488) ;
#95970=AXIS2_PLACEMENT_3D('',#148214,#115489,#115490) ;
#95971=AXIS2_PLACEMENT_3D('',#148215,#115491,#115492) ;
#95972=AXIS2_PLACEMENT_3D('',#148216,#115493,#115494) ;
#95973=AXIS2_PLACEMENT_3D('',#148217,#115495,#115496) ;
#95974=AXIS2_PLACEMENT_3D('',#148218,#115497,#115498) ;
#95975=AXIS2_PLACEMENT_3D('',#148219,#115499,#115500) ;
#95976=AXIS2_PLACEMENT_3D('',#148220,#115501,#115502) ;
#95977=AXIS2_PLACEMENT_3D('',#148221,#115503,#115504) ;
#95978=AXIS2_PLACEMENT_3D('',#148222,#115505,#115506) ;
#95979=AXIS2_PLACEMENT_3D('',#148223,#115507,#115508) ;
#95980=AXIS2_PLACEMENT_3D('',#148225,#115509,#115510) ;
#95981=AXIS2_PLACEMENT_3D('',#148226,#115511,#115512) ;
#95982=AXIS2_PLACEMENT_3D('',#148227,#115513,#115514) ;
#95983=AXIS2_PLACEMENT_3D('',#148228,#115515,#115516) ;
#95984=AXIS2_PLACEMENT_3D('',#148229,#115517,#115518) ;
#95985=AXIS2_PLACEMENT_3D('',#148230,#115519,#115520) ;
#95986=AXIS2_PLACEMENT_3D('',#148231,#115521,#115522) ;
#95987=AXIS2_PLACEMENT_3D('',#148232,#115523,#115524) ;
#95988=AXIS2_PLACEMENT_3D('',#148233,#115525,#115526) ;
#95989=AXIS2_PLACEMENT_3D('',#148244,#115528,#115529) ;
#95990=AXIS2_PLACEMENT_3D('',#148301,#115531,#115532) ;
#95991=AXIS2_PLACEMENT_3D('',#148302,#115533,#115534) ;
#95992=AXIS2_PLACEMENT_3D('',#148303,#115535,#115536) ;
#95993=AXIS2_PLACEMENT_3D('',#148304,#115537,#115538) ;
#95994=AXIS2_PLACEMENT_3D('',#148305,#115539,#115540) ;
#95995=AXIS2_PLACEMENT_3D('',#148306,#115541,#115542) ;
#95996=AXIS2_PLACEMENT_3D('',#148307,#115543,#115544) ;
#95997=AXIS2_PLACEMENT_3D('',#148308,#115545,#115546) ;
#95998=AXIS2_PLACEMENT_3D('',#148309,#115547,#115548) ;
#95999=AXIS2_PLACEMENT_3D('',#148310,#115549,#115550) ;
#96000=AXIS2_PLACEMENT_3D('',#148311,#115551,#115552) ;
#96001=AXIS2_PLACEMENT_3D('',#148312,#115553,#115554) ;
#96002=AXIS2_PLACEMENT_3D('',#148313,#115555,#115556) ;
#96003=AXIS2_PLACEMENT_3D('',#148314,#115557,#115558) ;
#96004=AXIS2_PLACEMENT_3D('',#148315,#115559,#115560) ;
#96005=AXIS2_PLACEMENT_3D('',#148316,#115561,#115562) ;
#96006=AXIS2_PLACEMENT_3D('',#148317,#115563,#115564) ;
#96007=AXIS2_PLACEMENT_3D('',#148318,#115565,#115566) ;
#96008=AXIS2_PLACEMENT_3D('',#148319,#115567,#115568) ;
#96009=AXIS2_PLACEMENT_3D('',#148320,#115569,#115570) ;
#96010=AXIS2_PLACEMENT_3D('',#148321,#115571,#115572) ;
#96011=AXIS2_PLACEMENT_3D('',#148322,#115573,#115574) ;
#96012=AXIS2_PLACEMENT_3D('',#148323,#115575,#115576) ;
#96013=AXIS2_PLACEMENT_3D('',#148326,#115578,#115579) ;
#96014=AXIS2_PLACEMENT_3D('',#148327,#115580,#115581) ;
#96015=AXIS2_PLACEMENT_3D('',#148328,#115582,#115583) ;
#96016=AXIS2_PLACEMENT_3D('',#148329,#115584,#115585) ;
#96017=AXIS2_PLACEMENT_3D('',#148330,#115586,#115587) ;
#96018=AXIS2_PLACEMENT_3D('',#148331,#115588,#115589) ;
#96019=AXIS2_PLACEMENT_3D('',#148332,#115590,#115591) ;
#96020=AXIS2_PLACEMENT_3D('',#148333,#115592,#115593) ;
#96021=AXIS2_PLACEMENT_3D('',#148334,#115594,#115595) ;
#96022=AXIS2_PLACEMENT_3D('',#148335,#115596,#115597) ;
#96023=AXIS2_PLACEMENT_3D('',#148336,#115598,#115599) ;
#96024=AXIS2_PLACEMENT_3D('',#148337,#115600,#115601) ;
#96025=AXIS2_PLACEMENT_3D('',#148338,#115602,#115603) ;
#96026=AXIS2_PLACEMENT_3D('',#148339,#115604,#115605) ;
#96027=AXIS2_PLACEMENT_3D('',#148340,#115606,#115607) ;
#96028=AXIS2_PLACEMENT_3D('',#148341,#115608,#115609) ;
#96029=AXIS2_PLACEMENT_3D('',#148343,#115610,#115611) ;
#96030=AXIS2_PLACEMENT_3D('',#148344,#115612,#115613) ;
#96031=AXIS2_PLACEMENT_3D('',#148345,#115614,#115615) ;
#96032=AXIS2_PLACEMENT_3D('',#148346,#115616,#115617) ;
#96033=AXIS2_PLACEMENT_3D('',#148347,#115618,#115619) ;
#96034=AXIS2_PLACEMENT_3D('',#148348,#115620,#115621) ;
#96035=AXIS2_PLACEMENT_3D('',#148349,#115622,#115623) ;
#96036=AXIS2_PLACEMENT_3D('',#148350,#115624,#115625) ;
#96037=AXIS2_PLACEMENT_3D('',#148351,#115626,#115627) ;
#96038=AXIS2_PLACEMENT_3D('',#148352,#115628,#115629) ;
#96039=AXIS2_PLACEMENT_3D('',#148353,#115630,#115631) ;
#96040=AXIS2_PLACEMENT_3D('',#148354,#115632,#115633) ;
#96041=AXIS2_PLACEMENT_3D('',#148355,#115634,#115635) ;
#96042=AXIS2_PLACEMENT_3D('',#148358,#115637,#115638) ;
#96043=AXIS2_PLACEMENT_3D('',#148359,#115639,#115640) ;
#96044=AXIS2_PLACEMENT_3D('',#148360,#115641,#115642) ;
#96045=AXIS2_PLACEMENT_3D('',#148361,#115643,#115644) ;
#96046=AXIS2_PLACEMENT_3D('',#148362,#115645,#115646) ;
#96047=AXIS2_PLACEMENT_3D('',#148363,#115647,#115648) ;
#96048=AXIS2_PLACEMENT_3D('',#148364,#115649,#115650) ;
#96049=AXIS2_PLACEMENT_3D('',#148365,#115651,#115652) ;
#96050=AXIS2_PLACEMENT_3D('',#148366,#115653,#115654) ;
#96051=AXIS2_PLACEMENT_3D('',#148367,#115655,#115656) ;
#96052=AXIS2_PLACEMENT_3D('',#148368,#115657,#115658) ;
#96053=AXIS2_PLACEMENT_3D('',#148369,#115659,#115660) ;
#96054=AXIS2_PLACEMENT_3D('',#148370,#115661,#115662) ;
#96055=AXIS2_PLACEMENT_3D('',#148372,#115663,#115664) ;
#96056=AXIS2_PLACEMENT_3D('',#148373,#115665,#115666) ;
#96057=AXIS2_PLACEMENT_3D('',#148374,#115667,#115668) ;
#96058=AXIS2_PLACEMENT_3D('',#148375,#115669,#115670) ;
#96059=AXIS2_PLACEMENT_3D('',#148376,#115671,#115672) ;
#96060=AXIS2_PLACEMENT_3D('',#148377,#115673,#115674) ;
#96061=AXIS2_PLACEMENT_3D('',#148378,#115675,#115676) ;
#96062=AXIS2_PLACEMENT_3D('',#148379,#115677,#115678) ;
#96063=AXIS2_PLACEMENT_3D('',#148380,#115679,#115680) ;
#96064=AXIS2_PLACEMENT_3D('',#148381,#115681,#115682) ;
#96065=AXIS2_PLACEMENT_3D('',#148382,#115683,#115684) ;
#96066=AXIS2_PLACEMENT_3D('',#148384,#115686,#115687) ;
#96067=AXIS2_PLACEMENT_3D('',#148385,#115688,#115689) ;
#96068=AXIS2_PLACEMENT_3D('',#148386,#115690,#115691) ;
#96069=AXIS2_PLACEMENT_3D('',#148387,#115692,#115693) ;
#96070=AXIS2_PLACEMENT_3D('',#148388,#115694,#115695) ;
#96071=AXIS2_PLACEMENT_3D('',#148389,#115696,#115697) ;
#96072=AXIS2_PLACEMENT_3D('',#148390,#115698,#115699) ;
#96073=AXIS2_PLACEMENT_3D('',#148391,#115700,#115701) ;
#96074=AXIS2_PLACEMENT_3D('',#148392,#115702,#115703) ;
#96075=AXIS2_PLACEMENT_3D('',#148393,#115704,#115705) ;
#96076=AXIS2_PLACEMENT_3D('',#148394,#115706,#115707) ;
#96077=AXIS2_PLACEMENT_3D('',#148395,#115708,#115709) ;
#96078=AXIS2_PLACEMENT_3D('',#148396,#115710,#115711) ;
#96079=AXIS2_PLACEMENT_3D('',#148397,#115712,#115713) ;
#96080=AXIS2_PLACEMENT_3D('',#148398,#115714,#115715) ;
#96081=AXIS2_PLACEMENT_3D('',#148399,#115716,#115717) ;
#96082=AXIS2_PLACEMENT_3D('',#148400,#115718,#115719) ;
#96083=AXIS2_PLACEMENT_3D('',#148401,#115720,#115721) ;
#96084=AXIS2_PLACEMENT_3D('',#148402,#115722,#115723) ;
#96085=AXIS2_PLACEMENT_3D('',#148403,#115724,#115725) ;
#96086=AXIS2_PLACEMENT_3D('',#148404,#115726,#115727) ;
#96087=AXIS2_PLACEMENT_3D('',#148405,#115728,#115729) ;
#96088=AXIS2_PLACEMENT_3D('',#148406,#115730,#115731) ;
#96089=AXIS2_PLACEMENT_3D('',#148407,#115732,#115733) ;
#96090=AXIS2_PLACEMENT_3D('',#148408,#115734,#115735) ;
#96091=AXIS2_PLACEMENT_3D('',#148409,#115736,#115737) ;
#96092=AXIS2_PLACEMENT_3D('',#148410,#115738,#115739) ;
#96093=AXIS2_PLACEMENT_3D('',#148411,#115740,#115741) ;
#96094=AXIS2_PLACEMENT_3D('',#148412,#115742,#115743) ;
#96095=AXIS2_PLACEMENT_3D('',#148413,#115744,#115745) ;
#96096=AXIS2_PLACEMENT_3D('',#148414,#115746,#115747) ;
#96097=AXIS2_PLACEMENT_3D('',#148415,#115748,#115749) ;
#96098=AXIS2_PLACEMENT_3D('',#148416,#115750,#115751) ;
#96099=AXIS2_PLACEMENT_3D('',#148417,#115752,#115753) ;
#96100=AXIS2_PLACEMENT_3D('',#148418,#115754,#115755) ;
#96101=AXIS2_PLACEMENT_3D('',#148419,#115756,#115757) ;
#96102=AXIS2_PLACEMENT_3D('',#148420,#115758,#115759) ;
#96103=AXIS2_PLACEMENT_3D('',#148421,#115760,#115761) ;
#96104=AXIS2_PLACEMENT_3D('',#148422,#115762,#115763) ;
#96105=AXIS2_PLACEMENT_3D('',#148423,#115764,#115765) ;
#96106=AXIS2_PLACEMENT_3D('',#148424,#115766,#115767) ;
#96107=AXIS2_PLACEMENT_3D('',#148425,#115768,#115769) ;
#96108=AXIS2_PLACEMENT_3D('',#148426,#115770,#115771) ;
#96109=AXIS2_PLACEMENT_3D('',#148427,#115772,#115773) ;
#96110=AXIS2_PLACEMENT_3D('',#148428,#115774,#115775) ;
#96111=AXIS2_PLACEMENT_3D('',#148429,#115776,#115777) ;
#96112=AXIS2_PLACEMENT_3D('',#148430,#115778,#115779) ;
#96113=AXIS2_PLACEMENT_3D('',#148431,#115780,#115781) ;
#96114=AXIS2_PLACEMENT_3D('',#148432,#115782,#115783) ;
#96115=AXIS2_PLACEMENT_3D('',#148433,#115784,#115785) ;
#96116=AXIS2_PLACEMENT_3D('',#148434,#115786,#115787) ;
#96117=AXIS2_PLACEMENT_3D('',#148435,#115788,#115789) ;
#96118=AXIS2_PLACEMENT_3D('',#148436,#115790,#115791) ;
#96119=AXIS2_PLACEMENT_3D('',#148437,#115792,#115793) ;
#96120=AXIS2_PLACEMENT_3D('',#148438,#115794,#115795) ;
#96121=AXIS2_PLACEMENT_3D('',#148439,#115796,#115797) ;
#96122=AXIS2_PLACEMENT_3D('',#148440,#115798,#115799) ;
#96123=AXIS2_PLACEMENT_3D('',#148441,#115800,#115801) ;
#96124=AXIS2_PLACEMENT_3D('',#148442,#115802,#115803) ;
#96125=AXIS2_PLACEMENT_3D('',#148443,#115804,#115805) ;
#96126=AXIS2_PLACEMENT_3D('',#148444,#115806,#115807) ;
#96127=AXIS2_PLACEMENT_3D('',#148445,#115808,#115809) ;
#96128=AXIS2_PLACEMENT_3D('',#148446,#115810,#115811) ;
#96129=AXIS2_PLACEMENT_3D('',#148447,#115812,#115813) ;
#96130=AXIS2_PLACEMENT_3D('',#148448,#115814,#115815) ;
#96131=AXIS2_PLACEMENT_3D('',#148449,#115816,#115817) ;
#96132=AXIS2_PLACEMENT_3D('',#148450,#115818,#115819) ;
#96133=AXIS2_PLACEMENT_3D('',#148452,#115820,#115821) ;
#96134=AXIS2_PLACEMENT_3D('',#148453,#115822,#115823) ;
#96135=AXIS2_PLACEMENT_3D('',#148454,#115824,#115825) ;
#96136=AXIS2_PLACEMENT_3D('',#148455,#115826,#115827) ;
#96137=AXIS2_PLACEMENT_3D('',#148456,#115828,#115829) ;
#96138=AXIS2_PLACEMENT_3D('',#148457,#115830,#115831) ;
#96139=AXIS2_PLACEMENT_3D('',#148458,#115832,#115833) ;
#96140=AXIS2_PLACEMENT_3D('',#148459,#115834,#115835) ;
#96141=AXIS2_PLACEMENT_3D('',#148460,#115836,#115837) ;
#96142=AXIS2_PLACEMENT_3D('',#148471,#115839,#115840) ;
#96143=AXIS2_PLACEMENT_3D('',#148528,#115842,#115843) ;
#96144=AXIS2_PLACEMENT_3D('',#148529,#115844,#115845) ;
#96145=AXIS2_PLACEMENT_3D('',#148530,#115846,#115847) ;
#96146=AXIS2_PLACEMENT_3D('',#148531,#115848,#115849) ;
#96147=AXIS2_PLACEMENT_3D('',#148532,#115850,#115851) ;
#96148=AXIS2_PLACEMENT_3D('',#148533,#115852,#115853) ;
#96149=AXIS2_PLACEMENT_3D('',#148534,#115854,#115855) ;
#96150=AXIS2_PLACEMENT_3D('',#148535,#115856,#115857) ;
#96151=AXIS2_PLACEMENT_3D('',#148536,#115858,#115859) ;
#96152=AXIS2_PLACEMENT_3D('',#148537,#115860,#115861) ;
#96153=AXIS2_PLACEMENT_3D('',#148538,#115862,#115863) ;
#96154=AXIS2_PLACEMENT_3D('',#148539,#115864,#115865) ;
#96155=AXIS2_PLACEMENT_3D('',#148540,#115866,#115867) ;
#96156=AXIS2_PLACEMENT_3D('',#148541,#115868,#115869) ;
#96157=AXIS2_PLACEMENT_3D('',#148542,#115870,#115871) ;
#96158=AXIS2_PLACEMENT_3D('',#148543,#115872,#115873) ;
#96159=AXIS2_PLACEMENT_3D('',#148544,#115874,#115875) ;
#96160=AXIS2_PLACEMENT_3D('',#148545,#115876,#115877) ;
#96161=AXIS2_PLACEMENT_3D('',#148546,#115878,#115879) ;
#96162=AXIS2_PLACEMENT_3D('',#148547,#115880,#115881) ;
#96163=AXIS2_PLACEMENT_3D('',#148548,#115882,#115883) ;
#96164=AXIS2_PLACEMENT_3D('',#148549,#115884,#115885) ;
#96165=AXIS2_PLACEMENT_3D('',#148550,#115886,#115887) ;
#96166=AXIS2_PLACEMENT_3D('',#148553,#115889,#115890) ;
#96167=AXIS2_PLACEMENT_3D('',#148554,#115891,#115892) ;
#96168=AXIS2_PLACEMENT_3D('',#148555,#115893,#115894) ;
#96169=AXIS2_PLACEMENT_3D('',#148556,#115895,#115896) ;
#96170=AXIS2_PLACEMENT_3D('',#148557,#115897,#115898) ;
#96171=AXIS2_PLACEMENT_3D('',#148558,#115899,#115900) ;
#96172=AXIS2_PLACEMENT_3D('',#148559,#115901,#115902) ;
#96173=AXIS2_PLACEMENT_3D('',#148560,#115903,#115904) ;
#96174=AXIS2_PLACEMENT_3D('',#148561,#115905,#115906) ;
#96175=AXIS2_PLACEMENT_3D('',#148562,#115907,#115908) ;
#96176=AXIS2_PLACEMENT_3D('',#148563,#115909,#115910) ;
#96177=AXIS2_PLACEMENT_3D('',#148564,#115911,#115912) ;
#96178=AXIS2_PLACEMENT_3D('',#148565,#115913,#115914) ;
#96179=AXIS2_PLACEMENT_3D('',#148566,#115915,#115916) ;
#96180=AXIS2_PLACEMENT_3D('',#148567,#115917,#115918) ;
#96181=AXIS2_PLACEMENT_3D('',#148568,#115919,#115920) ;
#96182=AXIS2_PLACEMENT_3D('',#148570,#115921,#115922) ;
#96183=AXIS2_PLACEMENT_3D('',#148571,#115923,#115924) ;
#96184=AXIS2_PLACEMENT_3D('',#148572,#115925,#115926) ;
#96185=AXIS2_PLACEMENT_3D('',#148573,#115927,#115928) ;
#96186=AXIS2_PLACEMENT_3D('',#148574,#115929,#115930) ;
#96187=AXIS2_PLACEMENT_3D('',#148575,#115931,#115932) ;
#96188=AXIS2_PLACEMENT_3D('',#148576,#115933,#115934) ;
#96189=AXIS2_PLACEMENT_3D('',#148577,#115935,#115936) ;
#96190=AXIS2_PLACEMENT_3D('',#148578,#115937,#115938) ;
#96191=AXIS2_PLACEMENT_3D('',#148579,#115939,#115940) ;
#96192=AXIS2_PLACEMENT_3D('',#148580,#115941,#115942) ;
#96193=AXIS2_PLACEMENT_3D('',#148581,#115943,#115944) ;
#96194=AXIS2_PLACEMENT_3D('',#148582,#115945,#115946) ;
#96195=AXIS2_PLACEMENT_3D('',#148585,#115948,#115949) ;
#96196=AXIS2_PLACEMENT_3D('',#148586,#115950,#115951) ;
#96197=AXIS2_PLACEMENT_3D('',#148587,#115952,#115953) ;
#96198=AXIS2_PLACEMENT_3D('',#148588,#115954,#115955) ;
#96199=AXIS2_PLACEMENT_3D('',#148589,#115956,#115957) ;
#96200=AXIS2_PLACEMENT_3D('',#148590,#115958,#115959) ;
#96201=AXIS2_PLACEMENT_3D('',#148591,#115960,#115961) ;
#96202=AXIS2_PLACEMENT_3D('',#148592,#115962,#115963) ;
#96203=AXIS2_PLACEMENT_3D('',#148593,#115964,#115965) ;
#96204=AXIS2_PLACEMENT_3D('',#148594,#115966,#115967) ;
#96205=AXIS2_PLACEMENT_3D('',#148595,#115968,#115969) ;
#96206=AXIS2_PLACEMENT_3D('',#148596,#115970,#115971) ;
#96207=AXIS2_PLACEMENT_3D('',#148597,#115972,#115973) ;
#96208=AXIS2_PLACEMENT_3D('',#148599,#115974,#115975) ;
#96209=AXIS2_PLACEMENT_3D('',#148600,#115976,#115977) ;
#96210=AXIS2_PLACEMENT_3D('',#148601,#115978,#115979) ;
#96211=AXIS2_PLACEMENT_3D('',#148602,#115980,#115981) ;
#96212=AXIS2_PLACEMENT_3D('',#148603,#115982,#115983) ;
#96213=AXIS2_PLACEMENT_3D('',#148604,#115984,#115985) ;
#96214=AXIS2_PLACEMENT_3D('',#148605,#115986,#115987) ;
#96215=AXIS2_PLACEMENT_3D('',#148606,#115988,#115989) ;
#96216=AXIS2_PLACEMENT_3D('',#148607,#115990,#115991) ;
#96217=AXIS2_PLACEMENT_3D('',#148608,#115992,#115993) ;
#96218=AXIS2_PLACEMENT_3D('',#148609,#115994,#115995) ;
#96219=AXIS2_PLACEMENT_3D('',#148611,#115997,#115998) ;
#96220=AXIS2_PLACEMENT_3D('',#148612,#115999,#116000) ;
#96221=AXIS2_PLACEMENT_3D('',#148613,#116001,#116002) ;
#96222=AXIS2_PLACEMENT_3D('',#148614,#116003,#116004) ;
#96223=AXIS2_PLACEMENT_3D('',#148615,#116005,#116006) ;
#96224=AXIS2_PLACEMENT_3D('',#148616,#116007,#116008) ;
#96225=AXIS2_PLACEMENT_3D('',#148617,#116009,#116010) ;
#96226=AXIS2_PLACEMENT_3D('',#148618,#116011,#116012) ;
#96227=AXIS2_PLACEMENT_3D('',#148619,#116013,#116014) ;
#96228=AXIS2_PLACEMENT_3D('',#148620,#116015,#116016) ;
#96229=AXIS2_PLACEMENT_3D('',#148621,#116017,#116018) ;
#96230=AXIS2_PLACEMENT_3D('',#148622,#116019,#116020) ;
#96231=AXIS2_PLACEMENT_3D('',#148623,#116021,#116022) ;
#96232=AXIS2_PLACEMENT_3D('',#148624,#116023,#116024) ;
#96233=AXIS2_PLACEMENT_3D('',#148625,#116025,#116026) ;
#96234=AXIS2_PLACEMENT_3D('',#148626,#116027,#116028) ;
#96235=AXIS2_PLACEMENT_3D('',#148627,#116029,#116030) ;
#96236=AXIS2_PLACEMENT_3D('',#148628,#116031,#116032) ;
#96237=AXIS2_PLACEMENT_3D('',#148629,#116033,#116034) ;
#96238=AXIS2_PLACEMENT_3D('',#148630,#116035,#116036) ;
#96239=AXIS2_PLACEMENT_3D('',#148631,#116037,#116038) ;
#96240=AXIS2_PLACEMENT_3D('',#148632,#116039,#116040) ;
#96241=AXIS2_PLACEMENT_3D('',#148633,#116041,#116042) ;
#96242=AXIS2_PLACEMENT_3D('',#148634,#116043,#116044) ;
#96243=AXIS2_PLACEMENT_3D('',#148635,#116045,#116046) ;
#96244=AXIS2_PLACEMENT_3D('',#148636,#116047,#116048) ;
#96245=AXIS2_PLACEMENT_3D('',#148637,#116049,#116050) ;
#96246=AXIS2_PLACEMENT_3D('',#148638,#116051,#116052) ;
#96247=AXIS2_PLACEMENT_3D('',#148639,#116053,#116054) ;
#96248=AXIS2_PLACEMENT_3D('',#148640,#116055,#116056) ;
#96249=AXIS2_PLACEMENT_3D('',#148641,#116057,#116058) ;
#96250=AXIS2_PLACEMENT_3D('',#148642,#116059,#116060) ;
#96251=AXIS2_PLACEMENT_3D('',#148643,#116061,#116062) ;
#96252=AXIS2_PLACEMENT_3D('',#148644,#116063,#116064) ;
#96253=AXIS2_PLACEMENT_3D('',#148645,#116065,#116066) ;
#96254=AXIS2_PLACEMENT_3D('',#148646,#116067,#116068) ;
#96255=AXIS2_PLACEMENT_3D('',#148647,#116069,#116070) ;
#96256=AXIS2_PLACEMENT_3D('',#148648,#116071,#116072) ;
#96257=AXIS2_PLACEMENT_3D('',#148649,#116073,#116074) ;
#96258=AXIS2_PLACEMENT_3D('',#148650,#116075,#116076) ;
#96259=AXIS2_PLACEMENT_3D('',#148651,#116077,#116078) ;
#96260=AXIS2_PLACEMENT_3D('',#148652,#116079,#116080) ;
#96261=AXIS2_PLACEMENT_3D('',#148653,#116081,#116082) ;
#96262=AXIS2_PLACEMENT_3D('',#148654,#116083,#116084) ;
#96263=AXIS2_PLACEMENT_3D('',#148655,#116085,#116086) ;
#96264=AXIS2_PLACEMENT_3D('',#148656,#116087,#116088) ;
#96265=AXIS2_PLACEMENT_3D('',#148657,#116089,#116090) ;
#96266=AXIS2_PLACEMENT_3D('',#148658,#116091,#116092) ;
#96267=AXIS2_PLACEMENT_3D('',#148659,#116093,#116094) ;
#96268=AXIS2_PLACEMENT_3D('',#148660,#116095,#116096) ;
#96269=AXIS2_PLACEMENT_3D('',#148661,#116097,#116098) ;
#96270=AXIS2_PLACEMENT_3D('',#148662,#116099,#116100) ;
#96271=AXIS2_PLACEMENT_3D('',#148663,#116101,#116102) ;
#96272=AXIS2_PLACEMENT_3D('',#148664,#116103,#116104) ;
#96273=AXIS2_PLACEMENT_3D('',#148665,#116105,#116106) ;
#96274=AXIS2_PLACEMENT_3D('',#148666,#116107,#116108) ;
#96275=AXIS2_PLACEMENT_3D('',#148667,#116109,#116110) ;
#96276=AXIS2_PLACEMENT_3D('',#148668,#116111,#116112) ;
#96277=AXIS2_PLACEMENT_3D('',#148669,#116113,#116114) ;
#96278=AXIS2_PLACEMENT_3D('',#148670,#116115,#116116) ;
#96279=AXIS2_PLACEMENT_3D('',#148671,#116117,#116118) ;
#96280=AXIS2_PLACEMENT_3D('',#148672,#116119,#116120) ;
#96281=AXIS2_PLACEMENT_3D('',#148673,#116121,#116122) ;
#96282=AXIS2_PLACEMENT_3D('',#148674,#116123,#116124) ;
#96283=AXIS2_PLACEMENT_3D('',#148675,#116125,#116126) ;
#96284=AXIS2_PLACEMENT_3D('',#148676,#116127,#116128) ;
#96285=AXIS2_PLACEMENT_3D('',#148677,#116129,#116130) ;
#96286=AXIS2_PLACEMENT_3D('',#148679,#116131,#116132) ;
#96287=AXIS2_PLACEMENT_3D('',#148680,#116133,#116134) ;
#96288=AXIS2_PLACEMENT_3D('',#148681,#116135,#116136) ;
#96289=AXIS2_PLACEMENT_3D('',#148682,#116137,#116138) ;
#96290=AXIS2_PLACEMENT_3D('',#148683,#116139,#116140) ;
#96291=AXIS2_PLACEMENT_3D('',#148684,#116141,#116142) ;
#96292=AXIS2_PLACEMENT_3D('',#148685,#116143,#116144) ;
#96293=AXIS2_PLACEMENT_3D('',#148686,#116145,#116146) ;
#96294=AXIS2_PLACEMENT_3D('',#148687,#116147,#116148) ;
#96295=AXIS2_PLACEMENT_3D('',#148698,#116150,#116151) ;
#96296=AXIS2_PLACEMENT_3D('',#148755,#116153,#116154) ;
#96297=AXIS2_PLACEMENT_3D('',#148756,#116155,#116156) ;
#96298=AXIS2_PLACEMENT_3D('',#148757,#116157,#116158) ;
#96299=AXIS2_PLACEMENT_3D('',#148758,#116159,#116160) ;
#96300=AXIS2_PLACEMENT_3D('',#148759,#116161,#116162) ;
#96301=AXIS2_PLACEMENT_3D('',#148760,#116163,#116164) ;
#96302=AXIS2_PLACEMENT_3D('',#148761,#116165,#116166) ;
#96303=AXIS2_PLACEMENT_3D('',#148762,#116167,#116168) ;
#96304=AXIS2_PLACEMENT_3D('',#148763,#116169,#116170) ;
#96305=AXIS2_PLACEMENT_3D('',#148764,#116171,#116172) ;
#96306=AXIS2_PLACEMENT_3D('',#148765,#116173,#116174) ;
#96307=AXIS2_PLACEMENT_3D('',#148766,#116175,#116176) ;
#96308=AXIS2_PLACEMENT_3D('',#148767,#116177,#116178) ;
#96309=AXIS2_PLACEMENT_3D('',#148768,#116179,#116180) ;
#96310=AXIS2_PLACEMENT_3D('',#148769,#116181,#116182) ;
#96311=AXIS2_PLACEMENT_3D('',#148770,#116183,#116184) ;
#96312=AXIS2_PLACEMENT_3D('',#148771,#116185,#116186) ;
#96313=AXIS2_PLACEMENT_3D('',#148772,#116187,#116188) ;
#96314=AXIS2_PLACEMENT_3D('',#148773,#116189,#116190) ;
#96315=AXIS2_PLACEMENT_3D('',#148774,#116191,#116192) ;
#96316=AXIS2_PLACEMENT_3D('',#148775,#116193,#116194) ;
#96317=AXIS2_PLACEMENT_3D('',#148776,#116195,#116196) ;
#96318=AXIS2_PLACEMENT_3D('',#148777,#116197,#116198) ;
#96319=AXIS2_PLACEMENT_3D('',#148780,#116200,#116201) ;
#96320=AXIS2_PLACEMENT_3D('',#148781,#116202,#116203) ;
#96321=AXIS2_PLACEMENT_3D('',#148782,#116204,#116205) ;
#96322=AXIS2_PLACEMENT_3D('',#148783,#116206,#116207) ;
#96323=AXIS2_PLACEMENT_3D('',#148784,#116208,#116209) ;
#96324=AXIS2_PLACEMENT_3D('',#148785,#116210,#116211) ;
#96325=AXIS2_PLACEMENT_3D('',#148786,#116212,#116213) ;
#96326=AXIS2_PLACEMENT_3D('',#148787,#116214,#116215) ;
#96327=AXIS2_PLACEMENT_3D('',#148788,#116216,#116217) ;
#96328=AXIS2_PLACEMENT_3D('',#148789,#116218,#116219) ;
#96329=AXIS2_PLACEMENT_3D('',#148790,#116220,#116221) ;
#96330=AXIS2_PLACEMENT_3D('',#148791,#116222,#116223) ;
#96331=AXIS2_PLACEMENT_3D('',#148792,#116224,#116225) ;
#96332=AXIS2_PLACEMENT_3D('',#148793,#116226,#116227) ;
#96333=AXIS2_PLACEMENT_3D('',#148794,#116228,#116229) ;
#96334=AXIS2_PLACEMENT_3D('',#148795,#116230,#116231) ;
#96335=AXIS2_PLACEMENT_3D('',#148797,#116232,#116233) ;
#96336=AXIS2_PLACEMENT_3D('',#148798,#116234,#116235) ;
#96337=AXIS2_PLACEMENT_3D('',#148799,#116236,#116237) ;
#96338=AXIS2_PLACEMENT_3D('',#148800,#116238,#116239) ;
#96339=AXIS2_PLACEMENT_3D('',#148801,#116240,#116241) ;
#96340=AXIS2_PLACEMENT_3D('',#148802,#116242,#116243) ;
#96341=AXIS2_PLACEMENT_3D('',#148803,#116244,#116245) ;
#96342=AXIS2_PLACEMENT_3D('',#148804,#116246,#116247) ;
#96343=AXIS2_PLACEMENT_3D('',#148805,#116248,#116249) ;
#96344=AXIS2_PLACEMENT_3D('',#148806,#116250,#116251) ;
#96345=AXIS2_PLACEMENT_3D('',#148807,#116252,#116253) ;
#96346=AXIS2_PLACEMENT_3D('',#148808,#116254,#116255) ;
#96347=AXIS2_PLACEMENT_3D('',#148809,#116256,#116257) ;
#96348=AXIS2_PLACEMENT_3D('',#148812,#116259,#116260) ;
#96349=AXIS2_PLACEMENT_3D('',#148813,#116261,#116262) ;
#96350=AXIS2_PLACEMENT_3D('',#148814,#116263,#116264) ;
#96351=AXIS2_PLACEMENT_3D('',#148815,#116265,#116266) ;
#96352=AXIS2_PLACEMENT_3D('',#148816,#116267,#116268) ;
#96353=AXIS2_PLACEMENT_3D('',#148817,#116269,#116270) ;
#96354=AXIS2_PLACEMENT_3D('',#148818,#116271,#116272) ;
#96355=AXIS2_PLACEMENT_3D('',#148819,#116273,#116274) ;
#96356=AXIS2_PLACEMENT_3D('',#148820,#116275,#116276) ;
#96357=AXIS2_PLACEMENT_3D('',#148821,#116277,#116278) ;
#96358=AXIS2_PLACEMENT_3D('',#148822,#116279,#116280) ;
#96359=AXIS2_PLACEMENT_3D('',#148823,#116281,#116282) ;
#96360=AXIS2_PLACEMENT_3D('',#148824,#116283,#116284) ;
#96361=AXIS2_PLACEMENT_3D('',#148826,#116285,#116286) ;
#96362=AXIS2_PLACEMENT_3D('',#148827,#116287,#116288) ;
#96363=AXIS2_PLACEMENT_3D('',#148828,#116289,#116290) ;
#96364=AXIS2_PLACEMENT_3D('',#148829,#116291,#116292) ;
#96365=AXIS2_PLACEMENT_3D('',#148830,#116293,#116294) ;
#96366=AXIS2_PLACEMENT_3D('',#148831,#116295,#116296) ;
#96367=AXIS2_PLACEMENT_3D('',#148832,#116297,#116298) ;
#96368=AXIS2_PLACEMENT_3D('',#148833,#116299,#116300) ;
#96369=AXIS2_PLACEMENT_3D('',#148834,#116301,#116302) ;
#96370=AXIS2_PLACEMENT_3D('',#148835,#116303,#116304) ;
#96371=AXIS2_PLACEMENT_3D('',#148836,#116305,#116306) ;
#96372=AXIS2_PLACEMENT_3D('',#148838,#116308,#116309) ;
#96373=AXIS2_PLACEMENT_3D('',#148839,#116310,#116311) ;
#96374=AXIS2_PLACEMENT_3D('',#148840,#116312,#116313) ;
#96375=AXIS2_PLACEMENT_3D('',#148841,#116314,#116315) ;
#96376=AXIS2_PLACEMENT_3D('',#148842,#116316,#116317) ;
#96377=AXIS2_PLACEMENT_3D('',#148843,#116318,#116319) ;
#96378=AXIS2_PLACEMENT_3D('',#148844,#116320,#116321) ;
#96379=AXIS2_PLACEMENT_3D('',#148845,#116322,#116323) ;
#96380=AXIS2_PLACEMENT_3D('',#148846,#116324,#116325) ;
#96381=AXIS2_PLACEMENT_3D('',#148847,#116326,#116327) ;
#96382=AXIS2_PLACEMENT_3D('',#148848,#116328,#116329) ;
#96383=AXIS2_PLACEMENT_3D('',#148849,#116330,#116331) ;
#96384=AXIS2_PLACEMENT_3D('',#148850,#116332,#116333) ;
#96385=AXIS2_PLACEMENT_3D('',#148851,#116334,#116335) ;
#96386=AXIS2_PLACEMENT_3D('',#148852,#116336,#116337) ;
#96387=AXIS2_PLACEMENT_3D('',#148853,#116338,#116339) ;
#96388=AXIS2_PLACEMENT_3D('',#148854,#116340,#116341) ;
#96389=AXIS2_PLACEMENT_3D('',#148855,#116342,#116343) ;
#96390=AXIS2_PLACEMENT_3D('',#148856,#116344,#116345) ;
#96391=AXIS2_PLACEMENT_3D('',#148857,#116346,#116347) ;
#96392=AXIS2_PLACEMENT_3D('',#148858,#116348,#116349) ;
#96393=AXIS2_PLACEMENT_3D('',#148859,#116350,#116351) ;
#96394=AXIS2_PLACEMENT_3D('',#148860,#116352,#116353) ;
#96395=AXIS2_PLACEMENT_3D('',#148861,#116354,#116355) ;
#96396=AXIS2_PLACEMENT_3D('',#148862,#116356,#116357) ;
#96397=AXIS2_PLACEMENT_3D('',#148863,#116358,#116359) ;
#96398=AXIS2_PLACEMENT_3D('',#148864,#116360,#116361) ;
#96399=AXIS2_PLACEMENT_3D('',#148865,#116362,#116363) ;
#96400=AXIS2_PLACEMENT_3D('',#148866,#116364,#116365) ;
#96401=AXIS2_PLACEMENT_3D('',#148867,#116366,#116367) ;
#96402=AXIS2_PLACEMENT_3D('',#148868,#116368,#116369) ;
#96403=AXIS2_PLACEMENT_3D('',#148869,#116370,#116371) ;
#96404=AXIS2_PLACEMENT_3D('',#148870,#116372,#116373) ;
#96405=AXIS2_PLACEMENT_3D('',#148871,#116374,#116375) ;
#96406=AXIS2_PLACEMENT_3D('',#148872,#116376,#116377) ;
#96407=AXIS2_PLACEMENT_3D('',#148873,#116378,#116379) ;
#96408=AXIS2_PLACEMENT_3D('',#148874,#116380,#116381) ;
#96409=AXIS2_PLACEMENT_3D('',#148875,#116382,#116383) ;
#96410=AXIS2_PLACEMENT_3D('',#148876,#116384,#116385) ;
#96411=AXIS2_PLACEMENT_3D('',#148877,#116386,#116387) ;
#96412=AXIS2_PLACEMENT_3D('',#148878,#116388,#116389) ;
#96413=AXIS2_PLACEMENT_3D('',#148879,#116390,#116391) ;
#96414=AXIS2_PLACEMENT_3D('',#148880,#116392,#116393) ;
#96415=AXIS2_PLACEMENT_3D('',#148881,#116394,#116395) ;
#96416=AXIS2_PLACEMENT_3D('',#148882,#116396,#116397) ;
#96417=AXIS2_PLACEMENT_3D('',#148883,#116398,#116399) ;
#96418=AXIS2_PLACEMENT_3D('',#148884,#116400,#116401) ;
#96419=AXIS2_PLACEMENT_3D('',#148885,#116402,#116403) ;
#96420=AXIS2_PLACEMENT_3D('',#148886,#116404,#116405) ;
#96421=AXIS2_PLACEMENT_3D('',#148887,#116406,#116407) ;
#96422=AXIS2_PLACEMENT_3D('',#148888,#116408,#116409) ;
#96423=AXIS2_PLACEMENT_3D('',#148889,#116410,#116411) ;
#96424=AXIS2_PLACEMENT_3D('',#148890,#116412,#116413) ;
#96425=AXIS2_PLACEMENT_3D('',#148891,#116414,#116415) ;
#96426=AXIS2_PLACEMENT_3D('',#148892,#116416,#116417) ;
#96427=AXIS2_PLACEMENT_3D('',#148893,#116418,#116419) ;
#96428=AXIS2_PLACEMENT_3D('',#148894,#116420,#116421) ;
#96429=AXIS2_PLACEMENT_3D('',#148895,#116422,#116423) ;
#96430=AXIS2_PLACEMENT_3D('',#148896,#116424,#116425) ;
#96431=AXIS2_PLACEMENT_3D('',#148897,#116426,#116427) ;
#96432=AXIS2_PLACEMENT_3D('',#148898,#116428,#116429) ;
#96433=AXIS2_PLACEMENT_3D('',#148899,#116430,#116431) ;
#96434=AXIS2_PLACEMENT_3D('',#148900,#116432,#116433) ;
#96435=AXIS2_PLACEMENT_3D('',#148901,#116434,#116435) ;
#96436=AXIS2_PLACEMENT_3D('',#148902,#116436,#116437) ;
#96437=AXIS2_PLACEMENT_3D('',#148903,#116438,#116439) ;
#96438=AXIS2_PLACEMENT_3D('',#148904,#116440,#116441) ;
#96439=AXIS2_PLACEMENT_3D('',#148906,#116442,#116443) ;
#96440=AXIS2_PLACEMENT_3D('',#148907,#116444,#116445) ;
#96441=AXIS2_PLACEMENT_3D('',#148908,#116446,#116447) ;
#96442=AXIS2_PLACEMENT_3D('',#148909,#116448,#116449) ;
#96443=AXIS2_PLACEMENT_3D('',#148910,#116450,#116451) ;
#96444=AXIS2_PLACEMENT_3D('',#148911,#116452,#116453) ;
#96445=AXIS2_PLACEMENT_3D('',#148912,#116454,#116455) ;
#96446=AXIS2_PLACEMENT_3D('',#148913,#116456,#116457) ;
#96447=AXIS2_PLACEMENT_3D('',#148914,#116458,#116459) ;
#96448=AXIS2_PLACEMENT_3D('',#148925,#116461,#116462) ;
#96449=AXIS2_PLACEMENT_3D('',#148982,#116464,#116465) ;
#96450=AXIS2_PLACEMENT_3D('',#148983,#116466,#116467) ;
#96451=AXIS2_PLACEMENT_3D('',#148984,#116468,#116469) ;
#96452=AXIS2_PLACEMENT_3D('',#148985,#116470,#116471) ;
#96453=AXIS2_PLACEMENT_3D('',#148986,#116472,#116473) ;
#96454=AXIS2_PLACEMENT_3D('',#148987,#116474,#116475) ;
#96455=AXIS2_PLACEMENT_3D('',#148988,#116476,#116477) ;
#96456=AXIS2_PLACEMENT_3D('',#148989,#116478,#116479) ;
#96457=AXIS2_PLACEMENT_3D('',#148990,#116480,#116481) ;
#96458=AXIS2_PLACEMENT_3D('',#148991,#116482,#116483) ;
#96459=AXIS2_PLACEMENT_3D('',#148992,#116484,#116485) ;
#96460=AXIS2_PLACEMENT_3D('',#148993,#116486,#116487) ;
#96461=AXIS2_PLACEMENT_3D('',#148994,#116488,#116489) ;
#96462=AXIS2_PLACEMENT_3D('',#148995,#116490,#116491) ;
#96463=AXIS2_PLACEMENT_3D('',#148996,#116492,#116493) ;
#96464=AXIS2_PLACEMENT_3D('',#148997,#116494,#116495) ;
#96465=AXIS2_PLACEMENT_3D('',#148998,#116496,#116497) ;
#96466=AXIS2_PLACEMENT_3D('',#148999,#116498,#116499) ;
#96467=AXIS2_PLACEMENT_3D('',#149000,#116500,#116501) ;
#96468=AXIS2_PLACEMENT_3D('',#149001,#116502,#116503) ;
#96469=AXIS2_PLACEMENT_3D('',#149002,#116504,#116505) ;
#96470=AXIS2_PLACEMENT_3D('',#149003,#116506,#116507) ;
#96471=AXIS2_PLACEMENT_3D('',#149004,#116508,#116509) ;
#96472=AXIS2_PLACEMENT_3D('',#149007,#116511,#116512) ;
#96473=AXIS2_PLACEMENT_3D('',#149008,#116513,#116514) ;
#96474=AXIS2_PLACEMENT_3D('',#149009,#116515,#116516) ;
#96475=AXIS2_PLACEMENT_3D('',#149010,#116517,#116518) ;
#96476=AXIS2_PLACEMENT_3D('',#149011,#116519,#116520) ;
#96477=AXIS2_PLACEMENT_3D('',#149012,#116521,#116522) ;
#96478=AXIS2_PLACEMENT_3D('',#149013,#116523,#116524) ;
#96479=AXIS2_PLACEMENT_3D('',#149014,#116525,#116526) ;
#96480=AXIS2_PLACEMENT_3D('',#149015,#116527,#116528) ;
#96481=AXIS2_PLACEMENT_3D('',#149016,#116529,#116530) ;
#96482=AXIS2_PLACEMENT_3D('',#149017,#116531,#116532) ;
#96483=AXIS2_PLACEMENT_3D('',#149018,#116533,#116534) ;
#96484=AXIS2_PLACEMENT_3D('',#149019,#116535,#116536) ;
#96485=AXIS2_PLACEMENT_3D('',#149020,#116537,#116538) ;
#96486=AXIS2_PLACEMENT_3D('',#149021,#116539,#116540) ;
#96487=AXIS2_PLACEMENT_3D('',#149022,#116541,#116542) ;
#96488=AXIS2_PLACEMENT_3D('',#149024,#116543,#116544) ;
#96489=AXIS2_PLACEMENT_3D('',#149025,#116545,#116546) ;
#96490=AXIS2_PLACEMENT_3D('',#149026,#116547,#116548) ;
#96491=AXIS2_PLACEMENT_3D('',#149027,#116549,#116550) ;
#96492=AXIS2_PLACEMENT_3D('',#149028,#116551,#116552) ;
#96493=AXIS2_PLACEMENT_3D('',#149029,#116553,#116554) ;
#96494=AXIS2_PLACEMENT_3D('',#149030,#116555,#116556) ;
#96495=AXIS2_PLACEMENT_3D('',#149031,#116557,#116558) ;
#96496=AXIS2_PLACEMENT_3D('',#149032,#116559,#116560) ;
#96497=AXIS2_PLACEMENT_3D('',#149033,#116561,#116562) ;
#96498=AXIS2_PLACEMENT_3D('',#149034,#116563,#116564) ;
#96499=AXIS2_PLACEMENT_3D('',#149035,#116565,#116566) ;
#96500=AXIS2_PLACEMENT_3D('',#149036,#116567,#116568) ;
#96501=AXIS2_PLACEMENT_3D('',#149039,#116570,#116571) ;
#96502=AXIS2_PLACEMENT_3D('',#149040,#116572,#116573) ;
#96503=AXIS2_PLACEMENT_3D('',#149041,#116574,#116575) ;
#96504=AXIS2_PLACEMENT_3D('',#149042,#116576,#116577) ;
#96505=AXIS2_PLACEMENT_3D('',#149043,#116578,#116579) ;
#96506=AXIS2_PLACEMENT_3D('',#149044,#116580,#116581) ;
#96507=AXIS2_PLACEMENT_3D('',#149045,#116582,#116583) ;
#96508=AXIS2_PLACEMENT_3D('',#149046,#116584,#116585) ;
#96509=AXIS2_PLACEMENT_3D('',#149047,#116586,#116587) ;
#96510=AXIS2_PLACEMENT_3D('',#149048,#116588,#116589) ;
#96511=AXIS2_PLACEMENT_3D('',#149049,#116590,#116591) ;
#96512=AXIS2_PLACEMENT_3D('',#149050,#116592,#116593) ;
#96513=AXIS2_PLACEMENT_3D('',#149051,#116594,#116595) ;
#96514=AXIS2_PLACEMENT_3D('',#149053,#116596,#116597) ;
#96515=AXIS2_PLACEMENT_3D('',#149054,#116598,#116599) ;
#96516=AXIS2_PLACEMENT_3D('',#149055,#116600,#116601) ;
#96517=AXIS2_PLACEMENT_3D('',#149056,#116602,#116603) ;
#96518=AXIS2_PLACEMENT_3D('',#149057,#116604,#116605) ;
#96519=AXIS2_PLACEMENT_3D('',#149058,#116606,#116607) ;
#96520=AXIS2_PLACEMENT_3D('',#149059,#116608,#116609) ;
#96521=AXIS2_PLACEMENT_3D('',#149060,#116610,#116611) ;
#96522=AXIS2_PLACEMENT_3D('',#149061,#116612,#116613) ;
#96523=AXIS2_PLACEMENT_3D('',#149062,#116614,#116615) ;
#96524=AXIS2_PLACEMENT_3D('',#149063,#116616,#116617) ;
#96525=AXIS2_PLACEMENT_3D('',#149065,#116619,#116620) ;
#96526=AXIS2_PLACEMENT_3D('',#149066,#116621,#116622) ;
#96527=AXIS2_PLACEMENT_3D('',#149067,#116623,#116624) ;
#96528=AXIS2_PLACEMENT_3D('',#149068,#116625,#116626) ;
#96529=AXIS2_PLACEMENT_3D('',#149069,#116627,#116628) ;
#96530=AXIS2_PLACEMENT_3D('',#149070,#116629,#116630) ;
#96531=AXIS2_PLACEMENT_3D('',#149071,#116631,#116632) ;
#96532=AXIS2_PLACEMENT_3D('',#149072,#116633,#116634) ;
#96533=AXIS2_PLACEMENT_3D('',#149073,#116635,#116636) ;
#96534=AXIS2_PLACEMENT_3D('',#149074,#116637,#116638) ;
#96535=AXIS2_PLACEMENT_3D('',#149075,#116639,#116640) ;
#96536=AXIS2_PLACEMENT_3D('',#149076,#116641,#116642) ;
#96537=AXIS2_PLACEMENT_3D('',#149077,#116643,#116644) ;
#96538=AXIS2_PLACEMENT_3D('',#149078,#116645,#116646) ;
#96539=AXIS2_PLACEMENT_3D('',#149079,#116647,#116648) ;
#96540=AXIS2_PLACEMENT_3D('',#149080,#116649,#116650) ;
#96541=AXIS2_PLACEMENT_3D('',#149081,#116651,#116652) ;
#96542=AXIS2_PLACEMENT_3D('',#149082,#116653,#116654) ;
#96543=AXIS2_PLACEMENT_3D('',#149083,#116655,#116656) ;
#96544=AXIS2_PLACEMENT_3D('',#149084,#116657,#116658) ;
#96545=AXIS2_PLACEMENT_3D('',#149085,#116659,#116660) ;
#96546=AXIS2_PLACEMENT_3D('',#149086,#116661,#116662) ;
#96547=AXIS2_PLACEMENT_3D('',#149087,#116663,#116664) ;
#96548=AXIS2_PLACEMENT_3D('',#149088,#116665,#116666) ;
#96549=AXIS2_PLACEMENT_3D('',#149089,#116667,#116668) ;
#96550=AXIS2_PLACEMENT_3D('',#149090,#116669,#116670) ;
#96551=AXIS2_PLACEMENT_3D('',#149091,#116671,#116672) ;
#96552=AXIS2_PLACEMENT_3D('',#149092,#116673,#116674) ;
#96553=AXIS2_PLACEMENT_3D('',#149093,#116675,#116676) ;
#96554=AXIS2_PLACEMENT_3D('',#149094,#116677,#116678) ;
#96555=AXIS2_PLACEMENT_3D('',#149095,#116679,#116680) ;
#96556=AXIS2_PLACEMENT_3D('',#149096,#116681,#116682) ;
#96557=AXIS2_PLACEMENT_3D('',#149097,#116683,#116684) ;
#96558=AXIS2_PLACEMENT_3D('',#149098,#116685,#116686) ;
#96559=AXIS2_PLACEMENT_3D('',#149099,#116687,#116688) ;
#96560=AXIS2_PLACEMENT_3D('',#149100,#116689,#116690) ;
#96561=AXIS2_PLACEMENT_3D('',#149101,#116691,#116692) ;
#96562=AXIS2_PLACEMENT_3D('',#149102,#116693,#116694) ;
#96563=AXIS2_PLACEMENT_3D('',#149103,#116695,#116696) ;
#96564=AXIS2_PLACEMENT_3D('',#149104,#116697,#116698) ;
#96565=AXIS2_PLACEMENT_3D('',#149105,#116699,#116700) ;
#96566=AXIS2_PLACEMENT_3D('',#149106,#116701,#116702) ;
#96567=AXIS2_PLACEMENT_3D('',#149107,#116703,#116704) ;
#96568=AXIS2_PLACEMENT_3D('',#149108,#116705,#116706) ;
#96569=AXIS2_PLACEMENT_3D('',#149109,#116707,#116708) ;
#96570=AXIS2_PLACEMENT_3D('',#149110,#116709,#116710) ;
#96571=AXIS2_PLACEMENT_3D('',#149111,#116711,#116712) ;
#96572=AXIS2_PLACEMENT_3D('',#149112,#116713,#116714) ;
#96573=AXIS2_PLACEMENT_3D('',#149113,#116715,#116716) ;
#96574=AXIS2_PLACEMENT_3D('',#149114,#116717,#116718) ;
#96575=AXIS2_PLACEMENT_3D('',#149115,#116719,#116720) ;
#96576=AXIS2_PLACEMENT_3D('',#149116,#116721,#116722) ;
#96577=AXIS2_PLACEMENT_3D('',#149117,#116723,#116724) ;
#96578=AXIS2_PLACEMENT_3D('',#149118,#116725,#116726) ;
#96579=AXIS2_PLACEMENT_3D('',#149119,#116727,#116728) ;
#96580=AXIS2_PLACEMENT_3D('',#149120,#116729,#116730) ;
#96581=AXIS2_PLACEMENT_3D('',#149121,#116731,#116732) ;
#96582=AXIS2_PLACEMENT_3D('',#149122,#116733,#116734) ;
#96583=AXIS2_PLACEMENT_3D('',#149123,#116735,#116736) ;
#96584=AXIS2_PLACEMENT_3D('',#149124,#116737,#116738) ;
#96585=AXIS2_PLACEMENT_3D('',#149125,#116739,#116740) ;
#96586=AXIS2_PLACEMENT_3D('',#149126,#116741,#116742) ;
#96587=AXIS2_PLACEMENT_3D('',#149127,#116743,#116744) ;
#96588=AXIS2_PLACEMENT_3D('',#149128,#116745,#116746) ;
#96589=AXIS2_PLACEMENT_3D('',#149129,#116747,#116748) ;
#96590=AXIS2_PLACEMENT_3D('',#149130,#116749,#116750) ;
#96591=AXIS2_PLACEMENT_3D('',#149131,#116751,#116752) ;
#96592=AXIS2_PLACEMENT_3D('',#149133,#116753,#116754) ;
#96593=AXIS2_PLACEMENT_3D('',#149134,#116755,#116756) ;
#96594=AXIS2_PLACEMENT_3D('',#149135,#116757,#116758) ;
#96595=AXIS2_PLACEMENT_3D('',#149136,#116759,#116760) ;
#96596=AXIS2_PLACEMENT_3D('',#149137,#116761,#116762) ;
#96597=AXIS2_PLACEMENT_3D('',#149138,#116763,#116764) ;
#96598=AXIS2_PLACEMENT_3D('',#149139,#116765,#116766) ;
#96599=AXIS2_PLACEMENT_3D('',#149140,#116767,#116768) ;
#96600=AXIS2_PLACEMENT_3D('',#149141,#116769,#116770) ;
#96601=AXIS2_PLACEMENT_3D('',#149152,#116772,#116773) ;
#96602=AXIS2_PLACEMENT_3D('',#149209,#116775,#116776) ;
#96603=AXIS2_PLACEMENT_3D('',#149210,#116777,#116778) ;
#96604=AXIS2_PLACEMENT_3D('',#149211,#116779,#116780) ;
#96605=AXIS2_PLACEMENT_3D('',#149212,#116781,#116782) ;
#96606=AXIS2_PLACEMENT_3D('',#149213,#116783,#116784) ;
#96607=AXIS2_PLACEMENT_3D('',#149214,#116785,#116786) ;
#96608=AXIS2_PLACEMENT_3D('',#149215,#116787,#116788) ;
#96609=AXIS2_PLACEMENT_3D('',#149216,#116789,#116790) ;
#96610=AXIS2_PLACEMENT_3D('',#149217,#116791,#116792) ;
#96611=AXIS2_PLACEMENT_3D('',#149218,#116793,#116794) ;
#96612=AXIS2_PLACEMENT_3D('',#149219,#116795,#116796) ;
#96613=AXIS2_PLACEMENT_3D('',#149220,#116797,#116798) ;
#96614=AXIS2_PLACEMENT_3D('',#149221,#116799,#116800) ;
#96615=AXIS2_PLACEMENT_3D('',#149222,#116801,#116802) ;
#96616=AXIS2_PLACEMENT_3D('',#149223,#116803,#116804) ;
#96617=AXIS2_PLACEMENT_3D('',#149224,#116805,#116806) ;
#96618=AXIS2_PLACEMENT_3D('',#149225,#116807,#116808) ;
#96619=AXIS2_PLACEMENT_3D('',#149226,#116809,#116810) ;
#96620=AXIS2_PLACEMENT_3D('',#149227,#116811,#116812) ;
#96621=AXIS2_PLACEMENT_3D('',#149228,#116813,#116814) ;
#96622=AXIS2_PLACEMENT_3D('',#149229,#116815,#116816) ;
#96623=AXIS2_PLACEMENT_3D('',#149230,#116817,#116818) ;
#96624=AXIS2_PLACEMENT_3D('',#149231,#116819,#116820) ;
#96625=AXIS2_PLACEMENT_3D('',#149234,#116822,#116823) ;
#96626=AXIS2_PLACEMENT_3D('',#149235,#116824,#116825) ;
#96627=AXIS2_PLACEMENT_3D('',#149236,#116826,#116827) ;
#96628=AXIS2_PLACEMENT_3D('',#149237,#116828,#116829) ;
#96629=AXIS2_PLACEMENT_3D('',#149238,#116830,#116831) ;
#96630=AXIS2_PLACEMENT_3D('',#149239,#116832,#116833) ;
#96631=AXIS2_PLACEMENT_3D('',#149240,#116834,#116835) ;
#96632=AXIS2_PLACEMENT_3D('',#149241,#116836,#116837) ;
#96633=AXIS2_PLACEMENT_3D('',#149242,#116838,#116839) ;
#96634=AXIS2_PLACEMENT_3D('',#149243,#116840,#116841) ;
#96635=AXIS2_PLACEMENT_3D('',#149244,#116842,#116843) ;
#96636=AXIS2_PLACEMENT_3D('',#149245,#116844,#116845) ;
#96637=AXIS2_PLACEMENT_3D('',#149246,#116846,#116847) ;
#96638=AXIS2_PLACEMENT_3D('',#149247,#116848,#116849) ;
#96639=AXIS2_PLACEMENT_3D('',#149248,#116850,#116851) ;
#96640=AXIS2_PLACEMENT_3D('',#149249,#116852,#116853) ;
#96641=AXIS2_PLACEMENT_3D('',#149251,#116854,#116855) ;
#96642=AXIS2_PLACEMENT_3D('',#149252,#116856,#116857) ;
#96643=AXIS2_PLACEMENT_3D('',#149253,#116858,#116859) ;
#96644=AXIS2_PLACEMENT_3D('',#149254,#116860,#116861) ;
#96645=AXIS2_PLACEMENT_3D('',#149255,#116862,#116863) ;
#96646=AXIS2_PLACEMENT_3D('',#149256,#116864,#116865) ;
#96647=AXIS2_PLACEMENT_3D('',#149257,#116866,#116867) ;
#96648=AXIS2_PLACEMENT_3D('',#149258,#116868,#116869) ;
#96649=AXIS2_PLACEMENT_3D('',#149259,#116870,#116871) ;
#96650=AXIS2_PLACEMENT_3D('',#149260,#116872,#116873) ;
#96651=AXIS2_PLACEMENT_3D('',#149261,#116874,#116875) ;
#96652=AXIS2_PLACEMENT_3D('',#149262,#116876,#116877) ;
#96653=AXIS2_PLACEMENT_3D('',#149263,#116878,#116879) ;
#96654=AXIS2_PLACEMENT_3D('',#149266,#116881,#116882) ;
#96655=AXIS2_PLACEMENT_3D('',#149267,#116883,#116884) ;
#96656=AXIS2_PLACEMENT_3D('',#149268,#116885,#116886) ;
#96657=AXIS2_PLACEMENT_3D('',#149269,#116887,#116888) ;
#96658=AXIS2_PLACEMENT_3D('',#149270,#116889,#116890) ;
#96659=AXIS2_PLACEMENT_3D('',#149271,#116891,#116892) ;
#96660=AXIS2_PLACEMENT_3D('',#149272,#116893,#116894) ;
#96661=AXIS2_PLACEMENT_3D('',#149273,#116895,#116896) ;
#96662=AXIS2_PLACEMENT_3D('',#149274,#116897,#116898) ;
#96663=AXIS2_PLACEMENT_3D('',#149275,#116899,#116900) ;
#96664=AXIS2_PLACEMENT_3D('',#149276,#116901,#116902) ;
#96665=AXIS2_PLACEMENT_3D('',#149277,#116903,#116904) ;
#96666=AXIS2_PLACEMENT_3D('',#149278,#116905,#116906) ;
#96667=AXIS2_PLACEMENT_3D('',#149280,#116907,#116908) ;
#96668=AXIS2_PLACEMENT_3D('',#149281,#116909,#116910) ;
#96669=AXIS2_PLACEMENT_3D('',#149282,#116911,#116912) ;
#96670=AXIS2_PLACEMENT_3D('',#149283,#116913,#116914) ;
#96671=AXIS2_PLACEMENT_3D('',#149284,#116915,#116916) ;
#96672=AXIS2_PLACEMENT_3D('',#149285,#116917,#116918) ;
#96673=AXIS2_PLACEMENT_3D('',#149286,#116919,#116920) ;
#96674=AXIS2_PLACEMENT_3D('',#149287,#116921,#116922) ;
#96675=AXIS2_PLACEMENT_3D('',#149288,#116923,#116924) ;
#96676=AXIS2_PLACEMENT_3D('',#149289,#116925,#116926) ;
#96677=AXIS2_PLACEMENT_3D('',#149290,#116927,#116928) ;
#96678=AXIS2_PLACEMENT_3D('',#149292,#116930,#116931) ;
#96679=AXIS2_PLACEMENT_3D('',#149293,#116932,#116933) ;
#96680=AXIS2_PLACEMENT_3D('',#149294,#116934,#116935) ;
#96681=AXIS2_PLACEMENT_3D('',#149295,#116936,#116937) ;
#96682=AXIS2_PLACEMENT_3D('',#149296,#116938,#116939) ;
#96683=AXIS2_PLACEMENT_3D('',#149297,#116940,#116941) ;
#96684=AXIS2_PLACEMENT_3D('',#149298,#116942,#116943) ;
#96685=AXIS2_PLACEMENT_3D('',#149299,#116944,#116945) ;
#96686=AXIS2_PLACEMENT_3D('',#149300,#116946,#116947) ;
#96687=AXIS2_PLACEMENT_3D('',#149301,#116948,#116949) ;
#96688=AXIS2_PLACEMENT_3D('',#149302,#116950,#116951) ;
#96689=AXIS2_PLACEMENT_3D('',#149303,#116952,#116953) ;
#96690=AXIS2_PLACEMENT_3D('',#149304,#116954,#116955) ;
#96691=AXIS2_PLACEMENT_3D('',#149305,#116956,#116957) ;
#96692=AXIS2_PLACEMENT_3D('',#149306,#116958,#116959) ;
#96693=AXIS2_PLACEMENT_3D('',#149307,#116960,#116961) ;
#96694=AXIS2_PLACEMENT_3D('',#149308,#116962,#116963) ;
#96695=AXIS2_PLACEMENT_3D('',#149309,#116964,#116965) ;
#96696=AXIS2_PLACEMENT_3D('',#149310,#116966,#116967) ;
#96697=AXIS2_PLACEMENT_3D('',#149311,#116968,#116969) ;
#96698=AXIS2_PLACEMENT_3D('',#149312,#116970,#116971) ;
#96699=AXIS2_PLACEMENT_3D('',#149313,#116972,#116973) ;
#96700=AXIS2_PLACEMENT_3D('',#149314,#116974,#116975) ;
#96701=AXIS2_PLACEMENT_3D('',#149315,#116976,#116977) ;
#96702=AXIS2_PLACEMENT_3D('',#149316,#116978,#116979) ;
#96703=AXIS2_PLACEMENT_3D('',#149317,#116980,#116981) ;
#96704=AXIS2_PLACEMENT_3D('',#149318,#116982,#116983) ;
#96705=AXIS2_PLACEMENT_3D('',#149319,#116984,#116985) ;
#96706=AXIS2_PLACEMENT_3D('',#149320,#116986,#116987) ;
#96707=AXIS2_PLACEMENT_3D('',#149321,#116988,#116989) ;
#96708=AXIS2_PLACEMENT_3D('',#149322,#116990,#116991) ;
#96709=AXIS2_PLACEMENT_3D('',#149323,#116992,#116993) ;
#96710=AXIS2_PLACEMENT_3D('',#149324,#116994,#116995) ;
#96711=AXIS2_PLACEMENT_3D('',#149325,#116996,#116997) ;
#96712=AXIS2_PLACEMENT_3D('',#149326,#116998,#116999) ;
#96713=AXIS2_PLACEMENT_3D('',#149327,#117000,#117001) ;
#96714=AXIS2_PLACEMENT_3D('',#149328,#117002,#117003) ;
#96715=AXIS2_PLACEMENT_3D('',#149329,#117004,#117005) ;
#96716=AXIS2_PLACEMENT_3D('',#149330,#117006,#117007) ;
#96717=AXIS2_PLACEMENT_3D('',#149331,#117008,#117009) ;
#96718=AXIS2_PLACEMENT_3D('',#149332,#117010,#117011) ;
#96719=AXIS2_PLACEMENT_3D('',#149333,#117012,#117013) ;
#96720=AXIS2_PLACEMENT_3D('',#149334,#117014,#117015) ;
#96721=AXIS2_PLACEMENT_3D('',#149335,#117016,#117017) ;
#96722=AXIS2_PLACEMENT_3D('',#149336,#117018,#117019) ;
#96723=AXIS2_PLACEMENT_3D('',#149337,#117020,#117021) ;
#96724=AXIS2_PLACEMENT_3D('',#149338,#117022,#117023) ;
#96725=AXIS2_PLACEMENT_3D('',#149339,#117024,#117025) ;
#96726=AXIS2_PLACEMENT_3D('',#149340,#117026,#117027) ;
#96727=AXIS2_PLACEMENT_3D('',#149341,#117028,#117029) ;
#96728=AXIS2_PLACEMENT_3D('',#149342,#117030,#117031) ;
#96729=AXIS2_PLACEMENT_3D('',#149343,#117032,#117033) ;
#96730=AXIS2_PLACEMENT_3D('',#149344,#117034,#117035) ;
#96731=AXIS2_PLACEMENT_3D('',#149345,#117036,#117037) ;
#96732=AXIS2_PLACEMENT_3D('',#149346,#117038,#117039) ;
#96733=AXIS2_PLACEMENT_3D('',#149347,#117040,#117041) ;
#96734=AXIS2_PLACEMENT_3D('',#149348,#117042,#117043) ;
#96735=AXIS2_PLACEMENT_3D('',#149349,#117044,#117045) ;
#96736=AXIS2_PLACEMENT_3D('',#149350,#117046,#117047) ;
#96737=AXIS2_PLACEMENT_3D('',#149351,#117048,#117049) ;
#96738=AXIS2_PLACEMENT_3D('',#149352,#117050,#117051) ;
#96739=AXIS2_PLACEMENT_3D('',#149353,#117052,#117053) ;
#96740=AXIS2_PLACEMENT_3D('',#149354,#117054,#117055) ;
#96741=AXIS2_PLACEMENT_3D('',#149355,#117056,#117057) ;
#96742=AXIS2_PLACEMENT_3D('',#149356,#117058,#117059) ;
#96743=AXIS2_PLACEMENT_3D('',#149357,#117060,#117061) ;
#96744=AXIS2_PLACEMENT_3D('',#149358,#117062,#117063) ;
#96745=AXIS2_PLACEMENT_3D('',#149360,#117064,#117065) ;
#96746=AXIS2_PLACEMENT_3D('',#149361,#117066,#117067) ;
#96747=AXIS2_PLACEMENT_3D('',#149362,#117068,#117069) ;
#96748=AXIS2_PLACEMENT_3D('',#149363,#117070,#117071) ;
#96749=AXIS2_PLACEMENT_3D('',#149364,#117072,#117073) ;
#96750=AXIS2_PLACEMENT_3D('',#149365,#117074,#117075) ;
#96751=AXIS2_PLACEMENT_3D('',#149366,#117076,#117077) ;
#96752=AXIS2_PLACEMENT_3D('',#149367,#117078,#117079) ;
#96753=AXIS2_PLACEMENT_3D('',#149368,#117080,#117081) ;
#96754=AXIS2_PLACEMENT_3D('',#149379,#117083,#117084) ;
#96755=AXIS2_PLACEMENT_3D('',#149436,#117086,#117087) ;
#96756=AXIS2_PLACEMENT_3D('',#149437,#117088,#117089) ;
#96757=AXIS2_PLACEMENT_3D('',#149438,#117090,#117091) ;
#96758=AXIS2_PLACEMENT_3D('',#149439,#117092,#117093) ;
#96759=AXIS2_PLACEMENT_3D('',#149440,#117094,#117095) ;
#96760=AXIS2_PLACEMENT_3D('',#149441,#117096,#117097) ;
#96761=AXIS2_PLACEMENT_3D('',#149442,#117098,#117099) ;
#96762=AXIS2_PLACEMENT_3D('',#149443,#117100,#117101) ;
#96763=AXIS2_PLACEMENT_3D('',#149444,#117102,#117103) ;
#96764=AXIS2_PLACEMENT_3D('',#149445,#117104,#117105) ;
#96765=AXIS2_PLACEMENT_3D('',#149446,#117106,#117107) ;
#96766=AXIS2_PLACEMENT_3D('',#149447,#117108,#117109) ;
#96767=AXIS2_PLACEMENT_3D('',#149448,#117110,#117111) ;
#96768=AXIS2_PLACEMENT_3D('',#149449,#117112,#117113) ;
#96769=AXIS2_PLACEMENT_3D('',#149450,#117114,#117115) ;
#96770=AXIS2_PLACEMENT_3D('',#149451,#117116,#117117) ;
#96771=AXIS2_PLACEMENT_3D('',#149452,#117118,#117119) ;
#96772=AXIS2_PLACEMENT_3D('',#149453,#117120,#117121) ;
#96773=AXIS2_PLACEMENT_3D('',#149454,#117122,#117123) ;
#96774=AXIS2_PLACEMENT_3D('',#149455,#117124,#117125) ;
#96775=AXIS2_PLACEMENT_3D('',#149456,#117126,#117127) ;
#96776=AXIS2_PLACEMENT_3D('',#149457,#117128,#117129) ;
#96777=AXIS2_PLACEMENT_3D('',#149458,#117130,#117131) ;
#96778=AXIS2_PLACEMENT_3D('',#149461,#117133,#117134) ;
#96779=AXIS2_PLACEMENT_3D('',#149462,#117135,#117136) ;
#96780=AXIS2_PLACEMENT_3D('',#149463,#117137,#117138) ;
#96781=AXIS2_PLACEMENT_3D('',#149464,#117139,#117140) ;
#96782=AXIS2_PLACEMENT_3D('',#149465,#117141,#117142) ;
#96783=AXIS2_PLACEMENT_3D('',#149466,#117143,#117144) ;
#96784=AXIS2_PLACEMENT_3D('',#149467,#117145,#117146) ;
#96785=AXIS2_PLACEMENT_3D('',#149468,#117147,#117148) ;
#96786=AXIS2_PLACEMENT_3D('',#149469,#117149,#117150) ;
#96787=AXIS2_PLACEMENT_3D('',#149470,#117151,#117152) ;
#96788=AXIS2_PLACEMENT_3D('',#149471,#117153,#117154) ;
#96789=AXIS2_PLACEMENT_3D('',#149472,#117155,#117156) ;
#96790=AXIS2_PLACEMENT_3D('',#149473,#117157,#117158) ;
#96791=AXIS2_PLACEMENT_3D('',#149474,#117159,#117160) ;
#96792=AXIS2_PLACEMENT_3D('',#149475,#117161,#117162) ;
#96793=AXIS2_PLACEMENT_3D('',#149476,#117163,#117164) ;
#96794=AXIS2_PLACEMENT_3D('',#149478,#117165,#117166) ;
#96795=AXIS2_PLACEMENT_3D('',#149479,#117167,#117168) ;
#96796=AXIS2_PLACEMENT_3D('',#149480,#117169,#117170) ;
#96797=AXIS2_PLACEMENT_3D('',#149481,#117171,#117172) ;
#96798=AXIS2_PLACEMENT_3D('',#149482,#117173,#117174) ;
#96799=AXIS2_PLACEMENT_3D('',#149483,#117175,#117176) ;
#96800=AXIS2_PLACEMENT_3D('',#149484,#117177,#117178) ;
#96801=AXIS2_PLACEMENT_3D('',#149485,#117179,#117180) ;
#96802=AXIS2_PLACEMENT_3D('',#149486,#117181,#117182) ;
#96803=AXIS2_PLACEMENT_3D('',#149487,#117183,#117184) ;
#96804=AXIS2_PLACEMENT_3D('',#149488,#117185,#117186) ;
#96805=AXIS2_PLACEMENT_3D('',#149489,#117187,#117188) ;
#96806=AXIS2_PLACEMENT_3D('',#149490,#117189,#117190) ;
#96807=AXIS2_PLACEMENT_3D('',#149493,#117192,#117193) ;
#96808=AXIS2_PLACEMENT_3D('',#149494,#117194,#117195) ;
#96809=AXIS2_PLACEMENT_3D('',#149495,#117196,#117197) ;
#96810=AXIS2_PLACEMENT_3D('',#149496,#117198,#117199) ;
#96811=AXIS2_PLACEMENT_3D('',#149497,#117200,#117201) ;
#96812=AXIS2_PLACEMENT_3D('',#149498,#117202,#117203) ;
#96813=AXIS2_PLACEMENT_3D('',#149499,#117204,#117205) ;
#96814=AXIS2_PLACEMENT_3D('',#149500,#117206,#117207) ;
#96815=AXIS2_PLACEMENT_3D('',#149501,#117208,#117209) ;
#96816=AXIS2_PLACEMENT_3D('',#149502,#117210,#117211) ;
#96817=AXIS2_PLACEMENT_3D('',#149503,#117212,#117213) ;
#96818=AXIS2_PLACEMENT_3D('',#149504,#117214,#117215) ;
#96819=AXIS2_PLACEMENT_3D('',#149505,#117216,#117217) ;
#96820=AXIS2_PLACEMENT_3D('',#149507,#117218,#117219) ;
#96821=AXIS2_PLACEMENT_3D('',#149508,#117220,#117221) ;
#96822=AXIS2_PLACEMENT_3D('',#149509,#117222,#117223) ;
#96823=AXIS2_PLACEMENT_3D('',#149510,#117224,#117225) ;
#96824=AXIS2_PLACEMENT_3D('',#149511,#117226,#117227) ;
#96825=AXIS2_PLACEMENT_3D('',#149512,#117228,#117229) ;
#96826=AXIS2_PLACEMENT_3D('',#149513,#117230,#117231) ;
#96827=AXIS2_PLACEMENT_3D('',#149514,#117232,#117233) ;
#96828=AXIS2_PLACEMENT_3D('',#149515,#117234,#117235) ;
#96829=AXIS2_PLACEMENT_3D('',#149516,#117236,#117237) ;
#96830=AXIS2_PLACEMENT_3D('',#149517,#117238,#117239) ;
#96831=AXIS2_PLACEMENT_3D('',#149519,#117241,#117242) ;
#96832=AXIS2_PLACEMENT_3D('',#149520,#117243,#117244) ;
#96833=AXIS2_PLACEMENT_3D('',#149521,#117245,#117246) ;
#96834=AXIS2_PLACEMENT_3D('',#149522,#117247,#117248) ;
#96835=AXIS2_PLACEMENT_3D('',#149523,#117249,#117250) ;
#96836=AXIS2_PLACEMENT_3D('',#149524,#117251,#117252) ;
#96837=AXIS2_PLACEMENT_3D('',#149525,#117253,#117254) ;
#96838=AXIS2_PLACEMENT_3D('',#149526,#117255,#117256) ;
#96839=AXIS2_PLACEMENT_3D('',#149527,#117257,#117258) ;
#96840=AXIS2_PLACEMENT_3D('',#149528,#117259,#117260) ;
#96841=AXIS2_PLACEMENT_3D('',#149529,#117261,#117262) ;
#96842=AXIS2_PLACEMENT_3D('',#149530,#117263,#117264) ;
#96843=AXIS2_PLACEMENT_3D('',#149531,#117265,#117266) ;
#96844=AXIS2_PLACEMENT_3D('',#149532,#117267,#117268) ;
#96845=AXIS2_PLACEMENT_3D('',#149533,#117269,#117270) ;
#96846=AXIS2_PLACEMENT_3D('',#149534,#117271,#117272) ;
#96847=AXIS2_PLACEMENT_3D('',#149535,#117273,#117274) ;
#96848=AXIS2_PLACEMENT_3D('',#149536,#117275,#117276) ;
#96849=AXIS2_PLACEMENT_3D('',#149537,#117277,#117278) ;
#96850=AXIS2_PLACEMENT_3D('',#149538,#117279,#117280) ;
#96851=AXIS2_PLACEMENT_3D('',#149539,#117281,#117282) ;
#96852=AXIS2_PLACEMENT_3D('',#149540,#117283,#117284) ;
#96853=AXIS2_PLACEMENT_3D('',#149541,#117285,#117286) ;
#96854=AXIS2_PLACEMENT_3D('',#149542,#117287,#117288) ;
#96855=AXIS2_PLACEMENT_3D('',#149543,#117289,#117290) ;
#96856=AXIS2_PLACEMENT_3D('',#149544,#117291,#117292) ;
#96857=AXIS2_PLACEMENT_3D('',#149545,#117293,#117294) ;
#96858=AXIS2_PLACEMENT_3D('',#149546,#117295,#117296) ;
#96859=AXIS2_PLACEMENT_3D('',#149547,#117297,#117298) ;
#96860=AXIS2_PLACEMENT_3D('',#149548,#117299,#117300) ;
#96861=AXIS2_PLACEMENT_3D('',#149549,#117301,#117302) ;
#96862=AXIS2_PLACEMENT_3D('',#149550,#117303,#117304) ;
#96863=AXIS2_PLACEMENT_3D('',#149551,#117305,#117306) ;
#96864=AXIS2_PLACEMENT_3D('',#149552,#117307,#117308) ;
#96865=AXIS2_PLACEMENT_3D('',#149553,#117309,#117310) ;
#96866=AXIS2_PLACEMENT_3D('',#149554,#117311,#117312) ;
#96867=AXIS2_PLACEMENT_3D('',#149555,#117313,#117314) ;
#96868=AXIS2_PLACEMENT_3D('',#149556,#117315,#117316) ;
#96869=AXIS2_PLACEMENT_3D('',#149557,#117317,#117318) ;
#96870=AXIS2_PLACEMENT_3D('',#149558,#117319,#117320) ;
#96871=AXIS2_PLACEMENT_3D('',#149559,#117321,#117322) ;
#96872=AXIS2_PLACEMENT_3D('',#149560,#117323,#117324) ;
#96873=AXIS2_PLACEMENT_3D('',#149561,#117325,#117326) ;
#96874=AXIS2_PLACEMENT_3D('',#149562,#117327,#117328) ;
#96875=AXIS2_PLACEMENT_3D('',#149563,#117329,#117330) ;
#96876=AXIS2_PLACEMENT_3D('',#149564,#117331,#117332) ;
#96877=AXIS2_PLACEMENT_3D('',#149565,#117333,#117334) ;
#96878=AXIS2_PLACEMENT_3D('',#149566,#117335,#117336) ;
#96879=AXIS2_PLACEMENT_3D('',#149567,#117337,#117338) ;
#96880=AXIS2_PLACEMENT_3D('',#149568,#117339,#117340) ;
#96881=AXIS2_PLACEMENT_3D('',#149569,#117341,#117342) ;
#96882=AXIS2_PLACEMENT_3D('',#149570,#117343,#117344) ;
#96883=AXIS2_PLACEMENT_3D('',#149571,#117345,#117346) ;
#96884=AXIS2_PLACEMENT_3D('',#149572,#117347,#117348) ;
#96885=AXIS2_PLACEMENT_3D('',#149573,#117349,#117350) ;
#96886=AXIS2_PLACEMENT_3D('',#149574,#117351,#117352) ;
#96887=AXIS2_PLACEMENT_3D('',#149575,#117353,#117354) ;
#96888=AXIS2_PLACEMENT_3D('',#149576,#117355,#117356) ;
#96889=AXIS2_PLACEMENT_3D('',#149577,#117357,#117358) ;
#96890=AXIS2_PLACEMENT_3D('',#149578,#117359,#117360) ;
#96891=AXIS2_PLACEMENT_3D('',#149579,#117361,#117362) ;
#96892=AXIS2_PLACEMENT_3D('',#149588,#117367,#117368) ;
#96893=AXIS2_PLACEMENT_3D('',#149597,#117373,#117374) ;
#96894=AXIS2_PLACEMENT_3D('',#149606,#117379,#117380) ;
#96895=AXIS2_PLACEMENT_3D('',#149615,#117385,#117386) ;
#96896=AXIS2_PLACEMENT_3D('',#149624,#117391,#117392) ;
#96897=AXIS2_PLACEMENT_3D('',#149628,#117394,#117395) ;
#96898=AXIS2_PLACEMENT_3D('',#149630,#117396,#117397) ;
#96899=AXIS2_PLACEMENT_3D('',#149634,#117400,#117401) ;
#96900=AXIS2_PLACEMENT_3D('',#149638,#117403,#117404) ;
#96901=AXIS2_PLACEMENT_3D('',#149640,#117405,#117406) ;
#96902=AXIS2_PLACEMENT_3D('',#149644,#117409,#117410) ;
#96903=AXIS2_PLACEMENT_3D('',#149645,#117411,#117412) ;
#96904=AXIS2_PLACEMENT_3D('',#149646,#117413,#117414) ;
#96905=AXIS2_PLACEMENT_3D('',#149647,#117415,#117416) ;
#96906=AXIS2_PLACEMENT_3D('',#149648,#117417,#117418) ;
#96907=AXIS2_PLACEMENT_3D('',#149649,#117419,#117420) ;
#96908=AXIS2_PLACEMENT_3D('',#149650,#117421,#117422) ;
#96909=AXIS2_PLACEMENT_3D('',#149659,#117427,#117428) ;
#96910=AXIS2_PLACEMENT_3D('',#149665,#117432,#117433) ;
#96911=AXIS2_PLACEMENT_3D('',#149671,#117437,#117438) ;
#96912=AXIS2_PLACEMENT_3D('',#149680,#117443,#117444) ;
#96913=AXIS2_PLACEMENT_3D('',#149689,#117449,#117450) ;
#96914=AXIS2_PLACEMENT_3D('',#149695,#117454,#117455) ;
#96915=AXIS2_PLACEMENT_3D('',#149701,#117459,#117460) ;
#96916=AXIS2_PLACEMENT_3D('',#149710,#117465,#117466) ;
#96917=AXIS2_PLACEMENT_3D('',#149719,#117471,#117472) ;
#96918=AXIS2_PLACEMENT_3D('',#149728,#117477,#117478) ;
#96919=AXIS2_PLACEMENT_3D('',#149737,#117483,#117484) ;
#96920=AXIS2_PLACEMENT_3D('',#149746,#117489,#117490) ;
#96921=AXIS2_PLACEMENT_3D('',#149750,#117492,#117493) ;
#96922=AXIS2_PLACEMENT_3D('',#149752,#117494,#117495) ;
#96923=AXIS2_PLACEMENT_3D('',#149756,#117498,#117499) ;
#96924=AXIS2_PLACEMENT_3D('',#149760,#117501,#117502) ;
#96925=AXIS2_PLACEMENT_3D('',#149762,#117503,#117504) ;
#96926=AXIS2_PLACEMENT_3D('',#149766,#117507,#117508) ;
#96927=AXIS2_PLACEMENT_3D('',#149767,#117509,#117510) ;
#96928=AXIS2_PLACEMENT_3D('',#149768,#117511,#117512) ;
#96929=AXIS2_PLACEMENT_3D('',#149769,#117513,#117514) ;
#96930=AXIS2_PLACEMENT_3D('',#149770,#117515,#117516) ;
#96931=AXIS2_PLACEMENT_3D('',#149771,#117517,#117518) ;
#96932=AXIS2_PLACEMENT_3D('',#149772,#117519,#117520) ;
#96933=AXIS2_PLACEMENT_3D('',#149781,#117525,#117526) ;
#96934=AXIS2_PLACEMENT_3D('',#149787,#117530,#117531) ;
#96935=AXIS2_PLACEMENT_3D('',#149793,#117535,#117536) ;
#96936=AXIS2_PLACEMENT_3D('',#149802,#117541,#117542) ;
#96937=AXIS2_PLACEMENT_3D('',#149811,#117547,#117548) ;
#96938=AXIS2_PLACEMENT_3D('',#149817,#117552,#117553) ;
#96939=AXIS2_PLACEMENT_3D('',#149823,#117557,#117558) ;
#96940=AXIS2_PLACEMENT_3D('',#149832,#117563,#117564) ;
#96941=AXIS2_PLACEMENT_3D('',#149841,#117569,#117570) ;
#96942=AXIS2_PLACEMENT_3D('',#149850,#117575,#117576) ;
#96943=AXIS2_PLACEMENT_3D('',#149859,#117581,#117582) ;
#96944=AXIS2_PLACEMENT_3D('',#149868,#117587,#117588) ;
#96945=AXIS2_PLACEMENT_3D('',#149872,#117590,#117591) ;
#96946=AXIS2_PLACEMENT_3D('',#149874,#117592,#117593) ;
#96947=AXIS2_PLACEMENT_3D('',#149878,#117596,#117597) ;
#96948=AXIS2_PLACEMENT_3D('',#149882,#117599,#117600) ;
#96949=AXIS2_PLACEMENT_3D('',#149884,#117601,#117602) ;
#96950=AXIS2_PLACEMENT_3D('',#149888,#117605,#117606) ;
#96951=AXIS2_PLACEMENT_3D('',#149889,#117607,#117608) ;
#96952=AXIS2_PLACEMENT_3D('',#149890,#117609,#117610) ;
#96953=AXIS2_PLACEMENT_3D('',#149891,#117611,#117612) ;
#96954=AXIS2_PLACEMENT_3D('',#149892,#117613,#117614) ;
#96955=AXIS2_PLACEMENT_3D('',#149893,#117615,#117616) ;
#96956=AXIS2_PLACEMENT_3D('',#149894,#117617,#117618) ;
#96957=AXIS2_PLACEMENT_3D('',#149903,#117623,#117624) ;
#96958=AXIS2_PLACEMENT_3D('',#149909,#117628,#117629) ;
#96959=AXIS2_PLACEMENT_3D('',#149915,#117633,#117634) ;
#96960=AXIS2_PLACEMENT_3D('',#149924,#117639,#117640) ;
#96961=AXIS2_PLACEMENT_3D('',#149933,#117645,#117646) ;
#96962=AXIS2_PLACEMENT_3D('',#149939,#117650,#117651) ;
#96963=AXIS2_PLACEMENT_3D('',#149945,#117655,#117656) ;
#96964=AXIS2_PLACEMENT_3D('',#149954,#117661,#117662) ;
#96965=AXIS2_PLACEMENT_3D('',#149963,#117667,#117668) ;
#96966=AXIS2_PLACEMENT_3D('',#149972,#117673,#117674) ;
#96967=AXIS2_PLACEMENT_3D('',#149981,#117679,#117680) ;
#96968=AXIS2_PLACEMENT_3D('',#149990,#117685,#117686) ;
#96969=AXIS2_PLACEMENT_3D('',#149994,#117688,#117689) ;
#96970=AXIS2_PLACEMENT_3D('',#149996,#117690,#117691) ;
#96971=AXIS2_PLACEMENT_3D('',#150000,#117694,#117695) ;
#96972=AXIS2_PLACEMENT_3D('',#150004,#117697,#117698) ;
#96973=AXIS2_PLACEMENT_3D('',#150006,#117699,#117700) ;
#96974=AXIS2_PLACEMENT_3D('',#150010,#117703,#117704) ;
#96975=AXIS2_PLACEMENT_3D('',#150011,#117705,#117706) ;
#96976=AXIS2_PLACEMENT_3D('',#150012,#117707,#117708) ;
#96977=AXIS2_PLACEMENT_3D('',#150013,#117709,#117710) ;
#96978=AXIS2_PLACEMENT_3D('',#150014,#117711,#117712) ;
#96979=AXIS2_PLACEMENT_3D('',#150015,#117713,#117714) ;
#96980=AXIS2_PLACEMENT_3D('',#150016,#117715,#117716) ;
#96981=AXIS2_PLACEMENT_3D('',#150025,#117721,#117722) ;
#96982=AXIS2_PLACEMENT_3D('',#150031,#117726,#117727) ;
#96983=AXIS2_PLACEMENT_3D('',#150037,#117731,#117732) ;
#96984=AXIS2_PLACEMENT_3D('',#150046,#117737,#117738) ;
#96985=AXIS2_PLACEMENT_3D('',#150055,#117743,#117744) ;
#96986=AXIS2_PLACEMENT_3D('',#150061,#117748,#117749) ;
#96987=AXIS2_PLACEMENT_3D('',#150067,#117753,#117754) ;
#96988=AXIS2_PLACEMENT_3D('',#150076,#117759,#117760) ;
#96989=AXIS2_PLACEMENT_3D('',#150085,#117765,#117766) ;
#96990=AXIS2_PLACEMENT_3D('',#150094,#117771,#117772) ;
#96991=AXIS2_PLACEMENT_3D('',#150103,#117777,#117778) ;
#96992=AXIS2_PLACEMENT_3D('',#150112,#117783,#117784) ;
#96993=AXIS2_PLACEMENT_3D('',#150116,#117786,#117787) ;
#96994=AXIS2_PLACEMENT_3D('',#150118,#117788,#117789) ;
#96995=AXIS2_PLACEMENT_3D('',#150122,#117792,#117793) ;
#96996=AXIS2_PLACEMENT_3D('',#150126,#117795,#117796) ;
#96997=AXIS2_PLACEMENT_3D('',#150128,#117797,#117798) ;
#96998=AXIS2_PLACEMENT_3D('',#150132,#117801,#117802) ;
#96999=AXIS2_PLACEMENT_3D('',#150133,#117803,#117804) ;
#97000=AXIS2_PLACEMENT_3D('',#150134,#117805,#117806) ;
#97001=AXIS2_PLACEMENT_3D('',#150135,#117807,#117808) ;
#97002=AXIS2_PLACEMENT_3D('',#150136,#117809,#117810) ;
#97003=AXIS2_PLACEMENT_3D('',#150137,#117811,#117812) ;
#97004=AXIS2_PLACEMENT_3D('',#150138,#117813,#117814) ;
#97005=AXIS2_PLACEMENT_3D('',#150147,#117819,#117820) ;
#97006=AXIS2_PLACEMENT_3D('',#150153,#117824,#117825) ;
#97007=AXIS2_PLACEMENT_3D('',#150159,#117829,#117830) ;
#97008=AXIS2_PLACEMENT_3D('',#150168,#117835,#117836) ;
#97009=AXIS2_PLACEMENT_3D('',#150177,#117841,#117842) ;
#97010=AXIS2_PLACEMENT_3D('',#150183,#117846,#117847) ;
#97011=AXIS2_PLACEMENT_3D('',#150189,#117851,#117852) ;
#97012=AXIS2_PLACEMENT_3D('',#150198,#117857,#117858) ;
#97013=AXIS2_PLACEMENT_3D('',#150207,#117863,#117864) ;
#97014=AXIS2_PLACEMENT_3D('',#150216,#117869,#117870) ;
#97015=AXIS2_PLACEMENT_3D('',#150225,#117875,#117876) ;
#97016=AXIS2_PLACEMENT_3D('',#150234,#117881,#117882) ;
#97017=AXIS2_PLACEMENT_3D('',#150238,#117884,#117885) ;
#97018=AXIS2_PLACEMENT_3D('',#150240,#117886,#117887) ;
#97019=AXIS2_PLACEMENT_3D('',#150244,#117890,#117891) ;
#97020=AXIS2_PLACEMENT_3D('',#150248,#117893,#117894) ;
#97021=AXIS2_PLACEMENT_3D('',#150250,#117895,#117896) ;
#97022=AXIS2_PLACEMENT_3D('',#150254,#117899,#117900) ;
#97023=AXIS2_PLACEMENT_3D('',#150255,#117901,#117902) ;
#97024=AXIS2_PLACEMENT_3D('',#150256,#117903,#117904) ;
#97025=AXIS2_PLACEMENT_3D('',#150257,#117905,#117906) ;
#97026=AXIS2_PLACEMENT_3D('',#150258,#117907,#117908) ;
#97027=AXIS2_PLACEMENT_3D('',#150259,#117909,#117910) ;
#97028=AXIS2_PLACEMENT_3D('',#150260,#117911,#117912) ;
#97029=AXIS2_PLACEMENT_3D('',#150269,#117917,#117918) ;
#97030=AXIS2_PLACEMENT_3D('',#150275,#117922,#117923) ;
#97031=AXIS2_PLACEMENT_3D('',#150281,#117927,#117928) ;
#97032=AXIS2_PLACEMENT_3D('',#150290,#117933,#117934) ;
#97033=AXIS2_PLACEMENT_3D('',#150299,#117939,#117940) ;
#97034=AXIS2_PLACEMENT_3D('',#150305,#117944,#117945) ;
#97035=AXIS2_PLACEMENT_3D('',#150311,#117949,#117950) ;
#97036=AXIS2_PLACEMENT_3D('',#150320,#117955,#117956) ;
#97037=AXIS2_PLACEMENT_3D('',#150329,#117961,#117962) ;
#97038=AXIS2_PLACEMENT_3D('',#150338,#117967,#117968) ;
#97039=AXIS2_PLACEMENT_3D('',#150347,#117973,#117974) ;
#97040=AXIS2_PLACEMENT_3D('',#150356,#117979,#117980) ;
#97041=AXIS2_PLACEMENT_3D('',#150360,#117982,#117983) ;
#97042=AXIS2_PLACEMENT_3D('',#150362,#117984,#117985) ;
#97043=AXIS2_PLACEMENT_3D('',#150366,#117988,#117989) ;
#97044=AXIS2_PLACEMENT_3D('',#150370,#117991,#117992) ;
#97045=AXIS2_PLACEMENT_3D('',#150372,#117993,#117994) ;
#97046=AXIS2_PLACEMENT_3D('',#150376,#117997,#117998) ;
#97047=AXIS2_PLACEMENT_3D('',#150377,#117999,#118000) ;
#97048=AXIS2_PLACEMENT_3D('',#150378,#118001,#118002) ;
#97049=AXIS2_PLACEMENT_3D('',#150379,#118003,#118004) ;
#97050=AXIS2_PLACEMENT_3D('',#150380,#118005,#118006) ;
#97051=AXIS2_PLACEMENT_3D('',#150381,#118007,#118008) ;
#97052=AXIS2_PLACEMENT_3D('',#150382,#118009,#118010) ;
#97053=AXIS2_PLACEMENT_3D('',#150391,#118015,#118016) ;
#97054=AXIS2_PLACEMENT_3D('',#150397,#118020,#118021) ;
#97055=AXIS2_PLACEMENT_3D('',#150403,#118025,#118026) ;
#97056=AXIS2_PLACEMENT_3D('',#150412,#118031,#118032) ;
#97057=AXIS2_PLACEMENT_3D('',#150421,#118037,#118038) ;
#97058=AXIS2_PLACEMENT_3D('',#150427,#118042,#118043) ;
#97059=AXIS2_PLACEMENT_3D('',#150433,#118047,#118048) ;
#97060=AXIS2_PLACEMENT_3D('',#150442,#118053,#118054) ;
#97061=AXIS2_PLACEMENT_3D('',#150451,#118059,#118060) ;
#97062=AXIS2_PLACEMENT_3D('',#150460,#118065,#118066) ;
#97063=AXIS2_PLACEMENT_3D('',#150469,#118071,#118072) ;
#97064=AXIS2_PLACEMENT_3D('',#150478,#118077,#118078) ;
#97065=AXIS2_PLACEMENT_3D('',#150482,#118080,#118081) ;
#97066=AXIS2_PLACEMENT_3D('',#150484,#118082,#118083) ;
#97067=AXIS2_PLACEMENT_3D('',#150488,#118086,#118087) ;
#97068=AXIS2_PLACEMENT_3D('',#150492,#118089,#118090) ;
#97069=AXIS2_PLACEMENT_3D('',#150494,#118091,#118092) ;
#97070=AXIS2_PLACEMENT_3D('',#150498,#118095,#118096) ;
#97071=AXIS2_PLACEMENT_3D('',#150499,#118097,#118098) ;
#97072=AXIS2_PLACEMENT_3D('',#150500,#118099,#118100) ;
#97073=AXIS2_PLACEMENT_3D('',#150501,#118101,#118102) ;
#97074=AXIS2_PLACEMENT_3D('',#150502,#118103,#118104) ;
#97075=AXIS2_PLACEMENT_3D('',#150503,#118105,#118106) ;
#97076=AXIS2_PLACEMENT_3D('',#150504,#118107,#118108) ;
#97077=AXIS2_PLACEMENT_3D('',#150513,#118113,#118114) ;
#97078=AXIS2_PLACEMENT_3D('',#150519,#118118,#118119) ;
#97079=AXIS2_PLACEMENT_3D('',#150525,#118123,#118124) ;
#97080=AXIS2_PLACEMENT_3D('',#150534,#118129,#118130) ;
#97081=AXIS2_PLACEMENT_3D('',#150543,#118135,#118136) ;
#97082=AXIS2_PLACEMENT_3D('',#150549,#118140,#118141) ;
#97083=AXIS2_PLACEMENT_3D('',#150555,#118145,#118146) ;
#97084=AXIS2_PLACEMENT_3D('',#150564,#118151,#118152) ;
#97085=AXIS2_PLACEMENT_3D('',#150573,#118157,#118158) ;
#97086=AXIS2_PLACEMENT_3D('',#150582,#118163,#118164) ;
#97087=AXIS2_PLACEMENT_3D('',#150591,#118169,#118170) ;
#97088=AXIS2_PLACEMENT_3D('',#150600,#118175,#118176) ;
#97089=AXIS2_PLACEMENT_3D('',#150604,#118178,#118179) ;
#97090=AXIS2_PLACEMENT_3D('',#150606,#118180,#118181) ;
#97091=AXIS2_PLACEMENT_3D('',#150610,#118184,#118185) ;
#97092=AXIS2_PLACEMENT_3D('',#150614,#118187,#118188) ;
#97093=AXIS2_PLACEMENT_3D('',#150616,#118189,#118190) ;
#97094=AXIS2_PLACEMENT_3D('',#150620,#118193,#118194) ;
#97095=AXIS2_PLACEMENT_3D('',#150621,#118195,#118196) ;
#97096=AXIS2_PLACEMENT_3D('',#150622,#118197,#118198) ;
#97097=AXIS2_PLACEMENT_3D('',#150623,#118199,#118200) ;
#97098=AXIS2_PLACEMENT_3D('',#150624,#118201,#118202) ;
#97099=AXIS2_PLACEMENT_3D('',#150625,#118203,#118204) ;
#97100=AXIS2_PLACEMENT_3D('',#150626,#118205,#118206) ;
#97101=AXIS2_PLACEMENT_3D('',#150635,#118211,#118212) ;
#97102=AXIS2_PLACEMENT_3D('',#150641,#118216,#118217) ;
#97103=AXIS2_PLACEMENT_3D('',#150647,#118221,#118222) ;
#97104=AXIS2_PLACEMENT_3D('',#150656,#118227,#118228) ;
#97105=AXIS2_PLACEMENT_3D('',#150665,#118233,#118234) ;
#97106=AXIS2_PLACEMENT_3D('',#150671,#118238,#118239) ;
#97107=AXIS2_PLACEMENT_3D('',#150677,#118243,#118244) ;
#97108=AXIS2_PLACEMENT_3D('',#150686,#118249,#118250) ;
#97109=AXIS2_PLACEMENT_3D('',#150695,#118255,#118256) ;
#97110=AXIS2_PLACEMENT_3D('',#150704,#118261,#118262) ;
#97111=AXIS2_PLACEMENT_3D('',#150713,#118267,#118268) ;
#97112=AXIS2_PLACEMENT_3D('',#150722,#118273,#118274) ;
#97113=AXIS2_PLACEMENT_3D('',#150731,#118279,#118280) ;
#97114=AXIS2_PLACEMENT_3D('',#150740,#118285,#118286) ;
#97115=AXIS2_PLACEMENT_3D('',#150749,#118291,#118292) ;
#97116=AXIS2_PLACEMENT_3D('',#150758,#118297,#118298) ;
#97117=AXIS2_PLACEMENT_3D('',#150767,#118303,#118304) ;
#97118=AXIS2_PLACEMENT_3D('',#150776,#118309,#118310) ;
#97119=AXIS2_PLACEMENT_3D('',#150785,#118315,#118316) ;
#97120=AXIS2_PLACEMENT_3D('',#150794,#118321,#118322) ;
#97121=AXIS2_PLACEMENT_3D('',#150803,#118327,#118328) ;
#97122=AXIS2_PLACEMENT_3D('',#150812,#118333,#118334) ;
#97123=AXIS2_PLACEMENT_3D('',#150821,#118339,#118340) ;
#97124=AXIS2_PLACEMENT_3D('',#150830,#118345,#118346) ;
#97125=AXIS2_PLACEMENT_3D('',#150839,#118351,#118352) ;
#97126=AXIS2_PLACEMENT_3D('',#150848,#118357,#118358) ;
#97127=AXIS2_PLACEMENT_3D('',#150857,#118363,#118364) ;
#97128=AXIS2_PLACEMENT_3D('',#150866,#118369,#118370) ;
#97129=AXIS2_PLACEMENT_3D('',#150875,#118375,#118376) ;
#97130=AXIS2_PLACEMENT_3D('',#150884,#118381,#118382) ;
#97131=AXIS2_PLACEMENT_3D('',#150893,#118387,#118388) ;
#97132=AXIS2_PLACEMENT_3D('',#150902,#118393,#118394) ;
#97133=AXIS2_PLACEMENT_3D('',#150911,#118399,#118400) ;
#97134=AXIS2_PLACEMENT_3D('',#150920,#118405,#118406) ;
#97135=AXIS2_PLACEMENT_3D('',#150929,#118411,#118412) ;
#97136=AXIS2_PLACEMENT_3D('',#150938,#118417,#118418) ;
#97137=AXIS2_PLACEMENT_3D('',#150947,#118423,#118424) ;
#97138=AXIS2_PLACEMENT_3D('',#150956,#118429,#118430) ;
#97139=AXIS2_PLACEMENT_3D('',#150965,#118435,#118436) ;
#97140=AXIS2_PLACEMENT_3D('',#150974,#118441,#118442) ;
#97141=AXIS2_PLACEMENT_3D('',#150983,#118447,#118448) ;
#97142=AXIS2_PLACEMENT_3D('',#150992,#118453,#118454) ;
#97143=AXIS2_PLACEMENT_3D('',#151001,#118459,#118460) ;
#97144=AXIS2_PLACEMENT_3D('',#151002,#118461,#118462) ;
#97145=AXIS2_PLACEMENT_3D('',#151003,#118463,#118464) ;
#97146=AXIS2_PLACEMENT_3D('',#151004,#118465,#118466) ;
#97147=AXIS2_PLACEMENT_3D('',#151005,#118467,#118468) ;
#97148=AXIS2_PLACEMENT_3D('',#151006,#118469,#118470) ;
#97149=AXIS2_PLACEMENT_3D('',#151007,#118471,#118472) ;
#97150=AXIS2_PLACEMENT_3D('',#151008,#118473,#118474) ;
#97151=AXIS2_PLACEMENT_3D('',#151009,#118475,#118476) ;
#97152=AXIS2_PLACEMENT_3D('',#151010,#118477,#118478) ;
#97153=AXIS2_PLACEMENT_3D('',#151011,#118479,#118480) ;
#97154=AXIS2_PLACEMENT_3D('',#151012,#118481,#118482) ;
#97155=AXIS2_PLACEMENT_3D('',#151013,#118483,#118484) ;
#97156=AXIS2_PLACEMENT_3D('',#151014,#118485,#118486) ;
#97157=AXIS2_PLACEMENT_3D('',#151015,#118487,#118488) ;
#97158=AXIS2_PLACEMENT_3D('',#151016,#118489,#118490) ;
#97159=AXIS2_PLACEMENT_3D('',#151017,#118491,#118492) ;
#97160=AXIS2_PLACEMENT_3D('',#151018,#118493,#118494) ;
#97161=AXIS2_PLACEMENT_3D('',#151019,#118495,#118496) ;
#97162=AXIS2_PLACEMENT_3D('',#151020,#118497,#118498) ;
#97163=AXIS2_PLACEMENT_3D('',#151021,#118499,#118500) ;
#97164=AXIS2_PLACEMENT_3D('',#151022,#118501,#118502) ;
#97165=AXIS2_PLACEMENT_3D('',#151023,#118503,#118504) ;
#97166=AXIS2_PLACEMENT_3D('',#151024,#118505,#118506) ;
#97167=AXIS2_PLACEMENT_3D('',#151025,#118507,#118508) ;
#97168=AXIS2_PLACEMENT_3D('',#151026,#118509,#118510) ;
#97169=AXIS2_PLACEMENT_3D('',#151027,#118511,#118512) ;
#97170=AXIS2_PLACEMENT_3D('',#151028,#118513,#118514) ;
#97171=AXIS2_PLACEMENT_3D('',#151029,#118515,#118516) ;
#97172=AXIS2_PLACEMENT_3D('',#151030,#118517,#118518) ;
#97173=AXIS2_PLACEMENT_3D('',#151031,#118519,#118520) ;
#97174=AXIS2_PLACEMENT_3D('',#151032,#118521,#118522) ;
#97175=AXIS2_PLACEMENT_3D('',#151033,#118523,#118524) ;
#97176=AXIS2_PLACEMENT_3D('',#151034,#118525,#118526) ;
#97177=AXIS2_PLACEMENT_3D('',#151035,#118527,#118528) ;
#97178=AXIS2_PLACEMENT_3D('',#151036,#118529,#118530) ;
#97179=AXIS2_PLACEMENT_3D('',#151037,#118531,#118532) ;
#97180=AXIS2_PLACEMENT_3D('',#151038,#118533,#118534) ;
#97181=AXIS2_PLACEMENT_3D('',#151039,#118535,#118536) ;
#97182=AXIS2_PLACEMENT_3D('',#151040,#118537,#118538) ;
#97183=AXIS2_PLACEMENT_3D('',#151041,#118539,#118540) ;
#97184=AXIS2_PLACEMENT_3D('',#151042,#118541,#118542) ;
#97185=AXIS2_PLACEMENT_3D('',#151043,#118543,#118544) ;
#97186=AXIS2_PLACEMENT_3D('',#151044,#118545,#118546) ;
#97187=AXIS2_PLACEMENT_3D('',#151045,#118547,#118548) ;
#97188=AXIS2_PLACEMENT_3D('',#151046,#118549,#118550) ;
#97189=AXIS2_PLACEMENT_3D('',#151047,#118551,#118552) ;
#97190=AXIS2_PLACEMENT_3D('',#151048,#118553,#118554) ;
#97191=AXIS2_PLACEMENT_3D('',#151049,#118555,#118556) ;
#97192=AXIS2_PLACEMENT_3D('',#151050,#118557,#118558) ;
#97193=AXIS2_PLACEMENT_3D('',#151051,#118559,#118560) ;
#97194=AXIS2_PLACEMENT_3D('',#151052,#118561,#118562) ;
#97195=AXIS2_PLACEMENT_3D('',#151053,#118563,#118564) ;
#97196=AXIS2_PLACEMENT_3D('',#151054,#118565,#118566) ;
#97197=AXIS2_PLACEMENT_3D('',#151055,#118567,#118568) ;
#97198=AXIS2_PLACEMENT_3D('',#151056,#118569,#118570) ;
#97199=AXIS2_PLACEMENT_3D('',#151057,#118571,#118572) ;
#97200=AXIS2_PLACEMENT_3D('',#151058,#118573,#118574) ;
#97201=AXIS2_PLACEMENT_3D('',#151059,#118575,#118576) ;
#97202=AXIS2_PLACEMENT_3D('',#151060,#118577,#118578) ;
#97203=AXIS2_PLACEMENT_3D('',#151061,#118579,#118580) ;
#97204=AXIS2_PLACEMENT_3D('',#151062,#118581,#118582) ;
#97205=AXIS2_PLACEMENT_3D('',#151063,#118583,#118584) ;
#97206=AXIS2_PLACEMENT_3D('',#151064,#118585,#118586) ;
#97207=AXIS2_PLACEMENT_3D('',#151065,#118587,#118588) ;
#97208=AXIS2_PLACEMENT_3D('',#151066,#118589,#118590) ;
#97209=AXIS2_PLACEMENT_3D('',#151067,#118591,#118592) ;
#97210=AXIS2_PLACEMENT_3D('',#151068,#118593,#118594) ;
#97211=AXIS2_PLACEMENT_3D('',#151069,#118595,#118596) ;
#97212=AXIS2_PLACEMENT_3D('',#151070,#118597,#118598) ;
#97213=AXIS2_PLACEMENT_3D('',#151071,#118599,#118600) ;
#97214=AXIS2_PLACEMENT_3D('',#151072,#118601,#118602) ;
#97215=AXIS2_PLACEMENT_3D('',#151073,#118603,#118604) ;
#97216=AXIS2_PLACEMENT_3D('',#151074,#118605,#118606) ;
#97217=AXIS2_PLACEMENT_3D('',#151075,#118607,#118608) ;
#97218=AXIS2_PLACEMENT_3D('',#151076,#118609,#118610) ;
#97219=AXIS2_PLACEMENT_3D('',#151077,#118611,#118612) ;
#97220=AXIS2_PLACEMENT_3D('',#151078,#118613,#118614) ;
#97221=AXIS2_PLACEMENT_3D('',#151079,#118615,#118616) ;
#97222=AXIS2_PLACEMENT_3D('',#151080,#118617,#118618) ;
#97223=AXIS2_PLACEMENT_3D('',#151081,#118619,#118620) ;
#97224=AXIS2_PLACEMENT_3D('',#151082,#118621,#118622) ;
#97225=AXIS2_PLACEMENT_3D('',#151083,#118623,#118624) ;
#97226=AXIS2_PLACEMENT_3D('',#151084,#118625,#118626) ;
#97227=AXIS2_PLACEMENT_3D('',#151085,#118627,#118628) ;
#97228=AXIS2_PLACEMENT_3D('',#151086,#118629,#118630) ;
#97229=AXIS2_PLACEMENT_3D('',#151087,#118631,#118632) ;
#97230=AXIS2_PLACEMENT_3D('',#151088,#118633,#118634) ;
#97231=AXIS2_PLACEMENT_3D('',#151089,#118635,#118636) ;
#97232=AXIS2_PLACEMENT_3D('',#151090,#118637,#118638) ;
#97233=AXIS2_PLACEMENT_3D('',#151091,#118639,#118640) ;
#97234=AXIS2_PLACEMENT_3D('',#151092,#118641,#118642) ;
#97235=AXIS2_PLACEMENT_3D('',#151093,#118643,#118644) ;
#97236=AXIS2_PLACEMENT_3D('',#151094,#118645,#118646) ;
#97237=AXIS2_PLACEMENT_3D('',#151095,#118647,#118648) ;
#97238=AXIS2_PLACEMENT_3D('',#151096,#118649,#118650) ;
#97239=AXIS2_PLACEMENT_3D('',#151097,#118651,#118652) ;
#97240=AXIS2_PLACEMENT_3D('',#151098,#118653,#118654) ;
#97241=AXIS2_PLACEMENT_3D('',#151099,#118655,#118656) ;
#97242=AXIS2_PLACEMENT_3D('',#151100,#118657,#118658) ;
#97243=AXIS2_PLACEMENT_3D('',#151101,#118659,#118660) ;
#97244=AXIS2_PLACEMENT_3D('',#151102,#118661,#118662) ;
#97245=AXIS2_PLACEMENT_3D('',#151103,#118663,#118664) ;
#97246=AXIS2_PLACEMENT_3D('',#151104,#118665,#118666) ;
#97247=AXIS2_PLACEMENT_3D('',#151105,#118667,#118668) ;
#97248=AXIS2_PLACEMENT_3D('',#151106,#118669,#118670) ;
#97249=AXIS2_PLACEMENT_3D('',#151107,#118671,#118672) ;
#97250=AXIS2_PLACEMENT_3D('',#151108,#118673,#118674) ;
#97251=AXIS2_PLACEMENT_3D('',#151109,#118675,#118676) ;
#97252=AXIS2_PLACEMENT_3D('',#151110,#118677,#118678) ;
#97253=AXIS2_PLACEMENT_3D('',#151111,#118679,#118680) ;
#97254=AXIS2_PLACEMENT_3D('',#151112,#118681,#118682) ;
#97255=AXIS2_PLACEMENT_3D('',#151113,#118683,#118684) ;
#97256=AXIS2_PLACEMENT_3D('',#151114,#118685,#118686) ;
#97257=AXIS2_PLACEMENT_3D('',#151115,#118687,#118688) ;
#97258=AXIS2_PLACEMENT_3D('',#151116,#118689,#118690) ;
#97259=AXIS2_PLACEMENT_3D('',#151117,#118691,#118692) ;
#97260=AXIS2_PLACEMENT_3D('',#151118,#118693,#118694) ;
#97261=AXIS2_PLACEMENT_3D('',#151119,#118695,#118696) ;
#97262=AXIS2_PLACEMENT_3D('',#151120,#118697,#118698) ;
#97263=AXIS2_PLACEMENT_3D('',#151121,#118699,#118700) ;
#97264=AXIS2_PLACEMENT_3D('',#151122,#118701,#118702) ;
#97265=AXIS2_PLACEMENT_3D('',#151123,#118703,#118704) ;
#97266=AXIS2_PLACEMENT_3D('',#151124,#118705,#118706) ;
#97267=AXIS2_PLACEMENT_3D('',#151125,#118707,#118708) ;
#97268=AXIS2_PLACEMENT_3D('',#151126,#118709,#118710) ;
#97269=AXIS2_PLACEMENT_3D('',#151127,#118711,#118712) ;
#97270=AXIS2_PLACEMENT_3D('',#151128,#118713,#118714) ;
#97271=AXIS2_PLACEMENT_3D('',#151129,#118715,#118716) ;
#97272=AXIS2_PLACEMENT_3D('',#151130,#118717,#118718) ;
#97273=AXIS2_PLACEMENT_3D('',#151131,#118719,#118720) ;
#97274=AXIS2_PLACEMENT_3D('',#151132,#118721,#118722) ;
#97275=AXIS2_PLACEMENT_3D('',#151133,#118723,#118724) ;
#97276=AXIS2_PLACEMENT_3D('',#151134,#118725,#118726) ;
#97277=AXIS2_PLACEMENT_3D('',#151135,#118727,#118728) ;
#97278=AXIS2_PLACEMENT_3D('',#151136,#118729,#118730) ;
#97279=AXIS2_PLACEMENT_3D('',#151137,#118731,#118732) ;
#97280=AXIS2_PLACEMENT_3D('',#151138,#118733,#118734) ;
#97281=AXIS2_PLACEMENT_3D('',#151139,#118735,#118736) ;
#97282=AXIS2_PLACEMENT_3D('',#151140,#118737,#118738) ;
#97283=AXIS2_PLACEMENT_3D('',#151141,#118739,#118740) ;
#97284=AXIS2_PLACEMENT_3D('',#151142,#118741,#118742) ;
#97285=AXIS2_PLACEMENT_3D('',#151143,#118743,#118744) ;
#97286=AXIS2_PLACEMENT_3D('',#151144,#118745,#118746) ;
#97287=AXIS2_PLACEMENT_3D('',#151145,#118747,#118748) ;
#97288=AXIS2_PLACEMENT_3D('',#151146,#118749,#118750) ;
#97289=AXIS2_PLACEMENT_3D('',#151147,#118751,#118752) ;
#97290=AXIS2_PLACEMENT_3D('',#151148,#118753,#118754) ;
#97291=AXIS2_PLACEMENT_3D('',#151149,#118755,#118756) ;
#97292=AXIS2_PLACEMENT_3D('',#151150,#118757,#118758) ;
#97293=AXIS2_PLACEMENT_3D('',#151151,#118759,#118760) ;
#97294=AXIS2_PLACEMENT_3D('',#151152,#118761,#118762) ;
#97295=AXIS2_PLACEMENT_3D('',#151153,#118763,#118764) ;
#97296=AXIS2_PLACEMENT_3D('',#151154,#118765,#118766) ;
#97297=AXIS2_PLACEMENT_3D('',#151155,#118767,#118768) ;
#97298=AXIS2_PLACEMENT_3D('',#151156,#118769,#118770) ;
#97299=AXIS2_PLACEMENT_3D('',#151157,#118771,#118772) ;
#97300=AXIS2_PLACEMENT_3D('',#151158,#118773,#118774) ;
#97301=AXIS2_PLACEMENT_3D('',#151159,#118775,#118776) ;
#97302=AXIS2_PLACEMENT_3D('',#151160,#118777,#118778) ;
#97303=AXIS2_PLACEMENT_3D('',#151161,#118779,#118780) ;
#97304=AXIS2_PLACEMENT_3D('',#151162,#118781,#118782) ;
#97305=AXIS2_PLACEMENT_3D('',#151163,#118783,#118784) ;
#97306=AXIS2_PLACEMENT_3D('',#151164,#118785,#118786) ;
#97307=AXIS2_PLACEMENT_3D('',#151165,#118787,#118788) ;
#97308=AXIS2_PLACEMENT_3D('',#151166,#118789,#118790) ;
#97309=AXIS2_PLACEMENT_3D('',#151167,#118791,#118792) ;
#97310=AXIS2_PLACEMENT_3D('',#151168,#118793,#118794) ;
#97311=AXIS2_PLACEMENT_3D('',#151169,#118795,#118796) ;
#97312=AXIS2_PLACEMENT_3D('',#151170,#118797,#118798) ;
#97313=AXIS2_PLACEMENT_3D('',#151171,#118799,#118800) ;
#97314=AXIS2_PLACEMENT_3D('',#151172,#118801,#118802) ;
#97315=AXIS2_PLACEMENT_3D('',#151173,#118803,#118804) ;
#97316=AXIS2_PLACEMENT_3D('',#151174,#118805,#118806) ;
#97317=AXIS2_PLACEMENT_3D('',#151175,#118807,#118808) ;
#97318=AXIS2_PLACEMENT_3D('',#151176,#118809,#118810) ;
#97319=AXIS2_PLACEMENT_3D('',#151177,#118811,#118812) ;
#97320=AXIS2_PLACEMENT_3D('',#151178,#118813,#118814) ;
#97321=AXIS2_PLACEMENT_3D('',#151179,#118815,#118816) ;
#97322=AXIS2_PLACEMENT_3D('',#151180,#118817,#118818) ;
#97323=AXIS2_PLACEMENT_3D('',#151181,#118819,#118820) ;
#97324=AXIS2_PLACEMENT_3D('',#151182,#118821,#118822) ;
#97325=AXIS2_PLACEMENT_3D('',#151183,#118823,#118824) ;
#97326=AXIS2_PLACEMENT_3D('',#151184,#118825,#118826) ;
#97327=AXIS2_PLACEMENT_3D('',#151185,#118827,#118828) ;
#97328=AXIS2_PLACEMENT_3D('',#151186,#118829,#118830) ;
#97329=AXIS2_PLACEMENT_3D('',#151187,#118831,#118832) ;
#97330=AXIS2_PLACEMENT_3D('',#151188,#118833,#118834) ;
#97331=AXIS2_PLACEMENT_3D('',#151189,#118835,#118836) ;
#97332=AXIS2_PLACEMENT_3D('',#151190,#118837,#118838) ;
#97333=AXIS2_PLACEMENT_3D('',#151191,#118839,#118840) ;
#97334=AXIS2_PLACEMENT_3D('',#151192,#118841,#118842) ;
#97335=AXIS2_PLACEMENT_3D('',#151193,#118843,#118844) ;
#97336=AXIS2_PLACEMENT_3D('',#151194,#118845,#118846) ;
#97337=AXIS2_PLACEMENT_3D('',#151195,#118847,#118848) ;
#97338=AXIS2_PLACEMENT_3D('',#151196,#118849,#118850) ;
#97339=AXIS2_PLACEMENT_3D('',#151197,#118851,#118852) ;
#97340=AXIS2_PLACEMENT_3D('',#151198,#118853,#118854) ;
#97341=AXIS2_PLACEMENT_3D('',#151199,#118855,#118856) ;
#97342=AXIS2_PLACEMENT_3D('',#151200,#118857,#118858) ;
#97343=AXIS2_PLACEMENT_3D('',#151201,#118859,#118860) ;
#97344=AXIS2_PLACEMENT_3D('',#151202,#118861,#118862) ;
#97345=AXIS2_PLACEMENT_3D('',#151203,#118863,#118864) ;
#97346=AXIS2_PLACEMENT_3D('',#151204,#118865,#118866) ;
#97347=AXIS2_PLACEMENT_3D('',#151205,#118867,#118868) ;
#97348=AXIS2_PLACEMENT_3D('',#151206,#118869,#118870) ;
#97349=AXIS2_PLACEMENT_3D('',#151207,#118871,#118872) ;
#97350=AXIS2_PLACEMENT_3D('',#151208,#118873,#118874) ;
#97351=AXIS2_PLACEMENT_3D('',#151209,#118875,#118876) ;
#97352=AXIS2_PLACEMENT_3D('',#151210,#118877,#118878) ;
#97353=AXIS2_PLACEMENT_3D('',#151211,#118879,#118880) ;
#97354=AXIS2_PLACEMENT_3D('',#151212,#118881,#118882) ;
#97355=AXIS2_PLACEMENT_3D('',#151213,#118883,#118884) ;
#97356=AXIS2_PLACEMENT_3D('',#151214,#118885,#118886) ;
#97357=AXIS2_PLACEMENT_3D('',#151215,#118887,#118888) ;
#97358=AXIS2_PLACEMENT_3D('',#151216,#118889,#118890) ;
#97359=AXIS2_PLACEMENT_3D('',#151217,#118891,#118892) ;
#97360=AXIS2_PLACEMENT_3D('',#151218,#118893,#118894) ;
#97361=AXIS2_PLACEMENT_3D('',#151219,#118895,#118896) ;
#97362=AXIS2_PLACEMENT_3D('',#151220,#118897,#118898) ;
#97363=AXIS2_PLACEMENT_3D('',#151221,#118899,#118900) ;
#97364=AXIS2_PLACEMENT_3D('',#151222,#118901,#118902) ;
#97365=AXIS2_PLACEMENT_3D('',#151223,#118903,#118904) ;
#97366=AXIS2_PLACEMENT_3D('',#151224,#118905,#118906) ;
#97367=AXIS2_PLACEMENT_3D('',#151225,#118907,#118908) ;
#97368=AXIS2_PLACEMENT_3D('',#151226,#118909,#118910) ;
#97369=AXIS2_PLACEMENT_3D('',#151227,#118911,#118912) ;
#97370=AXIS2_PLACEMENT_3D('',#151228,#118913,#118914) ;
#97371=AXIS2_PLACEMENT_3D('',#151229,#118915,#118916) ;
#97372=AXIS2_PLACEMENT_3D('',#151230,#118917,#118918) ;
#97373=AXIS2_PLACEMENT_3D('',#151231,#118919,#118920) ;
#97374=AXIS2_PLACEMENT_3D('',#151232,#118921,#118922) ;
#97375=AXIS2_PLACEMENT_3D('',#151233,#118923,#118924) ;
#97376=AXIS2_PLACEMENT_3D('',#151234,#118925,#118926) ;
#97377=AXIS2_PLACEMENT_3D('',#151235,#118927,#118928) ;
#97378=AXIS2_PLACEMENT_3D('',#151236,#118929,#118930) ;
#97379=AXIS2_PLACEMENT_3D('',#151237,#118931,#118932) ;
#97380=AXIS2_PLACEMENT_3D('',#151238,#118933,#118934) ;
#97381=AXIS2_PLACEMENT_3D('',#151239,#118935,#118936) ;
#97382=AXIS2_PLACEMENT_3D('',#151240,#118937,#118938) ;
#97383=AXIS2_PLACEMENT_3D('',#151241,#118939,#118940) ;
#97384=AXIS2_PLACEMENT_3D('',#151242,#118941,#118942) ;
#97385=AXIS2_PLACEMENT_3D('',#151243,#118943,#118944) ;
#97386=AXIS2_PLACEMENT_3D('',#151244,#118945,#118946) ;
#97387=AXIS2_PLACEMENT_3D('',#151245,#118947,#118948) ;
#97388=AXIS2_PLACEMENT_3D('',#151246,#118949,#118950) ;
#97389=AXIS2_PLACEMENT_3D('',#151247,#118951,#118952) ;
#97390=AXIS2_PLACEMENT_3D('',#151248,#118953,#118954) ;
#97391=AXIS2_PLACEMENT_3D('',#151249,#118955,#118956) ;
#97392=AXIS2_PLACEMENT_3D('',#151250,#118957,#118958) ;
#97393=AXIS2_PLACEMENT_3D('',#151251,#118959,#118960) ;
#97394=AXIS2_PLACEMENT_3D('',#151252,#118961,#118962) ;
#97395=AXIS2_PLACEMENT_3D('',#151253,#118963,#118964) ;
#97396=AXIS2_PLACEMENT_3D('',#151254,#118965,#118966) ;
#97397=AXIS2_PLACEMENT_3D('',#151255,#118967,#118968) ;
#97398=AXIS2_PLACEMENT_3D('',#151256,#118969,#118970) ;
#97399=AXIS2_PLACEMENT_3D('',#151257,#118971,#118972) ;
#97400=AXIS2_PLACEMENT_3D('',#151258,#118973,#118974) ;
#97401=AXIS2_PLACEMENT_3D('',#151259,#118975,#118976) ;
#97402=AXIS2_PLACEMENT_3D('',#151260,#118977,#118978) ;
#97403=AXIS2_PLACEMENT_3D('',#151261,#118979,#118980) ;
#97404=AXIS2_PLACEMENT_3D('',#151262,#118981,#118982) ;
#97405=AXIS2_PLACEMENT_3D('',#151263,#118983,#118984) ;
#97406=AXIS2_PLACEMENT_3D('',#151264,#118985,#118986) ;
#97407=AXIS2_PLACEMENT_3D('',#151265,#118987,#118988) ;
#97408=AXIS2_PLACEMENT_3D('',#151266,#118989,#118990) ;
#97409=AXIS2_PLACEMENT_3D('',#151267,#118991,#118992) ;
#97410=AXIS2_PLACEMENT_3D('',#151268,#118993,#118994) ;
#97411=AXIS2_PLACEMENT_3D('',#151269,#118995,#118996) ;
#97412=AXIS2_PLACEMENT_3D('',#151270,#118997,#118998) ;
#97413=AXIS2_PLACEMENT_3D('',#151271,#118999,#119000) ;
#97414=AXIS2_PLACEMENT_3D('',#151272,#119001,#119002) ;
#97415=AXIS2_PLACEMENT_3D('',#151273,#119003,#119004) ;
#97416=AXIS2_PLACEMENT_3D('',#151274,#119005,#119006) ;
#97417=AXIS2_PLACEMENT_3D('',#151275,#119007,#119008) ;
#97418=AXIS2_PLACEMENT_3D('',#151276,#119009,#119010) ;
#97419=AXIS2_PLACEMENT_3D('',#151277,#119011,#119012) ;
#97420=AXIS2_PLACEMENT_3D('',#151278,#119013,#119014) ;
#97421=AXIS2_PLACEMENT_3D('',#151279,#119015,#119016) ;
#97422=AXIS2_PLACEMENT_3D('',#151280,#119017,#119018) ;
#97423=AXIS2_PLACEMENT_3D('',#151281,#119019,#119020) ;
#97424=AXIS2_PLACEMENT_3D('',#151282,#119021,#119022) ;
#97425=AXIS2_PLACEMENT_3D('',#151283,#119023,#119024) ;
#97426=AXIS2_PLACEMENT_3D('',#151284,#119025,#119026) ;
#97427=AXIS2_PLACEMENT_3D('',#151285,#119027,#119028) ;
#97428=AXIS2_PLACEMENT_3D('',#151286,#119029,#119030) ;
#97429=AXIS2_PLACEMENT_3D('',#151287,#119031,#119032) ;
#97430=AXIS2_PLACEMENT_3D('',#151288,#119033,#119034) ;
#97431=AXIS2_PLACEMENT_3D('',#151289,#119035,#119036) ;
#97432=AXIS2_PLACEMENT_3D('',#151290,#119037,#119038) ;
#97433=AXIS2_PLACEMENT_3D('',#151291,#119039,#119040) ;
#97434=AXIS2_PLACEMENT_3D('',#151292,#119041,#119042) ;
#97435=AXIS2_PLACEMENT_3D('',#151293,#119043,#119044) ;
#97436=AXIS2_PLACEMENT_3D('',#151294,#119045,#119046) ;
#97437=AXIS2_PLACEMENT_3D('',#151295,#119047,#119048) ;
#97438=AXIS2_PLACEMENT_3D('',#151296,#119049,#119050) ;
#97439=AXIS2_PLACEMENT_3D('',#151297,#119051,#119052) ;
#97440=AXIS2_PLACEMENT_3D('',#151298,#119053,#119054) ;
#97441=AXIS2_PLACEMENT_3D('',#151299,#119055,#119056) ;
#97442=AXIS2_PLACEMENT_3D('',#151300,#119057,#119058) ;
#97443=AXIS2_PLACEMENT_3D('',#151301,#119059,#119060) ;
#97444=AXIS2_PLACEMENT_3D('',#151302,#119061,#119062) ;
#97445=AXIS2_PLACEMENT_3D('',#151303,#119063,#119064) ;
#97446=AXIS2_PLACEMENT_3D('',#151304,#119065,#119066) ;
#97447=AXIS2_PLACEMENT_3D('',#151305,#119067,#119068) ;
#97448=AXIS2_PLACEMENT_3D('',#151306,#119069,#119070) ;
#97449=AXIS2_PLACEMENT_3D('',#151307,#119071,#119072) ;
#97450=AXIS2_PLACEMENT_3D('',#151308,#119073,#119074) ;
#97451=AXIS2_PLACEMENT_3D('',#151309,#119075,#119076) ;
#97452=AXIS2_PLACEMENT_3D('',#151310,#119077,#119078) ;
#97453=AXIS2_PLACEMENT_3D('',#151311,#119079,#119080) ;
#97454=AXIS2_PLACEMENT_3D('',#151312,#119081,#119082) ;
#97455=AXIS2_PLACEMENT_3D('',#151313,#119083,#119084) ;
#97456=AXIS2_PLACEMENT_3D('',#151314,#119085,#119086) ;
#97457=AXIS2_PLACEMENT_3D('',#151315,#119087,#119088) ;
#97458=AXIS2_PLACEMENT_3D('',#151316,#119089,#119090) ;
#97459=AXIS2_PLACEMENT_3D('',#151317,#119091,#119092) ;
#97460=AXIS2_PLACEMENT_3D('',#151318,#119093,#119094) ;
#97461=AXIS2_PLACEMENT_3D('',#151319,#119095,#119096) ;
#97462=AXIS2_PLACEMENT_3D('',#151320,#119097,#119098) ;
#97463=AXIS2_PLACEMENT_3D('',#151321,#119099,#119100) ;
#97464=AXIS2_PLACEMENT_3D('',#151322,#119101,#119102) ;
#97465=AXIS2_PLACEMENT_3D('',#151323,#119103,#119104) ;
#97466=AXIS2_PLACEMENT_3D('',#151324,#119105,#119106) ;
#97467=AXIS2_PLACEMENT_3D('',#151325,#119107,#119108) ;
#97468=AXIS2_PLACEMENT_3D('',#151326,#119109,#119110) ;
#97469=AXIS2_PLACEMENT_3D('',#151327,#119111,#119112) ;
#97470=AXIS2_PLACEMENT_3D('',#151328,#119113,#119114) ;
#97471=AXIS2_PLACEMENT_3D('',#151329,#119115,#119116) ;
#97472=AXIS2_PLACEMENT_3D('',#151330,#119117,#119118) ;
#97473=AXIS2_PLACEMENT_3D('',#151331,#119119,#119120) ;
#97474=AXIS2_PLACEMENT_3D('',#151332,#119121,#119122) ;
#97475=AXIS2_PLACEMENT_3D('',#151333,#119123,#119124) ;
#97476=AXIS2_PLACEMENT_3D('',#151334,#119125,#119126) ;
#97477=AXIS2_PLACEMENT_3D('',#151335,#119127,#119128) ;
#97478=AXIS2_PLACEMENT_3D('',#151336,#119129,#119130) ;
#97479=AXIS2_PLACEMENT_3D('',#151337,#119131,#119132) ;
#97480=AXIS2_PLACEMENT_3D('',#151338,#119133,#119134) ;
#97481=AXIS2_PLACEMENT_3D('',#151339,#119135,#119136) ;
#97482=AXIS2_PLACEMENT_3D('',#151340,#119137,#119138) ;
#97483=AXIS2_PLACEMENT_3D('',#151341,#119139,#119140) ;
#97484=AXIS2_PLACEMENT_3D('',#151342,#119141,#119142) ;
#97485=AXIS2_PLACEMENT_3D('',#151343,#119143,#119144) ;
#97486=AXIS2_PLACEMENT_3D('',#151344,#119145,#119146) ;
#97487=AXIS2_PLACEMENT_3D('',#151345,#119147,#119148) ;
#97488=AXIS2_PLACEMENT_3D('',#151346,#119149,#119150) ;
#97489=AXIS2_PLACEMENT_3D('',#151347,#119151,#119152) ;
#97490=AXIS2_PLACEMENT_3D('',#151348,#119153,#119154) ;
#97491=AXIS2_PLACEMENT_3D('',#151349,#119155,#119156) ;
#97492=AXIS2_PLACEMENT_3D('',#151350,#119157,#119158) ;
#97493=AXIS2_PLACEMENT_3D('',#151351,#119159,#119160) ;
#97494=AXIS2_PLACEMENT_3D('',#151352,#119161,#119162) ;
#97495=AXIS2_PLACEMENT_3D('',#151353,#119163,#119164) ;
#97496=AXIS2_PLACEMENT_3D('',#151354,#119165,#119166) ;
#97497=AXIS2_PLACEMENT_3D('',#151355,#119167,#119168) ;
#97498=AXIS2_PLACEMENT_3D('',#151356,#119169,#119170) ;
#97499=AXIS2_PLACEMENT_3D('',#151357,#119171,#119172) ;
#97500=AXIS2_PLACEMENT_3D('',#151358,#119173,#119174) ;
#97501=AXIS2_PLACEMENT_3D('',#151359,#119175,#119176) ;
#97502=AXIS2_PLACEMENT_3D('',#151360,#119177,#119178) ;
#97503=AXIS2_PLACEMENT_3D('',#151361,#119179,#119180) ;
#97504=AXIS2_PLACEMENT_3D('',#151362,#119181,#119182) ;
#97505=AXIS2_PLACEMENT_3D('',#151363,#119183,#119184) ;
#97506=AXIS2_PLACEMENT_3D('',#151364,#119185,#119186) ;
#97507=AXIS2_PLACEMENT_3D('',#151365,#119187,#119188) ;
#97508=AXIS2_PLACEMENT_3D('',#151366,#119189,#119190) ;
#97509=AXIS2_PLACEMENT_3D('',#151367,#119191,#119192) ;
#97510=AXIS2_PLACEMENT_3D('',#151368,#119193,#119194) ;
#97511=AXIS2_PLACEMENT_3D('',#151369,#119195,#119196) ;
#97512=AXIS2_PLACEMENT_3D('',#151370,#119197,#119198) ;
#97513=AXIS2_PLACEMENT_3D('',#151371,#119199,#119200) ;
#97514=AXIS2_PLACEMENT_3D('',#151372,#119201,#119202) ;
#97515=AXIS2_PLACEMENT_3D('',#151373,#119203,#119204) ;
#97516=AXIS2_PLACEMENT_3D('',#151374,#119205,#119206) ;
#97517=AXIS2_PLACEMENT_3D('',#151375,#119207,#119208) ;
#97518=AXIS2_PLACEMENT_3D('',#151376,#119209,#119210) ;
#97519=AXIS2_PLACEMENT_3D('',#151377,#119211,#119212) ;
#97520=AXIS2_PLACEMENT_3D('',#151378,#119213,#119214) ;
#97521=AXIS2_PLACEMENT_3D('',#151379,#119215,#119216) ;
#97522=AXIS2_PLACEMENT_3D('',#151380,#119217,#119218) ;
#97523=AXIS2_PLACEMENT_3D('',#151381,#119219,#119220) ;
#97524=AXIS2_PLACEMENT_3D('',#151382,#119221,#119222) ;
#97525=AXIS2_PLACEMENT_3D('',#151383,#119223,#119224) ;
#97526=AXIS2_PLACEMENT_3D('',#151384,#119225,#119226) ;
#97527=AXIS2_PLACEMENT_3D('',#151385,#119227,#119228) ;
#97528=AXIS2_PLACEMENT_3D('',#151386,#119229,#119230) ;
#97529=AXIS2_PLACEMENT_3D('',#151387,#119231,#119232) ;
#97530=AXIS2_PLACEMENT_3D('',#151388,#119233,#119234) ;
#97531=AXIS2_PLACEMENT_3D('',#151389,#119235,#119236) ;
#97532=AXIS2_PLACEMENT_3D('',#151390,#119237,#119238) ;
#97533=AXIS2_PLACEMENT_3D('',#151391,#119239,#119240) ;
#97534=AXIS2_PLACEMENT_3D('',#151392,#119241,#119242) ;
#97535=AXIS2_PLACEMENT_3D('',#151393,#119243,#119244) ;
#97536=AXIS2_PLACEMENT_3D('',#151394,#119245,#119246) ;
#97537=AXIS2_PLACEMENT_3D('',#151395,#119247,#119248) ;
#97538=AXIS2_PLACEMENT_3D('',#151396,#119249,#119250) ;
#97539=AXIS2_PLACEMENT_3D('',#151397,#119251,#119252) ;
#97540=AXIS2_PLACEMENT_3D('',#151398,#119253,#119254) ;
#97541=AXIS2_PLACEMENT_3D('',#151399,#119255,#119256) ;
#97542=AXIS2_PLACEMENT_3D('',#151400,#119257,#119258) ;
#97543=AXIS2_PLACEMENT_3D('',#151401,#119259,#119260) ;
#97544=AXIS2_PLACEMENT_3D('',#151402,#119261,#119262) ;
#97545=AXIS2_PLACEMENT_3D('',#151403,#119263,#119264) ;
#97546=AXIS2_PLACEMENT_3D('',#151404,#119265,#119266) ;
#97547=AXIS2_PLACEMENT_3D('',#151405,#119267,#119268) ;
#97548=AXIS2_PLACEMENT_3D('',#151406,#119269,#119270) ;
#97549=AXIS2_PLACEMENT_3D('',#151407,#119271,#119272) ;
#97550=AXIS2_PLACEMENT_3D('',#151408,#119273,#119274) ;
#97551=AXIS2_PLACEMENT_3D('',#151409,#119275,#119276) ;
#97552=AXIS2_PLACEMENT_3D('',#151410,#119277,#119278) ;
#97553=AXIS2_PLACEMENT_3D('',#151411,#119279,#119280) ;
#97554=AXIS2_PLACEMENT_3D('',#151412,#119281,#119282) ;
#97555=AXIS2_PLACEMENT_3D('',#151413,#119283,#119284) ;
#97556=AXIS2_PLACEMENT_3D('',#151414,#119285,#119286) ;
#97557=AXIS2_PLACEMENT_3D('',#151415,#119287,#119288) ;
#97558=AXIS2_PLACEMENT_3D('',#151416,#119289,#119290) ;
#97559=AXIS2_PLACEMENT_3D('',#151417,#119291,#119292) ;
#97560=AXIS2_PLACEMENT_3D('',#151418,#119293,#119294) ;
#97561=AXIS2_PLACEMENT_3D('',#151419,#119295,#119296) ;
#97562=AXIS2_PLACEMENT_3D('',#151420,#119297,#119298) ;
#97563=AXIS2_PLACEMENT_3D('',#151421,#119299,#119300) ;
#97564=AXIS2_PLACEMENT_3D('',#151422,#119301,#119302) ;
#97565=AXIS2_PLACEMENT_3D('',#151423,#119303,#119304) ;
#97566=AXIS2_PLACEMENT_3D('',#151424,#119305,#119306) ;
#97567=AXIS2_PLACEMENT_3D('',#151425,#119307,#119308) ;
#97568=AXIS2_PLACEMENT_3D('',#151426,#119309,#119310) ;
#97569=AXIS2_PLACEMENT_3D('',#151427,#119311,#119312) ;
#97570=AXIS2_PLACEMENT_3D('',#151428,#119313,#119314) ;
#97571=AXIS2_PLACEMENT_3D('',#151429,#119315,#119316) ;
#97572=AXIS2_PLACEMENT_3D('',#151430,#119317,#119318) ;
#97573=AXIS2_PLACEMENT_3D('',#151431,#119319,#119320) ;
#97574=AXIS2_PLACEMENT_3D('',#151432,#119321,#119322) ;
#97575=AXIS2_PLACEMENT_3D('',#151433,#119323,#119324) ;
#97576=AXIS2_PLACEMENT_3D('',#151434,#119325,#119326) ;
#97577=AXIS2_PLACEMENT_3D('',#151435,#119327,#119328) ;
#97578=AXIS2_PLACEMENT_3D('',#151436,#119329,#119330) ;
#97579=AXIS2_PLACEMENT_3D('',#151437,#119331,#119332) ;
#97580=AXIS2_PLACEMENT_3D('',#151438,#119333,#119334) ;
#97581=AXIS2_PLACEMENT_3D('',#151439,#119335,#119336) ;
#97582=AXIS2_PLACEMENT_3D('',#151440,#119337,#119338) ;
#97583=AXIS2_PLACEMENT_3D('',#151441,#119339,#119340) ;
#97584=AXIS2_PLACEMENT_3D('',#151442,#119341,#119342) ;
#97585=AXIS2_PLACEMENT_3D('',#151443,#119343,#119344) ;
#97586=AXIS2_PLACEMENT_3D('',#151444,#119345,#119346) ;
#97587=AXIS2_PLACEMENT_3D('',#151445,#119347,#119348) ;
#97588=AXIS2_PLACEMENT_3D('',#151446,#119349,#119350) ;
#97589=AXIS2_PLACEMENT_3D('',#151447,#119351,#119352) ;
#97590=AXIS2_PLACEMENT_3D('',#151448,#119353,#119354) ;
#97591=AXIS2_PLACEMENT_3D('',#151449,#119355,#119356) ;
#97592=AXIS2_PLACEMENT_3D('',#151450,#119357,#119358) ;
#97593=AXIS2_PLACEMENT_3D('',#151451,#119359,#119360) ;
#97594=AXIS2_PLACEMENT_3D('',#151452,#119361,#119362) ;
#97595=AXIS2_PLACEMENT_3D('',#151453,#119363,#119364) ;
#97596=AXIS2_PLACEMENT_3D('',#151454,#119365,#119366) ;
#97597=AXIS2_PLACEMENT_3D('',#151455,#119367,#119368) ;
#97598=AXIS2_PLACEMENT_3D('',#151456,#119369,#119370) ;
#97599=AXIS2_PLACEMENT_3D('',#151457,#119371,#119372) ;
#97600=AXIS2_PLACEMENT_3D('',#151458,#119373,#119374) ;
#97601=AXIS2_PLACEMENT_3D('',#151459,#119375,#119376) ;
#97602=AXIS2_PLACEMENT_3D('',#151460,#119377,#119378) ;
#97603=AXIS2_PLACEMENT_3D('',#151461,#119379,#119380) ;
#97604=AXIS2_PLACEMENT_3D('',#151462,#119381,#119382) ;
#97605=AXIS2_PLACEMENT_3D('',#151463,#119383,#119384) ;
#97606=AXIS2_PLACEMENT_3D('',#151464,#119385,#119386) ;
#97607=AXIS2_PLACEMENT_3D('',#151465,#119387,#119388) ;
#97608=AXIS2_PLACEMENT_3D('',#151466,#119389,#119390) ;
#97609=AXIS2_PLACEMENT_3D('',#151467,#119391,#119392) ;
#97610=AXIS2_PLACEMENT_3D('',#151468,#119393,#119394) ;
#97611=AXIS2_PLACEMENT_3D('',#151469,#119395,#119396) ;
#97612=AXIS2_PLACEMENT_3D('',#151470,#119397,#119398) ;
#97613=AXIS2_PLACEMENT_3D('',#151471,#119399,#119400) ;
#97614=AXIS2_PLACEMENT_3D('',#151472,#119401,#119402) ;
#97615=AXIS2_PLACEMENT_3D('',#151473,#119403,#119404) ;
#97616=AXIS2_PLACEMENT_3D('',#151474,#119405,#119406) ;
#97617=AXIS2_PLACEMENT_3D('',#151475,#119407,#119408) ;
#97618=AXIS2_PLACEMENT_3D('',#151476,#119409,#119410) ;
#97619=AXIS2_PLACEMENT_3D('',#151477,#119411,#119412) ;
#97620=AXIS2_PLACEMENT_3D('',#151478,#119413,#119414) ;
#97621=AXIS2_PLACEMENT_3D('',#151479,#119415,#119416) ;
#97622=AXIS2_PLACEMENT_3D('',#151480,#119417,#119418) ;
#97623=AXIS2_PLACEMENT_3D('',#151481,#119419,#119420) ;
#97624=AXIS2_PLACEMENT_3D('',#151482,#119421,#119422) ;
#97625=AXIS2_PLACEMENT_3D('',#151483,#119423,#119424) ;
#97626=AXIS2_PLACEMENT_3D('',#151484,#119425,#119426) ;
#97627=AXIS2_PLACEMENT_3D('',#151485,#119427,#119428) ;
#97628=AXIS2_PLACEMENT_3D('',#151486,#119429,#119430) ;
#97629=AXIS2_PLACEMENT_3D('',#151487,#119431,#119432) ;
#97630=AXIS2_PLACEMENT_3D('',#151488,#119433,#119434) ;
#97631=AXIS2_PLACEMENT_3D('',#151489,#119435,#119436) ;
#97632=AXIS2_PLACEMENT_3D('',#151490,#119437,#119438) ;
#97633=AXIS2_PLACEMENT_3D('',#151491,#119439,#119440) ;
#97634=AXIS2_PLACEMENT_3D('',#151492,#119441,#119442) ;
#97635=AXIS2_PLACEMENT_3D('',#151493,#119443,#119444) ;
#97636=AXIS2_PLACEMENT_3D('',#151494,#119445,#119446) ;
#97637=AXIS2_PLACEMENT_3D('',#151495,#119447,#119448) ;
#97638=AXIS2_PLACEMENT_3D('',#151496,#119449,#119450) ;
#97639=AXIS2_PLACEMENT_3D('',#151497,#119451,#119452) ;
#97640=AXIS2_PLACEMENT_3D('',#151498,#119453,#119454) ;
#97641=AXIS2_PLACEMENT_3D('',#151499,#119455,#119456) ;
#97642=AXIS2_PLACEMENT_3D('',#151500,#119457,#119458) ;
#97643=AXIS2_PLACEMENT_3D('',#151501,#119459,#119460) ;
#97644=AXIS2_PLACEMENT_3D('',#151502,#119461,#119462) ;
#97645=AXIS2_PLACEMENT_3D('',#151503,#119463,#119464) ;
#97646=AXIS2_PLACEMENT_3D('',#151504,#119465,#119466) ;
#97647=AXIS2_PLACEMENT_3D('',#151505,#119467,#119468) ;
#97648=AXIS2_PLACEMENT_3D('',#151506,#119469,#119470) ;
#97649=AXIS2_PLACEMENT_3D('',#151507,#119471,#119472) ;
#97650=AXIS2_PLACEMENT_3D('',#151508,#119473,#119474) ;
#97651=AXIS2_PLACEMENT_3D('',#151509,#119475,#119476) ;
#97652=AXIS2_PLACEMENT_3D('',#151510,#119477,#119478) ;
#97653=AXIS2_PLACEMENT_3D('',#151511,#119479,#119480) ;
#97654=AXIS2_PLACEMENT_3D('',#151512,#119481,#119482) ;
#97655=AXIS2_PLACEMENT_3D('',#151513,#119483,#119484) ;
#97656=AXIS2_PLACEMENT_3D('',#151514,#119485,#119486) ;
#97657=AXIS2_PLACEMENT_3D('',#151515,#119487,#119488) ;
#97658=AXIS2_PLACEMENT_3D('',#151516,#119489,#119490) ;
#97659=AXIS2_PLACEMENT_3D('',#151517,#119491,#119492) ;
#97660=AXIS2_PLACEMENT_3D('',#151518,#119493,#119494) ;
#97661=AXIS2_PLACEMENT_3D('',#151519,#119495,#119496) ;
#97662=AXIS2_PLACEMENT_3D('',#151520,#119497,#119498) ;
#97663=AXIS2_PLACEMENT_3D('',#151521,#119499,#119500) ;
#97664=AXIS2_PLACEMENT_3D('',#151522,#119501,#119502) ;
#97665=AXIS2_PLACEMENT_3D('',#151523,#119503,#119504) ;
#97666=AXIS2_PLACEMENT_3D('',#151524,#119505,#119506) ;
#97667=AXIS2_PLACEMENT_3D('',#151525,#119507,#119508) ;
#97668=AXIS2_PLACEMENT_3D('',#151526,#119509,#119510) ;
#97669=AXIS2_PLACEMENT_3D('',#151527,#119511,#119512) ;
#97670=AXIS2_PLACEMENT_3D('',#151528,#119513,#119514) ;
#97671=AXIS2_PLACEMENT_3D('',#151529,#119515,#119516) ;
#97672=AXIS2_PLACEMENT_3D('',#151530,#119517,#119518) ;
#97673=AXIS2_PLACEMENT_3D('',#151531,#119519,#119520) ;
#97674=AXIS2_PLACEMENT_3D('',#151532,#119521,#119522) ;
#97675=AXIS2_PLACEMENT_3D('',#151533,#119523,#119524) ;
#97676=AXIS2_PLACEMENT_3D('',#151534,#119525,#119526) ;
#97677=AXIS2_PLACEMENT_3D('',#151535,#119527,#119528) ;
#97678=AXIS2_PLACEMENT_3D('',#151536,#119529,#119530) ;
#97679=AXIS2_PLACEMENT_3D('',#151537,#119531,#119532) ;
#97680=AXIS2_PLACEMENT_3D('',#151538,#119533,#119534) ;
#97681=AXIS2_PLACEMENT_3D('',#151539,#119535,#119536) ;
#97682=AXIS2_PLACEMENT_3D('',#151540,#119537,#119538) ;
#97683=AXIS2_PLACEMENT_3D('',#151541,#119539,#119540) ;
#97684=AXIS2_PLACEMENT_3D('',#151542,#119541,#119542) ;
#97685=AXIS2_PLACEMENT_3D('',#151543,#119543,#119544) ;
#97686=AXIS2_PLACEMENT_3D('',#151544,#119545,#119546) ;
#97687=AXIS2_PLACEMENT_3D('',#151545,#119547,#119548) ;
#97688=AXIS2_PLACEMENT_3D('',#151546,#119549,#119550) ;
#97689=AXIS2_PLACEMENT_3D('',#151547,#119551,#119552) ;
#97690=AXIS2_PLACEMENT_3D('',#151548,#119553,#119554) ;
#97691=AXIS2_PLACEMENT_3D('',#151549,#119555,#119556) ;
#97692=AXIS2_PLACEMENT_3D('',#151550,#119557,#119558) ;
#97693=AXIS2_PLACEMENT_3D('',#151551,#119559,#119560) ;
#97694=AXIS2_PLACEMENT_3D('',#151552,#119561,#119562) ;
#97695=AXIS2_PLACEMENT_3D('',#151553,#119563,#119564) ;
#97696=AXIS2_PLACEMENT_3D('',#151554,#119565,#119566) ;
#97697=AXIS2_PLACEMENT_3D('',#151555,#119567,#119568) ;
#97698=AXIS2_PLACEMENT_3D('',#151556,#119569,#119570) ;
#97699=AXIS2_PLACEMENT_3D('',#151557,#119571,#119572) ;
#97700=AXIS2_PLACEMENT_3D('',#151558,#119573,#119574) ;
#97701=AXIS2_PLACEMENT_3D('',#151559,#119575,#119576) ;
#97702=AXIS2_PLACEMENT_3D('',#151560,#119577,#119578) ;
#97703=AXIS2_PLACEMENT_3D('',#151561,#119579,#119580) ;
#97704=AXIS2_PLACEMENT_3D('',#151562,#119581,#119582) ;
#97705=AXIS2_PLACEMENT_3D('',#151563,#119583,#119584) ;
#97706=AXIS2_PLACEMENT_3D('',#151564,#119585,#119586) ;
#97707=AXIS2_PLACEMENT_3D('',#151565,#119587,#119588) ;
#97708=AXIS2_PLACEMENT_3D('',#151566,#119589,#119590) ;
#97709=AXIS2_PLACEMENT_3D('',#151567,#119591,#119592) ;
#97710=AXIS2_PLACEMENT_3D('',#151568,#119593,#119594) ;
#97711=AXIS2_PLACEMENT_3D('',#151569,#119595,#119596) ;
#97712=AXIS2_PLACEMENT_3D('',#151570,#119597,#119598) ;
#97713=AXIS2_PLACEMENT_3D('',#151571,#119599,#119600) ;
#97714=AXIS2_PLACEMENT_3D('',#151572,#119601,#119602) ;
#97715=AXIS2_PLACEMENT_3D('',#151573,#119603,#119604) ;
#97716=AXIS2_PLACEMENT_3D('',#151574,#119605,#119606) ;
#97717=AXIS2_PLACEMENT_3D('',#151575,#119607,#119608) ;
#97718=AXIS2_PLACEMENT_3D('',#151576,#119609,#119610) ;
#97719=AXIS2_PLACEMENT_3D('',#151577,#119611,#119612) ;
#97720=AXIS2_PLACEMENT_3D('',#151578,#119613,#119614) ;
#97721=AXIS2_PLACEMENT_3D('',#151579,#119615,#119616) ;
#97722=AXIS2_PLACEMENT_3D('',#151580,#119617,#119618) ;
#97723=AXIS2_PLACEMENT_3D('',#151581,#119619,#119620) ;
#97724=AXIS2_PLACEMENT_3D('',#151582,#119621,#119622) ;
#97725=AXIS2_PLACEMENT_3D('',#151583,#119623,#119624) ;
#97726=AXIS2_PLACEMENT_3D('',#151584,#119625,#119626) ;
#97727=AXIS2_PLACEMENT_3D('',#151585,#119627,#119628) ;
#97728=AXIS2_PLACEMENT_3D('',#151586,#119629,#119630) ;
#97729=AXIS2_PLACEMENT_3D('',#151587,#119631,#119632) ;
#97730=AXIS2_PLACEMENT_3D('',#151588,#119633,#119634) ;
#97731=AXIS2_PLACEMENT_3D('',#151589,#119635,#119636) ;
#97732=AXIS2_PLACEMENT_3D('',#151590,#119637,#119638) ;
#97733=AXIS2_PLACEMENT_3D('',#151591,#119639,#119640) ;
#97734=AXIS2_PLACEMENT_3D('',#151592,#119641,#119642) ;
#97735=AXIS2_PLACEMENT_3D('',#151593,#119643,#119644) ;
#97736=AXIS2_PLACEMENT_3D('',#151594,#119645,#119646) ;
#97737=AXIS2_PLACEMENT_3D('',#151595,#119647,#119648) ;
#97738=AXIS2_PLACEMENT_3D('',#151596,#119649,#119650) ;
#97739=AXIS2_PLACEMENT_3D('',#151597,#119651,#119652) ;
#97740=AXIS2_PLACEMENT_3D('',#151598,#119653,#119654) ;
#97741=AXIS2_PLACEMENT_3D('',#151599,#119655,#119656) ;
#97742=AXIS2_PLACEMENT_3D('',#151600,#119657,#119658) ;
#97743=AXIS2_PLACEMENT_3D('',#151601,#119659,#119660) ;
#97744=AXIS2_PLACEMENT_3D('',#151602,#119661,#119662) ;
#97745=AXIS2_PLACEMENT_3D('',#151603,#119663,#119664) ;
#97746=AXIS2_PLACEMENT_3D('',#151604,#119665,#119666) ;
#97747=AXIS2_PLACEMENT_3D('',#151605,#119667,#119668) ;
#97748=AXIS2_PLACEMENT_3D('',#151606,#119669,#119670) ;
#97749=AXIS2_PLACEMENT_3D('',#151607,#119671,#119672) ;
#97750=AXIS2_PLACEMENT_3D('',#151608,#119673,#119674) ;
#97751=AXIS2_PLACEMENT_3D('',#151609,#119675,#119676) ;
#97752=AXIS2_PLACEMENT_3D('',#151610,#119677,#119678) ;
#97753=AXIS2_PLACEMENT_3D('',#151611,#119679,#119680) ;
#97754=AXIS2_PLACEMENT_3D('',#151612,#119681,#119682) ;
#97755=AXIS2_PLACEMENT_3D('',#151613,#119683,#119684) ;
#97756=AXIS2_PLACEMENT_3D('',#151614,#119685,#119686) ;
#97757=AXIS2_PLACEMENT_3D('',#151615,#119687,#119688) ;
#97758=AXIS2_PLACEMENT_3D('',#151616,#119689,#119690) ;
#97759=AXIS2_PLACEMENT_3D('',#151617,#119691,#119692) ;
#97760=AXIS2_PLACEMENT_3D('',#151618,#119693,#119694) ;
#97761=AXIS2_PLACEMENT_3D('',#151619,#119695,#119696) ;
#97762=AXIS2_PLACEMENT_3D('',#151620,#119697,#119698) ;
#97763=AXIS2_PLACEMENT_3D('',#151621,#119699,#119700) ;
#97764=AXIS2_PLACEMENT_3D('',#151622,#119701,#119702) ;
#97765=AXIS2_PLACEMENT_3D('',#151623,#119703,#119704) ;
#97766=AXIS2_PLACEMENT_3D('',#151624,#119705,#119706) ;
#97767=AXIS2_PLACEMENT_3D('',#151625,#119707,#119708) ;
#97768=AXIS2_PLACEMENT_3D('',#151626,#119709,#119710) ;
#97769=AXIS2_PLACEMENT_3D('',#151627,#119711,#119712) ;
#97770=AXIS2_PLACEMENT_3D('',#151628,#119713,#119714) ;
#97771=AXIS2_PLACEMENT_3D('',#151629,#119715,#119716) ;
#97772=AXIS2_PLACEMENT_3D('',#151630,#119717,#119718) ;
#97773=AXIS2_PLACEMENT_3D('',#151631,#119719,#119720) ;
#97774=AXIS2_PLACEMENT_3D('',#151632,#119721,#119722) ;
#97775=AXIS2_PLACEMENT_3D('',#151633,#119723,#119724) ;
#97776=AXIS2_PLACEMENT_3D('',#151634,#119725,#119726) ;
#97777=AXIS2_PLACEMENT_3D('',#151635,#119727,#119728) ;
#97778=AXIS2_PLACEMENT_3D('',#151636,#119729,#119730) ;
#97779=AXIS2_PLACEMENT_3D('',#151637,#119731,#119732) ;
#97780=AXIS2_PLACEMENT_3D('',#151638,#119733,#119734) ;
#97781=AXIS2_PLACEMENT_3D('',#151639,#119735,#119736) ;
#97782=AXIS2_PLACEMENT_3D('',#151640,#119737,#119738) ;
#97783=AXIS2_PLACEMENT_3D('',#151641,#119739,#119740) ;
#97784=AXIS2_PLACEMENT_3D('',#151642,#119741,#119742) ;
#97785=AXIS2_PLACEMENT_3D('',#151643,#119743,#119744) ;
#97786=AXIS2_PLACEMENT_3D('',#151644,#119745,#119746) ;
#97787=AXIS2_PLACEMENT_3D('',#151645,#119747,#119748) ;
#97788=AXIS2_PLACEMENT_3D('',#151646,#119749,#119750) ;
#97789=AXIS2_PLACEMENT_3D('',#151647,#119751,#119752) ;
#97790=AXIS2_PLACEMENT_3D('',#151648,#119753,#119754) ;
#97791=AXIS2_PLACEMENT_3D('',#151649,#119755,#119756) ;
#97792=AXIS2_PLACEMENT_3D('',#151650,#119757,#119758) ;
#97793=AXIS2_PLACEMENT_3D('',#151651,#119759,#119760) ;
#97794=AXIS2_PLACEMENT_3D('',#151652,#119761,#119762) ;
#97795=AXIS2_PLACEMENT_3D('',#151653,#119763,#119764) ;
#97796=AXIS2_PLACEMENT_3D('',#151654,#119765,#119766) ;
#97797=AXIS2_PLACEMENT_3D('',#151655,#119767,#119768) ;
#97798=AXIS2_PLACEMENT_3D('',#151656,#119769,#119770) ;
#97799=AXIS2_PLACEMENT_3D('',#151657,#119771,#119772) ;
#97800=AXIS2_PLACEMENT_3D('',#151658,#119773,#119774) ;
#97801=AXIS2_PLACEMENT_3D('',#151659,#119775,#119776) ;
#97802=AXIS2_PLACEMENT_3D('',#151660,#119777,#119778) ;
#97803=AXIS2_PLACEMENT_3D('',#151661,#119779,#119780) ;
#97804=AXIS2_PLACEMENT_3D('',#151662,#119781,#119782) ;
#97805=AXIS2_PLACEMENT_3D('',#151663,#119783,#119784) ;
#97806=AXIS2_PLACEMENT_3D('',#151664,#119785,#119786) ;
#97807=AXIS2_PLACEMENT_3D('',#151665,#119787,#119788) ;
#97808=AXIS2_PLACEMENT_3D('',#151666,#119789,#119790) ;
#97809=AXIS2_PLACEMENT_3D('',#151667,#119791,#119792) ;
#97810=AXIS2_PLACEMENT_3D('',#151668,#119793,#119794) ;
#97811=AXIS2_PLACEMENT_3D('',#151669,#119795,#119796) ;
#97812=AXIS2_PLACEMENT_3D('',#151670,#119797,#119798) ;
#97813=AXIS2_PLACEMENT_3D('',#151671,#119799,#119800) ;
#97814=AXIS2_PLACEMENT_3D('',#151672,#119801,#119802) ;
#97815=AXIS2_PLACEMENT_3D('',#151673,#119803,#119804) ;
#97816=AXIS2_PLACEMENT_3D('',#151674,#119805,#119806) ;
#97817=AXIS2_PLACEMENT_3D('',#151675,#119807,#119808) ;
#97818=AXIS2_PLACEMENT_3D('',#151676,#119809,#119810) ;
#97819=AXIS2_PLACEMENT_3D('',#151677,#119811,#119812) ;
#97820=AXIS2_PLACEMENT_3D('',#151678,#119813,#119814) ;
#97821=AXIS2_PLACEMENT_3D('',#151679,#119815,#119816) ;
#97822=AXIS2_PLACEMENT_3D('',#151680,#119817,#119818) ;
#97823=AXIS2_PLACEMENT_3D('',#151681,#119819,#119820) ;
#97824=AXIS2_PLACEMENT_3D('',#151682,#119821,#119822) ;
#97825=AXIS2_PLACEMENT_3D('',#151683,#119823,#119824) ;
#97826=AXIS2_PLACEMENT_3D('',#151684,#119825,#119826) ;
#97827=AXIS2_PLACEMENT_3D('',#151685,#119827,#119828) ;
#97828=AXIS2_PLACEMENT_3D('',#151686,#119829,#119830) ;
#97829=AXIS2_PLACEMENT_3D('',#151687,#119831,#119832) ;
#97830=AXIS2_PLACEMENT_3D('',#151688,#119833,#119834) ;
#97831=AXIS2_PLACEMENT_3D('',#151689,#119835,#119836) ;
#97832=AXIS2_PLACEMENT_3D('',#151690,#119837,#119838) ;
#97833=AXIS2_PLACEMENT_3D('',#151691,#119839,#119840) ;
#97834=AXIS2_PLACEMENT_3D('',#151692,#119841,#119842) ;
#97835=AXIS2_PLACEMENT_3D('',#151693,#119843,#119844) ;
#97836=AXIS2_PLACEMENT_3D('',#151694,#119845,#119846) ;
#97837=AXIS2_PLACEMENT_3D('',#151695,#119847,#119848) ;
#97838=AXIS2_PLACEMENT_3D('',#151696,#119849,#119850) ;
#97839=AXIS2_PLACEMENT_3D('',#151697,#119851,#119852) ;
#97840=AXIS2_PLACEMENT_3D('',#151698,#119853,#119854) ;
#97841=AXIS2_PLACEMENT_3D('',#151699,#119855,#119856) ;
#97842=AXIS2_PLACEMENT_3D('',#151700,#119857,#119858) ;
#97843=AXIS2_PLACEMENT_3D('',#151701,#119859,#119860) ;
#97844=AXIS2_PLACEMENT_3D('',#151702,#119861,#119862) ;
#97845=AXIS2_PLACEMENT_3D('',#151703,#119863,#119864) ;
#97846=AXIS2_PLACEMENT_3D('',#151704,#119865,#119866) ;
#97847=AXIS2_PLACEMENT_3D('',#151705,#119867,#119868) ;
#97848=AXIS2_PLACEMENT_3D('',#151706,#119869,#119870) ;
#97849=AXIS2_PLACEMENT_3D('',#151707,#119871,#119872) ;
#97850=AXIS2_PLACEMENT_3D('',#151708,#119873,#119874) ;
#97851=AXIS2_PLACEMENT_3D('',#151709,#119875,#119876) ;
#97852=AXIS2_PLACEMENT_3D('',#151710,#119877,#119878) ;
#97853=AXIS2_PLACEMENT_3D('',#151711,#119879,#119880) ;
#97854=AXIS2_PLACEMENT_3D('',#151712,#119881,#119882) ;
#97855=AXIS2_PLACEMENT_3D('',#151713,#119883,#119884) ;
#97856=AXIS2_PLACEMENT_3D('',#151714,#119885,#119886) ;
#97857=AXIS2_PLACEMENT_3D('',#151715,#119887,#119888) ;
#97858=AXIS2_PLACEMENT_3D('',#151716,#119889,#119890) ;
#97859=AXIS2_PLACEMENT_3D('',#151717,#119891,#119892) ;
#97860=AXIS2_PLACEMENT_3D('',#151718,#119893,#119894) ;
#97861=AXIS2_PLACEMENT_3D('',#151719,#119895,#119896) ;
#97862=AXIS2_PLACEMENT_3D('',#151720,#119897,#119898) ;
#97863=AXIS2_PLACEMENT_3D('',#151721,#119899,#119900) ;
#97864=AXIS2_PLACEMENT_3D('',#151722,#119901,#119902) ;
#97865=AXIS2_PLACEMENT_3D('',#151723,#119903,#119904) ;
#97866=AXIS2_PLACEMENT_3D('',#151724,#119905,#119906) ;
#97867=AXIS2_PLACEMENT_3D('',#151725,#119907,#119908) ;
#97868=AXIS2_PLACEMENT_3D('',#151726,#119909,#119910) ;
#97869=AXIS2_PLACEMENT_3D('',#151727,#119911,#119912) ;
#97870=AXIS2_PLACEMENT_3D('',#151728,#119913,#119914) ;
#97871=AXIS2_PLACEMENT_3D('',#151729,#119915,#119916) ;
#97872=AXIS2_PLACEMENT_3D('',#151730,#119917,#119918) ;
#97873=AXIS2_PLACEMENT_3D('',#151731,#119919,#119920) ;
#97874=AXIS2_PLACEMENT_3D('',#151732,#119921,#119922) ;
#97875=AXIS2_PLACEMENT_3D('',#151733,#119923,#119924) ;
#97876=AXIS2_PLACEMENT_3D('',#151734,#119925,#119926) ;
#97877=AXIS2_PLACEMENT_3D('',#151735,#119927,#119928) ;
#97878=AXIS2_PLACEMENT_3D('',#151736,#119929,#119930) ;
#97879=AXIS2_PLACEMENT_3D('',#151737,#119931,#119932) ;
#97880=AXIS2_PLACEMENT_3D('',#151738,#119933,#119934) ;
#97881=AXIS2_PLACEMENT_3D('',#151739,#119935,#119936) ;
#97882=AXIS2_PLACEMENT_3D('',#151740,#119937,#119938) ;
#97883=AXIS2_PLACEMENT_3D('',#151741,#119939,#119940) ;
#97884=AXIS2_PLACEMENT_3D('',#151742,#119941,#119942) ;
#97885=AXIS2_PLACEMENT_3D('',#151743,#119943,#119944) ;
#97886=AXIS2_PLACEMENT_3D('',#151744,#119945,#119946) ;
#97887=AXIS2_PLACEMENT_3D('',#151745,#119947,#119948) ;
#97888=AXIS2_PLACEMENT_3D('',#151746,#119949,#119950) ;
#97889=AXIS2_PLACEMENT_3D('',#151747,#119951,#119952) ;
#97890=AXIS2_PLACEMENT_3D('',#151748,#119953,#119954) ;
#97891=AXIS2_PLACEMENT_3D('',#151749,#119955,#119956) ;
#97892=AXIS2_PLACEMENT_3D('',#151750,#119957,#119958) ;
#97893=AXIS2_PLACEMENT_3D('',#151751,#119959,#119960) ;
#97894=AXIS2_PLACEMENT_3D('',#151752,#119961,#119962) ;
#97895=AXIS2_PLACEMENT_3D('',#151753,#119963,#119964) ;
#97896=AXIS2_PLACEMENT_3D('',#151754,#119965,#119966) ;
#97897=AXIS2_PLACEMENT_3D('',#151755,#119967,#119968) ;
#97898=AXIS2_PLACEMENT_3D('',#151756,#119969,#119970) ;
#97899=AXIS2_PLACEMENT_3D('',#151757,#119971,#119972) ;
#97900=AXIS2_PLACEMENT_3D('',#151758,#119973,#119974) ;
#97901=AXIS2_PLACEMENT_3D('',#151759,#119975,#119976) ;
#97902=AXIS2_PLACEMENT_3D('',#151760,#119977,#119978) ;
#97903=AXIS2_PLACEMENT_3D('',#151761,#119979,#119980) ;
#97904=AXIS2_PLACEMENT_3D('',#151762,#119981,#119982) ;
#97905=AXIS2_PLACEMENT_3D('',#151763,#119983,#119984) ;
#97906=AXIS2_PLACEMENT_3D('',#151764,#119985,#119986) ;
#97907=AXIS2_PLACEMENT_3D('',#151765,#119987,#119988) ;
#97908=AXIS2_PLACEMENT_3D('',#151766,#119989,#119990) ;
#97909=AXIS2_PLACEMENT_3D('',#151767,#119991,#119992) ;
#97910=AXIS2_PLACEMENT_3D('',#151768,#119993,#119994) ;
#97911=AXIS2_PLACEMENT_3D('',#151769,#119995,#119996) ;
#97912=AXIS2_PLACEMENT_3D('',#151770,#119997,#119998) ;
#97913=AXIS2_PLACEMENT_3D('',#151771,#119999,#120000) ;
#97914=AXIS2_PLACEMENT_3D('',#151772,#120001,#120002) ;
#97915=AXIS2_PLACEMENT_3D('',#151773,#120003,#120004) ;
#97916=AXIS2_PLACEMENT_3D('',#151774,#120005,#120006) ;
#97917=AXIS2_PLACEMENT_3D('',#151775,#120007,#120008) ;
#97918=AXIS2_PLACEMENT_3D('',#151776,#120009,#120010) ;
#97919=AXIS2_PLACEMENT_3D('',#151777,#120011,#120012) ;
#97920=AXIS2_PLACEMENT_3D('',#151778,#120013,#120014) ;
#97921=AXIS2_PLACEMENT_3D('',#151779,#120015,#120016) ;
#97922=AXIS2_PLACEMENT_3D('',#151780,#120017,#120018) ;
#97923=AXIS2_PLACEMENT_3D('',#151781,#120019,#120020) ;
#97924=AXIS2_PLACEMENT_3D('',#151782,#120021,#120022) ;
#97925=AXIS2_PLACEMENT_3D('',#151783,#120023,#120024) ;
#97926=AXIS2_PLACEMENT_3D('',#151784,#120025,#120026) ;
#97927=AXIS2_PLACEMENT_3D('',#151785,#120027,#120028) ;
#97928=AXIS2_PLACEMENT_3D('',#151786,#120029,#120030) ;
#97929=AXIS2_PLACEMENT_3D('',#151787,#120031,#120032) ;
#97930=AXIS2_PLACEMENT_3D('',#151788,#120033,#120034) ;
#97931=AXIS2_PLACEMENT_3D('',#151789,#120035,#120036) ;
#97932=AXIS2_PLACEMENT_3D('',#151790,#120037,#120038) ;
#97933=AXIS2_PLACEMENT_3D('',#151791,#120039,#120040) ;
#97934=AXIS2_PLACEMENT_3D('',#151792,#120041,#120042) ;
#97935=AXIS2_PLACEMENT_3D('',#151793,#120043,#120044) ;
#97936=AXIS2_PLACEMENT_3D('',#151794,#120045,#120046) ;
#97937=AXIS2_PLACEMENT_3D('',#151795,#120047,#120048) ;
#97938=AXIS2_PLACEMENT_3D('',#151796,#120049,#120050) ;
#97939=AXIS2_PLACEMENT_3D('',#151797,#120051,#120052) ;
#97940=AXIS2_PLACEMENT_3D('',#151798,#120053,#120054) ;
#97941=AXIS2_PLACEMENT_3D('',#151799,#120055,#120056) ;
#97942=AXIS2_PLACEMENT_3D('',#151800,#120057,#120058) ;
#97943=AXIS2_PLACEMENT_3D('',#151801,#120059,#120060) ;
#97944=AXIS2_PLACEMENT_3D('',#151802,#120061,#120062) ;
#97945=AXIS2_PLACEMENT_3D('',#151803,#120063,#120064) ;
#97946=AXIS2_PLACEMENT_3D('',#151804,#120065,#120066) ;
#97947=AXIS2_PLACEMENT_3D('',#151805,#120067,#120068) ;
#97948=AXIS2_PLACEMENT_3D('',#151806,#120069,#120070) ;
#97949=AXIS2_PLACEMENT_3D('',#151807,#120071,#120072) ;
#97950=AXIS2_PLACEMENT_3D('',#151808,#120073,#120074) ;
#97951=AXIS2_PLACEMENT_3D('',#151809,#120075,#120076) ;
#97952=AXIS2_PLACEMENT_3D('',#151810,#120077,#120078) ;
#97953=AXIS2_PLACEMENT_3D('',#151811,#120079,#120080) ;
#97954=AXIS2_PLACEMENT_3D('',#151812,#120081,#120082) ;
#97955=AXIS2_PLACEMENT_3D('',#151813,#120083,#120084) ;
#97956=AXIS2_PLACEMENT_3D('',#151814,#120085,#120086) ;
#97957=AXIS2_PLACEMENT_3D('',#151815,#120087,#120088) ;
#97958=AXIS2_PLACEMENT_3D('',#151816,#120089,#120090) ;
#97959=AXIS2_PLACEMENT_3D('',#151817,#120091,#120092) ;
#97960=AXIS2_PLACEMENT_3D('',#151818,#120093,#120094) ;
#97961=AXIS2_PLACEMENT_3D('',#151819,#120095,#120096) ;
#97962=AXIS2_PLACEMENT_3D('',#151820,#120097,#120098) ;
#97963=AXIS2_PLACEMENT_3D('',#151821,#120099,#120100) ;
#97964=AXIS2_PLACEMENT_3D('',#151822,#120101,#120102) ;
#97965=AXIS2_PLACEMENT_3D('',#151823,#120103,#120104) ;
#97966=AXIS2_PLACEMENT_3D('',#151824,#120105,#120106) ;
#97967=AXIS2_PLACEMENT_3D('',#151825,#120107,#120108) ;
#97968=AXIS2_PLACEMENT_3D('',#151826,#120109,#120110) ;
#97969=AXIS2_PLACEMENT_3D('',#151827,#120111,#120112) ;
#97970=AXIS2_PLACEMENT_3D('',#151828,#120113,#120114) ;
#97971=AXIS2_PLACEMENT_3D('',#151829,#120115,#120116) ;
#97972=AXIS2_PLACEMENT_3D('',#151830,#120117,#120118) ;
#97973=AXIS2_PLACEMENT_3D('',#151831,#120119,#120120) ;
#97974=AXIS2_PLACEMENT_3D('',#151832,#120121,#120122) ;
#97975=AXIS2_PLACEMENT_3D('',#151833,#120123,#120124) ;
#97976=AXIS2_PLACEMENT_3D('',#151834,#120125,#120126) ;
#97977=AXIS2_PLACEMENT_3D('',#151835,#120127,#120128) ;
#97978=AXIS2_PLACEMENT_3D('',#151836,#120129,#120130) ;
#97979=AXIS2_PLACEMENT_3D('',#151837,#120131,#120132) ;
#97980=AXIS2_PLACEMENT_3D('',#151838,#120133,#120134) ;
#97981=AXIS2_PLACEMENT_3D('',#151839,#120135,#120136) ;
#97982=AXIS2_PLACEMENT_3D('',#151840,#120137,#120138) ;
#97983=AXIS2_PLACEMENT_3D('',#151841,#120139,#120140) ;
#97984=AXIS2_PLACEMENT_3D('',#151842,#120141,#120142) ;
#97985=AXIS2_PLACEMENT_3D('',#151843,#120143,#120144) ;
#97986=AXIS2_PLACEMENT_3D('',#151844,#120145,#120146) ;
#97987=AXIS2_PLACEMENT_3D('',#151845,#120147,#120148) ;
#97988=AXIS2_PLACEMENT_3D('',#151846,#120149,#120150) ;
#97989=AXIS2_PLACEMENT_3D('',#151847,#120151,#120152) ;
#97990=AXIS2_PLACEMENT_3D('',#151848,#120153,#120154) ;
#97991=AXIS2_PLACEMENT_3D('',#151849,#120155,#120156) ;
#97992=AXIS2_PLACEMENT_3D('',#151850,#120157,#120158) ;
#97993=AXIS2_PLACEMENT_3D('',#151851,#120159,#120160) ;
#97994=AXIS2_PLACEMENT_3D('',#151852,#120161,#120162) ;
#97995=AXIS2_PLACEMENT_3D('',#151853,#120163,#120164) ;
#97996=AXIS2_PLACEMENT_3D('',#151854,#120165,#120166) ;
#97997=AXIS2_PLACEMENT_3D('',#151855,#120167,#120168) ;
#97998=AXIS2_PLACEMENT_3D('',#151856,#120169,#120170) ;
#97999=AXIS2_PLACEMENT_3D('',#151857,#120171,#120172) ;
#98000=AXIS2_PLACEMENT_3D('',#151858,#120173,#120174) ;
#98001=AXIS2_PLACEMENT_3D('',#151859,#120175,#120176) ;
#98002=AXIS2_PLACEMENT_3D('',#151860,#120177,#120178) ;
#98003=AXIS2_PLACEMENT_3D('',#151861,#120179,#120180) ;
#98004=AXIS2_PLACEMENT_3D('',#151862,#120181,#120182) ;
#98005=AXIS2_PLACEMENT_3D('',#151863,#120183,#120184) ;
#98006=AXIS2_PLACEMENT_3D('',#151864,#120185,#120186) ;
#98007=AXIS2_PLACEMENT_3D('',#151865,#120187,#120188) ;
#98008=AXIS2_PLACEMENT_3D('',#151866,#120189,#120190) ;
#98009=AXIS2_PLACEMENT_3D('',#151867,#120191,#120192) ;
#98010=AXIS2_PLACEMENT_3D('',#151868,#120193,#120194) ;
#98011=AXIS2_PLACEMENT_3D('',#151869,#120195,#120196) ;
#98012=AXIS2_PLACEMENT_3D('',#151870,#120197,#120198) ;
#98013=AXIS2_PLACEMENT_3D('',#151871,#120199,#120200) ;
#98014=AXIS2_PLACEMENT_3D('',#151872,#120201,#120202) ;
#98015=AXIS2_PLACEMENT_3D('',#151873,#120203,#120204) ;
#98016=AXIS2_PLACEMENT_3D('',#151874,#120205,#120206) ;
#98017=AXIS2_PLACEMENT_3D('',#151875,#120207,#120208) ;
#98018=AXIS2_PLACEMENT_3D('',#151876,#120209,#120210) ;
#98019=AXIS2_PLACEMENT_3D('',#151877,#120211,#120212) ;
#98020=AXIS2_PLACEMENT_3D('',#151878,#120213,#120214) ;
#98021=AXIS2_PLACEMENT_3D('',#151879,#120215,#120216) ;
#98022=AXIS2_PLACEMENT_3D('',#151880,#120217,#120218) ;
#98023=AXIS2_PLACEMENT_3D('',#151881,#120219,#120220) ;
#98024=AXIS2_PLACEMENT_3D('',#151882,#120221,#120222) ;
#98025=AXIS2_PLACEMENT_3D('',#151883,#120223,#120224) ;
#98026=AXIS2_PLACEMENT_3D('',#151884,#120225,#120226) ;
#98027=AXIS2_PLACEMENT_3D('',#151885,#120227,#120228) ;
#98028=AXIS2_PLACEMENT_3D('',#151886,#120229,#120230) ;
#98029=AXIS2_PLACEMENT_3D('',#151887,#120231,#120232) ;
#98030=AXIS2_PLACEMENT_3D('',#151888,#120233,#120234) ;
#98031=AXIS2_PLACEMENT_3D('',#151889,#120235,#120236) ;
#98032=AXIS2_PLACEMENT_3D('',#151890,#120237,#120238) ;
#98033=AXIS2_PLACEMENT_3D('',#151891,#120239,#120240) ;
#98034=AXIS2_PLACEMENT_3D('',#151892,#120241,#120242) ;
#98035=AXIS2_PLACEMENT_3D('',#151893,#120243,#120244) ;
#98036=AXIS2_PLACEMENT_3D('',#151894,#120245,#120246) ;
#98037=AXIS2_PLACEMENT_3D('',#151895,#120247,#120248) ;
#98038=AXIS2_PLACEMENT_3D('',#151896,#120249,#120250) ;
#98039=AXIS2_PLACEMENT_3D('',#151897,#120251,#120252) ;
#98040=AXIS2_PLACEMENT_3D('',#151898,#120253,#120254) ;
#98041=AXIS2_PLACEMENT_3D('',#151899,#120255,#120256) ;
#98042=AXIS2_PLACEMENT_3D('',#151900,#120257,#120258) ;
#98043=AXIS2_PLACEMENT_3D('',#151901,#120259,#120260) ;
#98044=AXIS2_PLACEMENT_3D('',#151902,#120261,#120262) ;
#98045=AXIS2_PLACEMENT_3D('',#151903,#120263,#120264) ;
#98046=AXIS2_PLACEMENT_3D('',#151904,#120265,#120266) ;
#98047=AXIS2_PLACEMENT_3D('',#151905,#120267,#120268) ;
#98048=AXIS2_PLACEMENT_3D('',#151906,#120269,#120270) ;
#98049=AXIS2_PLACEMENT_3D('',#151907,#120271,#120272) ;
#98050=AXIS2_PLACEMENT_3D('',#151908,#120273,#120274) ;
#98051=AXIS2_PLACEMENT_3D('',#151909,#120275,#120276) ;
#98052=AXIS2_PLACEMENT_3D('',#151910,#120277,#120278) ;
#98053=AXIS2_PLACEMENT_3D('',#151911,#120279,#120280) ;
#98054=AXIS2_PLACEMENT_3D('',#151912,#120281,#120282) ;
#98055=AXIS2_PLACEMENT_3D('',#151913,#120283,#120284) ;
#98056=AXIS2_PLACEMENT_3D('',#151914,#120285,#120286) ;
#98057=AXIS2_PLACEMENT_3D('',#151915,#120287,#120288) ;
#98058=AXIS2_PLACEMENT_3D('',#151916,#120289,#120290) ;
#98059=AXIS2_PLACEMENT_3D('',#151917,#120291,#120292) ;
#98060=AXIS2_PLACEMENT_3D('',#151918,#120293,#120294) ;
#98061=AXIS2_PLACEMENT_3D('',#151919,#120295,#120296) ;
#98062=AXIS2_PLACEMENT_3D('',#151920,#120297,#120298) ;
#98063=AXIS2_PLACEMENT_3D('',#151921,#120299,#120300) ;
#98064=AXIS2_PLACEMENT_3D('',#151922,#120301,#120302) ;
#98065=AXIS2_PLACEMENT_3D('',#151923,#120303,#120304) ;
#98066=AXIS2_PLACEMENT_3D('',#151924,#120305,#120306) ;
#98067=AXIS2_PLACEMENT_3D('',#151925,#120307,#120308) ;
#98068=AXIS2_PLACEMENT_3D('',#151926,#120309,#120310) ;
#98069=AXIS2_PLACEMENT_3D('',#151927,#120311,#120312) ;
#98070=AXIS2_PLACEMENT_3D('',#151928,#120313,#120314) ;
#98071=AXIS2_PLACEMENT_3D('',#151929,#120315,#120316) ;
#98072=AXIS2_PLACEMENT_3D('',#151930,#120317,#120318) ;
#98073=AXIS2_PLACEMENT_3D('',#151931,#120319,#120320) ;
#98074=AXIS2_PLACEMENT_3D('',#151932,#120321,#120322) ;
#98075=AXIS2_PLACEMENT_3D('',#151933,#120323,#120324) ;
#98076=AXIS2_PLACEMENT_3D('',#151934,#120325,#120326) ;
#98077=AXIS2_PLACEMENT_3D('',#151935,#120327,#120328) ;
#98078=AXIS2_PLACEMENT_3D('',#151936,#120329,#120330) ;
#98079=AXIS2_PLACEMENT_3D('',#151937,#120331,#120332) ;
#98080=AXIS2_PLACEMENT_3D('',#151938,#120333,#120334) ;
#98081=AXIS2_PLACEMENT_3D('',#151939,#120335,#120336) ;
#98082=AXIS2_PLACEMENT_3D('',#151940,#120337,#120338) ;
#98083=AXIS2_PLACEMENT_3D('',#151941,#120339,#120340) ;
#98084=AXIS2_PLACEMENT_3D('',#151942,#120341,#120342) ;
#98085=AXIS2_PLACEMENT_3D('',#151943,#120343,#120344) ;
#98086=AXIS2_PLACEMENT_3D('',#151944,#120345,#120346) ;
#98087=AXIS2_PLACEMENT_3D('',#151945,#120347,#120348) ;
#98088=AXIS2_PLACEMENT_3D('',#151946,#120349,#120350) ;
#98089=AXIS2_PLACEMENT_3D('',#151947,#120351,#120352) ;
#98090=AXIS2_PLACEMENT_3D('',#151948,#120353,#120354) ;
#98091=AXIS2_PLACEMENT_3D('',#151949,#120355,#120356) ;
#98092=AXIS2_PLACEMENT_3D('',#151950,#120357,#120358) ;
#98093=AXIS2_PLACEMENT_3D('',#151951,#120359,#120360) ;
#98094=AXIS2_PLACEMENT_3D('',#151952,#120361,#120362) ;
#98095=AXIS2_PLACEMENT_3D('',#151953,#120363,#120364) ;
#98096=AXIS2_PLACEMENT_3D('',#151954,#120365,#120366) ;
#98097=AXIS2_PLACEMENT_3D('',#151955,#120367,#120368) ;
#98098=AXIS2_PLACEMENT_3D('',#151956,#120369,#120370) ;
#98099=AXIS2_PLACEMENT_3D('',#151957,#120371,#120372) ;
#98100=AXIS2_PLACEMENT_3D('',#151958,#120373,#120374) ;
#98101=AXIS2_PLACEMENT_3D('',#151959,#120375,#120376) ;
#98102=AXIS2_PLACEMENT_3D('',#151960,#120377,#120378) ;
#98103=AXIS2_PLACEMENT_3D('',#151961,#120379,#120380) ;
#98104=AXIS2_PLACEMENT_3D('',#151962,#120381,#120382) ;
#98105=AXIS2_PLACEMENT_3D('',#151963,#120383,#120384) ;
#98106=AXIS2_PLACEMENT_3D('',#151964,#120385,#120386) ;
#98107=AXIS2_PLACEMENT_3D('',#151965,#120387,#120388) ;
#98108=AXIS2_PLACEMENT_3D('',#151966,#120389,#120390) ;
#98109=AXIS2_PLACEMENT_3D('',#151967,#120391,#120392) ;
#98110=AXIS2_PLACEMENT_3D('',#151968,#120393,#120394) ;
#98111=AXIS2_PLACEMENT_3D('',#151969,#120395,#120396) ;
#98112=AXIS2_PLACEMENT_3D('',#151970,#120397,#120398) ;
#98113=AXIS2_PLACEMENT_3D('',#151971,#120399,#120400) ;
#98114=AXIS2_PLACEMENT_3D('',#151972,#120401,#120402) ;
#98115=AXIS2_PLACEMENT_3D('',#151973,#120403,#120404) ;
#98116=AXIS2_PLACEMENT_3D('',#151974,#120405,#120406) ;
#98117=AXIS2_PLACEMENT_3D('',#151975,#120407,#120408) ;
#98118=AXIS2_PLACEMENT_3D('',#151976,#120409,#120410) ;
#98119=AXIS2_PLACEMENT_3D('',#151977,#120411,#120412) ;
#98120=AXIS2_PLACEMENT_3D('',#151978,#120413,#120414) ;
#98121=AXIS2_PLACEMENT_3D('',#151979,#120415,#120416) ;
#98122=AXIS2_PLACEMENT_3D('',#151980,#120417,#120418) ;
#98123=AXIS2_PLACEMENT_3D('',#151981,#120419,#120420) ;
#98124=AXIS2_PLACEMENT_3D('',#151982,#120421,#120422) ;
#98125=AXIS2_PLACEMENT_3D('',#151983,#120423,#120424) ;
#98126=AXIS2_PLACEMENT_3D('',#151984,#120425,#120426) ;
#98127=AXIS2_PLACEMENT_3D('',#151985,#120427,#120428) ;
#98128=AXIS2_PLACEMENT_3D('',#151986,#120429,#120430) ;
#98129=AXIS2_PLACEMENT_3D('',#151987,#120431,#120432) ;
#98130=AXIS2_PLACEMENT_3D('',#151988,#120433,#120434) ;
#98131=AXIS2_PLACEMENT_3D('',#151989,#120435,#120436) ;
#98132=AXIS2_PLACEMENT_3D('',#151990,#120437,#120438) ;
#98133=AXIS2_PLACEMENT_3D('',#151991,#120439,#120440) ;
#98134=AXIS2_PLACEMENT_3D('',#151992,#120441,#120442) ;
#98135=AXIS2_PLACEMENT_3D('',#151993,#120443,#120444) ;
#98136=AXIS2_PLACEMENT_3D('',#151994,#120445,#120446) ;
#98137=AXIS2_PLACEMENT_3D('',#151995,#120447,#120448) ;
#98138=AXIS2_PLACEMENT_3D('',#151996,#120449,#120450) ;
#98139=AXIS2_PLACEMENT_3D('',#151997,#120451,#120452) ;
#98140=AXIS2_PLACEMENT_3D('',#151998,#120453,#120454) ;
#98141=AXIS2_PLACEMENT_3D('',#151999,#120455,#120456) ;
#98142=AXIS2_PLACEMENT_3D('',#152000,#120457,#120458) ;
#98143=AXIS2_PLACEMENT_3D('',#152001,#120459,#120460) ;
#98144=AXIS2_PLACEMENT_3D('',#152002,#120461,#120462) ;
#98145=AXIS2_PLACEMENT_3D('',#152003,#120463,#120464) ;
#98146=AXIS2_PLACEMENT_3D('',#152004,#120465,#120466) ;
#98147=AXIS2_PLACEMENT_3D('',#152005,#120467,#120468) ;
#98148=AXIS2_PLACEMENT_3D('',#152006,#120469,#120470) ;
#98149=AXIS2_PLACEMENT_3D('',#152007,#120471,#120472) ;
#98150=AXIS2_PLACEMENT_3D('',#152008,#120473,#120474) ;
#108731=DIRECTION('axis',(0.,0.,1.)) ;
#108732=DIRECTION('refdir',(1.,0.,0.)) ;
#108733=DIRECTION('center_axis',(1.,0.,0.)) ;
#108734=DIRECTION('ref_axis',(0.,0.,-1.)) ;
#108735=DIRECTION('center_axis',(1.,0.,0.)) ;
#108736=DIRECTION('ref_axis',(0.,0.,-1.)) ;
#108737=DIRECTION('center_axis',(0.,-1.,-1.22464679914735E-16)) ;
#108738=DIRECTION('ref_axis',(0.,-1.22464679914735E-16,1.)) ;
#108739=DIRECTION('center_axis',(-1.,0.,0.)) ;
#108740=DIRECTION('ref_axis',(0.,0.,-1.)) ;
#108741=DIRECTION('center_axis',(-1.,0.,0.)) ;
#108742=DIRECTION('ref_axis',(0.,0.,-1.)) ;
#108743=DIRECTION('center_axis',(-1.,0.,0.)) ;
#108744=DIRECTION('ref_axis',(0.,0.,1.)) ;
#108745=DIRECTION('center_axis',(-1.,0.,0.)) ;
#108746=DIRECTION('ref_axis',(0.,0.,1.)) ;
#108747=DIRECTION('center_axis',(0.,1.,-1.22464679914735E-16)) ;
#108748=DIRECTION('ref_axis',(0.,-1.22464679914735E-16,-1.)) ;
#108749=DIRECTION('center_axis',(1.,0.,0.)) ;
#108750=DIRECTION('ref_axis',(0.,0.,1.)) ;
#108751=DIRECTION('center_axis',(0.,1.,0.)) ;
#108752=DIRECTION('ref_axis',(0.,0.,1.)) ;
#108753=DIRECTION('center_axis',(-1.,0.,0.)) ;
#108754=DIRECTION('ref_axis',(0.,0.,-1.)) ;
#108755=DIRECTION('center_axis',(0.,0.707106781186532,0.707106781186563)) ;
#108756=DIRECTION('ref_axis',(0.,-0.707106781186563,0.707106781186532)) ;
#108757=DIRECTION('center_axis',(0.,0.,-1.)) ;
#108758=DIRECTION('ref_axis',(-1.,0.,0.)) ;
#108759=DIRECTION('center_axis',(2.16840434497101E-16,-1.,1.30104260698261E-16)) ;
#108760=DIRECTION('ref_axis',(1.,2.16840434497101E-16,-1.09476442525376E-47)) ;
#108761=DIRECTION('center_axis',(-2.25262403289994E-12,-0.707106781186411,
-0.707106781186684)) ;
#108762=DIRECTION('ref_axis',(2.77642807980434E-11,0.707106781186684,-0.707106781186411)) ;
#108763=DIRECTION('center_axis',(-5.42101086242752E-16,1.,0.)) ;
#108764=DIRECTION('ref_axis',(1.,5.42101086242752E-16,0.)) ;
#108765=DIRECTION('',(-2.16840434497101E-16,1.,-1.30104260698261E-16)) ;
#108766=DIRECTION('center_axis',(0.,1.,0.)) ;
#108767=DIRECTION('ref_axis',(0.,0.,1.)) ;
#108768=DIRECTION('',(2.16840434497101E-16,-1.,1.30104260698261E-16)) ;
#108769=DIRECTION('',(2.16840434497101E-16,-1.,1.30104260698261E-16)) ;
#108770=DIRECTION('center_axis',(1.,0.,0.)) ;
#108771=DIRECTION('ref_axis',(0.,0.,-1.)) ;
#108772=DIRECTION('center_axis',(1.,0.,0.)) ;
#108773=DIRECTION('ref_axis',(0.,0.,-1.)) ;
#108774=DIRECTION('center_axis',(0.,-1.,-1.22464679914735E-16)) ;
#108775=DIRECTION('ref_axis',(0.,-1.22464679914735E-16,1.)) ;
#108776=DIRECTION('center_axis',(-1.,0.,0.)) ;
#108777=DIRECTION('ref_axis',(0.,0.,-1.)) ;
#108778=DIRECTION('center_axis',(-1.,0.,0.)) ;
#108779=DIRECTION('ref_axis',(0.,0.,-1.)) ;
#108780=DIRECTION('center_axis',(-1.,0.,0.)) ;
#108781=DIRECTION('ref_axis',(0.,0.,1.)) ;
#108782=DIRECTION('center_axis',(-1.,0.,0.)) ;
#108783=DIRECTION('ref_axis',(0.,0.,1.)) ;
#108784=DIRECTION('center_axis',(0.,1.,-1.22464679914735E-16)) ;
#108785=DIRECTION('ref_axis',(0.,-1.22464679914735E-16,-1.)) ;
#108786=DIRECTION('center_axis',(1.,0.,0.)) ;
#108787=DIRECTION('ref_axis',(0.,0.,1.)) ;
#108788=DIRECTION('center_axis',(0.,1.,0.)) ;
#108789=DIRECTION('ref_axis',(0.,0.,1.)) ;
#108790=DIRECTION('center_axis',(-1.,0.,0.)) ;
#108791=DIRECTION('ref_axis',(0.,0.,-1.)) ;
#108792=DIRECTION('center_axis',(0.,0.707106781186558,0.707106781186537)) ;
#108793=DIRECTION('ref_axis',(0.,-0.707106781186537,0.707106781186558)) ;
#108794=DIRECTION('center_axis',(0.,0.,-1.)) ;
#108795=DIRECTION('ref_axis',(-1.,0.,0.)) ;
#108796=DIRECTION('center_axis',(2.16840434497101E-16,-1.,1.30104260698261E-16)) ;
#108797=DIRECTION('ref_axis',(1.,2.16840434497101E-16,-1.09476442525376E-47)) ;
#108798=DIRECTION('center_axis',(-2.85488809725132E-13,-0.707106781186525,
-0.70710678118657)) ;
#108799=DIRECTION('ref_axis',(7.82804041694617E-11,0.70710678118657,-0.707106781186525)) ;
#108800=DIRECTION('center_axis',(-5.42101086242752E-16,1.,0.)) ;
#108801=DIRECTION('ref_axis',(1.,5.42101086242752E-16,0.)) ;
#108802=DIRECTION('',(-2.16840434497101E-16,1.,-1.30104260698261E-16)) ;
#108803=DIRECTION('center_axis',(0.,1.,0.)) ;
#108804=DIRECTION('ref_axis',(0.,0.,1.)) ;
#108805=DIRECTION('',(2.16840434497101E-16,-1.,1.30104260698261E-16)) ;
#108806=DIRECTION('',(2.16840434497101E-16,-1.,1.30104260698261E-16)) ;
#108807=DIRECTION('center_axis',(1.,0.,0.)) ;
#108808=DIRECTION('ref_axis',(0.,0.,-1.)) ;
#108809=DIRECTION('center_axis',(1.,0.,0.)) ;
#108810=DIRECTION('ref_axis',(0.,0.,-1.)) ;
#108811=DIRECTION('center_axis',(0.,-1.,-1.22464679914735E-16)) ;
#108812=DIRECTION('ref_axis',(0.,-1.22464679914735E-16,1.)) ;
#108813=DIRECTION('center_axis',(-1.,0.,0.)) ;
#108814=DIRECTION('ref_axis',(0.,0.,-1.)) ;
#108815=DIRECTION('center_axis',(-1.,0.,0.)) ;
#108816=DIRECTION('ref_axis',(0.,0.,-1.)) ;
#108817=DIRECTION('center_axis',(-1.,0.,0.)) ;
#108818=DIRECTION('ref_axis',(0.,0.,1.)) ;
#108819=DIRECTION('center_axis',(-1.,0.,0.)) ;
#108820=DIRECTION('ref_axis',(0.,0.,1.)) ;
#108821=DIRECTION('center_axis',(0.,1.,-1.22464679914735E-16)) ;
#108822=DIRECTION('ref_axis',(0.,-1.22464679914735E-16,-1.)) ;
#108823=DIRECTION('center_axis',(1.,0.,0.)) ;
#108824=DIRECTION('ref_axis',(0.,0.,1.)) ;
#108825=DIRECTION('center_axis',(0.,1.,0.)) ;
#108826=DIRECTION('ref_axis',(0.,0.,1.)) ;
#108827=DIRECTION('center_axis',(-1.,0.,0.)) ;
#108828=DIRECTION('ref_axis',(0.,0.,-1.)) ;
#108829=DIRECTION('center_axis',(0.,0.707106781186558,0.707106781186537)) ;
#108830=DIRECTION('ref_axis',(0.,-0.707106781186537,0.707106781186558)) ;
#108831=DIRECTION('center_axis',(0.,0.,-1.)) ;
#108832=DIRECTION('ref_axis',(-1.,0.,0.)) ;
#108833=DIRECTION('center_axis',(2.16840434497101E-16,-1.,1.30104260698261E-16)) ;
#108834=DIRECTION('ref_axis',(1.,2.16840434497101E-16,-1.09476442525376E-47)) ;
#108835=DIRECTION('center_axis',(-4.61475062295438E-13,-0.707106781186512,
-0.707106781186583)) ;
#108836=DIRECTION('ref_axis',(8.02352901261504E-11,0.707106781186583,-0.707106781186512)) ;
#108837=DIRECTION('center_axis',(-5.42101086242752E-16,1.,0.)) ;
#108838=DIRECTION('ref_axis',(1.,5.42101086242752E-16,0.)) ;
#108839=DIRECTION('',(-2.16840434497101E-16,1.,-1.30104260698261E-16)) ;
#108840=DIRECTION('center_axis',(0.,1.,0.)) ;
#108841=DIRECTION('ref_axis',(0.,0.,1.)) ;
#108842=DIRECTION('',(2.16840434497101E-16,-1.,1.30104260698261E-16)) ;
#108843=DIRECTION('',(2.16840434497101E-16,-1.,1.30104260698261E-16)) ;
#108844=DIRECTION('center_axis',(1.,0.,0.)) ;
#108845=DIRECTION('ref_axis',(0.,0.,-1.)) ;
#108846=DIRECTION('center_axis',(1.,0.,0.)) ;
#108847=DIRECTION('ref_axis',(0.,0.,-1.)) ;
#108848=DIRECTION('center_axis',(0.,-1.,-1.22464679914735E-16)) ;
#108849=DIRECTION('ref_axis',(0.,-1.22464679914735E-16,1.)) ;
#108850=DIRECTION('center_axis',(-1.,0.,0.)) ;
#108851=DIRECTION('ref_axis',(0.,0.,-1.)) ;
#108852=DIRECTION('center_axis',(-1.,0.,0.)) ;
#108853=DIRECTION('ref_axis',(0.,0.,-1.)) ;
#108854=DIRECTION('center_axis',(-1.,0.,0.)) ;
#108855=DIRECTION('ref_axis',(0.,0.,1.)) ;
#108856=DIRECTION('center_axis',(-1.,0.,0.)) ;
#108857=DIRECTION('ref_axis',(0.,0.,1.)) ;
#108858=DIRECTION('center_axis',(0.,1.,-1.22464679914735E-16)) ;
#108859=DIRECTION('ref_axis',(0.,-1.22464679914735E-16,-1.)) ;
#108860=DIRECTION('center_axis',(1.,0.,0.)) ;
#108861=DIRECTION('ref_axis',(0.,0.,1.)) ;
#108862=DIRECTION('center_axis',(0.,1.,0.)) ;
#108863=DIRECTION('ref_axis',(0.,0.,1.)) ;
#108864=DIRECTION('center_axis',(-1.,0.,0.)) ;
#108865=DIRECTION('ref_axis',(0.,0.,-1.)) ;
#108866=DIRECTION('center_axis',(0.,0.707106781186558,0.707106781186537)) ;
#108867=DIRECTION('ref_axis',(0.,-0.707106781186537,0.707106781186558)) ;
#108868=DIRECTION('center_axis',(0.,0.,-1.)) ;
#108869=DIRECTION('ref_axis',(-1.,0.,0.)) ;
#108870=DIRECTION('center_axis',(2.16840434497101E-16,-1.,1.30104260698261E-16)) ;
#108871=DIRECTION('ref_axis',(1.,2.16840434497101E-16,-1.09476442525376E-47)) ;
#108872=DIRECTION('center_axis',(-5.4946818858058E-13,-0.707106781186505,
-0.70710678118659)) ;
#108873=DIRECTION('ref_axis',(1.03835885983909E-10,0.70710678118659,-0.707106781186505)) ;
#108874=DIRECTION('center_axis',(-5.42101086242752E-16,1.,0.)) ;
#108875=DIRECTION('ref_axis',(1.,5.42101086242752E-16,0.)) ;
#108876=DIRECTION('',(-2.16840434497101E-16,1.,-1.30104260698261E-16)) ;
#108877=DIRECTION('center_axis',(0.,1.,0.)) ;
#108878=DIRECTION('ref_axis',(0.,0.,1.)) ;
#108879=DIRECTION('',(2.16840434497101E-16,-1.,1.30104260698261E-16)) ;
#108880=DIRECTION('',(2.16840434497101E-16,-1.,1.30104260698261E-16)) ;
#108881=DIRECTION('center_axis',(1.,0.,0.)) ;
#108882=DIRECTION('ref_axis',(0.,0.,-1.)) ;
#108883=DIRECTION('center_axis',(1.,0.,0.)) ;
#108884=DIRECTION('ref_axis',(0.,0.,-1.)) ;
#108885=DIRECTION('center_axis',(0.,-1.,-1.22464679914735E-16)) ;
#108886=DIRECTION('ref_axis',(0.,-1.22464679914735E-16,1.)) ;
#108887=DIRECTION('center_axis',(-1.,0.,0.)) ;
#108888=DIRECTION('ref_axis',(0.,0.,-1.)) ;
#108889=DIRECTION('center_axis',(-1.,0.,0.)) ;
#108890=DIRECTION('ref_axis',(0.,0.,-1.)) ;
#108891=DIRECTION('center_axis',(-1.,0.,0.)) ;
#108892=DIRECTION('ref_axis',(0.,0.,1.)) ;
#108893=DIRECTION('center_axis',(-1.,0.,0.)) ;
#108894=DIRECTION('ref_axis',(0.,0.,1.)) ;
#108895=DIRECTION('center_axis',(0.,1.,-1.22464679914735E-16)) ;
#108896=DIRECTION('ref_axis',(0.,-1.22464679914735E-16,-1.)) ;
#108897=DIRECTION('center_axis',(1.,0.,0.)) ;
#108898=DIRECTION('ref_axis',(0.,0.,1.)) ;
#108899=DIRECTION('center_axis',(0.,1.,0.)) ;
#108900=DIRECTION('ref_axis',(0.,0.,1.)) ;
#108901=DIRECTION('center_axis',(-1.,0.,0.)) ;
#108902=DIRECTION('ref_axis',(0.,0.,-1.)) ;
#108903=DIRECTION('center_axis',(0.,0.707106781186558,0.707106781186537)) ;
#108904=DIRECTION('ref_axis',(0.,-0.707106781186537,0.707106781186558)) ;
#108905=DIRECTION('center_axis',(0.,0.,-1.)) ;
#108906=DIRECTION('ref_axis',(-1.,0.,0.)) ;
#108907=DIRECTION('center_axis',(2.16840434497101E-16,-1.,1.30104260698261E-16)) ;
#108908=DIRECTION('ref_axis',(1.,2.16840434497101E-16,-1.09476442525376E-47)) ;
#108909=DIRECTION('center_axis',(-4.61475062295467E-13,-0.707106781186512,
-0.707106781186583)) ;
#108910=DIRECTION('ref_axis',(8.2666922773353E-11,0.707106781186583,-0.707106781186512)) ;
#108911=DIRECTION('center_axis',(-5.42101086242752E-16,1.,0.)) ;
#108912=DIRECTION('ref_axis',(1.,5.42101086242752E-16,0.)) ;
#108913=DIRECTION('',(-2.16840434497101E-16,1.,-1.30104260698261E-16)) ;
#108914=DIRECTION('center_axis',(0.,1.,0.)) ;
#108915=DIRECTION('ref_axis',(0.,0.,1.)) ;
#108916=DIRECTION('',(2.16840434497101E-16,-1.,1.30104260698261E-16)) ;
#108917=DIRECTION('',(2.16840434497101E-16,-1.,1.30104260698261E-16)) ;
#108918=DIRECTION('center_axis',(1.,0.,0.)) ;
#108919=DIRECTION('ref_axis',(0.,0.,-1.)) ;
#108920=DIRECTION('center_axis',(1.,0.,0.)) ;
#108921=DIRECTION('ref_axis',(0.,0.,-1.)) ;
#108922=DIRECTION('center_axis',(0.,-1.,-1.22464679914735E-16)) ;
#108923=DIRECTION('ref_axis',(0.,-1.22464679914735E-16,1.)) ;
#108924=DIRECTION('center_axis',(-1.,0.,0.)) ;
#108925=DIRECTION('ref_axis',(0.,0.,-1.)) ;
#108926=DIRECTION('center_axis',(-1.,0.,0.)) ;
#108927=DIRECTION('ref_axis',(0.,0.,-1.)) ;
#108928=DIRECTION('center_axis',(-1.,0.,0.)) ;
#108929=DIRECTION('ref_axis',(0.,0.,1.)) ;
#108930=DIRECTION('center_axis',(-1.,0.,0.)) ;
#108931=DIRECTION('ref_axis',(0.,0.,1.)) ;
#108932=DIRECTION('center_axis',(0.,1.,-1.22464679914735E-16)) ;
#108933=DIRECTION('ref_axis',(0.,-1.22464679914735E-16,-1.)) ;
#108934=DIRECTION('center_axis',(1.,0.,0.)) ;
#108935=DIRECTION('ref_axis',(0.,0.,1.)) ;
#108936=DIRECTION('center_axis',(0.,1.,0.)) ;
#108937=DIRECTION('ref_axis',(0.,0.,1.)) ;
#108938=DIRECTION('center_axis',(-1.,0.,0.)) ;
#108939=DIRECTION('ref_axis',(0.,0.,-1.)) ;
#108940=DIRECTION('center_axis',(0.,0.707106781186545,0.70710678118655)) ;
#108941=DIRECTION('ref_axis',(0.,-0.70710678118655,0.707106781186545)) ;
#108942=DIRECTION('center_axis',(0.,0.,-1.)) ;
#108943=DIRECTION('ref_axis',(-1.,0.,0.)) ;
#108944=DIRECTION('center_axis',(2.16840434497101E-16,-1.,1.30104260698261E-16)) ;
#108945=DIRECTION('ref_axis',(1.,2.16840434497101E-16,-1.09476442525376E-47)) ;
#108946=DIRECTION('center_axis',(-6.37461314865721E-13,-0.707106781186499,
-0.707106781186596)) ;
#108947=DIRECTION('ref_axis',(-7.23831307879934E-11,0.707106781186596,-0.707106781186499)) ;
#108948=DIRECTION('center_axis',(-5.42101086242752E-16,1.,0.)) ;
#108949=DIRECTION('ref_axis',(1.,5.42101086242752E-16,0.)) ;
#108950=DIRECTION('',(-2.16840434497101E-16,1.,-1.30104260698261E-16)) ;
#108951=DIRECTION('center_axis',(0.,1.,0.)) ;
#108952=DIRECTION('ref_axis',(0.,0.,1.)) ;
#108953=DIRECTION('',(2.16840434497101E-16,-1.,1.30104260698261E-16)) ;
#108954=DIRECTION('',(2.16840434497101E-16,-1.,1.30104260698261E-16)) ;
#108955=DIRECTION('center_axis',(1.,0.,0.)) ;
#108956=DIRECTION('ref_axis',(0.,0.,-1.)) ;
#108957=DIRECTION('center_axis',(1.,0.,0.)) ;
#108958=DIRECTION('ref_axis',(0.,0.,-1.)) ;
#108959=DIRECTION('center_axis',(0.,-1.,-1.22464679914735E-16)) ;
#108960=DIRECTION('ref_axis',(0.,-1.22464679914735E-16,1.)) ;
#108961=DIRECTION('center_axis',(-1.,0.,0.)) ;
#108962=DIRECTION('ref_axis',(0.,0.,-1.)) ;
#108963=DIRECTION('center_axis',(-1.,0.,0.)) ;
#108964=DIRECTION('ref_axis',(0.,0.,-1.)) ;
#108965=DIRECTION('center_axis',(-1.,0.,0.)) ;
#108966=DIRECTION('ref_axis',(0.,0.,1.)) ;
#108967=DIRECTION('center_axis',(-1.,0.,0.)) ;
#108968=DIRECTION('ref_axis',(0.,0.,1.)) ;
#108969=DIRECTION('center_axis',(0.,1.,-1.22464679914735E-16)) ;
#108970=DIRECTION('ref_axis',(0.,-1.22464679914735E-16,-1.)) ;
#108971=DIRECTION('center_axis',(1.,0.,0.)) ;
#108972=DIRECTION('ref_axis',(0.,0.,1.)) ;
#108973=DIRECTION('center_axis',(0.,1.,0.)) ;
#108974=DIRECTION('ref_axis',(0.,0.,1.)) ;
#108975=DIRECTION('center_axis',(-1.,0.,0.)) ;
#108976=DIRECTION('ref_axis',(0.,0.,-1.)) ;
#108977=DIRECTION('center_axis',(0.,0.707106781186545,0.70710678118655)) ;
#108978=DIRECTION('ref_axis',(0.,-0.70710678118655,0.707106781186545)) ;
#108979=DIRECTION('center_axis',(0.,0.,-1.)) ;
#108980=DIRECTION('ref_axis',(-1.,0.,0.)) ;
#108981=DIRECTION('center_axis',(2.16840434497101E-16,-1.,1.30104260698261E-16)) ;
#108982=DIRECTION('ref_axis',(1.,2.16840434497101E-16,-1.09476442525376E-47)) ;
#108983=DIRECTION('center_axis',(-2.04144052981523E-12,-0.707106781186384,
-0.707106781186711)) ;
#108984=DIRECTION('ref_axis',(3.79286005912221E-12,0.707106781186711,-0.707106781186384)) ;
#108985=DIRECTION('center_axis',(-5.42101086242752E-16,1.,0.)) ;
#108986=DIRECTION('ref_axis',(1.,5.42101086242752E-16,0.)) ;
#108987=DIRECTION('',(-2.16840434497101E-16,1.,-1.30104260698261E-16)) ;
#108988=DIRECTION('center_axis',(0.,1.,0.)) ;
#108989=DIRECTION('ref_axis',(0.,0.,1.)) ;
#108990=DIRECTION('',(2.16840434497101E-16,-1.,1.30104260698261E-16)) ;
#108991=DIRECTION('',(2.16840434497101E-16,-1.,1.30104260698261E-16)) ;
#108992=DIRECTION('center_axis',(1.,0.,0.)) ;
#108993=DIRECTION('ref_axis',(0.,0.,-1.)) ;
#108994=DIRECTION('center_axis',(1.,0.,0.)) ;
#108995=DIRECTION('ref_axis',(0.,0.,-1.)) ;
#108996=DIRECTION('center_axis',(0.,-1.,-1.22464679914735E-16)) ;
#108997=DIRECTION('ref_axis',(0.,-1.22464679914735E-16,1.)) ;
#108998=DIRECTION('center_axis',(-1.,0.,0.)) ;
#108999=DIRECTION('ref_axis',(0.,0.,-1.)) ;
#109000=DIRECTION('center_axis',(-1.,0.,0.)) ;
#109001=DIRECTION('ref_axis',(0.,0.,-1.)) ;
#109002=DIRECTION('center_axis',(-1.,0.,0.)) ;
#109003=DIRECTION('ref_axis',(0.,0.,1.)) ;
#109004=DIRECTION('center_axis',(-1.,0.,0.)) ;
#109005=DIRECTION('ref_axis',(0.,0.,1.)) ;
#109006=DIRECTION('center_axis',(0.,1.,-1.22464679914735E-16)) ;
#109007=DIRECTION('ref_axis',(0.,-1.22464679914735E-16,-1.)) ;
#109008=DIRECTION('center_axis',(1.,0.,0.)) ;
#109009=DIRECTION('ref_axis',(0.,0.,1.)) ;
#109010=DIRECTION('center_axis',(0.,1.,0.)) ;
#109011=DIRECTION('ref_axis',(0.,0.,1.)) ;
#109012=DIRECTION('center_axis',(-1.,0.,0.)) ;
#109013=DIRECTION('ref_axis',(0.,0.,-1.)) ;
#109014=DIRECTION('center_axis',(0.,0.707106781186545,0.70710678118655)) ;
#109015=DIRECTION('ref_axis',(0.,-0.70710678118655,0.707106781186545)) ;
#109016=DIRECTION('center_axis',(0.,0.,-1.)) ;
#109017=DIRECTION('ref_axis',(-1.,0.,0.)) ;
#109018=DIRECTION('center_axis',(2.16840434497101E-16,-1.,1.30104260698261E-16)) ;
#109019=DIRECTION('ref_axis',(1.,2.16840434497101E-16,-1.09476442525376E-47)) ;
#109020=DIRECTION('center_axis',(-1.65035996854789E-12,-0.707106781186426,
-0.707106781186669)) ;
#109021=DIRECTION('ref_axis',(-9.42995735618098E-12,0.707106781186669,-0.707106781186426)) ;
#109022=DIRECTION('center_axis',(-5.42101086242752E-16,1.,0.)) ;
#109023=DIRECTION('ref_axis',(1.,5.42101086242752E-16,0.)) ;
#109024=DIRECTION('',(-2.16840434497101E-16,1.,-1.30104260698261E-16)) ;
#109025=DIRECTION('center_axis',(0.,1.,0.)) ;
#109026=DIRECTION('ref_axis',(0.,0.,1.)) ;
#109027=DIRECTION('',(2.16840434497101E-16,-1.,1.30104260698261E-16)) ;
#109028=DIRECTION('',(2.16840434497101E-16,-1.,1.30104260698261E-16)) ;
#109029=DIRECTION('center_axis',(1.,0.,0.)) ;
#109030=DIRECTION('ref_axis',(0.,0.,-1.)) ;
#109031=DIRECTION('center_axis',(1.,0.,0.)) ;
#109032=DIRECTION('ref_axis',(0.,0.,-1.)) ;
#109033=DIRECTION('center_axis',(0.,-1.,-1.22464679914735E-16)) ;
#109034=DIRECTION('ref_axis',(0.,-1.22464679914735E-16,1.)) ;
#109035=DIRECTION('center_axis',(-1.,0.,0.)) ;
#109036=DIRECTION('ref_axis',(0.,0.,-1.)) ;
#109037=DIRECTION('center_axis',(-1.,0.,0.)) ;
#109038=DIRECTION('ref_axis',(0.,0.,-1.)) ;
#109039=DIRECTION('center_axis',(1.,0.,0.)) ;
#109040=DIRECTION('ref_axis',(0.,0.,-1.)) ;
#109041=DIRECTION('center_axis',(-1.,0.,0.)) ;
#109042=DIRECTION('ref_axis',(0.,0.,-1.)) ;
#109043=DIRECTION('center_axis',(0.,0.,1.)) ;
#109044=DIRECTION('ref_axis',(1.,0.,0.)) ;
#109045=DIRECTION('center_axis',(1.,0.,0.)) ;
#109046=DIRECTION('ref_axis',(0.,0.,-1.)) ;
#109047=DIRECTION('center_axis',(0.,0.707106781186548,-0.707106781186548)) ;
#109048=DIRECTION('ref_axis',(0.,0.707106781186548,0.707106781186548)) ;
#109049=DIRECTION('center_axis',(1.,0.,0.)) ;
#109050=DIRECTION('ref_axis',(0.,0.,-1.)) ;
#109051=DIRECTION('center_axis',(-1.,0.,0.)) ;
#109052=DIRECTION('ref_axis',(0.,0.,-1.)) ;
#109053=DIRECTION('center_axis',(0.,0.,1.)) ;
#109054=DIRECTION('ref_axis',(1.,0.,0.)) ;
#109055=DIRECTION('center_axis',(1.,0.,0.)) ;
#109056=DIRECTION('ref_axis',(0.,0.,-1.)) ;
#109057=DIRECTION('center_axis',(0.,0.707106781186548,-0.707106781186548)) ;
#109058=DIRECTION('ref_axis',(0.,0.707106781186548,0.707106781186548)) ;
#109059=DIRECTION('center_axis',(1.,0.,0.)) ;
#109060=DIRECTION('ref_axis',(0.,0.,-1.)) ;
#109061=DIRECTION('center_axis',(-1.,0.,0.)) ;
#109062=DIRECTION('ref_axis',(0.,0.,-1.)) ;
#109063=DIRECTION('center_axis',(0.,0.,1.)) ;
#109064=DIRECTION('ref_axis',(1.,0.,0.)) ;
#109065=DIRECTION('center_axis',(1.,0.,0.)) ;
#109066=DIRECTION('ref_axis',(0.,0.,-1.)) ;
#109067=DIRECTION('center_axis',(0.,0.707106781186548,-0.707106781186548)) ;
#109068=DIRECTION('ref_axis',(0.,0.707106781186548,0.707106781186548)) ;
#109069=DIRECTION('center_axis',(1.,0.,0.)) ;
#109070=DIRECTION('ref_axis',(0.,0.,-1.)) ;
#109071=DIRECTION('center_axis',(-1.,0.,0.)) ;
#109072=DIRECTION('ref_axis',(0.,0.,-1.)) ;
#109073=DIRECTION('center_axis',(0.,0.,1.)) ;
#109074=DIRECTION('ref_axis',(1.,0.,0.)) ;
#109075=DIRECTION('center_axis',(1.,0.,0.)) ;
#109076=DIRECTION('ref_axis',(0.,0.,-1.)) ;
#109077=DIRECTION('center_axis',(0.,0.707106781186539,-0.707106781186556)) ;
#109078=DIRECTION('ref_axis',(0.,0.707106781186556,0.707106781186539)) ;
#109079=DIRECTION('center_axis',(1.,0.,0.)) ;
#109080=DIRECTION('ref_axis',(0.,0.,-1.)) ;
#109081=DIRECTION('center_axis',(-1.,0.,0.)) ;
#109082=DIRECTION('ref_axis',(0.,0.,-1.)) ;
#109083=DIRECTION('center_axis',(0.,0.,1.)) ;
#109084=DIRECTION('ref_axis',(1.,0.,0.)) ;
#109085=DIRECTION('center_axis',(1.,0.,0.)) ;
#109086=DIRECTION('ref_axis',(0.,0.,-1.)) ;
#109087=DIRECTION('center_axis',(0.,0.707106781186539,-0.707106781186556)) ;
#109088=DIRECTION('ref_axis',(0.,0.707106781186556,0.707106781186539)) ;
#109089=DIRECTION('center_axis',(1.,0.,0.)) ;
#109090=DIRECTION('ref_axis',(0.,0.,-1.)) ;
#109091=DIRECTION('center_axis',(-1.,0.,0.)) ;
#109092=DIRECTION('ref_axis',(0.,0.,-1.)) ;
#109093=DIRECTION('center_axis',(0.,0.,1.)) ;
#109094=DIRECTION('ref_axis',(1.,0.,0.)) ;
#109095=DIRECTION('center_axis',(1.,0.,0.)) ;
#109096=DIRECTION('ref_axis',(0.,0.,-1.)) ;
#109097=DIRECTION('center_axis',(0.,0.707106781186539,-0.707106781186556)) ;
#109098=DIRECTION('ref_axis',(0.,0.707106781186556,0.707106781186539)) ;
#109099=DIRECTION('center_axis',(1.,0.,0.)) ;
#109100=DIRECTION('ref_axis',(0.,0.,-1.)) ;
#109101=DIRECTION('center_axis',(-1.,0.,0.)) ;
#109102=DIRECTION('ref_axis',(0.,0.,-1.)) ;
#109103=DIRECTION('center_axis',(0.,0.,1.)) ;
#109104=DIRECTION('ref_axis',(1.,0.,0.)) ;
#109105=DIRECTION('center_axis',(1.,0.,0.)) ;
#109106=DIRECTION('ref_axis',(0.,0.,-1.)) ;
#109107=DIRECTION('center_axis',(0.,0.707106781186539,-0.707106781186556)) ;
#109108=DIRECTION('ref_axis',(0.,0.707106781186556,0.707106781186539)) ;
#109109=DIRECTION('center_axis',(1.,0.,0.)) ;
#109110=DIRECTION('ref_axis',(0.,0.,-1.)) ;
#109111=DIRECTION('center_axis',(-1.,0.,0.)) ;
#109112=DIRECTION('ref_axis',(0.,0.,-1.)) ;
#109113=DIRECTION('center_axis',(0.,0.,1.)) ;
#109114=DIRECTION('ref_axis',(1.,0.,0.)) ;
#109115=DIRECTION('center_axis',(1.,0.,0.)) ;
#109116=DIRECTION('ref_axis',(0.,0.,-1.)) ;
#109117=DIRECTION('center_axis',(-6.13317366673346E-15,0.707106781186539,
-0.707106781186556)) ;
#109118=DIRECTION('ref_axis',(3.80912633391397E-29,0.707106781186556,0.707106781186539)) ;
#109119=DIRECTION('center_axis',(1.,0.,0.)) ;
#109120=DIRECTION('ref_axis',(0.,0.,-1.)) ;
#109121=DIRECTION('center_axis',(-1.,0.,0.)) ;
#109122=DIRECTION('ref_axis',(0.,0.,-1.)) ;
#109123=DIRECTION('center_axis',(0.,0.,1.)) ;
#109124=DIRECTION('ref_axis',(1.,0.,0.)) ;
#109125=DIRECTION('center_axis',(1.,0.,0.)) ;
#109126=DIRECTION('ref_axis',(0.,0.,-1.)) ;
#109127=DIRECTION('center_axis',(-6.13317366673346E-15,0.707106781186539,
-0.707106781186556)) ;
#109128=DIRECTION('ref_axis',(3.80912633391397E-29,0.707106781186556,0.707106781186539)) ;
#109129=DIRECTION('center_axis',(-1.,0.,0.)) ;
#109130=DIRECTION('ref_axis',(0.,0.,1.)) ;
#109131=DIRECTION('center_axis',(-1.,0.,0.)) ;
#109132=DIRECTION('ref_axis',(0.,0.,1.)) ;
#109133=DIRECTION('center_axis',(0.,1.,-1.22464679914735E-16)) ;
#109134=DIRECTION('ref_axis',(0.,-1.22464679914735E-16,-1.)) ;
#109135=DIRECTION('center_axis',(1.,0.,0.)) ;
#109136=DIRECTION('ref_axis',(0.,0.,1.)) ;
#109137=DIRECTION('center_axis',(0.,1.,0.)) ;
#109138=DIRECTION('ref_axis',(0.,0.,1.)) ;
#109139=DIRECTION('center_axis',(-1.,0.,0.)) ;
#109140=DIRECTION('ref_axis',(0.,0.,-1.)) ;
#109141=DIRECTION('center_axis',(0.,0.70710678118655,0.707106781186545)) ;
#109142=DIRECTION('ref_axis',(0.,-0.707106781186545,0.70710678118655)) ;
#109143=DIRECTION('center_axis',(0.,0.,-1.)) ;
#109144=DIRECTION('ref_axis',(-1.,0.,0.)) ;
#109145=DIRECTION('center_axis',(2.16840434497101E-16,-1.,1.30104260698261E-16)) ;
#109146=DIRECTION('ref_axis',(1.,2.16840434497101E-16,-1.09476442525376E-47)) ;
#109147=DIRECTION('center_axis',(6.64836954154425E-14,-0.707106781186552,
-0.707106781186543)) ;
#109148=DIRECTION('ref_axis',(-1.70648371771735E-11,0.707106781186543,-0.707106781186552)) ;
#109149=DIRECTION('center_axis',(-5.42101086242752E-16,1.,0.)) ;
#109150=DIRECTION('ref_axis',(1.,5.42101086242752E-16,0.)) ;
#109151=DIRECTION('',(-2.16840434497101E-16,1.,-1.30104260698261E-16)) ;
#109152=DIRECTION('center_axis',(0.,1.,0.)) ;
#109153=DIRECTION('ref_axis',(0.,0.,1.)) ;
#109154=DIRECTION('',(2.16840434497101E-16,-1.,1.30104260698261E-16)) ;
#109155=DIRECTION('',(2.16840434497101E-16,-1.,1.30104260698261E-16)) ;
#109156=DIRECTION('center_axis',(-1.,0.,0.)) ;
#109157=DIRECTION('ref_axis',(0.,0.,1.)) ;
#109158=DIRECTION('',(1.,0.,0.)) ;
#109159=DIRECTION('center_axis',(-1.,0.,0.)) ;
#109160=DIRECTION('ref_axis',(0.,0.,1.)) ;
#109161=DIRECTION('',(1.,0.,0.)) ;
#109162=DIRECTION('center_axis',(-1.,0.,0.)) ;
#109163=DIRECTION('ref_axis',(0.,0.,1.)) ;
#109164=DIRECTION('',(1.,0.,0.)) ;
#109165=DIRECTION('center_axis',(-1.,0.,0.)) ;
#109166=DIRECTION('ref_axis',(0.,0.,1.)) ;
#109167=DIRECTION('',(1.,0.,0.)) ;
#109168=DIRECTION('center_axis',(-1.,0.,0.)) ;
#109169=DIRECTION('ref_axis',(0.,0.,1.)) ;
#109170=DIRECTION('',(1.,0.,0.)) ;
#109171=DIRECTION('center_axis',(-1.,0.,0.)) ;
#109172=DIRECTION('ref_axis',(0.,0.,1.)) ;
#109173=DIRECTION('',(1.,0.,0.)) ;
#109174=DIRECTION('center_axis',(-1.,0.,0.)) ;
#109175=DIRECTION('ref_axis',(0.,0.,1.)) ;
#109176=DIRECTION('',(1.,0.,0.)) ;
#109177=DIRECTION('center_axis',(-1.,0.,0.)) ;
#109178=DIRECTION('ref_axis',(0.,0.,1.)) ;
#109179=DIRECTION('',(1.,0.,0.)) ;
#109180=DIRECTION('center_axis',(-1.,0.,0.)) ;
#109181=DIRECTION('ref_axis',(0.,0.,1.)) ;
#109182=DIRECTION('',(1.,0.,0.)) ;
#109183=DIRECTION('center_axis',(1.,0.,0.)) ;
#109184=DIRECTION('ref_axis',(0.,0.,-1.)) ;
#109185=DIRECTION('center_axis',(-1.,0.,0.)) ;
#109186=DIRECTION('ref_axis',(0.,0.,-1.)) ;
#109187=DIRECTION('',(1.,0.,0.)) ;
#109188=DIRECTION('',(1.,0.,0.)) ;
#109189=DIRECTION('center_axis',(1.,0.,0.)) ;
#109190=DIRECTION('ref_axis',(0.,0.,-1.)) ;
#109191=DIRECTION('center_axis',(-1.,0.,0.)) ;
#109192=DIRECTION('ref_axis',(0.,0.,-1.)) ;
#109193=DIRECTION('',(1.,0.,0.)) ;
#109194=DIRECTION('',(1.,0.,0.)) ;
#109195=DIRECTION('center_axis',(1.,0.,0.)) ;
#109196=DIRECTION('ref_axis',(0.,0.,-1.)) ;
#109197=DIRECTION('center_axis',(-1.,0.,0.)) ;
#109198=DIRECTION('ref_axis',(0.,0.,-1.)) ;
#109199=DIRECTION('',(1.,0.,0.)) ;
#109200=DIRECTION('',(1.,0.,0.)) ;
#109201=DIRECTION('center_axis',(1.,0.,0.)) ;
#109202=DIRECTION('ref_axis',(0.,0.,-1.)) ;
#109203=DIRECTION('center_axis',(-1.,0.,0.)) ;
#109204=DIRECTION('ref_axis',(0.,0.,-1.)) ;
#109205=DIRECTION('',(1.,0.,0.)) ;
#109206=DIRECTION('',(1.,0.,0.)) ;
#109207=DIRECTION('center_axis',(1.,0.,0.)) ;
#109208=DIRECTION('ref_axis',(0.,0.,-1.)) ;
#109209=DIRECTION('center_axis',(-1.,0.,0.)) ;
#109210=DIRECTION('ref_axis',(0.,0.,-1.)) ;
#109211=DIRECTION('',(1.,0.,0.)) ;
#109212=DIRECTION('',(1.,0.,0.)) ;
#109213=DIRECTION('center_axis',(1.,0.,0.)) ;
#109214=DIRECTION('ref_axis',(0.,0.,-1.)) ;
#109215=DIRECTION('center_axis',(-1.,0.,0.)) ;
#109216=DIRECTION('ref_axis',(0.,0.,-1.)) ;
#109217=DIRECTION('',(1.,0.,0.)) ;
#109218=DIRECTION('',(1.,0.,0.)) ;
#109219=DIRECTION('center_axis',(1.,0.,0.)) ;
#109220=DIRECTION('ref_axis',(0.,0.,-1.)) ;
#109221=DIRECTION('center_axis',(-1.,0.,0.)) ;
#109222=DIRECTION('ref_axis',(0.,0.,-1.)) ;
#109223=DIRECTION('',(1.,0.,0.)) ;
#109224=DIRECTION('',(1.,0.,0.)) ;
#109225=DIRECTION('center_axis',(1.,0.,0.)) ;
#109226=DIRECTION('ref_axis',(0.,0.,-1.)) ;
#109227=DIRECTION('center_axis',(-1.,0.,0.)) ;
#109228=DIRECTION('ref_axis',(0.,0.,-1.)) ;
#109229=DIRECTION('',(1.,0.,0.)) ;
#109230=DIRECTION('',(1.,0.,0.)) ;
#109231=DIRECTION('center_axis',(1.,0.,0.)) ;
#109232=DIRECTION('ref_axis',(0.,0.,-1.)) ;
#109233=DIRECTION('center_axis',(-1.,0.,0.)) ;
#109234=DIRECTION('ref_axis',(0.,0.,-1.)) ;
#109235=DIRECTION('',(1.,0.,0.)) ;
#109236=DIRECTION('',(1.,0.,0.)) ;
#109237=DIRECTION('center_axis',(1.,0.,0.)) ;
#109238=DIRECTION('ref_axis',(0.,0.,-1.)) ;
#109239=DIRECTION('center_axis',(1.,0.,0.)) ;
#109240=DIRECTION('ref_axis',(0.,0.,-1.)) ;
#109241=DIRECTION('center_axis',(0.,-1.,-1.22464679914735E-16)) ;
#109242=DIRECTION('ref_axis',(0.,-1.22464679914735E-16,1.)) ;
#109243=DIRECTION('center_axis',(-1.,0.,0.)) ;
#109244=DIRECTION('ref_axis',(0.,0.,-1.)) ;
#109245=DIRECTION('center_axis',(-1.,0.,0.)) ;
#109246=DIRECTION('ref_axis',(0.,0.,-1.)) ;
#109247=DIRECTION('center_axis',(1.,0.,0.)) ;
#109248=DIRECTION('ref_axis',(0.,0.,-1.)) ;
#109249=DIRECTION('center_axis',(-1.,0.,0.)) ;
#109250=DIRECTION('ref_axis',(0.,0.,-1.)) ;
#109251=DIRECTION('center_axis',(0.,0.,1.)) ;
#109252=DIRECTION('ref_axis',(1.,0.,0.)) ;
#109253=DIRECTION('center_axis',(1.,0.,0.)) ;
#109254=DIRECTION('ref_axis',(0.,0.,-1.)) ;
#109255=DIRECTION('center_axis',(0.,0.707106781186548,-0.707106781186548)) ;
#109256=DIRECTION('ref_axis',(0.,0.707106781186548,0.707106781186548)) ;
#109257=DIRECTION('center_axis',(-1.,0.,0.)) ;
#109258=DIRECTION('ref_axis',(0.,0.,1.)) ;
#109259=DIRECTION('center_axis',(-1.,0.,0.)) ;
#109260=DIRECTION('ref_axis',(0.,0.,1.)) ;
#109261=DIRECTION('center_axis',(0.,1.,-1.22464679914735E-16)) ;
#109262=DIRECTION('ref_axis',(0.,-1.22464679914735E-16,-1.)) ;
#109263=DIRECTION('center_axis',(1.,0.,0.)) ;
#109264=DIRECTION('ref_axis',(0.,0.,1.)) ;
#109265=DIRECTION('center_axis',(0.,1.,0.)) ;
#109266=DIRECTION('ref_axis',(0.,0.,1.)) ;
#109267=DIRECTION('center_axis',(-1.,0.,0.)) ;
#109268=DIRECTION('ref_axis',(0.,0.,-1.)) ;
#109269=DIRECTION('center_axis',(0.,0.70710678118655,0.707106781186545)) ;
#109270=DIRECTION('ref_axis',(0.,-0.707106781186545,0.70710678118655)) ;
#109271=DIRECTION('center_axis',(0.,0.,-1.)) ;
#109272=DIRECTION('ref_axis',(-1.,0.,0.)) ;
#109273=DIRECTION('center_axis',(2.16840434497101E-16,-1.,1.30104260698261E-16)) ;
#109274=DIRECTION('ref_axis',(1.,2.16840434497101E-16,-1.09476442525376E-47)) ;
#109275=DIRECTION('center_axis',(-1.95540280633655E-15,-0.707106781186549,
-0.707106781186546)) ;
#109276=DIRECTION('ref_axis',(-2.18299406319968E-11,0.707106781186546,-0.707106781186549)) ;
#109277=DIRECTION('center_axis',(-5.42101086242752E-16,1.,0.)) ;
#109278=DIRECTION('ref_axis',(1.,5.42101086242752E-16,0.)) ;
#109279=DIRECTION('',(-2.16840434497101E-16,1.,-1.30104260698261E-16)) ;
#109280=DIRECTION('center_axis',(0.,1.,0.)) ;
#109281=DIRECTION('ref_axis',(0.,0.,1.)) ;
#109282=DIRECTION('',(2.16840434497101E-16,-1.,1.30104260698261E-16)) ;
#109283=DIRECTION('',(2.16840434497101E-16,-1.,1.30104260698261E-16)) ;
#109284=DIRECTION('center_axis',(-1.,0.,0.)) ;
#109285=DIRECTION('ref_axis',(0.,0.,1.)) ;
#109286=DIRECTION('',(1.,0.,0.)) ;
#109287=DIRECTION('center_axis',(1.,0.,0.)) ;
#109288=DIRECTION('ref_axis',(0.,0.,-1.)) ;
#109289=DIRECTION('center_axis',(-1.,0.,0.)) ;
#109290=DIRECTION('ref_axis',(0.,0.,-1.)) ;
#109291=DIRECTION('',(1.,0.,0.)) ;
#109292=DIRECTION('',(1.,0.,0.)) ;
#109293=DIRECTION('center_axis',(-1.,-2.16840434497101E-16,0.)) ;
#109294=DIRECTION('ref_axis',(2.16840434497101E-16,-1.,0.)) ;
#109295=DIRECTION('',(-2.16840434497101E-16,1.,1.30104260698261E-16)) ;
#109296=DIRECTION('center_axis',(1.,2.16840434497101E-16,0.)) ;
#109297=DIRECTION('ref_axis',(2.16840434497101E-16,-1.,0.)) ;
#109298=DIRECTION('',(0.,0.,-1.)) ;
#109299=DIRECTION('center_axis',(1.,2.16840434497101E-16,0.)) ;
#109300=DIRECTION('ref_axis',(2.16840434497101E-16,-1.,0.)) ;
#109301=DIRECTION('center_axis',(-1.,-2.16840434497101E-16,0.)) ;
#109302=DIRECTION('ref_axis',(2.16840434497101E-16,-1.,0.)) ;
#109303=DIRECTION('',(0.,0.,-1.)) ;
#109304=DIRECTION('',(2.16840434497101E-16,-1.,5.10212787052002E-17)) ;
#109305=DIRECTION('',(0.,0.,1.)) ;
#109306=DIRECTION('',(-2.16840434497101E-16,1.,-1.020425574104E-16)) ;
#109307=DIRECTION('',(0.,0.,-1.)) ;
#109308=DIRECTION('center_axis',(-1.,-2.16840434497101E-16,0.)) ;
#109309=DIRECTION('ref_axis',(2.16840434497101E-16,-1.,0.)) ;
#109310=DIRECTION('center_axis',(-1.,-2.16840434497101E-16,0.)) ;
#109311=DIRECTION('ref_axis',(2.16840434497101E-16,-1.,0.)) ;
#109312=DIRECTION('',(-2.16840434497101E-16,1.,1.30104260698261E-16)) ;
#109313=DIRECTION('center_axis',(1.,2.16840434497101E-16,0.)) ;
#109314=DIRECTION('ref_axis',(2.16840434497101E-16,-1.,0.)) ;
#109315=DIRECTION('',(0.,0.,-1.)) ;
#109316=DIRECTION('center_axis',(1.,2.16840434497101E-16,0.)) ;
#109317=DIRECTION('ref_axis',(2.16840434497101E-16,-1.,0.)) ;
#109318=DIRECTION('center_axis',(-1.,-2.16840434497101E-16,0.)) ;
#109319=DIRECTION('ref_axis',(2.16840434497101E-16,-1.,0.)) ;
#109320=DIRECTION('',(0.,0.,-1.)) ;
#109321=DIRECTION('',(2.16840434497101E-16,-1.,5.10212787052002E-17)) ;
#109322=DIRECTION('',(0.,0.,1.)) ;
#109323=DIRECTION('',(-2.16840434497101E-16,1.,-1.020425574104E-16)) ;
#109324=DIRECTION('',(0.,0.,-1.)) ;
#109325=DIRECTION('center_axis',(-1.,-2.16840434497101E-16,0.)) ;
#109326=DIRECTION('ref_axis',(2.16840434497101E-16,-1.,0.)) ;
#109327=DIRECTION('center_axis',(-1.,-2.16840434497101E-16,0.)) ;
#109328=DIRECTION('ref_axis',(2.16840434497101E-16,-1.,0.)) ;
#109329=DIRECTION('',(-2.16840434497101E-16,1.,1.30104260698261E-16)) ;
#109330=DIRECTION('center_axis',(1.,2.16840434497101E-16,0.)) ;
#109331=DIRECTION('ref_axis',(2.16840434497101E-16,-1.,0.)) ;
#109332=DIRECTION('',(0.,0.,-1.)) ;
#109333=DIRECTION('center_axis',(1.,2.16840434497101E-16,0.)) ;
#109334=DIRECTION('ref_axis',(2.16840434497101E-16,-1.,0.)) ;
#109335=DIRECTION('center_axis',(-1.,-2.16840434497101E-16,0.)) ;
#109336=DIRECTION('ref_axis',(2.16840434497101E-16,-1.,0.)) ;
#109337=DIRECTION('',(0.,0.,-1.)) ;
#109338=DIRECTION('',(2.16840434497101E-16,-1.,5.10212787052002E-17)) ;
#109339=DIRECTION('',(0.,0.,1.)) ;
#109340=DIRECTION('',(-2.16840434497101E-16,1.,-1.020425574104E-16)) ;
#109341=DIRECTION('',(0.,0.,-1.)) ;
#109342=DIRECTION('center_axis',(-1.,-2.16840434497101E-16,0.)) ;
#109343=DIRECTION('ref_axis',(2.16840434497101E-16,-1.,0.)) ;
#109344=DIRECTION('center_axis',(-1.,-2.16840434497101E-16,0.)) ;
#109345=DIRECTION('ref_axis',(2.16840434497101E-16,-1.,0.)) ;
#109346=DIRECTION('',(-2.16840434497101E-16,1.,1.30104260698261E-16)) ;
#109347=DIRECTION('center_axis',(1.,2.16840434497101E-16,0.)) ;
#109348=DIRECTION('ref_axis',(2.16840434497101E-16,-1.,0.)) ;
#109349=DIRECTION('',(0.,0.,-1.)) ;
#109350=DIRECTION('center_axis',(1.,2.16840434497101E-16,0.)) ;
#109351=DIRECTION('ref_axis',(2.16840434497101E-16,-1.,0.)) ;
#109352=DIRECTION('center_axis',(-1.,-2.16840434497101E-16,0.)) ;
#109353=DIRECTION('ref_axis',(2.16840434497101E-16,-1.,0.)) ;
#109354=DIRECTION('',(0.,0.,-1.)) ;
#109355=DIRECTION('',(2.16840434497101E-16,-1.,5.10212787052002E-17)) ;
#109356=DIRECTION('',(0.,0.,1.)) ;
#109357=DIRECTION('',(-2.16840434497101E-16,1.,-1.020425574104E-16)) ;
#109358=DIRECTION('',(0.,0.,-1.)) ;
#109359=DIRECTION('center_axis',(-1.,-2.16840434497101E-16,0.)) ;
#109360=DIRECTION('ref_axis',(2.16840434497101E-16,-1.,0.)) ;
#109361=DIRECTION('center_axis',(-1.,-2.16840434497101E-16,0.)) ;
#109362=DIRECTION('ref_axis',(2.16840434497101E-16,-1.,0.)) ;
#109363=DIRECTION('',(-2.16840434497101E-16,1.,1.30104260698261E-16)) ;
#109364=DIRECTION('center_axis',(1.,2.16840434497101E-16,0.)) ;
#109365=DIRECTION('ref_axis',(2.16840434497101E-16,-1.,0.)) ;
#109366=DIRECTION('',(0.,0.,-1.)) ;
#109367=DIRECTION('center_axis',(1.,2.16840434497101E-16,0.)) ;
#109368=DIRECTION('ref_axis',(2.16840434497101E-16,-1.,0.)) ;
#109369=DIRECTION('center_axis',(-1.,-2.16840434497101E-16,0.)) ;
#109370=DIRECTION('ref_axis',(2.16840434497101E-16,-1.,0.)) ;
#109371=DIRECTION('',(0.,0.,-1.)) ;
#109372=DIRECTION('',(2.16840434497101E-16,-1.,5.10212787052002E-17)) ;
#109373=DIRECTION('',(0.,0.,1.)) ;
#109374=DIRECTION('',(-2.16840434497101E-16,1.,-1.020425574104E-16)) ;
#109375=DIRECTION('',(0.,0.,-1.)) ;
#109376=DIRECTION('center_axis',(-1.,-2.16840434497101E-16,0.)) ;
#109377=DIRECTION('ref_axis',(2.16840434497101E-16,-1.,0.)) ;
#109378=DIRECTION('center_axis',(-1.,-2.16840434497101E-16,0.)) ;
#109379=DIRECTION('ref_axis',(2.16840434497101E-16,-1.,0.)) ;
#109380=DIRECTION('',(-2.16840434497101E-16,1.,1.30104260698261E-16)) ;
#109381=DIRECTION('center_axis',(1.,2.16840434497101E-16,0.)) ;
#109382=DIRECTION('ref_axis',(2.16840434497101E-16,-1.,0.)) ;
#109383=DIRECTION('',(0.,0.,-1.)) ;
#109384=DIRECTION('center_axis',(1.,2.16840434497101E-16,0.)) ;
#109385=DIRECTION('ref_axis',(2.16840434497101E-16,-1.,0.)) ;
#109386=DIRECTION('center_axis',(-1.,-2.16840434497101E-16,0.)) ;
#109387=DIRECTION('ref_axis',(2.16840434497101E-16,-1.,0.)) ;
#109388=DIRECTION('',(0.,0.,-1.)) ;
#109389=DIRECTION('',(2.16840434497101E-16,-1.,5.10212787052002E-17)) ;
#109390=DIRECTION('',(0.,0.,1.)) ;
#109391=DIRECTION('',(-2.16840434497101E-16,1.,-1.020425574104E-16)) ;
#109392=DIRECTION('',(0.,0.,-1.)) ;
#109393=DIRECTION('center_axis',(-1.,-2.16840434497101E-16,0.)) ;
#109394=DIRECTION('ref_axis',(2.16840434497101E-16,-1.,0.)) ;
#109395=DIRECTION('center_axis',(-1.,-2.16840434497101E-16,0.)) ;
#109396=DIRECTION('ref_axis',(2.16840434497101E-16,-1.,0.)) ;
#109397=DIRECTION('',(-2.16840434497101E-16,1.,1.30104260698261E-16)) ;
#109398=DIRECTION('center_axis',(1.,2.16840434497101E-16,0.)) ;
#109399=DIRECTION('ref_axis',(2.16840434497101E-16,-1.,0.)) ;
#109400=DIRECTION('',(0.,0.,-1.)) ;
#109401=DIRECTION('center_axis',(1.,2.16840434497101E-16,0.)) ;
#109402=DIRECTION('ref_axis',(2.16840434497101E-16,-1.,0.)) ;
#109403=DIRECTION('center_axis',(-1.,-2.16840434497101E-16,0.)) ;
#109404=DIRECTION('ref_axis',(2.16840434497101E-16,-1.,0.)) ;
#109405=DIRECTION('',(0.,0.,-1.)) ;
#109406=DIRECTION('',(2.16840434497101E-16,-1.,5.10212787052002E-17)) ;
#109407=DIRECTION('',(0.,0.,1.)) ;
#109408=DIRECTION('',(-2.16840434497101E-16,1.,-1.020425574104E-16)) ;
#109409=DIRECTION('',(0.,0.,-1.)) ;
#109410=DIRECTION('center_axis',(-1.,-2.16840434497101E-16,0.)) ;
#109411=DIRECTION('ref_axis',(2.16840434497101E-16,-1.,0.)) ;
#109412=DIRECTION('center_axis',(-1.,-2.16840434497101E-16,0.)) ;
#109413=DIRECTION('ref_axis',(2.16840434497101E-16,-1.,0.)) ;
#109414=DIRECTION('',(-2.16840434497101E-16,1.,1.30104260698261E-16)) ;
#109415=DIRECTION('center_axis',(1.,2.16840434497101E-16,0.)) ;
#109416=DIRECTION('ref_axis',(2.16840434497101E-16,-1.,0.)) ;
#109417=DIRECTION('',(0.,0.,-1.)) ;
#109418=DIRECTION('center_axis',(1.,2.16840434497101E-16,0.)) ;
#109419=DIRECTION('ref_axis',(2.16840434497101E-16,-1.,0.)) ;
#109420=DIRECTION('center_axis',(-1.,-2.16840434497101E-16,0.)) ;
#109421=DIRECTION('ref_axis',(2.16840434497101E-16,-1.,0.)) ;
#109422=DIRECTION('',(0.,0.,-1.)) ;
#109423=DIRECTION('',(2.16840434497101E-16,-1.,5.10212787052002E-17)) ;
#109424=DIRECTION('',(0.,0.,1.)) ;
#109425=DIRECTION('',(-2.16840434497101E-16,1.,-1.020425574104E-16)) ;
#109426=DIRECTION('',(0.,0.,-1.)) ;
#109427=DIRECTION('center_axis',(-1.,-2.16840434497101E-16,0.)) ;
#109428=DIRECTION('ref_axis',(2.16840434497101E-16,-1.,0.)) ;
#109429=DIRECTION('center_axis',(-1.,-2.16840434497101E-16,0.)) ;
#109430=DIRECTION('ref_axis',(2.16840434497101E-16,-1.,0.)) ;
#109431=DIRECTION('',(-2.16840434497101E-16,1.,1.30104260698261E-16)) ;
#109432=DIRECTION('center_axis',(1.,2.16840434497101E-16,0.)) ;
#109433=DIRECTION('ref_axis',(2.16840434497101E-16,-1.,0.)) ;
#109434=DIRECTION('',(0.,0.,-1.)) ;
#109435=DIRECTION('center_axis',(1.,2.16840434497101E-16,0.)) ;
#109436=DIRECTION('ref_axis',(2.16840434497101E-16,-1.,0.)) ;
#109437=DIRECTION('center_axis',(-1.,-2.16840434497101E-16,0.)) ;
#109438=DIRECTION('ref_axis',(2.16840434497101E-16,-1.,0.)) ;
#109439=DIRECTION('',(0.,0.,-1.)) ;
#109440=DIRECTION('',(2.16840434497101E-16,-1.,5.10212787052002E-17)) ;
#109441=DIRECTION('',(0.,0.,1.)) ;
#109442=DIRECTION('',(-2.16840434497101E-16,1.,-1.020425574104E-16)) ;
#109443=DIRECTION('',(0.,0.,-1.)) ;
#109444=DIRECTION('center_axis',(-1.,-2.16840434497101E-16,0.)) ;
#109445=DIRECTION('ref_axis',(2.16840434497101E-16,-1.,0.)) ;
#109446=DIRECTION('center_axis',(6.27714964143733E-33,-5.10212787052002E-17,
-1.)) ;
#109447=DIRECTION('ref_axis',(0.,1.,-5.10212787052002E-17)) ;
#109448=DIRECTION('center_axis',(-6.27714964143733E-33,5.10212787052002E-17,
1.)) ;
#109449=DIRECTION('ref_axis',(3.20268201330022E-49,1.,-5.10212787052002E-17)) ;
#109450=DIRECTION('',(1.2303003375722E-16,-1.,5.10212787052002E-17)) ;
#109451=DIRECTION('',(1.,0.,6.27714964143733E-33)) ;
#109452=DIRECTION('',(-2.16840434497101E-16,1.,-5.10212787052002E-17)) ;
#109453=DIRECTION('',(-1.,-1.53063836115601E-16,1.53236300070382E-33)) ;
#109454=DIRECTION('center_axis',(-1.25542992828747E-32,1.020425574104E-16,
1.)) ;
#109455=DIRECTION('ref_axis',(0.,-1.,1.020425574104E-16)) ;
#109456=DIRECTION('center_axis',(1.25542992828747E-32,-1.020425574104E-16,
-1.)) ;
#109457=DIRECTION('ref_axis',(-1.28107280532009E-48,-1.,1.020425574104E-16)) ;
#109458=DIRECTION('',(1.,1.53063836115601E-16,-3.06472600140763E-33)) ;
#109459=DIRECTION('',(2.16840434497101E-16,-1.,1.020425574104E-16)) ;
#109460=DIRECTION('',(-1.,0.,-1.25542992828747E-32)) ;
#109461=DIRECTION('',(-1.2303003375722E-16,1.,-1.020425574104E-16)) ;
#109462=DIRECTION('center_axis',(6.27714964143733E-33,-5.10212787052002E-17,
-1.)) ;
#109463=DIRECTION('ref_axis',(0.,1.,-5.10212787052002E-17)) ;
#109464=DIRECTION('center_axis',(-6.27714964143733E-33,5.10212787052002E-17,
1.)) ;
#109465=DIRECTION('ref_axis',(3.20268201330022E-49,1.,-5.10212787052002E-17)) ;
#109466=DIRECTION('',(1.2303003375722E-16,-1.,5.10212787052002E-17)) ;
#109467=DIRECTION('',(1.,0.,6.27714964143733E-33)) ;
#109468=DIRECTION('',(-2.16840434497101E-16,1.,-5.10212787052002E-17)) ;
#109469=DIRECTION('',(-1.,-1.53063836115601E-16,1.53236300070382E-33)) ;
#109470=DIRECTION('center_axis',(-1.25542992828747E-32,1.020425574104E-16,
1.)) ;
#109471=DIRECTION('ref_axis',(0.,-1.,1.020425574104E-16)) ;
#109472=DIRECTION('center_axis',(1.25542992828747E-32,-1.020425574104E-16,
-1.)) ;
#109473=DIRECTION('ref_axis',(-1.28107280532009E-48,-1.,1.020425574104E-16)) ;
#109474=DIRECTION('',(1.,1.53063836115601E-16,-3.06472600140763E-33)) ;
#109475=DIRECTION('',(2.16840434497101E-16,-1.,1.020425574104E-16)) ;
#109476=DIRECTION('',(-1.,0.,-1.25542992828747E-32)) ;
#109477=DIRECTION('',(-1.2303003375722E-16,1.,-1.020425574104E-16)) ;
#109478=DIRECTION('center_axis',(6.27714964143733E-33,-5.10212787052002E-17,
-1.)) ;
#109479=DIRECTION('ref_axis',(0.,1.,-5.10212787052002E-17)) ;
#109480=DIRECTION('center_axis',(-6.27714964143733E-33,5.10212787052002E-17,
1.)) ;
#109481=DIRECTION('ref_axis',(3.20268201330022E-49,1.,-5.10212787052002E-17)) ;
#109482=DIRECTION('',(1.2303003375722E-16,-1.,5.10212787052002E-17)) ;
#109483=DIRECTION('',(1.,0.,6.27714964143733E-33)) ;
#109484=DIRECTION('',(-2.16840434497101E-16,1.,-5.10212787052002E-17)) ;
#109485=DIRECTION('',(-1.,-1.53063836115601E-16,1.53236300070382E-33)) ;
#109486=DIRECTION('center_axis',(-1.25542992828747E-32,1.020425574104E-16,
1.)) ;
#109487=DIRECTION('ref_axis',(0.,-1.,1.020425574104E-16)) ;
#109488=DIRECTION('center_axis',(1.25542992828747E-32,-1.020425574104E-16,
-1.)) ;
#109489=DIRECTION('ref_axis',(-1.28107280532009E-48,-1.,1.020425574104E-16)) ;
#109490=DIRECTION('',(1.,1.53063836115601E-16,-3.06472600140763E-33)) ;
#109491=DIRECTION('',(2.16840434497101E-16,-1.,1.020425574104E-16)) ;
#109492=DIRECTION('',(-1.,0.,-1.25542992828747E-32)) ;
#109493=DIRECTION('',(-1.2303003375722E-16,1.,-1.020425574104E-16)) ;
#109494=DIRECTION('center_axis',(6.27714964143733E-33,-5.10212787052002E-17,
-1.)) ;
#109495=DIRECTION('ref_axis',(0.,1.,-5.10212787052002E-17)) ;
#109496=DIRECTION('center_axis',(-6.27714964143733E-33,5.10212787052002E-17,
1.)) ;
#109497=DIRECTION('ref_axis',(3.20268201330022E-49,1.,-5.10212787052002E-17)) ;
#109498=DIRECTION('',(1.2303003375722E-16,-1.,5.10212787052002E-17)) ;
#109499=DIRECTION('',(1.,0.,6.27714964143733E-33)) ;
#109500=DIRECTION('',(-2.16840434497101E-16,1.,-5.10212787052002E-17)) ;
#109501=DIRECTION('',(-1.,-1.53063836115601E-16,1.53236300070382E-33)) ;
#109502=DIRECTION('center_axis',(-1.25542992828747E-32,1.020425574104E-16,
1.)) ;
#109503=DIRECTION('ref_axis',(0.,-1.,1.020425574104E-16)) ;
#109504=DIRECTION('center_axis',(1.25542992828747E-32,-1.020425574104E-16,
-1.)) ;
#109505=DIRECTION('ref_axis',(-1.28107280532009E-48,-1.,1.020425574104E-16)) ;
#109506=DIRECTION('',(1.,1.53063836115601E-16,-3.06472600140763E-33)) ;
#109507=DIRECTION('',(2.16840434497101E-16,-1.,1.020425574104E-16)) ;
#109508=DIRECTION('',(-1.,0.,-1.25542992828747E-32)) ;
#109509=DIRECTION('',(-1.2303003375722E-16,1.,-1.020425574104E-16)) ;
#109510=DIRECTION('center_axis',(6.27714964143733E-33,-5.10212787052002E-17,
-1.)) ;
#109511=DIRECTION('ref_axis',(0.,1.,-5.10212787052002E-17)) ;
#109512=DIRECTION('center_axis',(-6.27714964143733E-33,5.10212787052002E-17,
1.)) ;
#109513=DIRECTION('ref_axis',(3.20268201330022E-49,1.,-5.10212787052002E-17)) ;
#109514=DIRECTION('',(1.2303003375722E-16,-1.,5.10212787052002E-17)) ;
#109515=DIRECTION('',(1.,0.,6.27714964143733E-33)) ;
#109516=DIRECTION('',(-2.16840434497101E-16,1.,-5.10212787052002E-17)) ;
#109517=DIRECTION('',(-1.,-1.53063836115601E-16,1.53236300070382E-33)) ;
#109518=DIRECTION('center_axis',(-1.25542992828747E-32,1.020425574104E-16,
1.)) ;
#109519=DIRECTION('ref_axis',(0.,-1.,1.020425574104E-16)) ;
#109520=DIRECTION('center_axis',(1.25542992828747E-32,-1.020425574104E-16,
-1.)) ;
#109521=DIRECTION('ref_axis',(-1.28107280532009E-48,-1.,1.020425574104E-16)) ;
#109522=DIRECTION('',(1.,1.53063836115601E-16,-3.06472600140763E-33)) ;
#109523=DIRECTION('',(2.16840434497101E-16,-1.,1.020425574104E-16)) ;
#109524=DIRECTION('',(-1.,0.,-1.25542992828747E-32)) ;
#109525=DIRECTION('',(-1.2303003375722E-16,1.,-1.020425574104E-16)) ;
#109526=DIRECTION('center_axis',(6.27714964143733E-33,-5.10212787052002E-17,
-1.)) ;
#109527=DIRECTION('ref_axis',(0.,1.,-5.10212787052002E-17)) ;
#109528=DIRECTION('center_axis',(-6.27714964143733E-33,5.10212787052002E-17,
1.)) ;
#109529=DIRECTION('ref_axis',(3.20268201330022E-49,1.,-5.10212787052002E-17)) ;
#109530=DIRECTION('',(1.2303003375722E-16,-1.,5.10212787052002E-17)) ;
#109531=DIRECTION('',(1.,0.,6.27714964143733E-33)) ;
#109532=DIRECTION('',(-2.16840434497101E-16,1.,-5.10212787052002E-17)) ;
#109533=DIRECTION('',(-1.,-1.53063836115601E-16,1.53236300070382E-33)) ;
#109534=DIRECTION('center_axis',(-1.25542992828747E-32,1.020425574104E-16,
1.)) ;
#109535=DIRECTION('ref_axis',(0.,-1.,1.020425574104E-16)) ;
#109536=DIRECTION('center_axis',(1.25542992828747E-32,-1.020425574104E-16,
-1.)) ;
#109537=DIRECTION('ref_axis',(-1.28107280532009E-48,-1.,1.020425574104E-16)) ;
#109538=DIRECTION('',(1.,1.53063836115601E-16,-3.06472600140763E-33)) ;
#109539=DIRECTION('',(2.16840434497101E-16,-1.,1.020425574104E-16)) ;
#109540=DIRECTION('',(-1.,0.,-1.25542992828747E-32)) ;
#109541=DIRECTION('',(-1.2303003375722E-16,1.,-1.020425574104E-16)) ;
#109542=DIRECTION('center_axis',(6.27714964143733E-33,-5.10212787052002E-17,
-1.)) ;
#109543=DIRECTION('ref_axis',(0.,1.,-5.10212787052002E-17)) ;
#109544=DIRECTION('center_axis',(-6.27714964143733E-33,5.10212787052002E-17,
1.)) ;
#109545=DIRECTION('ref_axis',(3.20268201330022E-49,1.,-5.10212787052002E-17)) ;
#109546=DIRECTION('',(1.2303003375722E-16,-1.,5.10212787052002E-17)) ;
#109547=DIRECTION('',(1.,0.,6.27714964143733E-33)) ;
#109548=DIRECTION('',(-2.16840434497101E-16,1.,-5.10212787052002E-17)) ;
#109549=DIRECTION('',(-1.,-1.53063836115601E-16,1.53236300070382E-33)) ;
#109550=DIRECTION('center_axis',(-1.25542992828747E-32,1.020425574104E-16,
1.)) ;
#109551=DIRECTION('ref_axis',(0.,-1.,1.020425574104E-16)) ;
#109552=DIRECTION('center_axis',(1.25542992828747E-32,-1.020425574104E-16,
-1.)) ;
#109553=DIRECTION('ref_axis',(-1.28107280532009E-48,-1.,1.020425574104E-16)) ;
#109554=DIRECTION('',(1.,1.53063836115601E-16,-3.06472600140763E-33)) ;
#109555=DIRECTION('',(2.16840434497101E-16,-1.,1.020425574104E-16)) ;
#109556=DIRECTION('',(-1.,0.,-1.25542992828747E-32)) ;
#109557=DIRECTION('',(-1.2303003375722E-16,1.,-1.020425574104E-16)) ;
#109558=DIRECTION('center_axis',(6.27714964143733E-33,-5.10212787052002E-17,
-1.)) ;
#109559=DIRECTION('ref_axis',(0.,1.,-5.10212787052002E-17)) ;
#109560=DIRECTION('center_axis',(-6.27714964143733E-33,5.10212787052002E-17,
1.)) ;
#109561=DIRECTION('ref_axis',(3.20268201330022E-49,1.,-5.10212787052002E-17)) ;
#109562=DIRECTION('',(1.2303003375722E-16,-1.,5.10212787052002E-17)) ;
#109563=DIRECTION('',(1.,0.,6.27714964143733E-33)) ;
#109564=DIRECTION('',(-2.16840434497101E-16,1.,-5.10212787052002E-17)) ;
#109565=DIRECTION('',(-1.,-1.53063836115601E-16,1.53236300070382E-33)) ;
#109566=DIRECTION('center_axis',(-1.25542992828747E-32,1.020425574104E-16,
1.)) ;
#109567=DIRECTION('ref_axis',(0.,-1.,1.020425574104E-16)) ;
#109568=DIRECTION('center_axis',(1.25542992828747E-32,-1.020425574104E-16,
-1.)) ;
#109569=DIRECTION('ref_axis',(-1.28107280532009E-48,-1.,1.020425574104E-16)) ;
#109570=DIRECTION('',(1.,1.53063836115601E-16,-3.06472600140763E-33)) ;
#109571=DIRECTION('',(2.16840434497101E-16,-1.,1.020425574104E-16)) ;
#109572=DIRECTION('',(-1.,0.,-1.25542992828747E-32)) ;
#109573=DIRECTION('',(-1.2303003375722E-16,1.,-1.020425574104E-16)) ;
#109574=DIRECTION('center_axis',(6.27714964143733E-33,-5.10212787052002E-17,
-1.)) ;
#109575=DIRECTION('ref_axis',(0.,1.,-5.10212787052002E-17)) ;
#109576=DIRECTION('center_axis',(-6.27714964143733E-33,5.10212787052002E-17,
1.)) ;
#109577=DIRECTION('ref_axis',(3.20268201330022E-49,1.,-5.10212787052002E-17)) ;
#109578=DIRECTION('',(1.2303003375722E-16,-1.,5.10212787052002E-17)) ;
#109579=DIRECTION('',(1.,0.,6.27714964143733E-33)) ;
#109580=DIRECTION('',(-2.16840434497101E-16,1.,-5.10212787052002E-17)) ;
#109581=DIRECTION('',(-1.,-1.53063836115601E-16,1.53236300070382E-33)) ;
#109582=DIRECTION('center_axis',(-1.25542992828747E-32,1.020425574104E-16,
1.)) ;
#109583=DIRECTION('ref_axis',(0.,-1.,1.020425574104E-16)) ;
#109584=DIRECTION('center_axis',(1.25542992828747E-32,-1.020425574104E-16,
-1.)) ;
#109585=DIRECTION('ref_axis',(-1.28107280532009E-48,-1.,1.020425574104E-16)) ;
#109586=DIRECTION('',(1.,1.53063836115601E-16,-3.06472600140763E-33)) ;
#109587=DIRECTION('',(2.16840434497101E-16,-1.,1.020425574104E-16)) ;
#109588=DIRECTION('',(-1.,0.,-1.25542992828747E-32)) ;
#109589=DIRECTION('',(-1.2303003375722E-16,1.,-1.020425574104E-16)) ;
#109590=DIRECTION('center_axis',(0.,0.,1.)) ;
#109591=DIRECTION('ref_axis',(1.,0.,0.)) ;
#109592=DIRECTION('',(0.,0.,1.)) ;
#109593=DIRECTION('center_axis',(0.,0.,1.)) ;
#109594=DIRECTION('ref_axis',(1.,0.,0.)) ;
#109595=DIRECTION('',(0.,0.,1.)) ;
#109596=DIRECTION('center_axis',(0.,0.,-1.)) ;
#109597=DIRECTION('ref_axis',(1.,0.,0.)) ;
#109598=DIRECTION('center_axis',(0.,0.,1.)) ;
#109599=DIRECTION('ref_axis',(1.,0.,0.)) ;
#109600=DIRECTION('',(0.,0.,1.)) ;
#109601=DIRECTION('center_axis',(0.,0.,1.)) ;
#109602=DIRECTION('ref_axis',(1.,0.,0.)) ;
#109603=DIRECTION('',(0.,0.,1.)) ;
#109604=DIRECTION('center_axis',(0.,0.,-1.)) ;
#109605=DIRECTION('ref_axis',(1.,0.,0.)) ;
#109606=DIRECTION('center_axis',(0.,0.,1.)) ;
#109607=DIRECTION('ref_axis',(1.,0.,0.)) ;
#109608=DIRECTION('',(0.,0.,1.)) ;
#109609=DIRECTION('center_axis',(0.,0.,1.)) ;
#109610=DIRECTION('ref_axis',(1.,0.,0.)) ;
#109611=DIRECTION('',(0.,0.,1.)) ;
#109612=DIRECTION('center_axis',(0.,0.,-1.)) ;
#109613=DIRECTION('ref_axis',(1.,0.,0.)) ;
#109614=DIRECTION('center_axis',(0.,0.,1.)) ;
#109615=DIRECTION('ref_axis',(1.,0.,0.)) ;
#109616=DIRECTION('',(0.,0.,1.)) ;
#109617=DIRECTION('center_axis',(0.,0.,1.)) ;
#109618=DIRECTION('ref_axis',(1.,0.,0.)) ;
#109619=DIRECTION('',(0.,0.,1.)) ;
#109620=DIRECTION('center_axis',(0.,0.,-1.)) ;
#109621=DIRECTION('ref_axis',(1.,0.,0.)) ;
#109622=DIRECTION('center_axis',(0.,0.,1.)) ;
#109623=DIRECTION('ref_axis',(1.,0.,0.)) ;
#109624=DIRECTION('',(0.,0.,1.)) ;
#109625=DIRECTION('center_axis',(0.,0.,1.)) ;
#109626=DIRECTION('ref_axis',(1.,0.,0.)) ;
#109627=DIRECTION('',(0.,0.,1.)) ;
#109628=DIRECTION('center_axis',(0.,0.,-1.)) ;
#109629=DIRECTION('ref_axis',(1.,0.,0.)) ;
#109630=DIRECTION('center_axis',(0.,0.,1.)) ;
#109631=DIRECTION('ref_axis',(1.,0.,0.)) ;
#109632=DIRECTION('',(0.,0.,1.)) ;
#109633=DIRECTION('center_axis',(0.,0.,1.)) ;
#109634=DIRECTION('ref_axis',(1.,0.,0.)) ;
#109635=DIRECTION('',(0.,0.,1.)) ;
#109636=DIRECTION('center_axis',(0.,0.,-1.)) ;
#109637=DIRECTION('ref_axis',(1.,0.,0.)) ;
#109638=DIRECTION('center_axis',(0.,0.,1.)) ;
#109639=DIRECTION('ref_axis',(1.,0.,0.)) ;
#109640=DIRECTION('',(0.,0.,1.)) ;
#109641=DIRECTION('center_axis',(0.,0.,1.)) ;
#109642=DIRECTION('ref_axis',(1.,0.,0.)) ;
#109643=DIRECTION('',(0.,0.,1.)) ;
#109644=DIRECTION('center_axis',(0.,0.,-1.)) ;
#109645=DIRECTION('ref_axis',(1.,0.,0.)) ;
#109646=DIRECTION('center_axis',(0.,0.,1.)) ;
#109647=DIRECTION('ref_axis',(1.,0.,0.)) ;
#109648=DIRECTION('',(0.,0.,1.)) ;
#109649=DIRECTION('center_axis',(0.,0.,1.)) ;
#109650=DIRECTION('ref_axis',(1.,0.,0.)) ;
#109651=DIRECTION('',(0.,0.,1.)) ;
#109652=DIRECTION('center_axis',(0.,0.,-1.)) ;
#109653=DIRECTION('ref_axis',(1.,0.,0.)) ;
#109654=DIRECTION('center_axis',(0.,0.,1.)) ;
#109655=DIRECTION('ref_axis',(1.,0.,0.)) ;
#109656=DIRECTION('',(0.,0.,1.)) ;
#109657=DIRECTION('center_axis',(0.,0.,1.)) ;
#109658=DIRECTION('ref_axis',(1.,0.,0.)) ;
#109659=DIRECTION('',(0.,0.,1.)) ;
#109660=DIRECTION('center_axis',(0.,0.,-1.)) ;
#109661=DIRECTION('ref_axis',(1.,0.,0.)) ;
#109662=DIRECTION('center_axis',(-1.,-2.16840434497101E-16,0.)) ;
#109663=DIRECTION('ref_axis',(2.16840434497101E-16,-1.,0.)) ;
#109664=DIRECTION('',(-2.16840434497101E-16,1.,1.30104260698261E-16)) ;
#109665=DIRECTION('center_axis',(1.,2.16840434497101E-16,0.)) ;
#109666=DIRECTION('ref_axis',(2.16840434497101E-16,-1.,0.)) ;
#109667=DIRECTION('',(0.,0.,-1.)) ;
#109668=DIRECTION('center_axis',(1.,2.16840434497101E-16,0.)) ;
#109669=DIRECTION('ref_axis',(2.16840434497101E-16,-1.,0.)) ;
#109670=DIRECTION('center_axis',(-1.,-2.16840434497101E-16,0.)) ;
#109671=DIRECTION('ref_axis',(2.16840434497101E-16,-1.,0.)) ;
#109672=DIRECTION('',(0.,0.,-1.)) ;
#109673=DIRECTION('',(2.16840434497101E-16,-1.,5.10212787052002E-17)) ;
#109674=DIRECTION('',(0.,0.,1.)) ;
#109675=DIRECTION('',(-2.16840434497101E-16,1.,-1.020425574104E-16)) ;
#109676=DIRECTION('',(0.,0.,-1.)) ;
#109677=DIRECTION('center_axis',(-1.,-2.16840434497101E-16,0.)) ;
#109678=DIRECTION('ref_axis',(2.16840434497101E-16,-1.,0.)) ;
#109679=DIRECTION('center_axis',(6.27714964143733E-33,-5.10212787052002E-17,
-1.)) ;
#109680=DIRECTION('ref_axis',(0.,1.,-5.10212787052002E-17)) ;
#109681=DIRECTION('center_axis',(-6.27714964143733E-33,5.10212787052002E-17,
1.)) ;
#109682=DIRECTION('ref_axis',(3.20268201330022E-49,1.,-5.10212787052002E-17)) ;
#109683=DIRECTION('',(1.2303003375722E-16,-1.,5.10212787052002E-17)) ;
#109684=DIRECTION('',(1.,0.,6.27714964143733E-33)) ;
#109685=DIRECTION('',(-2.16840434497101E-16,1.,-5.10212787052002E-17)) ;
#109686=DIRECTION('',(-1.,-1.53063836115601E-16,1.53236300070382E-33)) ;
#109687=DIRECTION('center_axis',(-1.25542992828747E-32,1.020425574104E-16,
1.)) ;
#109688=DIRECTION('ref_axis',(0.,-1.,1.020425574104E-16)) ;
#109689=DIRECTION('center_axis',(1.25542992828747E-32,-1.020425574104E-16,
-1.)) ;
#109690=DIRECTION('ref_axis',(-1.28107280532009E-48,-1.,1.020425574104E-16)) ;
#109691=DIRECTION('',(1.,1.53063836115601E-16,-3.06472600140763E-33)) ;
#109692=DIRECTION('',(2.16840434497101E-16,-1.,1.020425574104E-16)) ;
#109693=DIRECTION('',(-1.,0.,-1.25542992828747E-32)) ;
#109694=DIRECTION('',(-1.2303003375722E-16,1.,-1.020425574104E-16)) ;
#109695=DIRECTION('center_axis',(0.,0.,1.)) ;
#109696=DIRECTION('ref_axis',(1.,0.,0.)) ;
#109697=DIRECTION('',(0.,0.,1.)) ;
#109698=DIRECTION('center_axis',(0.,0.,1.)) ;
#109699=DIRECTION('ref_axis',(1.,0.,0.)) ;
#109700=DIRECTION('',(0.,0.,1.)) ;
#109701=DIRECTION('center_axis',(0.,0.,-1.)) ;
#109702=DIRECTION('ref_axis',(1.,0.,0.)) ;
#109703=DIRECTION('center_axis',(0.,0.,1.)) ;
#109704=DIRECTION('ref_axis',(1.,0.,0.)) ;
#109705=DIRECTION('',(0.,0.,1.)) ;
#109706=DIRECTION('center_axis',(0.,0.,1.)) ;
#109707=DIRECTION('ref_axis',(1.,0.,0.)) ;
#109708=DIRECTION('',(0.,0.,1.)) ;
#109709=DIRECTION('center_axis',(0.,0.,-1.)) ;
#109710=DIRECTION('ref_axis',(1.,0.,0.)) ;
#109711=DIRECTION('center_axis',(0.,-1.,0.)) ;
#109712=DIRECTION('ref_axis',(0.,0.,-1.)) ;
#109713=DIRECTION('center_axis',(0.,-1.,0.)) ;
#109714=DIRECTION('ref_axis',(0.,0.,-1.)) ;
#109715=DIRECTION('',(-1.,0.,-6.27714964143733E-33)) ;
#109716=DIRECTION('',(0.,0.,1.)) ;
#109717=DIRECTION('',(1.,0.,0.)) ;
#109718=DIRECTION('',(-1.,0.,0.)) ;
#109719=DIRECTION('',(1.,0.,1.25542992828747E-32)) ;
#109720=DIRECTION('center_axis',(0.,-1.,0.)) ;
#109721=DIRECTION('ref_axis',(0.,0.,-1.)) ;
#109722=DIRECTION('',(0.,0.,-1.)) ;
#109723=DIRECTION('center_axis',(0.,-1.,0.)) ;
#109724=DIRECTION('ref_axis',(0.,0.,-1.)) ;
#109725=DIRECTION('',(-1.,0.,-6.27714964143733E-33)) ;
#109726=DIRECTION('',(1.,0.,1.25542992828747E-32)) ;
#109727=DIRECTION('center_axis',(0.,-1.,0.)) ;
#109728=DIRECTION('ref_axis',(0.,0.,-1.)) ;
#109729=DIRECTION('',(0.,0.,-1.)) ;
#109730=DIRECTION('center_axis',(0.,-1.,0.)) ;
#109731=DIRECTION('ref_axis',(0.,0.,-1.)) ;
#109732=DIRECTION('',(-1.,0.,-6.27714964143733E-33)) ;
#109733=DIRECTION('',(1.,0.,1.25542992828747E-32)) ;
#109734=DIRECTION('center_axis',(0.,-1.,0.)) ;
#109735=DIRECTION('ref_axis',(0.,0.,-1.)) ;
#109736=DIRECTION('',(0.,0.,-1.)) ;
#109737=DIRECTION('center_axis',(0.,-1.,0.)) ;
#109738=DIRECTION('ref_axis',(0.,0.,-1.)) ;
#109739=DIRECTION('',(-1.,0.,-6.27714964143733E-33)) ;
#109740=DIRECTION('',(1.,0.,1.25542992828747E-32)) ;
#109741=DIRECTION('center_axis',(0.,-1.,0.)) ;
#109742=DIRECTION('ref_axis',(0.,0.,-1.)) ;
#109743=DIRECTION('',(0.,0.,-1.)) ;
#109744=DIRECTION('center_axis',(0.,-1.,0.)) ;
#109745=DIRECTION('ref_axis',(0.,0.,-1.)) ;
#109746=DIRECTION('',(-1.,0.,-6.27714964143733E-33)) ;
#109747=DIRECTION('',(1.,0.,1.25542992828747E-32)) ;
#109748=DIRECTION('center_axis',(0.,-1.,0.)) ;
#109749=DIRECTION('ref_axis',(0.,0.,-1.)) ;
#109750=DIRECTION('',(0.,0.,-1.)) ;
#109751=DIRECTION('center_axis',(0.,-1.,0.)) ;
#109752=DIRECTION('ref_axis',(0.,0.,-1.)) ;
#109753=DIRECTION('',(-1.,0.,-6.27714964143733E-33)) ;
#109754=DIRECTION('',(1.,0.,1.25542992828747E-32)) ;
#109755=DIRECTION('center_axis',(0.,-1.,0.)) ;
#109756=DIRECTION('ref_axis',(0.,0.,-1.)) ;
#109757=DIRECTION('',(0.,0.,-1.)) ;
#109758=DIRECTION('center_axis',(0.,-1.,0.)) ;
#109759=DIRECTION('ref_axis',(0.,0.,-1.)) ;
#109760=DIRECTION('',(-1.,0.,-6.27714964143733E-33)) ;
#109761=DIRECTION('',(1.,0.,1.25542992828747E-32)) ;
#109762=DIRECTION('center_axis',(0.,-1.,0.)) ;
#109763=DIRECTION('ref_axis',(0.,0.,-1.)) ;
#109764=DIRECTION('',(0.,0.,-1.)) ;
#109765=DIRECTION('center_axis',(0.,-1.,0.)) ;
#109766=DIRECTION('ref_axis',(0.,0.,-1.)) ;
#109767=DIRECTION('',(-1.,0.,-6.27714964143733E-33)) ;
#109768=DIRECTION('',(1.,0.,1.25542992828747E-32)) ;
#109769=DIRECTION('center_axis',(0.,-1.,0.)) ;
#109770=DIRECTION('ref_axis',(0.,0.,-1.)) ;
#109771=DIRECTION('',(0.,0.,-1.)) ;
#109772=DIRECTION('center_axis',(0.,-1.,0.)) ;
#109773=DIRECTION('ref_axis',(0.,0.,-1.)) ;
#109774=DIRECTION('',(-1.,0.,-6.27714964143733E-33)) ;
#109775=DIRECTION('',(1.,0.,1.25542992828747E-32)) ;
#109776=DIRECTION('center_axis',(0.,-1.,0.)) ;
#109777=DIRECTION('ref_axis',(0.,0.,-1.)) ;
#109778=DIRECTION('',(0.,0.,-1.)) ;
#109779=DIRECTION('center_axis',(0.,-1.,0.)) ;
#109780=DIRECTION('ref_axis',(0.,0.,-1.)) ;
#109781=DIRECTION('',(-1.,0.,-6.27714964143733E-33)) ;
#109782=DIRECTION('',(1.,0.,1.25542992828747E-32)) ;
#109783=DIRECTION('center_axis',(0.,-1.,0.)) ;
#109784=DIRECTION('ref_axis',(0.,0.,-1.)) ;
#109785=DIRECTION('',(0.,0.,-1.)) ;
#109786=DIRECTION('center_axis',(0.,0.,1.)) ;
#109787=DIRECTION('ref_axis',(1.,0.,0.)) ;
#109788=DIRECTION('center_axis',(0.,0.,-1.)) ;
#109789=DIRECTION('ref_axis',(1.,0.,0.)) ;
#109790=DIRECTION('',(0.,0.,1.)) ;
#109791=DIRECTION('center_axis',(0.,0.,1.)) ;
#109792=DIRECTION('ref_axis',(1.,0.,0.)) ;
#109793=DIRECTION('center_axis',(-1.,-1.2303003375722E-16,0.)) ;
#109794=DIRECTION('ref_axis',(1.2303003375722E-16,-1.,0.)) ;
#109795=DIRECTION('center_axis',(-1.,-1.2303003375722E-16,0.)) ;
#109796=DIRECTION('ref_axis',(1.2303003375722E-16,-1.,0.)) ;
#109797=DIRECTION('',(1.2303003375722E-16,-1.,1.020425574104E-16)) ;
#109798=DIRECTION('',(-1.2303003375722E-16,1.,-5.10212787052002E-17)) ;
#109799=DIRECTION('center_axis',(-1.,-1.2303003375722E-16,0.)) ;
#109800=DIRECTION('ref_axis',(1.2303003375722E-16,-1.,0.)) ;
#109801=DIRECTION('',(0.,0.,1.)) ;
#109802=DIRECTION('center_axis',(-1.,-1.2303003375722E-16,0.)) ;
#109803=DIRECTION('ref_axis',(1.2303003375722E-16,-1.,0.)) ;
#109804=DIRECTION('',(1.2303003375722E-16,-1.,1.020425574104E-16)) ;
#109805=DIRECTION('',(-1.2303003375722E-16,1.,-5.10212787052002E-17)) ;
#109806=DIRECTION('center_axis',(-1.,-1.2303003375722E-16,0.)) ;
#109807=DIRECTION('ref_axis',(1.2303003375722E-16,-1.,0.)) ;
#109808=DIRECTION('',(0.,0.,1.)) ;
#109809=DIRECTION('center_axis',(-1.,-1.2303003375722E-16,0.)) ;
#109810=DIRECTION('ref_axis',(1.2303003375722E-16,-1.,0.)) ;
#109811=DIRECTION('',(1.2303003375722E-16,-1.,1.020425574104E-16)) ;
#109812=DIRECTION('',(-1.2303003375722E-16,1.,-5.10212787052002E-17)) ;
#109813=DIRECTION('center_axis',(-1.,-1.2303003375722E-16,0.)) ;
#109814=DIRECTION('ref_axis',(1.2303003375722E-16,-1.,0.)) ;
#109815=DIRECTION('',(0.,0.,1.)) ;
#109816=DIRECTION('center_axis',(-1.,-1.2303003375722E-16,0.)) ;
#109817=DIRECTION('ref_axis',(1.2303003375722E-16,-1.,0.)) ;
#109818=DIRECTION('',(1.2303003375722E-16,-1.,1.020425574104E-16)) ;
#109819=DIRECTION('',(-1.2303003375722E-16,1.,-5.10212787052002E-17)) ;
#109820=DIRECTION('center_axis',(-1.,-1.2303003375722E-16,0.)) ;
#109821=DIRECTION('ref_axis',(1.2303003375722E-16,-1.,0.)) ;
#109822=DIRECTION('',(0.,0.,1.)) ;
#109823=DIRECTION('center_axis',(-1.,-1.2303003375722E-16,0.)) ;
#109824=DIRECTION('ref_axis',(1.2303003375722E-16,-1.,0.)) ;
#109825=DIRECTION('',(1.2303003375722E-16,-1.,1.020425574104E-16)) ;
#109826=DIRECTION('',(-1.2303003375722E-16,1.,-5.10212787052002E-17)) ;
#109827=DIRECTION('center_axis',(-1.,-1.2303003375722E-16,0.)) ;
#109828=DIRECTION('ref_axis',(1.2303003375722E-16,-1.,0.)) ;
#109829=DIRECTION('',(0.,0.,1.)) ;
#109830=DIRECTION('center_axis',(-1.,-1.2303003375722E-16,0.)) ;
#109831=DIRECTION('ref_axis',(1.2303003375722E-16,-1.,0.)) ;
#109832=DIRECTION('',(1.2303003375722E-16,-1.,1.020425574104E-16)) ;
#109833=DIRECTION('',(-1.2303003375722E-16,1.,-5.10212787052002E-17)) ;
#109834=DIRECTION('center_axis',(-1.,-1.2303003375722E-16,0.)) ;
#109835=DIRECTION('ref_axis',(1.2303003375722E-16,-1.,0.)) ;
#109836=DIRECTION('',(0.,0.,1.)) ;
#109837=DIRECTION('center_axis',(-1.,-1.2303003375722E-16,0.)) ;
#109838=DIRECTION('ref_axis',(1.2303003375722E-16,-1.,0.)) ;
#109839=DIRECTION('',(1.2303003375722E-16,-1.,1.020425574104E-16)) ;
#109840=DIRECTION('',(-1.2303003375722E-16,1.,-5.10212787052002E-17)) ;
#109841=DIRECTION('center_axis',(-1.,-1.2303003375722E-16,0.)) ;
#109842=DIRECTION('ref_axis',(1.2303003375722E-16,-1.,0.)) ;
#109843=DIRECTION('',(0.,0.,1.)) ;
#109844=DIRECTION('center_axis',(-1.,-1.2303003375722E-16,0.)) ;
#109845=DIRECTION('ref_axis',(1.2303003375722E-16,-1.,0.)) ;
#109846=DIRECTION('',(1.2303003375722E-16,-1.,1.020425574104E-16)) ;
#109847=DIRECTION('',(-1.2303003375722E-16,1.,-5.10212787052002E-17)) ;
#109848=DIRECTION('center_axis',(-1.,-1.2303003375722E-16,0.)) ;
#109849=DIRECTION('ref_axis',(1.2303003375722E-16,-1.,0.)) ;
#109850=DIRECTION('',(0.,0.,1.)) ;
#109851=DIRECTION('center_axis',(-1.,-1.2303003375722E-16,0.)) ;
#109852=DIRECTION('ref_axis',(1.2303003375722E-16,-1.,0.)) ;
#109853=DIRECTION('',(1.2303003375722E-16,-1.,1.020425574104E-16)) ;
#109854=DIRECTION('',(-1.2303003375722E-16,1.,-5.10212787052002E-17)) ;
#109855=DIRECTION('center_axis',(-1.,-1.2303003375722E-16,0.)) ;
#109856=DIRECTION('ref_axis',(1.2303003375722E-16,-1.,0.)) ;
#109857=DIRECTION('',(0.,0.,1.)) ;
#109858=DIRECTION('center_axis',(-1.,-1.2303003375722E-16,0.)) ;
#109859=DIRECTION('ref_axis',(1.2303003375722E-16,-1.,0.)) ;
#109860=DIRECTION('',(1.2303003375722E-16,-1.,1.020425574104E-16)) ;
#109861=DIRECTION('',(-1.2303003375722E-16,1.,0.)) ;
#109862=DIRECTION('',(0.,0.,1.)) ;
#109863=DIRECTION('',(1.2303003375722E-16,-1.,0.)) ;
#109864=DIRECTION('',(-1.2303003375722E-16,1.,-5.10212787052002E-17)) ;
#109865=DIRECTION('center_axis',(-1.,-1.2303003375722E-16,0.)) ;
#109866=DIRECTION('ref_axis',(1.2303003375722E-16,-1.,0.)) ;
#109867=DIRECTION('',(0.,0.,1.)) ;
#109868=DIRECTION('center_axis',(0.,0.,1.)) ;
#109869=DIRECTION('ref_axis',(1.,0.,0.)) ;
#109870=DIRECTION('',(0.,0.,1.)) ;
#109871=DIRECTION('center_axis',(0.,0.,1.)) ;
#109872=DIRECTION('ref_axis',(1.,0.,0.)) ;
#109873=DIRECTION('center_axis',(0.,0.,-1.)) ;
#109874=DIRECTION('ref_axis',(1.,0.,0.)) ;
#109875=DIRECTION('center_axis',(-1.59148942750166E-16,1.,0.)) ;
#109876=DIRECTION('ref_axis',(-1.,-1.59148942750166E-16,0.)) ;
#109877=DIRECTION('',(0.,0.,1.)) ;
#109878=DIRECTION('',(-1.,-1.59148942750166E-16,0.)) ;
#109879=DIRECTION('',(1.,1.59148942750166E-16,0.)) ;
#109880=DIRECTION('center_axis',(0.,0.,1.)) ;
#109881=DIRECTION('ref_axis',(1.,0.,0.)) ;
#109882=DIRECTION('',(0.,0.,1.)) ;
#109883=DIRECTION('center_axis',(0.,0.,-1.)) ;
#109884=DIRECTION('ref_axis',(1.,0.,0.)) ;
#109885=DIRECTION('center_axis',(0.,0.,1.)) ;
#109886=DIRECTION('ref_axis',(1.,0.,0.)) ;
#109887=DIRECTION('center_axis',(-1.,0.,0.)) ;
#109888=DIRECTION('ref_axis',(0.,0.,1.)) ;
#109889=DIRECTION('',(0.,0.,1.)) ;
#109890=DIRECTION('',(0.,-1.,0.)) ;
#109891=DIRECTION('',(0.,1.,0.)) ;
#109892=DIRECTION('center_axis',(0.,0.,1.)) ;
#109893=DIRECTION('ref_axis',(1.,0.,0.)) ;
#109894=DIRECTION('',(0.,0.,1.)) ;
#109895=DIRECTION('center_axis',(0.,0.,1.)) ;
#109896=DIRECTION('ref_axis',(1.,0.,0.)) ;
#109897=DIRECTION('center_axis',(0.,0.,-1.)) ;
#109898=DIRECTION('ref_axis',(1.,0.,0.)) ;
#109899=DIRECTION('center_axis',(0.,1.,0.)) ;
#109900=DIRECTION('ref_axis',(0.,0.,1.)) ;
#109901=DIRECTION('',(0.,0.,1.)) ;
#109902=DIRECTION('',(-1.,0.,0.)) ;
#109903=DIRECTION('',(1.,0.,0.)) ;
#109904=DIRECTION('center_axis',(0.,0.,1.)) ;
#109905=DIRECTION('ref_axis',(1.,0.,0.)) ;
#109906=DIRECTION('',(0.,0.,1.)) ;
#109907=DIRECTION('center_axis',(0.,0.,1.)) ;
#109908=DIRECTION('ref_axis',(1.,0.,0.)) ;
#109909=DIRECTION('center_axis',(0.,0.,-1.)) ;
#109910=DIRECTION('ref_axis',(1.,0.,0.)) ;
#109911=DIRECTION('center_axis',(1.,-4.33680868994203E-15,0.)) ;
#109912=DIRECTION('ref_axis',(4.33680868994203E-15,1.,0.)) ;
#109913=DIRECTION('',(0.,0.,1.)) ;
#109914=DIRECTION('',(4.33680868994203E-15,1.,0.)) ;
#109915=DIRECTION('',(-4.33680868994203E-15,-1.,0.)) ;
#109916=DIRECTION('center_axis',(0.,0.,1.)) ;
#109917=DIRECTION('ref_axis',(1.,0.,0.)) ;
#109918=DIRECTION('',(0.,0.,1.)) ;
#109919=DIRECTION('center_axis',(0.,0.,-1.)) ;
#109920=DIRECTION('ref_axis',(1.,0.,0.)) ;
#109921=DIRECTION('center_axis',(0.,0.,1.)) ;
#109922=DIRECTION('ref_axis',(1.,0.,0.)) ;
#109923=DIRECTION('center_axis',(5.88041856263325E-16,1.,0.)) ;
#109924=DIRECTION('ref_axis',(-1.,5.88041856263325E-16,0.)) ;
#109925=DIRECTION('',(0.,0.,1.)) ;
#109926=DIRECTION('',(-1.,5.88041856263325E-16,0.)) ;
#109927=DIRECTION('',(1.,-5.88041856263325E-16,0.)) ;
#109928=DIRECTION('center_axis',(0.,0.,1.)) ;
#109929=DIRECTION('ref_axis',(1.,0.,0.)) ;
#109930=DIRECTION('',(0.,0.,1.)) ;
#109931=DIRECTION('center_axis',(0.,0.,1.)) ;
#109932=DIRECTION('ref_axis',(1.,0.,0.)) ;
#109933=DIRECTION('center_axis',(0.,0.,-1.)) ;
#109934=DIRECTION('ref_axis',(1.,0.,0.)) ;
#109935=DIRECTION('center_axis',(1.,0.,0.)) ;
#109936=DIRECTION('ref_axis',(0.,0.,-1.)) ;
#109937=DIRECTION('',(0.,1.,0.)) ;
#109938=DIRECTION('',(0.,-1.,0.)) ;
#109939=DIRECTION('center_axis',(-1.,0.,0.)) ;
#109940=DIRECTION('ref_axis',(0.,0.,-1.)) ;
#109941=DIRECTION('',(0.,0.,-1.)) ;
#109942=DIRECTION('',(0.,1.,0.)) ;
#109943=DIRECTION('',(0.,3.99416362155027E-15,1.)) ;
#109944=DIRECTION('center_axis',(-1.,0.,0.)) ;
#109945=DIRECTION('ref_axis',(0.,6.50521303491307E-15,-1.)) ;
#109946=DIRECTION('',(0.,0.707106781186546,0.707106781186549)) ;
#109947=DIRECTION('center_axis',(-1.,0.,0.)) ;
#109948=DIRECTION('ref_axis',(0.,-1.51788304147972E-14,-1.)) ;
#109949=DIRECTION('',(0.,0.,-1.)) ;
#109950=DIRECTION('',(0.,-0.707106781186548,0.707106781186547)) ;
#109951=DIRECTION('center_axis',(-1.,0.,0.)) ;
#109952=DIRECTION('ref_axis',(0.,1.30104260698261E-14,-1.)) ;
#109953=DIRECTION('',(0.,0.,1.)) ;
#109954=DIRECTION('',(0.,-1.,0.)) ;
#109955=DIRECTION('',(0.,0.,-1.)) ;
#109956=DIRECTION('center_axis',(-1.,0.,0.)) ;
#109957=DIRECTION('ref_axis',(0.,1.19262238973406E-14,-1.)) ;
#109958=DIRECTION('',(0.,-1.,-1.07081696047951E-16)) ;
#109959=DIRECTION('center_axis',(-1.,0.,0.)) ;
#109960=DIRECTION('ref_axis',(0.,0.,-1.)) ;
#109961=DIRECTION('',(0.,0.,1.)) ;
#109962=DIRECTION('center_axis',(-1.,0.,0.)) ;
#109963=DIRECTION('ref_axis',(0.,4.33680868994204E-15,-1.)) ;
#109964=DIRECTION('center_axis',(1.,0.,0.)) ;
#109965=DIRECTION('ref_axis',(0.,0.,-1.)) ;
#109966=DIRECTION('center_axis',(-1.,0.,0.)) ;
#109967=DIRECTION('ref_axis',(0.,8.67361737988409E-15,-1.)) ;
#109968=DIRECTION('',(0.,0.,1.)) ;
#109969=DIRECTION('center_axis',(-1.,0.,0.)) ;
#109970=DIRECTION('ref_axis',(0.,0.,-1.)) ;
#109971=DIRECTION('',(0.,1.,1.07081696047951E-16)) ;
#109972=DIRECTION('center_axis',(-1.,0.,0.)) ;
#109973=DIRECTION('ref_axis',(0.,0.,-1.)) ;
#109974=DIRECTION('',(0.,0.,-1.)) ;
#109975=DIRECTION('',(0.,1.,0.)) ;
#109976=DIRECTION('',(0.,3.99416362155027E-15,1.)) ;
#109977=DIRECTION('center_axis',(-1.,0.,0.)) ;
#109978=DIRECTION('ref_axis',(0.,6.50521303491307E-15,-1.)) ;
#109979=DIRECTION('',(0.,0.707106781186546,0.707106781186549)) ;
#109980=DIRECTION('center_axis',(-1.,0.,0.)) ;
#109981=DIRECTION('ref_axis',(0.,0.,-1.)) ;
#109982=DIRECTION('',(0.,0.,-1.)) ;
#109983=DIRECTION('',(0.,-0.707106781186548,0.707106781186547)) ;
#109984=DIRECTION('center_axis',(-1.,0.,0.)) ;
#109985=DIRECTION('ref_axis',(0.,1.30104260698261E-14,-1.)) ;
#109986=DIRECTION('',(0.,0.,1.)) ;
#109987=DIRECTION('',(0.,-1.,0.)) ;
#109988=DIRECTION('',(0.,0.,-1.)) ;
#109989=DIRECTION('center_axis',(-1.,0.,0.)) ;
#109990=DIRECTION('ref_axis',(0.,1.08420217248551E-14,-1.)) ;
#109991=DIRECTION('',(0.,-1.,-1.07081696047951E-16)) ;
#109992=DIRECTION('center_axis',(-1.,0.,0.)) ;
#109993=DIRECTION('ref_axis',(0.,0.,-1.)) ;
#109994=DIRECTION('',(0.,0.,1.)) ;
#109995=DIRECTION('center_axis',(-1.,0.,0.)) ;
#109996=DIRECTION('ref_axis',(0.,4.33680868994204E-15,-1.)) ;
#109997=DIRECTION('center_axis',(1.,0.,0.)) ;
#109998=DIRECTION('ref_axis',(0.,0.,-1.)) ;
#109999=DIRECTION('center_axis',(-1.,0.,0.)) ;
#110000=DIRECTION('ref_axis',(0.,-2.16840434497102E-15,-1.)) ;
#110001=DIRECTION('',(0.,0.,1.)) ;
#110002=DIRECTION('center_axis',(-1.,0.,0.)) ;
#110003=DIRECTION('ref_axis',(0.,0.,-1.)) ;
#110004=DIRECTION('',(0.,1.,1.07081696047951E-16)) ;
#110005=DIRECTION('center_axis',(-1.,0.,0.)) ;
#110006=DIRECTION('ref_axis',(0.,0.,-1.)) ;
#110007=DIRECTION('',(0.,0.,-1.)) ;
#110008=DIRECTION('',(0.,1.,0.)) ;
#110009=DIRECTION('',(0.,3.99416362155027E-15,1.)) ;
#110010=DIRECTION('center_axis',(-1.,0.,0.)) ;
#110011=DIRECTION('ref_axis',(0.,6.50521303491307E-15,-1.)) ;
#110012=DIRECTION('',(0.,0.707106781186546,0.707106781186549)) ;
#110013=DIRECTION('center_axis',(-1.,0.,0.)) ;
#110014=DIRECTION('ref_axis',(0.,0.,-1.)) ;
#110015=DIRECTION('',(0.,0.,-1.)) ;
#110016=DIRECTION('',(0.,-0.707106781186548,0.707106781186547)) ;
#110017=DIRECTION('center_axis',(-1.,0.,0.)) ;
#110018=DIRECTION('ref_axis',(0.,0.,-1.)) ;
#110019=DIRECTION('',(0.,0.,1.)) ;
#110020=DIRECTION('',(0.,-1.,0.)) ;
#110021=DIRECTION('',(0.,0.,-1.)) ;
#110022=DIRECTION('center_axis',(-1.,0.,0.)) ;
#110023=DIRECTION('ref_axis',(0.,1.08420217248551E-14,-1.)) ;
#110024=DIRECTION('',(0.,-1.,-1.07081696047951E-16)) ;
#110025=DIRECTION('center_axis',(-1.,0.,0.)) ;
#110026=DIRECTION('ref_axis',(0.,0.,-1.)) ;
#110027=DIRECTION('',(0.,0.,1.)) ;
#110028=DIRECTION('center_axis',(-1.,0.,0.)) ;
#110029=DIRECTION('ref_axis',(0.,0.,-1.)) ;
#110030=DIRECTION('center_axis',(1.,0.,0.)) ;
#110031=DIRECTION('ref_axis',(0.,0.,-1.)) ;
#110032=DIRECTION('center_axis',(-1.,0.,0.)) ;
#110033=DIRECTION('ref_axis',(0.,-2.16840434497102E-15,-1.)) ;
#110034=DIRECTION('',(0.,0.,1.)) ;
#110035=DIRECTION('center_axis',(-1.,0.,0.)) ;
#110036=DIRECTION('ref_axis',(0.,0.,-1.)) ;
#110037=DIRECTION('',(0.,1.,1.07081696047951E-16)) ;
#110038=DIRECTION('center_axis',(-1.,0.,0.)) ;
#110039=DIRECTION('ref_axis',(0.,0.,-1.)) ;
#110040=DIRECTION('',(0.,0.,-1.)) ;
#110041=DIRECTION('',(0.,1.,0.)) ;
#110042=DIRECTION('',(0.,3.99416362155027E-15,1.)) ;
#110043=DIRECTION('center_axis',(-1.,0.,0.)) ;
#110044=DIRECTION('ref_axis',(0.,6.50521303491307E-15,-1.)) ;
#110045=DIRECTION('',(0.,0.707106781186546,0.707106781186549)) ;
#110046=DIRECTION('center_axis',(-1.,0.,0.)) ;
#110047=DIRECTION('ref_axis',(0.,0.,-1.)) ;
#110048=DIRECTION('',(0.,0.,-1.)) ;
#110049=DIRECTION('',(0.,-0.707106781186548,0.707106781186547)) ;
#110050=DIRECTION('center_axis',(-1.,0.,0.)) ;
#110051=DIRECTION('ref_axis',(0.,0.,-1.)) ;
#110052=DIRECTION('',(0.,0.,1.)) ;
#110053=DIRECTION('',(0.,-1.,0.)) ;
#110054=DIRECTION('',(0.,0.,-1.)) ;
#110055=DIRECTION('center_axis',(-1.,0.,0.)) ;
#110056=DIRECTION('ref_axis',(0.,1.08420217248551E-14,-1.)) ;
#110057=DIRECTION('',(0.,-1.,-1.07081696047951E-16)) ;
#110058=DIRECTION('center_axis',(-1.,0.,0.)) ;
#110059=DIRECTION('ref_axis',(0.,0.,-1.)) ;
#110060=DIRECTION('',(0.,0.,1.)) ;
#110061=DIRECTION('center_axis',(-1.,0.,0.)) ;
#110062=DIRECTION('ref_axis',(0.,0.,-1.)) ;
#110063=DIRECTION('center_axis',(1.,0.,0.)) ;
#110064=DIRECTION('ref_axis',(0.,0.,-1.)) ;
#110065=DIRECTION('center_axis',(-1.,0.,0.)) ;
#110066=DIRECTION('ref_axis',(0.,-2.16840434497102E-15,-1.)) ;
#110067=DIRECTION('',(0.,0.,1.)) ;
#110068=DIRECTION('center_axis',(-1.,0.,0.)) ;
#110069=DIRECTION('ref_axis',(0.,0.,-1.)) ;
#110070=DIRECTION('',(0.,1.,1.07081696047951E-16)) ;
#110071=DIRECTION('center_axis',(-1.,0.,0.)) ;
#110072=DIRECTION('ref_axis',(0.,0.,-1.)) ;
#110073=DIRECTION('',(0.,0.,-1.)) ;
#110074=DIRECTION('',(0.,1.,0.)) ;
#110075=DIRECTION('',(0.,3.99416362155027E-15,1.)) ;
#110076=DIRECTION('center_axis',(-1.,0.,0.)) ;
#110077=DIRECTION('ref_axis',(0.,6.50521303491307E-15,-1.)) ;
#110078=DIRECTION('',(0.,0.707106781186546,0.707106781186549)) ;
#110079=DIRECTION('center_axis',(-1.,0.,0.)) ;
#110080=DIRECTION('ref_axis',(0.,0.,-1.)) ;
#110081=DIRECTION('',(0.,0.,-1.)) ;
#110082=DIRECTION('',(0.,-0.707106781186548,0.707106781186547)) ;
#110083=DIRECTION('center_axis',(-1.,0.,0.)) ;
#110084=DIRECTION('ref_axis',(0.,0.,-1.)) ;
#110085=DIRECTION('',(0.,0.,1.)) ;
#110086=DIRECTION('',(0.,-1.,0.)) ;
#110087=DIRECTION('',(0.,0.,-1.)) ;
#110088=DIRECTION('center_axis',(-1.,0.,0.)) ;
#110089=DIRECTION('ref_axis',(0.,1.08420217248551E-14,-1.)) ;
#110090=DIRECTION('',(0.,-1.,-1.07081696047951E-16)) ;
#110091=DIRECTION('center_axis',(-1.,0.,0.)) ;
#110092=DIRECTION('ref_axis',(0.,0.,-1.)) ;
#110093=DIRECTION('',(0.,0.,1.)) ;
#110094=DIRECTION('center_axis',(-1.,0.,0.)) ;
#110095=DIRECTION('ref_axis',(0.,0.,-1.)) ;
#110096=DIRECTION('center_axis',(1.,0.,0.)) ;
#110097=DIRECTION('ref_axis',(0.,0.,-1.)) ;
#110098=DIRECTION('center_axis',(-1.,0.,0.)) ;
#110099=DIRECTION('ref_axis',(0.,-2.16840434497102E-15,-1.)) ;
#110100=DIRECTION('',(0.,0.,1.)) ;
#110101=DIRECTION('center_axis',(-1.,0.,0.)) ;
#110102=DIRECTION('ref_axis',(0.,0.,-1.)) ;
#110103=DIRECTION('',(0.,1.,1.07081696047951E-16)) ;
#110104=DIRECTION('center_axis',(-1.,0.,0.)) ;
#110105=DIRECTION('ref_axis',(0.,0.,-1.)) ;
#110106=DIRECTION('',(0.,0.,-1.)) ;
#110107=DIRECTION('',(0.,1.,0.)) ;
#110108=DIRECTION('',(0.,3.99416362155027E-15,1.)) ;
#110109=DIRECTION('center_axis',(-1.,0.,0.)) ;
#110110=DIRECTION('ref_axis',(0.,2.16840434497102E-15,-1.)) ;
#110111=DIRECTION('',(0.,0.707106781186546,0.707106781186549)) ;
#110112=DIRECTION('center_axis',(-1.,0.,0.)) ;
#110113=DIRECTION('ref_axis',(0.,0.,-1.)) ;
#110114=DIRECTION('',(0.,0.,-1.)) ;
#110115=DIRECTION('',(0.,-0.707106781186548,0.707106781186547)) ;
#110116=DIRECTION('center_axis',(-1.,0.,0.)) ;
#110117=DIRECTION('ref_axis',(0.,0.,-1.)) ;
#110118=DIRECTION('',(0.,0.,1.)) ;
#110119=DIRECTION('',(0.,-1.,0.)) ;
#110120=DIRECTION('',(0.,0.,-1.)) ;
#110121=DIRECTION('center_axis',(-1.,0.,0.)) ;
#110122=DIRECTION('ref_axis',(0.,1.08420217248551E-14,-1.)) ;
#110123=DIRECTION('',(0.,-1.,-1.07081696047951E-16)) ;
#110124=DIRECTION('center_axis',(-1.,0.,0.)) ;
#110125=DIRECTION('ref_axis',(0.,0.,-1.)) ;
#110126=DIRECTION('',(0.,0.,1.)) ;
#110127=DIRECTION('center_axis',(-1.,0.,0.)) ;
#110128=DIRECTION('ref_axis',(0.,0.,-1.)) ;
#110129=DIRECTION('center_axis',(1.,0.,0.)) ;
#110130=DIRECTION('ref_axis',(0.,0.,-1.)) ;
#110131=DIRECTION('center_axis',(-1.,0.,0.)) ;
#110132=DIRECTION('ref_axis',(0.,-2.168404344971E-15,-1.)) ;
#110133=DIRECTION('',(0.,0.,1.)) ;
#110134=DIRECTION('center_axis',(-1.,0.,0.)) ;
#110135=DIRECTION('ref_axis',(0.,0.,-1.)) ;
#110136=DIRECTION('',(0.,1.,1.07081696047951E-16)) ;
#110137=DIRECTION('center_axis',(-1.,0.,0.)) ;
#110138=DIRECTION('ref_axis',(0.,0.,-1.)) ;
#110139=DIRECTION('',(0.,0.,-1.)) ;
#110140=DIRECTION('',(0.,1.,0.)) ;
#110141=DIRECTION('',(0.,3.99416362155027E-15,1.)) ;
#110142=DIRECTION('center_axis',(-1.,0.,0.)) ;
#110143=DIRECTION('ref_axis',(0.,2.16840434497102E-15,-1.)) ;
#110144=DIRECTION('',(0.,0.707106781186546,0.707106781186549)) ;
#110145=DIRECTION('center_axis',(-1.,0.,0.)) ;
#110146=DIRECTION('ref_axis',(0.,0.,-1.)) ;
#110147=DIRECTION('',(0.,0.,-1.)) ;
#110148=DIRECTION('',(0.,-0.707106781186548,0.707106781186547)) ;
#110149=DIRECTION('center_axis',(-1.,0.,0.)) ;
#110150=DIRECTION('ref_axis',(0.,0.,-1.)) ;
#110151=DIRECTION('',(0.,0.,1.)) ;
#110152=DIRECTION('',(0.,-1.,0.)) ;
#110153=DIRECTION('',(0.,0.,-1.)) ;
#110154=DIRECTION('center_axis',(-1.,0.,0.)) ;
#110155=DIRECTION('ref_axis',(0.,1.0842021724855E-14,-1.)) ;
#110156=DIRECTION('',(0.,-1.,-1.07081696047951E-16)) ;
#110157=DIRECTION('center_axis',(-1.,0.,0.)) ;
#110158=DIRECTION('ref_axis',(0.,0.,-1.)) ;
#110159=DIRECTION('',(0.,0.,1.)) ;
#110160=DIRECTION('center_axis',(-1.,0.,0.)) ;
#110161=DIRECTION('ref_axis',(0.,-2.168404344971E-15,-1.)) ;
#110162=DIRECTION('center_axis',(1.,0.,0.)) ;
#110163=DIRECTION('ref_axis',(0.,0.,-1.)) ;
#110164=DIRECTION('center_axis',(-1.,0.,0.)) ;
#110165=DIRECTION('ref_axis',(0.,-2.168404344971E-15,-1.)) ;
#110166=DIRECTION('',(0.,0.,1.)) ;
#110167=DIRECTION('center_axis',(-1.,0.,0.)) ;
#110168=DIRECTION('ref_axis',(0.,0.,-1.)) ;
#110169=DIRECTION('',(0.,1.,1.07081696047951E-16)) ;
#110170=DIRECTION('center_axis',(-1.,0.,0.)) ;
#110171=DIRECTION('ref_axis',(0.,0.,-1.)) ;
#110172=DIRECTION('',(0.,0.,-1.)) ;
#110173=DIRECTION('',(0.,1.,0.)) ;
#110174=DIRECTION('',(0.,3.99416362155027E-15,1.)) ;
#110175=DIRECTION('center_axis',(-1.,0.,0.)) ;
#110176=DIRECTION('ref_axis',(0.,0.,-1.)) ;
#110177=DIRECTION('',(0.,0.707106781186546,0.707106781186549)) ;
#110178=DIRECTION('center_axis',(-1.,0.,0.)) ;
#110179=DIRECTION('ref_axis',(0.,0.,-1.)) ;
#110180=DIRECTION('',(0.,0.,-1.)) ;
#110181=DIRECTION('',(0.,-0.707106781186548,0.707106781186547)) ;
#110182=DIRECTION('center_axis',(-1.,0.,0.)) ;
#110183=DIRECTION('ref_axis',(0.,0.,-1.)) ;
#110184=DIRECTION('',(0.,0.,1.)) ;
#110185=DIRECTION('',(0.,-1.,0.)) ;
#110186=DIRECTION('',(0.,0.,-1.)) ;
#110187=DIRECTION('center_axis',(-1.,0.,0.)) ;
#110188=DIRECTION('ref_axis',(0.,1.0842021724855E-14,-1.)) ;
#110189=DIRECTION('',(0.,-1.,-1.07081696047951E-16)) ;
#110190=DIRECTION('center_axis',(-1.,0.,0.)) ;
#110191=DIRECTION('ref_axis',(0.,0.,-1.)) ;
#110192=DIRECTION('',(0.,0.,1.)) ;
#110193=DIRECTION('center_axis',(-1.,0.,0.)) ;
#110194=DIRECTION('ref_axis',(0.,-2.168404344971E-15,-1.)) ;
#110195=DIRECTION('center_axis',(1.,0.,0.)) ;
#110196=DIRECTION('ref_axis',(0.,0.,-1.)) ;
#110197=DIRECTION('center_axis',(-1.,0.,0.)) ;
#110198=DIRECTION('ref_axis',(0.,0.,-1.)) ;
#110199=DIRECTION('',(0.,0.,1.)) ;
#110200=DIRECTION('center_axis',(-1.,0.,0.)) ;
#110201=DIRECTION('ref_axis',(0.,0.,-1.)) ;
#110202=DIRECTION('',(0.,1.,1.07081696047951E-16)) ;
#110203=DIRECTION('center_axis',(-1.,0.,0.)) ;
#110204=DIRECTION('ref_axis',(0.,0.,-1.)) ;
#110205=DIRECTION('',(0.,0.,-1.)) ;
#110206=DIRECTION('',(0.,1.,0.)) ;
#110207=DIRECTION('',(0.,3.99416362155027E-15,1.)) ;
#110208=DIRECTION('center_axis',(-1.,0.,0.)) ;
#110209=DIRECTION('ref_axis',(0.,0.,-1.)) ;
#110210=DIRECTION('',(0.,0.707106781186546,0.707106781186549)) ;
#110211=DIRECTION('center_axis',(-1.,0.,0.)) ;
#110212=DIRECTION('ref_axis',(0.,0.,-1.)) ;
#110213=DIRECTION('',(0.,0.,-1.)) ;
#110214=DIRECTION('',(0.,-0.707106781186548,0.707106781186547)) ;
#110215=DIRECTION('center_axis',(-1.,0.,0.)) ;
#110216=DIRECTION('ref_axis',(0.,0.,-1.)) ;
#110217=DIRECTION('',(0.,0.,1.)) ;
#110218=DIRECTION('',(0.,-1.,0.)) ;
#110219=DIRECTION('',(0.,0.,-1.)) ;
#110220=DIRECTION('center_axis',(-1.,0.,0.)) ;
#110221=DIRECTION('ref_axis',(0.,9.75781955236956E-15,-1.)) ;
#110222=DIRECTION('',(0.,-1.,-1.07081696047951E-16)) ;
#110223=DIRECTION('center_axis',(-1.,0.,0.)) ;
#110224=DIRECTION('ref_axis',(0.,0.,-1.)) ;
#110225=DIRECTION('',(0.,0.,1.)) ;
#110226=DIRECTION('center_axis',(-1.,0.,0.)) ;
#110227=DIRECTION('ref_axis',(0.,-2.16840434497101E-15,-1.)) ;
#110228=DIRECTION('center_axis',(1.,0.,0.)) ;
#110229=DIRECTION('ref_axis',(0.,0.,-1.)) ;
#110230=DIRECTION('center_axis',(-1.,0.,0.)) ;
#110231=DIRECTION('ref_axis',(0.,0.,-1.)) ;
#110232=DIRECTION('',(0.,0.,1.)) ;
#110233=DIRECTION('center_axis',(-1.,0.,0.)) ;
#110234=DIRECTION('ref_axis',(0.,0.,-1.)) ;
#110235=DIRECTION('',(0.,1.,1.07081696047951E-16)) ;
#110236=DIRECTION('center_axis',(-1.,0.,0.)) ;
#110237=DIRECTION('ref_axis',(0.,-1.0842021724855E-15,-1.)) ;
#110238=DIRECTION('',(0.,0.,-1.)) ;
#110239=DIRECTION('',(0.,1.,0.)) ;
#110240=DIRECTION('',(0.,3.99416362155027E-15,1.)) ;
#110241=DIRECTION('center_axis',(-1.,0.,0.)) ;
#110242=DIRECTION('ref_axis',(0.,2.16840434497101E-15,-1.)) ;
#110243=DIRECTION('',(0.,0.707106781186546,0.707106781186549)) ;
#110244=DIRECTION('center_axis',(-1.,0.,0.)) ;
#110245=DIRECTION('ref_axis',(0.,0.,-1.)) ;
#110246=DIRECTION('',(0.,0.,-1.)) ;
#110247=DIRECTION('',(0.,-0.707106781186548,0.707106781186547)) ;
#110248=DIRECTION('center_axis',(-1.,0.,0.)) ;
#110249=DIRECTION('ref_axis',(0.,0.,-1.)) ;
#110250=DIRECTION('',(0.,0.,1.)) ;
#110251=DIRECTION('',(0.,-1.,0.)) ;
#110252=DIRECTION('',(0.,0.,-1.)) ;
#110253=DIRECTION('center_axis',(-1.,0.,0.)) ;
#110254=DIRECTION('ref_axis',(0.,8.67361737988403E-15,-1.)) ;
#110255=DIRECTION('',(0.,-1.,-1.07081696047951E-16)) ;
#110256=DIRECTION('center_axis',(-1.,0.,0.)) ;
#110257=DIRECTION('ref_axis',(0.,0.,-1.)) ;
#110258=DIRECTION('',(0.,0.,1.)) ;
#110259=DIRECTION('center_axis',(-1.,0.,0.)) ;
#110260=DIRECTION('ref_axis',(0.,2.16840434497101E-15,-1.)) ;
#110261=DIRECTION('center_axis',(1.,0.,0.)) ;
#110262=DIRECTION('ref_axis',(0.,0.,-1.)) ;
#110263=DIRECTION('center_axis',(-1.,0.,0.)) ;
#110264=DIRECTION('ref_axis',(0.,0.,-1.)) ;
#110265=DIRECTION('',(0.,0.,1.)) ;
#110266=DIRECTION('center_axis',(-1.,0.,0.)) ;
#110267=DIRECTION('ref_axis',(0.,0.,-1.)) ;
#110268=DIRECTION('',(0.,1.,1.07081696047951E-16)) ;
#110269=DIRECTION('center_axis',(0.,0.,1.)) ;
#110270=DIRECTION('ref_axis',(1.,0.,0.)) ;
#110271=DIRECTION('',(0.,-1.,0.)) ;
#110272=DIRECTION('',(-1.,0.,0.)) ;
#110273=DIRECTION('',(-1.2303003375722E-16,1.,0.)) ;
#110274=DIRECTION('',(1.,1.59148942750166E-16,0.)) ;
#110275=DIRECTION('center_axis',(0.,0.,1.)) ;
#110276=DIRECTION('ref_axis',(1.,0.,0.)) ;
#110277=DIRECTION('',(0.,1.,0.)) ;
#110278=DIRECTION('',(1.,0.,0.)) ;
#110279=DIRECTION('',(-4.33680868994203E-15,-1.,0.)) ;
#110280=DIRECTION('center_axis',(0.,0.,1.)) ;
#110281=DIRECTION('ref_axis',(1.,0.,0.)) ;
#110282=DIRECTION('',(1.,-5.88041856263325E-16,0.)) ;
#110283=DIRECTION('center_axis',(0.,0.,1.)) ;
#110284=DIRECTION('ref_axis',(1.,0.,0.)) ;
#110285=DIRECTION('',(1.2303003375722E-16,-1.,0.)) ;
#110286=DIRECTION('',(1.,0.,0.)) ;
#110287=DIRECTION('',(0.,1.,0.)) ;
#110288=DIRECTION('',(-1.,5.88041856263325E-16,0.)) ;
#110289=DIRECTION('center_axis',(0.,0.,-1.)) ;
#110290=DIRECTION('ref_axis',(1.,0.,0.)) ;
#110291=DIRECTION('',(4.33680868994203E-15,1.,0.)) ;
#110292=DIRECTION('',(-1.,0.,0.)) ;
#110293=DIRECTION('',(0.,-1.,0.)) ;
#110294=DIRECTION('center_axis',(0.,0.,-1.)) ;
#110295=DIRECTION('ref_axis',(1.,0.,0.)) ;
#110296=DIRECTION('',(-1.,-1.59148942750166E-16,0.)) ;
#110297=DIRECTION('center_axis',(-1.,-1.53063836115601E-16,0.)) ;
#110298=DIRECTION('ref_axis',(1.53063836115601E-16,-1.,0.)) ;
#110299=DIRECTION('',(0.,0.,1.)) ;
#110300=DIRECTION('',(-1.53063836115601E-16,1.,-1.020425574104E-16)) ;
#110301=DIRECTION('',(0.,0.,-1.)) ;
#110302=DIRECTION('',(1.53063836115601E-16,-1.,5.10212787052002E-17)) ;
#110303=DIRECTION('',(0.,0.,1.)) ;
#110304=DIRECTION('',(-1.53063836115601E-16,1.,-1.30104260698261E-16)) ;
#110305=DIRECTION('center_axis',(-1.,-1.53063836115601E-16,0.)) ;
#110306=DIRECTION('ref_axis',(1.53063836115601E-16,-1.,0.)) ;
#110307=DIRECTION('',(0.,0.,1.)) ;
#110308=DIRECTION('center_axis',(-1.,-1.53063836115601E-16,0.)) ;
#110309=DIRECTION('ref_axis',(1.53063836115601E-16,-1.,0.)) ;
#110310=DIRECTION('',(1.53063836115601E-16,-1.,-1.30104260698261E-16)) ;
#110311=DIRECTION('center_axis',(-1.53063836115601E-16,1.,0.)) ;
#110312=DIRECTION('ref_axis',(-1.,-1.53063836115601E-16,0.)) ;
#110313=DIRECTION('',(-1.,-1.53063836115601E-16,2.73691106313441E-48)) ;
#110314=DIRECTION('',(0.,0.,-1.)) ;
#110315=DIRECTION('',(1.,1.53063836115601E-16,-1.53236300070382E-33)) ;
#110316=DIRECTION('',(0.,0.,1.)) ;
#110317=DIRECTION('center_axis',(1.99142572374599E-32,-1.30104260698261E-16,
-1.)) ;
#110318=DIRECTION('ref_axis',(0.,1.,-1.30104260698261E-16)) ;
#110319=DIRECTION('',(-1.,-1.53063836115601E-16,2.73691106313441E-48)) ;
#110320=DIRECTION('',(1.53063836115601E-16,-1.,1.30104260698261E-16)) ;
#110321=DIRECTION('',(1.,1.53063836115601E-16,-2.73691106313441E-48)) ;
#110322=DIRECTION('center_axis',(-1.53063836115601E-16,1.,0.)) ;
#110323=DIRECTION('ref_axis',(-1.,-1.53063836115601E-16,0.)) ;
#110324=DIRECTION('',(-1.,-1.53063836115601E-16,-2.73691106313441E-48)) ;
#110325=DIRECTION('',(0.,0.,-1.)) ;
#110326=DIRECTION('',(1.,1.53063836115601E-16,-2.73691106313441E-48)) ;
#110327=DIRECTION('',(0.,0.,1.)) ;
#110328=DIRECTION('center_axis',(1.99142572374599E-32,-1.30104260698261E-16,
1.)) ;
#110329=DIRECTION('ref_axis',(0.,-1.,-1.30104260698261E-16)) ;
#110330=DIRECTION('',(-1.,-1.53063836115601E-16,-2.73691106313441E-48)) ;
#110331=DIRECTION('',(-1.53063836115601E-16,1.,1.30104260698261E-16)) ;
#110332=DIRECTION('',(1.,1.53063836115601E-16,2.73691106313441E-48)) ;
#110333=DIRECTION('',(2.16840434497101E-16,-1.,-1.30104260698261E-16)) ;
#110334=DIRECTION('center_axis',(-1.53063836115601E-16,1.,0.)) ;
#110335=DIRECTION('ref_axis',(-1.,-1.53063836115601E-16,0.)) ;
#110336=DIRECTION('',(-1.,-1.53063836115601E-16,3.06472600140763E-33)) ;
#110337=DIRECTION('',(0.,0.,-1.)) ;
#110338=DIRECTION('',(1.,1.53063836115601E-16,2.73691106313441E-48)) ;
#110339=DIRECTION('',(0.,0.,1.)) ;
#110340=DIRECTION('center_axis',(1.,0.,0.)) ;
#110341=DIRECTION('ref_axis',(0.,0.,-1.)) ;
#110342=DIRECTION('',(1.,0.,0.)) ;
#110343=DIRECTION('center_axis',(1.,0.,0.)) ;
#110344=DIRECTION('ref_axis',(0.,0.,1.)) ;
#110345=DIRECTION('',(1.,0.,0.)) ;
#110346=DIRECTION('center_axis',(-1.,0.,0.)) ;
#110347=DIRECTION('ref_axis',(0.,0.,-1.)) ;
#110348=DIRECTION('center_axis',(0.,0.,1.)) ;
#110349=DIRECTION('ref_axis',(1.,0.,0.)) ;
#110350=DIRECTION('',(0.,1.,0.)) ;
#110351=DIRECTION('',(1.,0.,0.)) ;
#110352=DIRECTION('',(0.,-1.,0.)) ;
#110353=DIRECTION('center_axis',(1.,0.,0.)) ;
#110354=DIRECTION('ref_axis',(0.,0.,-1.)) ;
#110355=DIRECTION('center_axis',(1.,0.,0.)) ;
#110356=DIRECTION('ref_axis',(0.,0.,1.)) ;
#110357=DIRECTION('',(1.,0.,0.)) ;
#110358=DIRECTION('center_axis',(-1.,0.,0.)) ;
#110359=DIRECTION('ref_axis',(0.,0.,-1.)) ;
#110360=DIRECTION('center_axis',(0.,-1.,3.99416362155027E-15)) ;
#110361=DIRECTION('ref_axis',(0.,-3.99416362155027E-15,-1.)) ;
#110362=DIRECTION('',(0.,3.99416362155027E-15,1.)) ;
#110363=DIRECTION('',(1.,0.,0.)) ;
#110364=DIRECTION('',(0.,-3.99416362155027E-15,-1.)) ;
#110365=DIRECTION('center_axis',(1.,0.,0.)) ;
#110366=DIRECTION('ref_axis',(0.,0.,-1.)) ;
#110367=DIRECTION('center_axis',(-1.,0.,0.)) ;
#110368=DIRECTION('ref_axis',(0.,0.,-1.)) ;
#110369=DIRECTION('',(1.,0.,0.)) ;
#110370=DIRECTION('center_axis',(1.,0.,0.)) ;
#110371=DIRECTION('ref_axis',(0.,0.,-1.)) ;
#110372=DIRECTION('center_axis',(0.,-0.707106781186549,0.707106781186546)) ;
#110373=DIRECTION('ref_axis',(0.,-0.707106781186546,-0.707106781186549)) ;
#110374=DIRECTION('',(0.,0.707106781186546,0.707106781186549)) ;
#110375=DIRECTION('',(1.,0.,0.)) ;
#110376=DIRECTION('',(0.,-0.707106781186546,-0.707106781186549)) ;
#110377=DIRECTION('center_axis',(1.,0.,0.)) ;
#110378=DIRECTION('ref_axis',(0.,0.382683432365091,0.923879532511286)) ;
#110379=DIRECTION('',(1.,0.,0.)) ;
#110380=DIRECTION('center_axis',(1.,0.,0.)) ;
#110381=DIRECTION('ref_axis',(0.,0.,-1.)) ;
#110382=DIRECTION('center_axis',(0.,1.,0.)) ;
#110383=DIRECTION('ref_axis',(0.,0.,1.)) ;
#110384=DIRECTION('',(0.,0.,-1.)) ;
#110385=DIRECTION('',(0.,0.,1.)) ;
#110386=DIRECTION('center_axis',(0.,-0.707106781186547,-0.707106781186548)) ;
#110387=DIRECTION('ref_axis',(0.,0.707106781186548,-0.707106781186547)) ;
#110388=DIRECTION('',(0.,-0.707106781186548,0.707106781186547)) ;
#110389=DIRECTION('',(1.,0.,0.)) ;
#110390=DIRECTION('',(0.,0.707106781186548,-0.707106781186547)) ;
#110391=DIRECTION('center_axis',(1.,0.,0.)) ;
#110392=DIRECTION('ref_axis',(0.,0.,-1.)) ;
#110393=DIRECTION('center_axis',(-1.,0.,0.)) ;
#110394=DIRECTION('ref_axis',(0.,0.,-1.)) ;
#110395=DIRECTION('',(1.,0.,0.)) ;
#110396=DIRECTION('center_axis',(1.,0.,0.)) ;
#110397=DIRECTION('ref_axis',(0.,0.,-1.)) ;
#110398=DIRECTION('center_axis',(0.,-1.,0.)) ;
#110399=DIRECTION('ref_axis',(0.,0.,-1.)) ;
#110400=DIRECTION('',(0.,0.,1.)) ;
#110401=DIRECTION('',(1.,0.,0.)) ;
#110402=DIRECTION('',(0.,0.,-1.)) ;
#110403=DIRECTION('center_axis',(1.,0.,0.)) ;
#110404=DIRECTION('ref_axis',(0.,0.,-1.)) ;
#110405=DIRECTION('center_axis',(1.,0.,0.)) ;
#110406=DIRECTION('ref_axis',(0.,0.,1.)) ;
#110407=DIRECTION('',(1.,0.,0.)) ;
#110408=DIRECTION('center_axis',(-1.,0.,0.)) ;
#110409=DIRECTION('ref_axis',(0.,0.,-1.)) ;
#110410=DIRECTION('center_axis',(0.,0.,-1.)) ;
#110411=DIRECTION('ref_axis',(-1.,0.,0.)) ;
#110412=DIRECTION('',(0.,-1.,0.)) ;
#110413=DIRECTION('',(1.,0.,0.)) ;
#110414=DIRECTION('',(0.,1.,0.)) ;
#110415=DIRECTION('center_axis',(1.,0.,0.)) ;
#110416=DIRECTION('ref_axis',(0.,0.,-1.)) ;
#110417=DIRECTION('center_axis',(1.,0.,0.)) ;
#110418=DIRECTION('ref_axis',(0.,0.,1.)) ;
#110419=DIRECTION('',(1.,0.,0.)) ;
#110420=DIRECTION('center_axis',(-1.,0.,0.)) ;
#110421=DIRECTION('ref_axis',(0.,0.,-1.)) ;
#110422=DIRECTION('center_axis',(0.,1.,0.)) ;
#110423=DIRECTION('ref_axis',(0.,0.,1.)) ;
#110424=DIRECTION('',(0.,0.,-1.)) ;
#110425=DIRECTION('',(1.,0.,0.)) ;
#110426=DIRECTION('',(0.,0.,1.)) ;
#110427=DIRECTION('center_axis',(1.,0.,0.)) ;
#110428=DIRECTION('ref_axis',(0.,0.,-1.)) ;
#110429=DIRECTION('center_axis',(-1.,0.,0.)) ;
#110430=DIRECTION('ref_axis',(0.,1.51788304147971E-14,-1.)) ;
#110431=DIRECTION('',(1.,0.,0.)) ;
#110432=DIRECTION('center_axis',(1.,0.,0.)) ;
#110433=DIRECTION('ref_axis',(0.,0.,-1.)) ;
#110434=DIRECTION('center_axis',(0.,1.07081696047951E-16,-1.)) ;
#110435=DIRECTION('ref_axis',(0.,1.,1.07081696047951E-16)) ;
#110436=DIRECTION('',(0.,-1.,-1.07081696047951E-16)) ;
#110437=DIRECTION('',(1.,0.,0.)) ;
#110438=DIRECTION('',(0.,1.,1.07081696047951E-16)) ;
#110439=DIRECTION('center_axis',(1.,0.,0.)) ;
#110440=DIRECTION('ref_axis',(0.,0.,-1.)) ;
#110441=DIRECTION('center_axis',(-1.,0.,0.)) ;
#110442=DIRECTION('ref_axis',(0.,0.,-1.)) ;
#110443=DIRECTION('',(1.,0.,0.)) ;
#110444=DIRECTION('center_axis',(1.,0.,0.)) ;
#110445=DIRECTION('ref_axis',(0.,0.,-1.)) ;
#110446=DIRECTION('center_axis',(0.,-1.,0.)) ;
#110447=DIRECTION('ref_axis',(0.,0.,-1.)) ;
#110448=DIRECTION('',(0.,0.,1.)) ;
#110449=DIRECTION('',(1.,0.,0.)) ;
#110450=DIRECTION('',(0.,0.,-1.)) ;
#110451=DIRECTION('center_axis',(1.,0.,0.)) ;
#110452=DIRECTION('ref_axis',(0.,0.,-1.)) ;
#110453=DIRECTION('center_axis',(-1.,0.,0.)) ;
#110454=DIRECTION('ref_axis',(0.,0.,-1.)) ;
#110455=DIRECTION('',(1.,0.,0.)) ;
#110456=DIRECTION('center_axis',(1.,0.,0.)) ;
#110457=DIRECTION('ref_axis',(0.,0.,-1.)) ;
#110458=DIRECTION('center_axis',(1.,0.,0.)) ;
#110459=DIRECTION('ref_axis',(0.,0.,-1.)) ;
#110460=DIRECTION('center_axis',(1.,0.,0.)) ;
#110461=DIRECTION('ref_axis',(0.,0.,1.)) ;
#110462=DIRECTION('',(1.,0.,0.)) ;
#110463=DIRECTION('center_axis',(-1.,0.,0.)) ;
#110464=DIRECTION('ref_axis',(0.,0.,-1.)) ;
#110465=DIRECTION('center_axis',(1.,0.,0.)) ;
#110466=DIRECTION('ref_axis',(0.,0.,-1.)) ;
#110467=DIRECTION('center_axis',(-1.,0.,0.)) ;
#110468=DIRECTION('ref_axis',(0.,0.,-1.)) ;
#110469=DIRECTION('',(1.,0.,0.)) ;
#110470=DIRECTION('center_axis',(1.,0.,0.)) ;
#110471=DIRECTION('ref_axis',(0.,0.,-1.)) ;
#110472=DIRECTION('center_axis',(0.,-1.,0.)) ;
#110473=DIRECTION('ref_axis',(0.,0.,-1.)) ;
#110474=DIRECTION('',(0.,0.,1.)) ;
#110475=DIRECTION('',(1.,0.,0.)) ;
#110476=DIRECTION('',(0.,0.,-1.)) ;
#110477=DIRECTION('center_axis',(1.,0.,0.)) ;
#110478=DIRECTION('ref_axis',(0.,0.,-1.)) ;
#110479=DIRECTION('center_axis',(-1.,0.,0.)) ;
#110480=DIRECTION('ref_axis',(0.,0.,-1.)) ;
#110481=DIRECTION('',(1.,0.,0.)) ;
#110482=DIRECTION('center_axis',(1.,0.,0.)) ;
#110483=DIRECTION('ref_axis',(0.,0.,-1.)) ;
#110484=DIRECTION('center_axis',(0.,-1.07081696047951E-16,1.)) ;
#110485=DIRECTION('ref_axis',(0.,-1.,-1.07081696047951E-16)) ;
#110486=DIRECTION('',(0.,1.,1.07081696047951E-16)) ;
#110487=DIRECTION('',(1.,0.,0.)) ;
#110488=DIRECTION('',(0.,-1.,-1.07081696047951E-16)) ;
#110489=DIRECTION('center_axis',(1.,0.,0.)) ;
#110490=DIRECTION('ref_axis',(0.,0.,-1.)) ;
#110491=DIRECTION('center_axis',(-1.,0.,0.)) ;
#110492=DIRECTION('ref_axis',(0.,0.,-1.)) ;
#110493=DIRECTION('',(1.,0.,0.)) ;
#110494=DIRECTION('center_axis',(1.,0.,0.)) ;
#110495=DIRECTION('ref_axis',(0.,0.,-1.)) ;
#110496=DIRECTION('center_axis',(0.,1.,0.)) ;
#110497=DIRECTION('ref_axis',(0.,0.,1.)) ;
#110498=DIRECTION('',(0.,0.,-1.)) ;
#110499=DIRECTION('',(0.,0.,1.)) ;
#110500=DIRECTION('center_axis',(-1.,0.,0.)) ;
#110501=DIRECTION('ref_axis',(0.,0.,1.)) ;
#110502=DIRECTION('center_axis',(-1.,0.,0.)) ;
#110503=DIRECTION('ref_axis',(0.,0.,1.)) ;
#110504=DIRECTION('',(0.,-1.,0.)) ;
#110505=DIRECTION('center_axis',(-1.,0.,0.)) ;
#110506=DIRECTION('ref_axis',(0.,0.,1.)) ;
#110507=DIRECTION('',(0.,0.,1.)) ;
#110508=DIRECTION('',(0.,-1.,-1.07081696047951E-16)) ;
#110509=DIRECTION('',(0.,0.,-1.)) ;
#110510=DIRECTION('center_axis',(-1.,0.,0.)) ;
#110511=DIRECTION('ref_axis',(0.,0.,1.)) ;
#110512=DIRECTION('',(0.,0.,-1.)) ;
#110513=DIRECTION('',(0.,1.,1.07081696047951E-16)) ;
#110514=DIRECTION('',(0.,0.,1.)) ;
#110515=DIRECTION('center_axis',(-1.,0.,0.)) ;
#110516=DIRECTION('ref_axis',(0.,0.,1.)) ;
#110517=DIRECTION('',(0.,1.,0.)) ;
#110518=DIRECTION('center_axis',(-1.,0.,0.)) ;
#110519=DIRECTION('ref_axis',(0.,0.,1.)) ;
#110520=DIRECTION('',(0.,0.,-1.)) ;
#110521=DIRECTION('',(0.,0.707106781186548,-0.707106781186547)) ;
#110522=DIRECTION('',(0.,0.,1.)) ;
#110523=DIRECTION('',(0.,-0.707106781186546,-0.707106781186549)) ;
#110524=DIRECTION('',(0.,-3.99416362155027E-15,-1.)) ;
#110525=DIRECTION('center_axis',(1.,0.,0.)) ;
#110526=DIRECTION('ref_axis',(0.,0.,-1.)) ;
#110527=DIRECTION('',(0.,-1.,0.)) ;
#110528=DIRECTION('center_axis',(-1.,0.,0.)) ;
#110529=DIRECTION('ref_axis',(0.,0.,-1.)) ;
#110530=DIRECTION('',(0.,0.,-1.)) ;
#110531=DIRECTION('center_axis',(-1.,0.,0.)) ;
#110532=DIRECTION('ref_axis',(0.,-1.0842021724855E-15,-1.)) ;
#110533=DIRECTION('',(0.,-1.,0.)) ;
#110534=DIRECTION('center_axis',(-1.,0.,0.)) ;
#110535=DIRECTION('ref_axis',(0.,0.,-1.)) ;
#110536=DIRECTION('',(0.,0.,1.)) ;
#110537=DIRECTION('center_axis',(-1.,0.,0.)) ;
#110538=DIRECTION('ref_axis',(0.,0.,-1.)) ;
#110539=DIRECTION('center_axis',(1.53063836115601E-16,-1.,-1.30104260698261E-16)) ;
#110540=DIRECTION('ref_axis',(1.,1.53063836115601E-16,1.99142572374599E-32)) ;
#110541=DIRECTION('center_axis',(0.,1.,0.)) ;
#110542=DIRECTION('ref_axis',(0.,0.,1.)) ;
#110543=DIRECTION('center_axis',(0.,-1.,0.)) ;
#110544=DIRECTION('ref_axis',(0.,0.,-1.)) ;
#110545=DIRECTION('center_axis',(1.,1.53063836115601E-16,2.73691106313441E-48)) ;
#110546=DIRECTION('ref_axis',(-1.53063836115601E-16,1.,-4.18922106430579E-64)) ;
#110547=DIRECTION('center_axis',(-1.,0.,0.)) ;
#110548=DIRECTION('ref_axis',(0.,0.,1.)) ;
#110549=DIRECTION('center_axis',(1.,1.53063836115601E-16,0.)) ;
#110550=DIRECTION('ref_axis',(1.53063836115601E-16,-1.,0.)) ;
#110551=DIRECTION('center_axis',(0.,1.,0.)) ;
#110552=DIRECTION('ref_axis',(1.,0.,0.)) ;
#110553=DIRECTION('center_axis',(0.,1.,0.)) ;
#110554=DIRECTION('ref_axis',(0.,0.,-1.)) ;
#110555=DIRECTION('center_axis',(0.,0.,1.)) ;
#110556=DIRECTION('ref_axis',(-1.,0.,0.)) ;
#110557=DIRECTION('center_axis',(0.,1.,0.)) ;
#110558=DIRECTION('ref_axis',(1.,0.,0.)) ;
#110559=DIRECTION('center_axis',(0.,0.,1.)) ;
#110560=DIRECTION('ref_axis',(-1.,0.,0.)) ;
#110561=DIRECTION('center_axis',(1.,1.0842021724855E-15,0.)) ;
#110562=DIRECTION('ref_axis',(1.0842021724855E-15,-1.,0.)) ;
#110563=DIRECTION('center_axis',(-1.,-1.53063836115601E-16,0.)) ;
#110564=DIRECTION('ref_axis',(0.,-1.,0.)) ;
#110565=DIRECTION('center_axis',(0.,0.,-1.)) ;
#110566=DIRECTION('ref_axis',(1.,0.,0.)) ;
#110567=DIRECTION('center_axis',(0.,0.,-1.)) ;
#110568=DIRECTION('ref_axis',(0.804034447892617,0.594582716366709,0.)) ;
#110569=DIRECTION('center_axis',(0.,0.,1.)) ;
#110570=DIRECTION('ref_axis',(1.,0.,0.)) ;
#110571=DIRECTION('',(0.,0.,-1.)) ;
#110572=DIRECTION('center_axis',(-2.16840434497101E-16,1.,1.30104260698261E-16)) ;
#110573=DIRECTION('ref_axis',(1.,2.16840434497101E-16,1.22464679914735E-16)) ;
#110574=DIRECTION('',(-2.16840434497101E-16,1.,1.30104260698261E-16)) ;
#110575=DIRECTION('center_axis',(0.,1.,0.)) ;
#110576=DIRECTION('ref_axis',(0.,0.,1.)) ;
#110577=DIRECTION('center_axis',(-1.,-1.53063836115601E-16,-2.73691106313441E-48)) ;
#110578=DIRECTION('ref_axis',(1.53063836115601E-16,-1.,4.18922106430579E-64)) ;
#110579=DIRECTION('center_axis',(1.,2.16840434497101E-16,0.)) ;
#110580=DIRECTION('ref_axis',(2.16840434497101E-16,-1.,0.)) ;
#110581=DIRECTION('center_axis',(0.,0.,1.)) ;
#110582=DIRECTION('ref_axis',(1.,0.,0.)) ;
#110583=DIRECTION('center_axis',(-1.25542992828747E-32,1.020425574104E-16,
1.)) ;
#110584=DIRECTION('ref_axis',(-1.28107280532009E-48,-1.,1.020425574104E-16)) ;
#110585=DIRECTION('center_axis',(0.,0.,1.)) ;
#110586=DIRECTION('ref_axis',(1.,0.,0.)) ;
#110587=DIRECTION('center_axis',(0.,0.,-1.)) ;
#110588=DIRECTION('ref_axis',(-1.,0.,0.)) ;
#110589=DIRECTION('center_axis',(1.,1.53063836115601E-16,-2.73691106313441E-48)) ;
#110590=DIRECTION('ref_axis',(-1.53063836115601E-16,1.,4.18922106430579E-64)) ;
#110591=DIRECTION('center_axis',(-1.,0.,0.)) ;
#110592=DIRECTION('ref_axis',(0.,0.,1.)) ;
#110593=DIRECTION('center_axis',(1.,1.53063836115601E-16,0.)) ;
#110594=DIRECTION('ref_axis',(1.53063836115601E-16,-1.,0.)) ;
#110595=DIRECTION('center_axis',(0.,1.,0.)) ;
#110596=DIRECTION('ref_axis',(1.,0.,0.)) ;
#110597=DIRECTION('center_axis',(-1.,-2.16840434497101E-16,0.)) ;
#110598=DIRECTION('ref_axis',(0.,-1.,0.)) ;
#110599=DIRECTION('center_axis',(0.,0.,-1.)) ;
#110600=DIRECTION('ref_axis',(1.,0.,0.)) ;
#110601=DIRECTION('center_axis',(-1.25542992828747E-32,1.020425574104E-16,
1.)) ;
#110602=DIRECTION('ref_axis',(0.,-1.,0.)) ;
#110603=DIRECTION('center_axis',(0.,-1.,0.)) ;
#110604=DIRECTION('ref_axis',(-6.50521303491302E-15,0.,1.)) ;
#110605=DIRECTION('center_axis',(-1.,0.,0.)) ;
#110606=DIRECTION('ref_axis',(0.,0.,-1.)) ;
#110607=DIRECTION('center_axis',(-1.,-1.53063836115601E-16,0.)) ;
#110608=DIRECTION('ref_axis',(0.,-1.,0.)) ;
#110609=DIRECTION('center_axis',(0.,-1.,0.)) ;
#110610=DIRECTION('ref_axis',(0.,0.,1.)) ;
#110611=DIRECTION('center_axis',(0.,0.,-1.)) ;
#110612=DIRECTION('ref_axis',(-1.,0.,0.)) ;
#110613=DIRECTION('center_axis',(0.,0.,-1.)) ;
#110614=DIRECTION('ref_axis',(-1.,0.,0.)) ;
#110615=DIRECTION('center_axis',(1.,1.53063836115601E-16,-3.06472600140763E-33)) ;
#110616=DIRECTION('ref_axis',(-1.53063836115601E-16,1.,4.69098718418678E-49)) ;
#110617=DIRECTION('center_axis',(-1.,0.,0.)) ;
#110618=DIRECTION('ref_axis',(0.,0.,1.)) ;
#110619=DIRECTION('center_axis',(-1.53063836115601E-16,1.,-1.020425574104E-16)) ;
#110620=DIRECTION('ref_axis',(-1.,-1.53063836115601E-16,1.3684555315672E-47)) ;
#110621=DIRECTION('',(1.53063836115601E-16,-1.,1.020425574104E-16)) ;
#110622=DIRECTION('center_axis',(0.,-1.,0.)) ;
#110623=DIRECTION('ref_axis',(0.,0.,-1.)) ;
#110624=DIRECTION('center_axis',(-1.53063836115601E-16,1.,-1.30104260698261E-16)) ;
#110625=DIRECTION('ref_axis',(-1.,-1.53063836115601E-16,1.99142572374599E-32)) ;
#110626=DIRECTION('center_axis',(0.,-1.,0.)) ;
#110627=DIRECTION('ref_axis',(0.,0.,-1.)) ;
#110628=DIRECTION('center_axis',(-1.,-1.53063836115601E-16,2.73691106313441E-48)) ;
#110629=DIRECTION('ref_axis',(1.53063836115601E-16,-1.,-4.18922106430579E-64)) ;
#110630=DIRECTION('center_axis',(1.,2.16840434497101E-16,0.)) ;
#110631=DIRECTION('ref_axis',(2.16840434497101E-16,-1.,0.)) ;
#110632=DIRECTION('center_axis',(-1.,0.,2.16840434497101E-15)) ;
#110633=DIRECTION('ref_axis',(2.16840434497101E-15,0.,1.)) ;
#110634=DIRECTION('center_axis',(-1.,-2.16840434497101E-16,0.)) ;
#110635=DIRECTION('ref_axis',(0.,-1.,0.)) ;
#110636=DIRECTION('center_axis',(0.,0.,1.)) ;
#110637=DIRECTION('ref_axis',(-1.,0.,0.)) ;
#110638=DIRECTION('center_axis',(0.,1.,0.)) ;
#110639=DIRECTION('ref_axis',(1.,0.,0.)) ;
#110640=DIRECTION('center_axis',(0.,1.,0.)) ;
#110641=DIRECTION('ref_axis',(0.,0.,-1.)) ;
#110642=DIRECTION('center_axis',(1.,0.,0.)) ;
#110643=DIRECTION('ref_axis',(0.,-1.,0.)) ;
#110644=DIRECTION('center_axis',(1.,6.50521303491304E-15,0.)) ;
#110645=DIRECTION('ref_axis',(-6.50521303491304E-15,1.,0.)) ;
#110646=DIRECTION('center_axis',(8.67361737988403E-15,1.,0.)) ;
#110647=DIRECTION('ref_axis',(-1.,8.67361737988403E-15,0.)) ;
#110648=DIRECTION('center_axis',(1.2303003375722E-16,-1.,1.020425574104E-16)) ;
#110649=DIRECTION('ref_axis',(1.,1.2303003375722E-16,-1.25542992828747E-32)) ;
#110650=DIRECTION('center_axis',(0.,1.,0.)) ;
#110651=DIRECTION('ref_axis',(0.,0.,1.)) ;
#110652=DIRECTION('center_axis',(0.,1.,0.)) ;
#110653=DIRECTION('ref_axis',(1.,0.,0.)) ;
#110654=DIRECTION('center_axis',(1.,1.2303003375722E-16,0.)) ;
#110655=DIRECTION('ref_axis',(1.2303003375722E-16,-1.,0.)) ;
#110656=DIRECTION('center_axis',(-2.16840434497101E-15,0.,1.)) ;
#110657=DIRECTION('ref_axis',(-1.,0.,-2.16840434497101E-15)) ;
#110658=DIRECTION('center_axis',(0.,1.,0.)) ;
#110659=DIRECTION('ref_axis',(1.,0.,0.)) ;
#110660=DIRECTION('center_axis',(0.,0.,-1.)) ;
#110661=DIRECTION('ref_axis',(1.,0.,0.)) ;
#110662=DIRECTION('center_axis',(0.,0.,-1.)) ;
#110663=DIRECTION('ref_axis',(-1.,0.,0.)) ;
#110664=DIRECTION('center_axis',(0.,0.,1.)) ;
#110665=DIRECTION('ref_axis',(1.,0.,0.)) ;
#110666=DIRECTION('center_axis',(-2.16840434497101E-16,1.,-1.020425574104E-16)) ;
#110667=DIRECTION('ref_axis',(-1.,-2.16840434497101E-16,5.47382212626882E-48)) ;
#110668=DIRECTION('center_axis',(0.,1.,0.)) ;
#110669=DIRECTION('ref_axis',(0.,0.,-1.)) ;
#110670=DIRECTION('center_axis',(1.,0.,1.25542992828747E-32)) ;
#110671=DIRECTION('ref_axis',(1.25542992828747E-32,0.,-1.)) ;
#110672=DIRECTION('center_axis',(1.,0.,0.)) ;
#110673=DIRECTION('ref_axis',(0.,0.,-1.)) ;
#110674=DIRECTION('center_axis',(-1.,-1.2303003375722E-16,0.)) ;
#110675=DIRECTION('ref_axis',(0.,-1.,0.)) ;
#110676=DIRECTION('center_axis',(0.,0.,-1.)) ;
#110677=DIRECTION('ref_axis',(1.,0.,0.)) ;
#110678=DIRECTION('center_axis',(0.,0.,-1.)) ;
#110679=DIRECTION('ref_axis',(-1.,0.,0.)) ;
#110680=DIRECTION('',(0.,0.,1.)) ;
#110681=DIRECTION('center_axis',(0.,-2.16840434497101E-15,1.)) ;
#110682=DIRECTION('ref_axis',(0.,-1.,-2.16840434497101E-15)) ;
#110683=DIRECTION('center_axis',(0.,0.,1.)) ;
#110684=DIRECTION('ref_axis',(1.,0.,0.)) ;
#110685=DIRECTION('center_axis',(6.27714964143733E-33,-5.10212787052002E-17,
-1.)) ;
#110686=DIRECTION('ref_axis',(3.20268201330022E-49,1.,-5.10212787052002E-17)) ;
#110687=DIRECTION('center_axis',(1.,1.53063836115601E-16,-1.53236300070382E-33)) ;
#110688=DIRECTION('ref_axis',(-1.53063836115601E-16,1.,2.34549359209339E-49)) ;
#110689=DIRECTION('center_axis',(-1.,0.,0.)) ;
#110690=DIRECTION('ref_axis',(0.,0.,1.)) ;
#110691=DIRECTION('center_axis',(1.,0.,0.)) ;
#110692=DIRECTION('ref_axis',(0.,0.,-1.)) ;
#110693=DIRECTION('center_axis',(0.,1.,0.)) ;
#110694=DIRECTION('ref_axis',(1.,0.,0.)) ;
#110695=DIRECTION('center_axis',(-4.33680868994202E-15,1.,0.)) ;
#110696=DIRECTION('ref_axis',(1.,4.33680868994202E-15,0.)) ;
#110697=DIRECTION('center_axis',(0.,-1.,0.)) ;
#110698=DIRECTION('ref_axis',(0.,0.,-1.)) ;
#110699=DIRECTION('center_axis',(0.,0.,-1.)) ;
#110700=DIRECTION('ref_axis',(1.,0.,0.)) ;
#110701=DIRECTION('center_axis',(0.,0.,1.)) ;
#110702=DIRECTION('ref_axis',(1.,0.,0.)) ;
#110703=DIRECTION('center_axis',(0.,0.,-1.)) ;
#110704=DIRECTION('ref_axis',(-1.,0.,0.)) ;
#110705=DIRECTION('center_axis',(0.,1.,0.)) ;
#110706=DIRECTION('ref_axis',(1.,0.,0.)) ;
#110707=DIRECTION('center_axis',(1.,1.2303003375722E-16,0.)) ;
#110708=DIRECTION('ref_axis',(1.2303003375722E-16,-1.,0.)) ;
#110709=DIRECTION('center_axis',(0.,1.,0.)) ;
#110710=DIRECTION('ref_axis',(-6.50521303491302E-15,0.,-1.)) ;
#110711=DIRECTION('center_axis',(6.27714964143733E-33,-5.10212787052002E-17,
-1.)) ;
#110712=DIRECTION('ref_axis',(0.,1.,0.)) ;
#110713=DIRECTION('center_axis',(0.,-1.,0.)) ;
#110714=DIRECTION('ref_axis',(0.,0.,1.)) ;
#110715=DIRECTION('center_axis',(2.16840434497101E-16,-1.,5.10212787052002E-17)) ;
#110716=DIRECTION('ref_axis',(1.,2.16840434497101E-16,-5.47382212626882E-48)) ;
#110717=DIRECTION('center_axis',(0.,1.,0.)) ;
#110718=DIRECTION('ref_axis',(0.,0.,-1.)) ;
#110719=DIRECTION('center_axis',(0.,0.,1.)) ;
#110720=DIRECTION('ref_axis',(1.,0.,0.)) ;
#110721=DIRECTION('center_axis',(0.,0.,-1.)) ;
#110722=DIRECTION('ref_axis',(-1.,0.,0.)) ;
#110723=DIRECTION('center_axis',(-1.,-1.2303003375722E-16,0.)) ;
#110724=DIRECTION('ref_axis',(0.,-1.,0.)) ;
#110725=DIRECTION('center_axis',(0.,-1.,0.)) ;
#110726=DIRECTION('ref_axis',(0.,0.,1.)) ;
#110727=DIRECTION('center_axis',(1.53063836115601E-16,-1.,5.10212787052002E-17)) ;
#110728=DIRECTION('ref_axis',(1.,1.53063836115601E-16,-6.84227765783602E-48)) ;
#110729=DIRECTION('',(-1.53063836115601E-16,1.,-5.10212787052002E-17)) ;
#110730=DIRECTION('center_axis',(0.,-1.,0.)) ;
#110731=DIRECTION('ref_axis',(0.,0.,-1.)) ;
#110732=DIRECTION('center_axis',(-1.,0.,0.)) ;
#110733=DIRECTION('ref_axis',(0.,0.,-1.)) ;
#110734=DIRECTION('center_axis',(-1.2303003375722E-16,1.,-5.10212787052002E-17)) ;
#110735=DIRECTION('ref_axis',(-1.,-1.2303003375722E-16,6.27714964143733E-33)) ;
#110736=DIRECTION('center_axis',(-8.67361737988403E-15,-1.,0.)) ;
#110737=DIRECTION('ref_axis',(1.,-8.67361737988403E-15,0.)) ;
#110738=DIRECTION('center_axis',(1.,0.,6.27714964143733E-33)) ;
#110739=DIRECTION('ref_axis',(6.27714964143733E-33,0.,-1.)) ;
#110740=DIRECTION('center_axis',(-1.,0.,-6.5052130349128E-15)) ;
#110741=DIRECTION('ref_axis',(-6.5052130349128E-15,0.,1.)) ;
#110742=DIRECTION('center_axis',(1.,0.,0.)) ;
#110743=DIRECTION('ref_axis',(0.,1.,0.)) ;
#110744=DIRECTION('center_axis',(0.,1.,0.)) ;
#110745=DIRECTION('ref_axis',(1.,0.,0.)) ;
#110746=DIRECTION('center_axis',(1.,0.,0.)) ;
#110747=DIRECTION('ref_axis',(0.,0.,-1.)) ;
#110748=DIRECTION('center_axis',(0.,-1.,0.)) ;
#110749=DIRECTION('ref_axis',(0.,0.,-1.)) ;
#110750=DIRECTION('center_axis',(0.,1.,0.)) ;
#110751=DIRECTION('ref_axis',(0.,0.,1.)) ;
#110752=DIRECTION('center_axis',(0.,-1.,0.)) ;
#110753=DIRECTION('ref_axis',(0.,0.,-1.)) ;
#110754=DIRECTION('center_axis',(1.,0.,0.)) ;
#110755=DIRECTION('ref_axis',(0.,0.,-1.)) ;
#110756=DIRECTION('center_axis',(1.,0.,0.)) ;
#110757=DIRECTION('ref_axis',(0.,0.,-1.)) ;
#110758=DIRECTION('center_axis',(0.,0.,1.)) ;
#110759=DIRECTION('ref_axis',(1.,0.,0.)) ;
#110760=DIRECTION('center_axis',(-1.,8.67361737988401E-15,-8.67361737988379E-15)) ;
#110761=DIRECTION('ref_axis',(-8.67361737988401E-15,-1.,1.07724819444908E-44)) ;
#110762=DIRECTION('center_axis',(0.,1.,0.)) ;
#110763=DIRECTION('ref_axis',(1.,0.,0.)) ;
#110764=DIRECTION('center_axis',(0.,-1.,0.)) ;
#110765=DIRECTION('ref_axis',(0.,0.,-1.)) ;
#110766=DIRECTION('center_axis',(1.,1.59148942750166E-16,0.)) ;
#110767=DIRECTION('ref_axis',(-1.59148942750166E-16,1.,0.)) ;
#110768=DIRECTION('center_axis',(-1.,0.,6.50521303491284E-15)) ;
#110769=DIRECTION('ref_axis',(6.50521303491284E-15,0.,1.)) ;
#110770=DIRECTION('center_axis',(-4.33680868994203E-15,-1.,0.)) ;
#110771=DIRECTION('ref_axis',(1.,-4.33680868994203E-15,0.)) ;
#110772=DIRECTION('center_axis',(-8.67361737988401E-15,-1.,0.)) ;
#110773=DIRECTION('ref_axis',(1.,-8.67361737988401E-15,0.)) ;
#110774=DIRECTION('center_axis',(0.,1.,0.)) ;
#110775=DIRECTION('ref_axis',(1.,0.,0.)) ;
#110776=DIRECTION('center_axis',(8.67361737988403E-15,-1.,0.)) ;
#110777=DIRECTION('ref_axis',(1.,8.67361737988403E-15,0.)) ;
#110778=DIRECTION('center_axis',(0.,0.,1.)) ;
#110779=DIRECTION('ref_axis',(1.,0.,0.)) ;
#110780=DIRECTION('center_axis',(1.,8.67361737988401E-15,0.)) ;
#110781=DIRECTION('ref_axis',(-8.67361737988401E-15,1.,0.)) ;
#110782=DIRECTION('center_axis',(-1.2303003375722E-16,1.,0.)) ;
#110783=DIRECTION('ref_axis',(-1.,-1.2303003375722E-16,0.)) ;
#110784=DIRECTION('center_axis',(0.,-1.,8.67361737988379E-15)) ;
#110785=DIRECTION('ref_axis',(0.,-8.67361737988379E-15,-1.)) ;
#110786=DIRECTION('center_axis',(1.,-5.88041856263325E-16,0.)) ;
#110787=DIRECTION('ref_axis',(5.88041856263325E-16,1.,0.)) ;
#110788=DIRECTION('center_axis',(1.,0.,0.)) ;
#110789=DIRECTION('ref_axis',(0.,0.,-1.)) ;
#110790=DIRECTION('center_axis',(0.,1.,0.)) ;
#110791=DIRECTION('ref_axis',(1.,0.,0.)) ;
#110792=DIRECTION('center_axis',(1.,6.50521303491304E-15,0.)) ;
#110793=DIRECTION('ref_axis',(-6.50521303491304E-15,1.,0.)) ;
#110794=DIRECTION('center_axis',(0.,1.,0.)) ;
#110795=DIRECTION('ref_axis',(1.,0.,0.)) ;
#110796=DIRECTION('center_axis',(0.,-1.,0.)) ;
#110797=DIRECTION('ref_axis',(0.,0.,-1.)) ;
#110798=DIRECTION('center_axis',(-1.,0.,0.)) ;
#110799=DIRECTION('ref_axis',(0.,0.,1.)) ;
#110800=DIRECTION('center_axis',(1.,0.,1.73472347597676E-14)) ;
#110801=DIRECTION('ref_axis',(1.73472347597676E-14,0.,-1.)) ;
#110802=DIRECTION('center_axis',(0.,-1.,0.)) ;
#110803=DIRECTION('ref_axis',(0.,0.,-1.)) ;
#110804=DIRECTION('center_axis',(8.67361737988409E-15,-1.,0.)) ;
#110805=DIRECTION('ref_axis',(1.,8.67361737988409E-15,0.)) ;
#110806=DIRECTION('center_axis',(0.,1.,0.)) ;
#110807=DIRECTION('ref_axis',(1.,0.,0.)) ;
#110808=DIRECTION('center_axis',(0.,1.,0.)) ;
#110809=DIRECTION('ref_axis',(1.,0.,0.)) ;
#110810=DIRECTION('center_axis',(1.,0.,0.)) ;
#110811=DIRECTION('ref_axis',(0.,0.,-1.)) ;
#110812=DIRECTION('center_axis',(0.,-1.,0.)) ;
#110813=DIRECTION('ref_axis',(0.,0.,-1.)) ;
#110814=DIRECTION('center_axis',(0.,-1.,0.)) ;
#110815=DIRECTION('ref_axis',(0.,0.,-1.)) ;
#110816=DIRECTION('center_axis',(0.,-1.,0.)) ;
#110817=DIRECTION('ref_axis',(0.,0.,-1.)) ;
#110818=DIRECTION('center_axis',(-1.,0.,0.)) ;
#110819=DIRECTION('ref_axis',(0.,0.,1.)) ;
#110820=DIRECTION('center_axis',(1.,0.,0.)) ;
#110821=DIRECTION('ref_axis',(0.,0.,-1.)) ;
#110822=DIRECTION('center_axis',(0.,0.,1.)) ;
#110823=DIRECTION('ref_axis',(1.,0.,0.)) ;
#110824=DIRECTION('center_axis',(-1.,0.,0.)) ;
#110825=DIRECTION('ref_axis',(0.,0.,1.)) ;
#110826=DIRECTION('center_axis',(0.,1.,0.)) ;
#110827=DIRECTION('ref_axis',(1.,0.,0.)) ;
#110828=DIRECTION('center_axis',(0.,-1.,0.)) ;
#110829=DIRECTION('ref_axis',(0.,0.,-1.)) ;
#110830=DIRECTION('center_axis',(-1.,-1.59148942750166E-16,0.)) ;
#110831=DIRECTION('ref_axis',(1.59148942750166E-16,-1.,0.)) ;
#110832=DIRECTION('center_axis',(-1.,6.50521303491307E-15,0.)) ;
#110833=DIRECTION('ref_axis',(-6.50521303491307E-15,-1.,0.)) ;
#110834=DIRECTION('center_axis',(4.33680868994203E-15,1.,0.)) ;
#110835=DIRECTION('ref_axis',(-1.,4.33680868994203E-15,0.)) ;
#110836=DIRECTION('center_axis',(-8.67361737988401E-15,-1.,0.)) ;
#110837=DIRECTION('ref_axis',(1.,-8.67361737988401E-15,0.)) ;
#110838=DIRECTION('center_axis',(0.,1.,0.)) ;
#110839=DIRECTION('ref_axis',(1.,0.,0.)) ;
#110840=DIRECTION('center_axis',(8.67361737988403E-15,-1.,0.)) ;
#110841=DIRECTION('ref_axis',(1.,8.67361737988403E-15,0.)) ;
#110842=DIRECTION('center_axis',(0.,0.,1.)) ;
#110843=DIRECTION('ref_axis',(1.,0.,0.)) ;
#110844=DIRECTION('center_axis',(1.,8.67361737988401E-15,0.)) ;
#110845=DIRECTION('ref_axis',(-8.67361737988401E-15,1.,0.)) ;
#110846=DIRECTION('center_axis',(1.2303003375722E-16,-1.,0.)) ;
#110847=DIRECTION('ref_axis',(1.,1.2303003375722E-16,0.)) ;
#110848=DIRECTION('center_axis',(-8.67361737988416E-15,-1.,0.)) ;
#110849=DIRECTION('ref_axis',(1.,-8.67361737988416E-15,0.)) ;
#110850=DIRECTION('center_axis',(-1.,5.88041856263325E-16,0.)) ;
#110851=DIRECTION('ref_axis',(-5.88041856263325E-16,-1.,0.)) ;
#110852=DIRECTION('center_axis',(1.,0.,0.)) ;
#110853=DIRECTION('ref_axis',(0.,0.,-1.)) ;
#110854=DIRECTION('center_axis',(0.,1.,0.)) ;
#110855=DIRECTION('ref_axis',(1.,0.,0.)) ;
#110856=DIRECTION('center_axis',(1.,6.50521303491304E-15,0.)) ;
#110857=DIRECTION('ref_axis',(-6.50521303491304E-15,1.,0.)) ;
#110858=DIRECTION('center_axis',(0.,1.,0.)) ;
#110859=DIRECTION('ref_axis',(1.,0.,0.)) ;
#110860=DIRECTION('center_axis',(0.,-1.,0.)) ;
#110861=DIRECTION('ref_axis',(0.,0.,-1.)) ;
#110862=DIRECTION('center_axis',(1.,0.,0.)) ;
#110863=DIRECTION('ref_axis',(0.,0.,-1.)) ;
#110864=DIRECTION('center_axis',(1.,-1.73472347597681E-14,0.)) ;
#110865=DIRECTION('ref_axis',(1.73472347597681E-14,1.,0.)) ;
#110866=DIRECTION('center_axis',(0.,1.,0.)) ;
#110867=DIRECTION('ref_axis',(0.,0.,1.)) ;
#110868=DIRECTION('center_axis',(0.,-1.,-8.67361737988405E-15)) ;
#110869=DIRECTION('ref_axis',(0.,8.67361737988405E-15,-1.)) ;
#110870=DIRECTION('center_axis',(0.,1.,0.)) ;
#110871=DIRECTION('ref_axis',(1.,0.,0.)) ;
#110872=DIRECTION('center_axis',(0.,0.,-1.)) ;
#110873=DIRECTION('ref_axis',(-1.,0.,0.)) ;
#110874=DIRECTION('center_axis',(0.,0.,1.)) ;
#110875=DIRECTION('ref_axis',(1.,0.,0.)) ;
#110876=DIRECTION('center_axis',(0.,0.,-1.)) ;
#110877=DIRECTION('ref_axis',(-1.,0.,0.)) ;
#110878=DIRECTION('center_axis',(-1.,0.,0.)) ;
#110879=DIRECTION('ref_axis',(0.,0.,1.)) ;
#110880=DIRECTION('center_axis',(0.,-1.,0.)) ;
#110881=DIRECTION('ref_axis',(0.,0.,-1.)) ;
#110882=DIRECTION('center_axis',(0.,1.,0.)) ;
#110883=DIRECTION('ref_axis',(0.,0.,1.)) ;
#110884=DIRECTION('center_axis',(0.,1.,-6.50521303491302E-15)) ;
#110885=DIRECTION('ref_axis',(0.,6.50521303491302E-15,1.)) ;
#110886=DIRECTION('center_axis',(0.,-1.,0.)) ;
#110887=DIRECTION('ref_axis',(0.,0.,-1.)) ;
#110888=DIRECTION('center_axis',(0.,-1.,0.)) ;
#110889=DIRECTION('ref_axis',(0.,0.,-1.)) ;
#110890=DIRECTION('center_axis',(0.,-1.,-1.07081696047951E-16)) ;
#110891=DIRECTION('ref_axis',(0.,1.07081696047951E-16,-1.)) ;
#110892=DIRECTION('center_axis',(0.,1.,0.)) ;
#110893=DIRECTION('ref_axis',(0.,0.,1.)) ;
#110894=DIRECTION('center_axis',(-1.,0.,0.)) ;
#110895=DIRECTION('ref_axis',(0.,0.,1.)) ;
#110896=DIRECTION('center_axis',(0.,0.,1.)) ;
#110897=DIRECTION('ref_axis',(1.,0.,0.)) ;
#110898=DIRECTION('center_axis',(0.,1.,0.)) ;
#110899=DIRECTION('ref_axis',(0.,0.,1.)) ;
#110900=DIRECTION('center_axis',(0.,-6.50521303491304E-15,-1.)) ;
#110901=DIRECTION('ref_axis',(0.,1.,-6.50521303491304E-15)) ;
#110902=DIRECTION('center_axis',(0.,0.,1.)) ;
#110903=DIRECTION('ref_axis',(1.,0.,0.)) ;
#110904=DIRECTION('center_axis',(0.,-1.08420217248551E-15,1.)) ;
#110905=DIRECTION('ref_axis',(0.,-1.,-1.08420217248551E-15)) ;
#110906=DIRECTION('center_axis',(0.,0.,1.)) ;
#110907=DIRECTION('ref_axis',(1.,0.,0.)) ;
#110908=DIRECTION('center_axis',(0.,0.,-1.)) ;
#110909=DIRECTION('ref_axis',(-1.,0.,0.)) ;
#110910=DIRECTION('center_axis',(0.,1.,0.)) ;
#110911=DIRECTION('ref_axis',(0.,0.,1.)) ;
#110912=DIRECTION('center_axis',(0.,-0.707106781186548,0.707106781186547)) ;
#110913=DIRECTION('ref_axis',(0.,-0.707106781186547,-0.707106781186548)) ;
#110914=DIRECTION('center_axis',(0.,1.,0.)) ;
#110915=DIRECTION('ref_axis',(0.,0.,1.)) ;
#110916=DIRECTION('center_axis',(0.,-0.5142317969591,-0.857651245551602)) ;
#110917=DIRECTION('ref_axis',(0.,0.857651245551602,-0.5142317969591)) ;
#110918=DIRECTION('center_axis',(0.,-0.707106781186548,0.707106781186547)) ;
#110919=DIRECTION('ref_axis',(0.,-0.707106781186547,-0.707106781186548)) ;
#110920=DIRECTION('center_axis',(0.,-0.70710678118655,0.707106781186545)) ;
#110921=DIRECTION('ref_axis',(0.,-0.707106781186545,-0.70710678118655)) ;
#110922=DIRECTION('center_axis',(-1.,0.,0.)) ;
#110923=DIRECTION('ref_axis',(0.,0.,1.)) ;
#110924=DIRECTION('center_axis',(0.,0.514231796959101,-0.857651245551602)) ;
#110925=DIRECTION('ref_axis',(0.,0.857651245551602,0.514231796959101)) ;
#110926=DIRECTION('center_axis',(0.,1.,0.)) ;
#110927=DIRECTION('ref_axis',(0.,0.,1.)) ;
#110928=DIRECTION('center_axis',(0.,0.,-1.)) ;
#110929=DIRECTION('ref_axis',(-1.,0.,0.)) ;
#110930=DIRECTION('center_axis',(0.,1.,0.)) ;
#110931=DIRECTION('ref_axis',(0.,0.,1.)) ;
#110932=DIRECTION('center_axis',(0.,0.,-1.)) ;
#110933=DIRECTION('ref_axis',(-1.,0.,0.)) ;
#110934=DIRECTION('center_axis',(0.,0.,-1.)) ;
#110935=DIRECTION('ref_axis',(-1.,0.,0.)) ;
#110936=DIRECTION('center_axis',(0.,0.,1.)) ;
#110937=DIRECTION('ref_axis',(1.,0.,0.)) ;
#110938=DIRECTION('center_axis',(0.,0.,-1.)) ;
#110939=DIRECTION('ref_axis',(-1.,0.,0.)) ;
#110940=DIRECTION('center_axis',(0.,1.,0.)) ;
#110941=DIRECTION('ref_axis',(0.,0.,1.)) ;
#110942=DIRECTION('center_axis',(0.,-1.,8.67361737988403E-15)) ;
#110943=DIRECTION('ref_axis',(0.,-8.67361737988403E-15,-1.)) ;
#110944=DIRECTION('center_axis',(0.,0.707106781186546,0.707106781186549)) ;
#110945=DIRECTION('ref_axis',(0.,-0.707106781186549,0.707106781186546)) ;
#110946=DIRECTION('center_axis',(0.,0.707106781186547,0.707106781186548)) ;
#110947=DIRECTION('ref_axis',(0.,-0.707106781186548,0.707106781186547)) ;
#110948=DIRECTION('center_axis',(0.,1.,1.07081696047951E-16)) ;
#110949=DIRECTION('ref_axis',(0.,-1.07081696047951E-16,1.)) ;
#110950=DIRECTION('center_axis',(0.,-1.,0.)) ;
#110951=DIRECTION('ref_axis',(0.,0.,-1.)) ;
#110952=DIRECTION('center_axis',(0.,1.,0.)) ;
#110953=DIRECTION('ref_axis',(0.,0.,1.)) ;
#110954=DIRECTION('center_axis',(0.,-1.08420217248551E-15,1.)) ;
#110955=DIRECTION('ref_axis',(0.,-1.,-1.08420217248551E-15)) ;
#110956=DIRECTION('center_axis',(0.,1.,0.)) ;
#110957=DIRECTION('ref_axis',(0.,0.,1.)) ;
#110958=DIRECTION('center_axis',(0.,6.50521303491302E-15,1.)) ;
#110959=DIRECTION('ref_axis',(0.,-1.,6.50521303491302E-15)) ;
#110960=DIRECTION('center_axis',(0.,3.99416362155027E-15,1.)) ;
#110961=DIRECTION('ref_axis',(0.,-1.,3.99416362155027E-15)) ;
#110962=DIRECTION('center_axis',(0.,0.,1.)) ;
#110963=DIRECTION('ref_axis',(1.,0.,0.)) ;
#110964=DIRECTION('center_axis',(0.,0.,-1.)) ;
#110965=DIRECTION('ref_axis',(-1.,0.,0.)) ;
#110966=DIRECTION('center_axis',(0.,0.,1.)) ;
#110967=DIRECTION('ref_axis',(1.,0.,0.)) ;
#110968=DIRECTION('center_axis',(-1.,0.,0.)) ;
#110969=DIRECTION('ref_axis',(0.,0.,1.)) ;
#110970=DIRECTION('center_axis',(0.,1.,0.)) ;
#110971=DIRECTION('ref_axis',(0.,0.,1.)) ;
#110972=DIRECTION('center_axis',(-1.,0.,0.)) ;
#110973=DIRECTION('ref_axis',(0.,0.,1.)) ;
#110974=DIRECTION('center_axis',(0.,-1.,0.)) ;
#110975=DIRECTION('ref_axis',(0.,0.,-1.)) ;
#110976=DIRECTION('center_axis',(0.,1.,0.)) ;
#110977=DIRECTION('ref_axis',(0.,0.,1.)) ;
#110978=DIRECTION('center_axis',(0.,-1.,0.)) ;
#110979=DIRECTION('ref_axis',(0.,0.,-1.)) ;
#110980=DIRECTION('center_axis',(0.,1.,0.)) ;
#110981=DIRECTION('ref_axis',(0.,0.,1.)) ;
#110982=DIRECTION('center_axis',(0.,-1.,0.)) ;
#110983=DIRECTION('ref_axis',(0.,0.,-1.)) ;
#110984=DIRECTION('center_axis',(0.,1.,0.)) ;
#110985=DIRECTION('ref_axis',(0.,0.,-1.)) ;
#110986=DIRECTION('center_axis',(-4.70197740328919E-30,-1.08420217248551E-15,
-1.)) ;
#110987=DIRECTION('ref_axis',(6.22301527786114E-61,1.,-1.08420217248551E-15)) ;
#110988=DIRECTION('center_axis',(0.,1.,0.)) ;
#110989=DIRECTION('ref_axis',(0.,0.,-1.)) ;
#110990=DIRECTION('center_axis',(0.,0.,-1.)) ;
#110991=DIRECTION('ref_axis',(-1.,0.,0.)) ;
#110992=DIRECTION('center_axis',(0.,0.,1.)) ;
#110993=DIRECTION('ref_axis',(1.,0.,0.)) ;
#110994=DIRECTION('center_axis',(0.,0.,-1.)) ;
#110995=DIRECTION('ref_axis',(-1.,0.,0.)) ;
#110996=DIRECTION('center_axis',(0.,0.,-1.)) ;
#110997=DIRECTION('ref_axis',(-1.,0.,0.)) ;
#110998=DIRECTION('center_axis',(0.,6.50521303491304E-15,-1.)) ;
#110999=DIRECTION('ref_axis',(0.,1.,6.50521303491304E-15)) ;
#111000=DIRECTION('center_axis',(1.,0.,0.)) ;
#111001=DIRECTION('ref_axis',(0.,0.,-1.)) ;
#111002=DIRECTION('center_axis',(0.,0.707106781186548,-0.707106781186548)) ;
#111003=DIRECTION('ref_axis',(0.,0.707106781186548,0.707106781186548)) ;
#111004=DIRECTION('center_axis',(1.,0.,0.)) ;
#111005=DIRECTION('ref_axis',(0.,0.,-1.)) ;
#111006=DIRECTION('center_axis',(0.,-1.,0.)) ;
#111007=DIRECTION('ref_axis',(0.,0.,-1.)) ;
#111008=DIRECTION('center_axis',(0.,-0.707106781186548,0.707106781186547)) ;
#111009=DIRECTION('ref_axis',(0.,-0.707106781186547,-0.707106781186548)) ;
#111010=DIRECTION('center_axis',(0.,-1.,-1.07081696047951E-16)) ;
#111011=DIRECTION('ref_axis',(0.,1.07081696047951E-16,-1.)) ;
#111012=DIRECTION('center_axis',(0.,-1.,-8.67361737988403E-15)) ;
#111013=DIRECTION('ref_axis',(0.,8.67361737988403E-15,-1.)) ;
#111014=DIRECTION('center_axis',(1.,0.,0.)) ;
#111015=DIRECTION('ref_axis',(0.,0.,-1.)) ;
#111016=DIRECTION('center_axis',(0.,0.,1.)) ;
#111017=DIRECTION('ref_axis',(1.,0.,0.)) ;
#111018=DIRECTION('center_axis',(0.,0.,-1.)) ;
#111019=DIRECTION('ref_axis',(-1.,0.,0.)) ;
#111020=DIRECTION('center_axis',(0.,0.,1.)) ;
#111021=DIRECTION('ref_axis',(1.,0.,0.)) ;
#111022=DIRECTION('center_axis',(0.,0.,1.)) ;
#111023=DIRECTION('ref_axis',(1.,0.,0.)) ;
#111024=DIRECTION('center_axis',(0.,0.,1.)) ;
#111025=DIRECTION('ref_axis',(1.,0.,0.)) ;
#111026=DIRECTION('center_axis',(1.,0.,0.)) ;
#111027=DIRECTION('ref_axis',(0.,0.382683432365091,0.923879532511286)) ;
#111028=DIRECTION('center_axis',(0.,-0.707106781186551,-0.707106781186544)) ;
#111029=DIRECTION('ref_axis',(0.,0.707106781186544,-0.707106781186551)) ;
#111030=DIRECTION('center_axis',(1.,0.,0.)) ;
#111031=DIRECTION('ref_axis',(0.,0.,-1.)) ;
#111032=DIRECTION('center_axis',(0.,0.5142317969591,0.857651245551602)) ;
#111033=DIRECTION('ref_axis',(0.,-0.857651245551602,0.5142317969591)) ;
#111034=DIRECTION('center_axis',(0.,0.707106781186546,0.707106781186549)) ;
#111035=DIRECTION('ref_axis',(0.,-0.707106781186549,0.707106781186546)) ;
#111036=DIRECTION('center_axis',(0.,-0.707106781186546,-0.707106781186549)) ;
#111037=DIRECTION('ref_axis',(0.,0.707106781186549,-0.707106781186546)) ;
#111038=DIRECTION('center_axis',(1.,0.,0.)) ;
#111039=DIRECTION('ref_axis',(0.,0.,-1.)) ;
#111040=DIRECTION('center_axis',(0.,-0.514231796959099,0.857651245551603)) ;
#111041=DIRECTION('ref_axis',(0.,-0.857651245551603,-0.514231796959099)) ;
#111042=DIRECTION('center_axis',(1.,0.,0.)) ;
#111043=DIRECTION('ref_axis',(0.,0.,-1.)) ;
#111044=DIRECTION('center_axis',(0.,1.08420217248551E-15,-1.)) ;
#111045=DIRECTION('ref_axis',(0.,1.,1.08420217248551E-15)) ;
#111046=DIRECTION('center_axis',(1.,0.,0.)) ;
#111047=DIRECTION('ref_axis',(0.,0.,-1.)) ;
#111048=DIRECTION('center_axis',(0.,0.,1.)) ;
#111049=DIRECTION('ref_axis',(1.,0.,0.)) ;
#111050=DIRECTION('center_axis',(0.,3.99416362155027E-15,1.)) ;
#111051=DIRECTION('ref_axis',(0.,-1.,3.99416362155027E-15)) ;
#111052=DIRECTION('center_axis',(0.,-4.33680868994202E-15,-1.)) ;
#111053=DIRECTION('ref_axis',(0.,1.,-4.33680868994202E-15)) ;
#111054=DIRECTION('center_axis',(0.,0.,1.)) ;
#111055=DIRECTION('ref_axis',(1.,0.,0.)) ;
#111056=DIRECTION('center_axis',(0.,-6.50521303491304E-15,1.)) ;
#111057=DIRECTION('ref_axis',(0.,-1.,-6.50521303491304E-15)) ;
#111058=DIRECTION('center_axis',(0.,1.,0.)) ;
#111059=DIRECTION('ref_axis',(0.,0.,-1.)) ;
#111060=DIRECTION('center_axis',(0.,-1.,0.)) ;
#111061=DIRECTION('ref_axis',(0.,0.,-1.)) ;
#111062=DIRECTION('center_axis',(1.,0.,0.)) ;
#111063=DIRECTION('ref_axis',(0.,0.,-1.)) ;
#111064=DIRECTION('center_axis',(0.,1.,0.)) ;
#111065=DIRECTION('ref_axis',(0.,0.,1.)) ;
#111066=DIRECTION('center_axis',(0.,1.,0.)) ;
#111067=DIRECTION('ref_axis',(0.,0.,1.)) ;
#111068=DIRECTION('center_axis',(0.,-1.,0.)) ;
#111069=DIRECTION('ref_axis',(0.,0.,-1.)) ;
#111070=DIRECTION('center_axis',(0.,1.,1.07081696047951E-16)) ;
#111071=DIRECTION('ref_axis',(0.,-1.07081696047951E-16,1.)) ;
#111072=DIRECTION('center_axis',(0.,1.,6.50521303491302E-15)) ;
#111073=DIRECTION('ref_axis',(0.,-6.50521303491302E-15,1.)) ;
#111074=DIRECTION('center_axis',(0.,1.,0.)) ;
#111075=DIRECTION('ref_axis',(0.,0.,-1.)) ;
#111076=DIRECTION('center_axis',(0.,0.,1.)) ;
#111077=DIRECTION('ref_axis',(1.,0.,0.)) ;
#111078=DIRECTION('center_axis',(1.,0.,0.)) ;
#111079=DIRECTION('ref_axis',(0.,0.,-1.)) ;
#111080=DIRECTION('center_axis',(0.,0.,-1.)) ;
#111081=DIRECTION('ref_axis',(-1.,0.,0.)) ;
#111082=DIRECTION('center_axis',(0.,0.,-1.)) ;
#111083=DIRECTION('ref_axis',(-1.,0.,0.)) ;
#111084=DIRECTION('center_axis',(1.,-9.85638338623186E-18,0.)) ;
#111085=DIRECTION('ref_axis',(9.85638338623186E-18,1.,0.)) ;
#111086=DIRECTION('',(0.,0.,-1.)) ;
#111087=DIRECTION('',(-9.85638338623186E-18,-1.,0.)) ;
#111088=DIRECTION('',(0.,0.,1.)) ;
#111089=DIRECTION('',(9.85638338623186E-18,1.,0.)) ;
#111090=DIRECTION('center_axis',(0.707106781186548,0.707106781186548,0.)) ;
#111091=DIRECTION('ref_axis',(-0.707106781186548,0.707106781186548,0.)) ;
#111092=DIRECTION('',(0.,0.,1.)) ;
#111093=DIRECTION('',(-0.577350269189625,0.577350269189625,0.577350269189627)) ;
#111094=DIRECTION('',(0.,0.,-1.)) ;
#111095=DIRECTION('',(0.577350269189625,-0.577350269189625,0.577350269189627)) ;
#111096=DIRECTION('center_axis',(0.,1.,0.)) ;
#111097=DIRECTION('ref_axis',(0.,0.,1.)) ;
#111098=DIRECTION('',(0.,0.,1.)) ;
#111099=DIRECTION('',(-1.,0.,-9.8563833862319E-18)) ;
#111100=DIRECTION('',(0.,0.,-1.)) ;
#111101=DIRECTION('',(1.,0.,-9.8563833862319E-18)) ;
#111102=DIRECTION('center_axis',(-0.707106781186548,0.707106781186548,0.)) ;
#111103=DIRECTION('ref_axis',(-0.707106781186548,-0.707106781186548,0.)) ;
#111104=DIRECTION('',(0.,0.,1.)) ;
#111105=DIRECTION('',(-0.577350269189625,-0.577350269189625,-0.577350269189627)) ;
#111106=DIRECTION('',(0.,0.,-1.)) ;
#111107=DIRECTION('',(0.577350269189625,0.577350269189625,-0.577350269189627)) ;
#111108=DIRECTION('center_axis',(-1.,9.85638338623186E-18,0.)) ;
#111109=DIRECTION('ref_axis',(-9.85638338623186E-18,-1.,0.)) ;
#111110=DIRECTION('',(0.,0.,-1.)) ;
#111111=DIRECTION('',(9.85638338623186E-18,1.,0.)) ;
#111112=DIRECTION('',(0.,0.,-1.)) ;
#111113=DIRECTION('',(-9.85638338623186E-18,-1.,0.)) ;
#111114=DIRECTION('center_axis',(0.,0.,1.)) ;
#111115=DIRECTION('ref_axis',(1.,0.,0.)) ;
#111116=DIRECTION('',(9.85638338623186E-18,1.,0.)) ;
#111117=DIRECTION('center_axis',(0.,0.,-1.)) ;
#111118=DIRECTION('ref_axis',(1.,0.,0.)) ;
#111119=DIRECTION('center_axis',(0.,0.,1.)) ;
#111120=DIRECTION('ref_axis',(1.,0.,0.)) ;
#111121=DIRECTION('',(-9.85638338623186E-18,-1.,0.)) ;
#111122=DIRECTION('',(1.,-9.85638338623186E-18,0.)) ;
#111123=DIRECTION('center_axis',(0.,0.,1.)) ;
#111124=DIRECTION('ref_axis',(1.,0.,0.)) ;
#111125=DIRECTION('',(9.85638338623186E-18,1.,0.)) ;
#111126=DIRECTION('center_axis',(0.,0.,-1.)) ;
#111127=DIRECTION('ref_axis',(1.,0.,0.)) ;
#111128=DIRECTION('center_axis',(0.,0.,1.)) ;
#111129=DIRECTION('ref_axis',(1.,0.,0.)) ;
#111130=DIRECTION('',(-9.85638338623186E-18,-1.,0.)) ;
#111131=DIRECTION('',(-1.,9.85638338623186E-18,0.)) ;
#111132=DIRECTION('center_axis',(0.,0.,-1.)) ;
#111133=DIRECTION('ref_axis',(-1.,0.,0.)) ;
#111134=DIRECTION('center_axis',(0.,0.,1.)) ;
#111135=DIRECTION('ref_axis',(1.,0.,0.)) ;
#111136=DIRECTION('center_axis',(0.,0.,-1.)) ;
#111137=DIRECTION('ref_axis',(1.,0.,0.)) ;
#111138=DIRECTION('center_axis',(0.,0.,-1.)) ;
#111139=DIRECTION('ref_axis',(-1.,0.,0.)) ;
#111140=DIRECTION('center_axis',(0.,0.,-1.)) ;
#111141=DIRECTION('ref_axis',(1.,0.,0.)) ;
#111142=DIRECTION('center_axis',(0.,0.,1.)) ;
#111143=DIRECTION('ref_axis',(1.,0.,0.)) ;
#111144=DIRECTION('center_axis',(-0.707106781186548,-0.707106781186547,
0.)) ;
#111145=DIRECTION('ref_axis',(0.707106781186547,-0.707106781186548,0.)) ;
#111146=DIRECTION('',(0.,0.,1.)) ;
#111147=DIRECTION('',(0.577350269189625,-0.577350269189626,-0.577350269189626)) ;
#111148=DIRECTION('',(0.,0.,-1.)) ;
#111149=DIRECTION('',(-0.577350269189625,0.577350269189626,-0.577350269189626)) ;
#111150=DIRECTION('center_axis',(1.95511867169517E-16,-1.,0.)) ;
#111151=DIRECTION('ref_axis',(1.,1.95511867169517E-16,0.)) ;
#111152=DIRECTION('',(0.,0.,-1.)) ;
#111153=DIRECTION('',(-1.,-1.95511867169517E-16,0.)) ;
#111154=DIRECTION('',(1.,1.95511867169517E-16,0.)) ;
#111155=DIRECTION('center_axis',(1.06642836637918E-16,1.,0.)) ;
#111156=DIRECTION('ref_axis',(-1.,1.06642836637918E-16,0.)) ;
#111157=DIRECTION('',(1.,-1.06642836637919E-16,0.)) ;
#111158=DIRECTION('',(0.,0.,1.)) ;
#111159=DIRECTION('',(-1.,1.06642836637919E-16,0.)) ;
#111160=DIRECTION('center_axis',(-0.707106781186548,0.707106781186547,0.)) ;
#111161=DIRECTION('ref_axis',(-0.707106781186547,-0.707106781186548,0.)) ;
#111162=DIRECTION('',(0.,0.,1.)) ;
#111163=DIRECTION('',(-0.577350269189625,-0.577350269189626,0.577350269189627)) ;
#111164=DIRECTION('',(0.,0.,-1.)) ;
#111165=DIRECTION('',(0.577350269189625,0.577350269189626,0.577350269189627)) ;
#111166=DIRECTION('center_axis',(-1.,0.,0.)) ;
#111167=DIRECTION('ref_axis',(0.,0.,1.)) ;
#111168=DIRECTION('',(0.,0.,-1.)) ;
#111169=DIRECTION('',(0.,1.,1.95511867169518E-16)) ;
#111170=DIRECTION('',(0.,0.,1.)) ;
#111171=DIRECTION('',(0.,-1.,1.95511867169518E-16)) ;
#111172=DIRECTION('center_axis',(0.,0.,1.)) ;
#111173=DIRECTION('ref_axis',(1.,0.,0.)) ;
#111174=DIRECTION('',(-1.95511867169517E-16,1.,0.)) ;
#111175=DIRECTION('',(-1.,-1.95511867169517E-16,0.)) ;
#111176=DIRECTION('',(1.,-1.06642836637919E-16,0.)) ;
#111177=DIRECTION('center_axis',(0.,0.,1.)) ;
#111178=DIRECTION('ref_axis',(1.,0.,0.)) ;
#111179=DIRECTION('',(1.,1.95511867169517E-16,0.)) ;
#111180=DIRECTION('',(1.95511867169517E-16,-1.,0.)) ;
#111181=DIRECTION('',(-1.,1.06642836637919E-16,0.)) ;
#111182=DIRECTION('center_axis',(6.96951553037899E-18,0.707106781186549,
0.707106781186546)) ;
#111183=DIRECTION('ref_axis',(-8.6424177776148E-34,-0.707106781186546,0.707106781186549)) ;
#111184=DIRECTION('',(-0.577350269189625,0.577350269189625,-0.577350269189627)) ;
#111185=DIRECTION('',(1.,-9.85638338623186E-18,0.)) ;
#111186=DIRECTION('',(-0.577350269189625,-0.577350269189625,0.577350269189627)) ;
#111187=DIRECTION('',(-1.,7.70371977754894E-34,9.8563833862319E-18)) ;
#111188=DIRECTION('center_axis',(6.96951553037899E-18,0.707106781186549,
-0.707106781186546)) ;
#111189=DIRECTION('ref_axis',(8.6424177776148E-34,0.707106781186546,0.707106781186549)) ;
#111190=DIRECTION('',(0.577350269189625,0.577350269189625,0.577350269189627)) ;
#111191=DIRECTION('',(-1.,9.85638338623186E-18,0.)) ;
#111192=DIRECTION('',(0.577350269189625,-0.577350269189625,-0.577350269189627)) ;
#111193=DIRECTION('',(1.,-7.70371977754894E-34,9.8563833862319E-18)) ;
#111194=DIRECTION('center_axis',(-0.707106781186548,-1.38247767078009E-16,
0.707106781186547)) ;
#111195=DIRECTION('ref_axis',(0.707106781186547,8.815972061965E-34,0.707106781186548)) ;
#111196=DIRECTION('',(-0.577350269189625,-0.577350269189626,-0.577350269189626)) ;
#111197=DIRECTION('',(-1.95511867169517E-16,1.,0.)) ;
#111198=DIRECTION('',(0.577350269189625,-0.577350269189626,0.577350269189626)) ;
#111199=DIRECTION('',(0.,-1.,-1.95511867169518E-16)) ;
#111200=DIRECTION('center_axis',(-0.707106781186548,-1.38247767078009E-16,
-0.707106781186547)) ;
#111201=DIRECTION('ref_axis',(-0.707106781186547,-8.815972061965E-34,0.707106781186548)) ;
#111202=DIRECTION('',(-0.577350269189625,0.577350269189626,0.577350269189626)) ;
#111203=DIRECTION('',(1.95511867169517E-16,-1.,0.)) ;
#111204=DIRECTION('',(0.577350269189625,0.577350269189626,-0.577350269189626)) ;
#111205=DIRECTION('',(0.,1.,-1.95511867169518E-16)) ;
#111206=DIRECTION('center_axis',(0.577350269189625,0.577350269189625,-0.577350269189628)) ;
#111207=DIRECTION('ref_axis',(-0.707106781186549,-3.37019869349033E-16,
-0.707106781186546)) ;
#111208=DIRECTION('center_axis',(-0.577350269189625,-0.577350269189625,
0.577350269189628)) ;
#111209=DIRECTION('ref_axis',(-0.707106781186549,-5.7623968423712E-16,-0.707106781186546)) ;
#111210=DIRECTION('center_axis',(-0.577350269189625,-0.577350269189625,
0.577350269189627)) ;
#111211=DIRECTION('ref_axis',(0.707106781186549,-3.64954285315842E-16,0.707106781186546)) ;
#111212=DIRECTION('center_axis',(0.,0.,-1.)) ;
#111213=DIRECTION('ref_axis',(-1.,0.,0.)) ;
#111214=DIRECTION('center_axis',(0.,0.,1.)) ;
#111215=DIRECTION('ref_axis',(-1.,0.,0.)) ;
#111216=DIRECTION('center_axis',(0.,0.,-1.)) ;
#111217=DIRECTION('ref_axis',(-1.,0.,0.)) ;
#111218=DIRECTION('center_axis',(2.08166817117218E-16,1.,0.)) ;
#111219=DIRECTION('ref_axis',(1.,0.,0.)) ;
#111220=DIRECTION('center_axis',(-1.,0.,-3.25824851045218E-15)) ;
#111221=DIRECTION('ref_axis',(3.25824851045218E-15,0.,-1.)) ;
#111222=DIRECTION('center_axis',(2.71050543121376E-15,2.71050543121375E-15,
1.)) ;
#111223=DIRECTION('ref_axis',(-1.,-1.07215069759461E-44,2.71050543121376E-15)) ;
#111224=DIRECTION('center_axis',(-0.577350269189625,-0.577350269189625,
-0.577350269189628)) ;
#111225=DIRECTION('ref_axis',(-0.707106781186549,-3.37019869349033E-16,
0.707106781186546)) ;
#111226=DIRECTION('center_axis',(-0.577350269189625,-0.577350269189625,
-0.577350269189628)) ;
#111227=DIRECTION('ref_axis',(-0.707106781186549,-3.64775444964662E-16,
0.707106781186546)) ;
#111228=DIRECTION('center_axis',(-0.577350269189625,-0.577350269189625,
-0.577350269189628)) ;
#111229=DIRECTION('ref_axis',(-0.707106781186549,-3.37019869349033E-16,
0.707106781186546)) ;
#111230=DIRECTION('center_axis',(0.,0.,-1.)) ;
#111231=DIRECTION('ref_axis',(-1.,0.,0.)) ;
#111232=DIRECTION('center_axis',(6.99565121361789E-15,0.,1.)) ;
#111233=DIRECTION('ref_axis',(1.,0.,-6.99565121361789E-15)) ;
#111234=DIRECTION('center_axis',(-1.,0.,9.8563833862319E-18)) ;
#111235=DIRECTION('ref_axis',(9.8563833862319E-18,0.,1.)) ;
#111236=DIRECTION('center_axis',(-1.,-1.62630325872825E-15,1.62630325872826E-15)) ;
#111237=DIRECTION('ref_axis',(1.62630325872826E-15,2.45227231256843E-45,
1.)) ;
#111238=DIRECTION('center_axis',(2.08166817117218E-16,1.,0.)) ;
#111239=DIRECTION('ref_axis',(1.,0.,0.)) ;
#111240=DIRECTION('center_axis',(-1.,-5.82758667710957E-15,-5.82758667710959E-15)) ;
#111241=DIRECTION('ref_axis',(5.82758667710959E-15,3.92363570010949E-44,
-1.)) ;
#111242=DIRECTION('center_axis',(2.08166817117218E-16,1.,0.)) ;
#111243=DIRECTION('ref_axis',(1.,0.,0.)) ;
#111244=DIRECTION('center_axis',(-0.577350269189626,0.577350269189625,-0.577350269189627)) ;
#111245=DIRECTION('ref_axis',(0.707106781186548,-3.45739798078984E-16,-0.707106781186547)) ;
#111246=DIRECTION('center_axis',(-1.91661677085422E-15,0.,1.)) ;
#111247=DIRECTION('ref_axis',(-1.,0.,-1.91661677085422E-15)) ;
#111248=DIRECTION('center_axis',(-1.,0.,-9.8563833862319E-18)) ;
#111249=DIRECTION('ref_axis',(-9.8563833862319E-18,0.,1.)) ;
#111250=DIRECTION('center_axis',(-1.,0.,-2.77909431773862E-15)) ;
#111251=DIRECTION('ref_axis',(-2.77909431773862E-15,0.,1.)) ;
#111252=DIRECTION('center_axis',(0.,0.,-1.)) ;
#111253=DIRECTION('ref_axis',(-1.,0.,0.)) ;
#111254=DIRECTION('center_axis',(1.49077798716757E-15,-1.49077798716756E-15,
1.)) ;
#111255=DIRECTION('ref_axis',(1.,-2.47036158412635E-45,-1.49077798716757E-15)) ;
#111256=DIRECTION('center_axis',(0.577350269189625,-0.577350269189625,0.577350269189628)) ;
#111257=DIRECTION('ref_axis',(0.707106781186549,-3.37019869349033E-16,-0.707106781186546)) ;
#111258=DIRECTION('center_axis',(0.577350269189625,-0.577350269189625,0.577350269189628)) ;
#111259=DIRECTION('ref_axis',(0.707106781186549,-3.64775444964662E-16,-0.707106781186546)) ;
#111260=DIRECTION('center_axis',(2.08166817117218E-16,1.,0.)) ;
#111261=DIRECTION('ref_axis',(1.,0.,0.)) ;
#111262=DIRECTION('center_axis',(-0.577350269189626,0.577350269189625,0.577350269189627)) ;
#111263=DIRECTION('ref_axis',(-0.707106781186549,-1.20060139371205E-15,
-0.707106781186546)) ;
#111264=DIRECTION('center_axis',(0.,0.,-1.)) ;
#111265=DIRECTION('ref_axis',(-1.,0.,0.)) ;
#111266=DIRECTION('center_axis',(0.,0.,1.)) ;
#111267=DIRECTION('ref_axis',(-1.,0.,0.)) ;
#111268=DIRECTION('center_axis',(0.,0.,-1.)) ;
#111269=DIRECTION('ref_axis',(-1.,0.,0.)) ;
#111270=DIRECTION('center_axis',(-0.577350269189625,0.577350269189625,0.577350269189628)) ;
#111271=DIRECTION('ref_axis',(0.707106781186549,-3.64775444964662E-16,0.707106781186546)) ;
#111272=DIRECTION('center_axis',(0.577350269189625,-0.577350269189625,-0.577350269189628)) ;
#111273=DIRECTION('ref_axis',(0.707106781186549,-4.84385352408706E-16,0.707106781186546)) ;
#111274=DIRECTION('center_axis',(-0.577350269189625,0.577350269189626,-0.577350269189626)) ;
#111275=DIRECTION('ref_axis',(5.0289788758123E-16,0.707106781186548,0.707106781186547)) ;
#111276=DIRECTION('center_axis',(0.577350269189625,-0.577350269189626,0.577350269189626)) ;
#111277=DIRECTION('ref_axis',(5.0289788758123E-16,0.707106781186548,0.707106781186547)) ;
#111278=DIRECTION('center_axis',(0.577350269189625,-0.577350269189627,0.577350269189626)) ;
#111279=DIRECTION('ref_axis',(-1.3856936129729E-16,-0.707106781186547,-0.707106781186548)) ;
#111280=DIRECTION('center_axis',(0.,0.,-1.)) ;
#111281=DIRECTION('ref_axis',(-1.,0.,0.)) ;
#111282=DIRECTION('center_axis',(0.,0.,1.)) ;
#111283=DIRECTION('ref_axis',(-1.,-5.42101086242751E-15,0.)) ;
#111284=DIRECTION('center_axis',(0.,0.,-1.)) ;
#111285=DIRECTION('ref_axis',(-1.,0.,0.)) ;
#111286=DIRECTION('center_axis',(0.,1.,0.)) ;
#111287=DIRECTION('ref_axis',(1.,0.,0.)) ;
#111288=DIRECTION('center_axis',(0.,-1.,-4.79154192713555E-15)) ;
#111289=DIRECTION('ref_axis',(0.,-4.79154192713555E-15,1.)) ;
#111290=DIRECTION('center_axis',(-3.18484388167616E-15,3.18484388167617E-15,
1.)) ;
#111291=DIRECTION('ref_axis',(-4.20389539297445E-45,1.,-3.18484388167617E-15)) ;
#111292=DIRECTION('center_axis',(0.577350269189625,-0.577350269189626,-0.577350269189626)) ;
#111293=DIRECTION('ref_axis',(5.0289788758123E-16,0.707106781186548,-0.707106781186547)) ;
#111294=DIRECTION('center_axis',(0.577350269189625,-0.577350269189626,-0.577350269189626)) ;
#111295=DIRECTION('ref_axis',(5.0289788758123E-16,0.707106781186548,-0.707106781186547)) ;
#111296=DIRECTION('center_axis',(0.577350269189625,-0.577350269189626,-0.577350269189626)) ;
#111297=DIRECTION('ref_axis',(5.0289788758123E-16,0.707106781186548,-0.707106781186547)) ;
#111298=DIRECTION('center_axis',(0.,0.,-1.)) ;
#111299=DIRECTION('ref_axis',(-1.,0.,0.)) ;
#111300=DIRECTION('center_axis',(0.,-2.87492515628133E-15,1.)) ;
#111301=DIRECTION('ref_axis',(0.,-1.,-2.87492515628133E-15)) ;
#111302=DIRECTION('center_axis',(0.,1.,1.95511867169518E-16)) ;
#111303=DIRECTION('ref_axis',(0.,-1.95511867169518E-16,1.)) ;
#111304=DIRECTION('center_axis',(2.71050543121375E-15,-1.,2.51884375412834E-15)) ;
#111305=DIRECTION('ref_axis',(1.,2.71050543121375E-15,2.80259692864963E-45)) ;
#111306=DIRECTION('center_axis',(0.,1.,0.)) ;
#111307=DIRECTION('ref_axis',(1.,0.,0.)) ;
#111308=DIRECTION('center_axis',(-2.30392961653169E-15,-1.,2.49559129361712E-15)) ;
#111309=DIRECTION('ref_axis',(-2.67860162145163E-32,2.49559129361712E-15,
1.)) ;
#111310=DIRECTION('center_axis',(0.,1.,0.)) ;
#111311=DIRECTION('ref_axis',(1.,0.,0.)) ;
#111312=DIRECTION('center_axis',(-0.577350269189625,-0.577350269189626,
-0.577350269189627)) ;
#111313=DIRECTION('ref_axis',(-8.18676000863892E-15,-0.707106781186544,
0.707106781186551)) ;
#111314=DIRECTION('center_axis',(0.,-4.50404941150742E-15,1.)) ;
#111315=DIRECTION('ref_axis',(0.,1.,4.50404941150742E-15)) ;
#111316=DIRECTION('center_axis',(0.,1.,-1.95511867169518E-16)) ;
#111317=DIRECTION('ref_axis',(0.,1.95511867169518E-16,1.)) ;
#111318=DIRECTION('center_axis',(0.,-1.,-2.10827844793964E-15)) ;
#111319=DIRECTION('ref_axis',(0.,2.10827844793964E-15,-1.)) ;
#111320=DIRECTION('center_axis',(0.,0.,-1.)) ;
#111321=DIRECTION('ref_axis',(-1.,0.,0.)) ;
#111322=DIRECTION('center_axis',(-6.77626357803439E-17,-6.7762635780344E-17,
1.)) ;
#111323=DIRECTION('ref_axis',(-1.3684555315672E-48,-1.,-6.7762635780344E-17)) ;
#111324=DIRECTION('center_axis',(0.577350269189625,0.577350269189626,0.577350269189627)) ;
#111325=DIRECTION('ref_axis',(-9.19305248608458E-17,-0.707106781186548,
0.707106781186547)) ;
#111326=DIRECTION('center_axis',(0.577350269189625,0.577350269189626,0.577350269189627)) ;
#111327=DIRECTION('ref_axis',(-9.19305248608458E-17,-0.707106781186548,
0.707106781186547)) ;
#111328=DIRECTION('center_axis',(0.,1.,0.)) ;
#111329=DIRECTION('ref_axis',(1.,0.,0.)) ;
#111330=DIRECTION('center_axis',(-0.577350269189624,-0.577350269189627,
0.577350269189626)) ;
#111331=DIRECTION('ref_axis',(-1.46369207068818E-16,0.707106781186547,0.707106781186548)) ;
#111332=DIRECTION('center_axis',(0.,0.,-1.)) ;
#111333=DIRECTION('ref_axis',(-1.,0.,0.)) ;
#111334=DIRECTION('center_axis',(0.,0.,1.)) ;
#111335=DIRECTION('ref_axis',(-1.,1.0842021724855E-15,0.)) ;
#111336=DIRECTION('center_axis',(0.,0.,-1.)) ;
#111337=DIRECTION('ref_axis',(-1.,0.,0.)) ;
#111338=DIRECTION('center_axis',(-0.577350269189625,-0.577350269189626,
0.577350269189627)) ;
#111339=DIRECTION('ref_axis',(-1.51735478582867E-16,-0.707106781186548,
-0.707106781186547)) ;
#111340=DIRECTION('center_axis',(0.577350269189625,0.577350269189626,-0.577350269189627)) ;
#111341=DIRECTION('ref_axis',(-8.00734514747286E-15,-0.707106781186544,
-0.707106781186551)) ;
#111342=DIRECTION('center_axis',(0.,0.,1.)) ;
#111343=DIRECTION('ref_axis',(1.,0.,0.)) ;
#111344=DIRECTION('center_axis',(0.,-1.,0.)) ;
#111345=DIRECTION('ref_axis',(0.,0.,-1.)) ;
#111346=DIRECTION('center_axis',(9.85638338623186E-18,1.,0.)) ;
#111347=DIRECTION('ref_axis',(-1.,9.85638338623186E-18,0.)) ;
#111348=DIRECTION('center_axis',(0.,-1.,0.)) ;
#111349=DIRECTION('ref_axis',(0.,0.,-1.)) ;
#111350=DIRECTION('center_axis',(0.,1.,0.)) ;
#111351=DIRECTION('ref_axis',(1.,0.,0.)) ;
#111352=DIRECTION('center_axis',(-1.,0.,0.)) ;
#111353=DIRECTION('ref_axis',(0.,0.,1.)) ;
#111354=DIRECTION('center_axis',(1.,-9.85638338623186E-18,0.)) ;
#111355=DIRECTION('ref_axis',(9.85638338623186E-18,1.,0.)) ;
#111356=DIRECTION('center_axis',(-1.,0.,0.)) ;
#111357=DIRECTION('ref_axis',(0.,0.,1.)) ;
#111358=DIRECTION('center_axis',(0.,1.,0.)) ;
#111359=DIRECTION('ref_axis',(1.,0.,0.)) ;
#111360=DIRECTION('center_axis',(0.,1.,0.)) ;
#111361=DIRECTION('ref_axis',(0.,0.,1.)) ;
#111362=DIRECTION('center_axis',(-9.85638338623186E-18,-1.,0.)) ;
#111363=DIRECTION('ref_axis',(1.,-9.85638338623186E-18,0.)) ;
#111364=DIRECTION('center_axis',(0.,1.,0.)) ;
#111365=DIRECTION('ref_axis',(0.,0.,1.)) ;
#111366=DIRECTION('center_axis',(0.,0.,1.)) ;
#111367=DIRECTION('ref_axis',(1.,0.,0.)) ;
#111368=DIRECTION('center_axis',(0.,0.,1.)) ;
#111369=DIRECTION('ref_axis',(1.,0.,0.)) ;
#111370=DIRECTION('center_axis',(0.,-1.,0.)) ;
#111371=DIRECTION('ref_axis',(0.,0.,-1.)) ;
#111372=DIRECTION('center_axis',(-9.85638338623186E-18,-1.,0.)) ;
#111373=DIRECTION('ref_axis',(1.,-9.85638338623186E-18,0.)) ;
#111374=DIRECTION('center_axis',(0.,-1.,0.)) ;
#111375=DIRECTION('ref_axis',(0.,0.,-1.)) ;
#111376=DIRECTION('center_axis',(0.,1.,0.)) ;
#111377=DIRECTION('ref_axis',(1.,0.,0.)) ;
#111378=DIRECTION('center_axis',(1.,-7.66646708341686E-16,0.)) ;
#111379=DIRECTION('ref_axis',(7.66646708341686E-16,1.,0.)) ;
#111380=DIRECTION('center_axis',(1.,-9.85638338623186E-18,0.)) ;
#111381=DIRECTION('ref_axis',(9.85638338623186E-18,1.,0.)) ;
#111382=DIRECTION('center_axis',(1.,0.,0.)) ;
#111383=DIRECTION('ref_axis',(0.,0.,-1.)) ;
#111384=DIRECTION('center_axis',(0.,1.,0.)) ;
#111385=DIRECTION('ref_axis',(1.,0.,0.)) ;
#111386=DIRECTION('center_axis',(0.,1.,0.)) ;
#111387=DIRECTION('ref_axis',(0.,0.,1.)) ;
#111388=DIRECTION('center_axis',(-9.85638338623186E-18,-1.,0.)) ;
#111389=DIRECTION('ref_axis',(1.,-9.85638338623186E-18,0.)) ;
#111390=DIRECTION('center_axis',(0.,1.,0.)) ;
#111391=DIRECTION('ref_axis',(0.,0.,1.)) ;
#111392=DIRECTION('center_axis',(0.,0.,1.)) ;
#111393=DIRECTION('ref_axis',(1.,0.,0.)) ;
#111394=DIRECTION('center_axis',(-1.,-1.95511867169517E-16,0.)) ;
#111395=DIRECTION('ref_axis',(1.95511867169517E-16,-1.,0.)) ;
#111396=DIRECTION('center_axis',(1.,0.,0.)) ;
#111397=DIRECTION('ref_axis',(0.,0.,-1.)) ;
#111398=DIRECTION('center_axis',(0.,1.,0.)) ;
#111399=DIRECTION('ref_axis',(1.,0.,0.)) ;
#111400=DIRECTION('center_axis',(-2.29994012502506E-15,-1.,0.)) ;
#111401=DIRECTION('ref_axis',(1.,-2.29994012502506E-15,0.)) ;
#111402=DIRECTION('center_axis',(-1.95511867169517E-16,1.,0.)) ;
#111403=DIRECTION('ref_axis',(-1.,-1.95511867169517E-16,0.)) ;
#111404=DIRECTION('center_axis',(0.,-1.,0.)) ;
#111405=DIRECTION('ref_axis',(0.,0.,-1.)) ;
#111406=DIRECTION('center_axis',(0.,1.,0.)) ;
#111407=DIRECTION('ref_axis',(1.,0.,0.)) ;
#111408=DIRECTION('center_axis',(-1.,0.,0.)) ;
#111409=DIRECTION('ref_axis',(0.,0.,1.)) ;
#111410=DIRECTION('center_axis',(1.,-1.06642836637918E-16,0.)) ;
#111411=DIRECTION('ref_axis',(1.06642836637918E-16,1.,0.)) ;
#111412=DIRECTION('center_axis',(1.,1.95511867169517E-16,0.)) ;
#111413=DIRECTION('ref_axis',(-1.95511867169517E-16,1.,0.)) ;
#111414=DIRECTION('center_axis',(1.,0.,0.)) ;
#111415=DIRECTION('ref_axis',(0.,0.,-1.)) ;
#111416=DIRECTION('center_axis',(0.,1.,0.)) ;
#111417=DIRECTION('ref_axis',(1.,0.,0.)) ;
#111418=DIRECTION('center_axis',(2.29994012502506E-15,-1.,0.)) ;
#111419=DIRECTION('ref_axis',(1.,2.29994012502506E-15,0.)) ;
#111420=DIRECTION('center_axis',(-1.95511867169517E-16,1.,0.)) ;
#111421=DIRECTION('ref_axis',(-1.,-1.95511867169517E-16,0.)) ;
#111422=DIRECTION('center_axis',(0.,-1.,0.)) ;
#111423=DIRECTION('ref_axis',(0.,0.,-1.)) ;
#111424=DIRECTION('center_axis',(-1.,1.06642836637918E-16,0.)) ;
#111425=DIRECTION('ref_axis',(-1.06642836637918E-16,-1.,0.)) ;
#111426=DIRECTION('center_axis',(1.,0.,0.)) ;
#111427=DIRECTION('ref_axis',(0.,0.,-1.)) ;
#111428=DIRECTION('center_axis',(0.,1.,0.)) ;
#111429=DIRECTION('ref_axis',(1.,0.,0.)) ;
#111430=DIRECTION('center_axis',(-1.,-1.53063836115601E-16,0.)) ;
#111431=DIRECTION('ref_axis',(1.53063836115601E-16,-1.,0.)) ;
#111432=DIRECTION('',(0.,0.,1.)) ;
#111433=DIRECTION('',(-1.53063836115601E-16,1.,-1.020425574104E-16)) ;
#111434=DIRECTION('',(0.,0.,-1.)) ;
#111435=DIRECTION('',(1.53063836115601E-16,-1.,5.10212787052002E-17)) ;
#111436=DIRECTION('',(0.,0.,1.)) ;
#111437=DIRECTION('',(-1.53063836115601E-16,1.,-1.30104260698261E-16)) ;
#111438=DIRECTION('center_axis',(-1.,-1.53063836115601E-16,0.)) ;
#111439=DIRECTION('ref_axis',(1.53063836115601E-16,-1.,0.)) ;
#111440=DIRECTION('',(0.,0.,1.)) ;
#111441=DIRECTION('center_axis',(-1.,-1.53063836115601E-16,0.)) ;
#111442=DIRECTION('ref_axis',(1.53063836115601E-16,-1.,0.)) ;
#111443=DIRECTION('',(1.53063836115601E-16,-1.,-1.30104260698261E-16)) ;
#111444=DIRECTION('center_axis',(-1.,-1.53063836115601E-16,0.)) ;
#111445=DIRECTION('ref_axis',(1.53063836115601E-16,-1.,0.)) ;
#111446=DIRECTION('',(0.,0.,1.)) ;
#111447=DIRECTION('',(-1.53063836115601E-16,1.,-1.020425574104E-16)) ;
#111448=DIRECTION('',(0.,0.,-1.)) ;
#111449=DIRECTION('',(1.53063836115601E-16,-1.,5.10212787052002E-17)) ;
#111450=DIRECTION('',(0.,0.,1.)) ;
#111451=DIRECTION('',(-1.53063836115601E-16,1.,-1.30104260698261E-16)) ;
#111452=DIRECTION('center_axis',(-1.,-1.53063836115601E-16,0.)) ;
#111453=DIRECTION('ref_axis',(1.53063836115601E-16,-1.,0.)) ;
#111454=DIRECTION('',(0.,0.,1.)) ;
#111455=DIRECTION('center_axis',(-1.,-1.53063836115601E-16,0.)) ;
#111456=DIRECTION('ref_axis',(1.53063836115601E-16,-1.,0.)) ;
#111457=DIRECTION('',(1.53063836115601E-16,-1.,-1.30104260698261E-16)) ;
#111458=DIRECTION('center_axis',(-1.,-1.53063836115601E-16,0.)) ;
#111459=DIRECTION('ref_axis',(1.53063836115601E-16,-1.,0.)) ;
#111460=DIRECTION('',(0.,0.,1.)) ;
#111461=DIRECTION('',(-1.53063836115601E-16,1.,-1.020425574104E-16)) ;
#111462=DIRECTION('',(0.,0.,-1.)) ;
#111463=DIRECTION('',(1.53063836115601E-16,-1.,5.10212787052002E-17)) ;
#111464=DIRECTION('',(0.,0.,1.)) ;
#111465=DIRECTION('',(-1.53063836115601E-16,1.,-1.30104260698261E-16)) ;
#111466=DIRECTION('center_axis',(-1.,-1.53063836115601E-16,0.)) ;
#111467=DIRECTION('ref_axis',(1.53063836115601E-16,-1.,0.)) ;
#111468=DIRECTION('',(0.,0.,1.)) ;
#111469=DIRECTION('center_axis',(-1.,-1.53063836115601E-16,0.)) ;
#111470=DIRECTION('ref_axis',(1.53063836115601E-16,-1.,0.)) ;
#111471=DIRECTION('',(1.53063836115601E-16,-1.,-1.30104260698261E-16)) ;
#111472=DIRECTION('center_axis',(-1.,-1.53063836115601E-16,0.)) ;
#111473=DIRECTION('ref_axis',(1.53063836115601E-16,-1.,0.)) ;
#111474=DIRECTION('',(0.,0.,1.)) ;
#111475=DIRECTION('',(-1.53063836115601E-16,1.,-1.020425574104E-16)) ;
#111476=DIRECTION('',(0.,0.,-1.)) ;
#111477=DIRECTION('',(1.53063836115601E-16,-1.,5.10212787052002E-17)) ;
#111478=DIRECTION('',(0.,0.,1.)) ;
#111479=DIRECTION('',(-1.53063836115601E-16,1.,-1.30104260698261E-16)) ;
#111480=DIRECTION('center_axis',(-1.,-1.53063836115601E-16,0.)) ;
#111481=DIRECTION('ref_axis',(1.53063836115601E-16,-1.,0.)) ;
#111482=DIRECTION('',(0.,0.,1.)) ;
#111483=DIRECTION('center_axis',(-1.,-1.53063836115601E-16,0.)) ;
#111484=DIRECTION('ref_axis',(1.53063836115601E-16,-1.,0.)) ;
#111485=DIRECTION('',(1.53063836115601E-16,-1.,-1.30104260698261E-16)) ;
#111486=DIRECTION('center_axis',(-1.,-1.53063836115601E-16,0.)) ;
#111487=DIRECTION('ref_axis',(1.53063836115601E-16,-1.,0.)) ;
#111488=DIRECTION('',(0.,0.,1.)) ;
#111489=DIRECTION('',(-1.53063836115601E-16,1.,-1.020425574104E-16)) ;
#111490=DIRECTION('',(0.,0.,-1.)) ;
#111491=DIRECTION('',(1.53063836115601E-16,-1.,5.10212787052002E-17)) ;
#111492=DIRECTION('',(0.,0.,1.)) ;
#111493=DIRECTION('',(-1.53063836115601E-16,1.,-1.30104260698261E-16)) ;
#111494=DIRECTION('center_axis',(-1.,-1.53063836115601E-16,0.)) ;
#111495=DIRECTION('ref_axis',(1.53063836115601E-16,-1.,0.)) ;
#111496=DIRECTION('',(0.,0.,1.)) ;
#111497=DIRECTION('center_axis',(-1.,-1.53063836115601E-16,0.)) ;
#111498=DIRECTION('ref_axis',(1.53063836115601E-16,-1.,0.)) ;
#111499=DIRECTION('',(1.53063836115601E-16,-1.,-1.30104260698261E-16)) ;
#111500=DIRECTION('center_axis',(-1.,-1.53063836115601E-16,0.)) ;
#111501=DIRECTION('ref_axis',(1.53063836115601E-16,-1.,0.)) ;
#111502=DIRECTION('',(0.,0.,1.)) ;
#111503=DIRECTION('',(-1.53063836115601E-16,1.,-1.020425574104E-16)) ;
#111504=DIRECTION('',(0.,0.,-1.)) ;
#111505=DIRECTION('',(1.53063836115601E-16,-1.,5.10212787052002E-17)) ;
#111506=DIRECTION('',(0.,0.,1.)) ;
#111507=DIRECTION('',(-1.53063836115601E-16,1.,-1.30104260698261E-16)) ;
#111508=DIRECTION('center_axis',(-1.,-1.53063836115601E-16,0.)) ;
#111509=DIRECTION('ref_axis',(1.53063836115601E-16,-1.,0.)) ;
#111510=DIRECTION('',(0.,0.,1.)) ;
#111511=DIRECTION('center_axis',(-1.,-1.53063836115601E-16,0.)) ;
#111512=DIRECTION('ref_axis',(1.53063836115601E-16,-1.,0.)) ;
#111513=DIRECTION('',(1.53063836115601E-16,-1.,-1.30104260698261E-16)) ;
#111514=DIRECTION('center_axis',(-1.,-1.53063836115601E-16,0.)) ;
#111515=DIRECTION('ref_axis',(1.53063836115601E-16,-1.,0.)) ;
#111516=DIRECTION('',(0.,0.,1.)) ;
#111517=DIRECTION('',(-1.53063836115601E-16,1.,-1.020425574104E-16)) ;
#111518=DIRECTION('',(0.,0.,-1.)) ;
#111519=DIRECTION('',(1.53063836115601E-16,-1.,5.10212787052002E-17)) ;
#111520=DIRECTION('',(0.,0.,1.)) ;
#111521=DIRECTION('',(-1.53063836115601E-16,1.,-1.30104260698261E-16)) ;
#111522=DIRECTION('center_axis',(-1.,-1.53063836115601E-16,0.)) ;
#111523=DIRECTION('ref_axis',(1.53063836115601E-16,-1.,0.)) ;
#111524=DIRECTION('',(0.,0.,1.)) ;
#111525=DIRECTION('center_axis',(-1.,-1.53063836115601E-16,0.)) ;
#111526=DIRECTION('ref_axis',(1.53063836115601E-16,-1.,0.)) ;
#111527=DIRECTION('',(1.53063836115601E-16,-1.,-1.30104260698261E-16)) ;
#111528=DIRECTION('center_axis',(-1.,-1.53063836115601E-16,0.)) ;
#111529=DIRECTION('ref_axis',(1.53063836115601E-16,-1.,0.)) ;
#111530=DIRECTION('',(0.,0.,1.)) ;
#111531=DIRECTION('',(-1.53063836115601E-16,1.,-1.020425574104E-16)) ;
#111532=DIRECTION('',(0.,0.,-1.)) ;
#111533=DIRECTION('',(1.53063836115601E-16,-1.,5.10212787052002E-17)) ;
#111534=DIRECTION('',(0.,0.,1.)) ;
#111535=DIRECTION('',(-1.53063836115601E-16,1.,-1.30104260698261E-16)) ;
#111536=DIRECTION('center_axis',(-1.,-1.53063836115601E-16,0.)) ;
#111537=DIRECTION('ref_axis',(1.53063836115601E-16,-1.,0.)) ;
#111538=DIRECTION('',(0.,0.,1.)) ;
#111539=DIRECTION('center_axis',(-1.,-1.53063836115601E-16,0.)) ;
#111540=DIRECTION('ref_axis',(1.53063836115601E-16,-1.,0.)) ;
#111541=DIRECTION('',(1.53063836115601E-16,-1.,-1.30104260698261E-16)) ;
#111542=DIRECTION('center_axis',(-1.,-1.53063836115601E-16,0.)) ;
#111543=DIRECTION('ref_axis',(1.53063836115601E-16,-1.,0.)) ;
#111544=DIRECTION('',(0.,0.,1.)) ;
#111545=DIRECTION('',(-1.53063836115601E-16,1.,-1.020425574104E-16)) ;
#111546=DIRECTION('',(0.,0.,-1.)) ;
#111547=DIRECTION('',(1.53063836115601E-16,-1.,5.10212787052002E-17)) ;
#111548=DIRECTION('',(0.,0.,1.)) ;
#111549=DIRECTION('',(-1.53063836115601E-16,1.,-1.30104260698261E-16)) ;
#111550=DIRECTION('center_axis',(-1.,-1.53063836115601E-16,0.)) ;
#111551=DIRECTION('ref_axis',(1.53063836115601E-16,-1.,0.)) ;
#111552=DIRECTION('',(0.,0.,1.)) ;
#111553=DIRECTION('center_axis',(-1.,-1.53063836115601E-16,0.)) ;
#111554=DIRECTION('ref_axis',(1.53063836115601E-16,-1.,0.)) ;
#111555=DIRECTION('',(1.53063836115601E-16,-1.,-1.30104260698261E-16)) ;
#111556=DIRECTION('center_axis',(-1.53063836115601E-16,1.,0.)) ;
#111557=DIRECTION('ref_axis',(-1.,-1.53063836115601E-16,0.)) ;
#111558=DIRECTION('',(-1.,-1.53063836115601E-16,2.73691106313441E-48)) ;
#111559=DIRECTION('',(0.,0.,-1.)) ;
#111560=DIRECTION('',(1.,1.53063836115601E-16,-1.53236300070382E-33)) ;
#111561=DIRECTION('',(0.,0.,1.)) ;
#111562=DIRECTION('center_axis',(1.99142572374599E-32,-1.30104260698261E-16,
-1.)) ;
#111563=DIRECTION('ref_axis',(0.,1.,-1.30104260698261E-16)) ;
#111564=DIRECTION('',(-1.,-1.53063836115601E-16,2.73691106313441E-48)) ;
#111565=DIRECTION('',(1.53063836115601E-16,-1.,1.30104260698261E-16)) ;
#111566=DIRECTION('',(1.,1.53063836115601E-16,-2.73691106313441E-48)) ;
#111567=DIRECTION('center_axis',(-1.53063836115601E-16,1.,0.)) ;
#111568=DIRECTION('ref_axis',(-1.,-1.53063836115601E-16,0.)) ;
#111569=DIRECTION('',(-1.,-1.53063836115601E-16,-2.73691106313441E-48)) ;
#111570=DIRECTION('',(0.,0.,-1.)) ;
#111571=DIRECTION('',(1.,1.53063836115601E-16,-2.73691106313441E-48)) ;
#111572=DIRECTION('',(0.,0.,1.)) ;
#111573=DIRECTION('center_axis',(1.99142572374599E-32,-1.30104260698261E-16,
1.)) ;
#111574=DIRECTION('ref_axis',(0.,-1.,-1.30104260698261E-16)) ;
#111575=DIRECTION('',(-1.,-1.53063836115601E-16,-2.73691106313441E-48)) ;
#111576=DIRECTION('',(-1.53063836115601E-16,1.,1.30104260698261E-16)) ;
#111577=DIRECTION('',(1.,1.53063836115601E-16,2.73691106313441E-48)) ;
#111578=DIRECTION('',(2.16840434497101E-16,-1.,-1.30104260698261E-16)) ;
#111579=DIRECTION('center_axis',(-1.53063836115601E-16,1.,0.)) ;
#111580=DIRECTION('ref_axis',(-1.,-1.53063836115601E-16,0.)) ;
#111581=DIRECTION('',(-1.,-1.53063836115601E-16,3.06472600140763E-33)) ;
#111582=DIRECTION('',(0.,0.,-1.)) ;
#111583=DIRECTION('',(1.,1.53063836115601E-16,2.73691106313441E-48)) ;
#111584=DIRECTION('',(0.,0.,1.)) ;
#111585=DIRECTION('center_axis',(-1.53063836115601E-16,1.,0.)) ;
#111586=DIRECTION('ref_axis',(-1.,-1.53063836115601E-16,0.)) ;
#111587=DIRECTION('',(-1.,-1.53063836115601E-16,2.73691106313441E-48)) ;
#111588=DIRECTION('',(0.,0.,-1.)) ;
#111589=DIRECTION('',(1.,1.53063836115601E-16,-1.53236300070382E-33)) ;
#111590=DIRECTION('',(0.,0.,1.)) ;
#111591=DIRECTION('center_axis',(1.99142572374599E-32,-1.30104260698261E-16,
-1.)) ;
#111592=DIRECTION('ref_axis',(0.,1.,-1.30104260698261E-16)) ;
#111593=DIRECTION('',(-1.,-1.53063836115601E-16,2.73691106313441E-48)) ;
#111594=DIRECTION('',(1.53063836115601E-16,-1.,1.30104260698261E-16)) ;
#111595=DIRECTION('',(1.,1.53063836115601E-16,-2.73691106313441E-48)) ;
#111596=DIRECTION('center_axis',(-1.53063836115601E-16,1.,0.)) ;
#111597=DIRECTION('ref_axis',(-1.,-1.53063836115601E-16,0.)) ;
#111598=DIRECTION('',(-1.,-1.53063836115601E-16,-2.73691106313441E-48)) ;
#111599=DIRECTION('',(0.,0.,-1.)) ;
#111600=DIRECTION('',(1.,1.53063836115601E-16,-2.73691106313441E-48)) ;
#111601=DIRECTION('',(0.,0.,1.)) ;
#111602=DIRECTION('center_axis',(1.99142572374599E-32,-1.30104260698261E-16,
1.)) ;
#111603=DIRECTION('ref_axis',(0.,-1.,-1.30104260698261E-16)) ;
#111604=DIRECTION('',(-1.,-1.53063836115601E-16,-2.73691106313441E-48)) ;
#111605=DIRECTION('',(-1.53063836115601E-16,1.,1.30104260698261E-16)) ;
#111606=DIRECTION('',(1.,1.53063836115601E-16,2.73691106313441E-48)) ;
#111607=DIRECTION('',(2.16840434497101E-16,-1.,-1.30104260698261E-16)) ;
#111608=DIRECTION('center_axis',(-1.53063836115601E-16,1.,0.)) ;
#111609=DIRECTION('ref_axis',(-1.,-1.53063836115601E-16,0.)) ;
#111610=DIRECTION('',(-1.,-1.53063836115601E-16,3.06472600140763E-33)) ;
#111611=DIRECTION('',(0.,0.,-1.)) ;
#111612=DIRECTION('',(1.,1.53063836115601E-16,2.73691106313441E-48)) ;
#111613=DIRECTION('',(0.,0.,1.)) ;
#111614=DIRECTION('center_axis',(-1.53063836115601E-16,1.,0.)) ;
#111615=DIRECTION('ref_axis',(-1.,-1.53063836115601E-16,0.)) ;
#111616=DIRECTION('',(-1.,-1.53063836115601E-16,2.73691106313441E-48)) ;
#111617=DIRECTION('',(0.,0.,-1.)) ;
#111618=DIRECTION('',(1.,1.53063836115601E-16,-1.53236300070382E-33)) ;
#111619=DIRECTION('',(0.,0.,1.)) ;
#111620=DIRECTION('center_axis',(1.99142572374599E-32,-1.30104260698261E-16,
-1.)) ;
#111621=DIRECTION('ref_axis',(0.,1.,-1.30104260698261E-16)) ;
#111622=DIRECTION('',(-1.,-1.53063836115601E-16,2.73691106313441E-48)) ;
#111623=DIRECTION('',(1.53063836115601E-16,-1.,1.30104260698261E-16)) ;
#111624=DIRECTION('',(1.,1.53063836115601E-16,-2.73691106313441E-48)) ;
#111625=DIRECTION('center_axis',(-1.53063836115601E-16,1.,0.)) ;
#111626=DIRECTION('ref_axis',(-1.,-1.53063836115601E-16,0.)) ;
#111627=DIRECTION('',(-1.,-1.53063836115601E-16,-2.73691106313441E-48)) ;
#111628=DIRECTION('',(0.,0.,-1.)) ;
#111629=DIRECTION('',(1.,1.53063836115601E-16,-2.73691106313441E-48)) ;
#111630=DIRECTION('',(0.,0.,1.)) ;
#111631=DIRECTION('center_axis',(1.99142572374599E-32,-1.30104260698261E-16,
1.)) ;
#111632=DIRECTION('ref_axis',(0.,-1.,-1.30104260698261E-16)) ;
#111633=DIRECTION('',(-1.,-1.53063836115601E-16,-2.73691106313441E-48)) ;
#111634=DIRECTION('',(-1.53063836115601E-16,1.,1.30104260698261E-16)) ;
#111635=DIRECTION('',(1.,1.53063836115601E-16,2.73691106313441E-48)) ;
#111636=DIRECTION('',(2.16840434497101E-16,-1.,-1.30104260698261E-16)) ;
#111637=DIRECTION('center_axis',(-1.53063836115601E-16,1.,0.)) ;
#111638=DIRECTION('ref_axis',(-1.,-1.53063836115601E-16,0.)) ;
#111639=DIRECTION('',(-1.,-1.53063836115601E-16,3.06472600140763E-33)) ;
#111640=DIRECTION('',(0.,0.,-1.)) ;
#111641=DIRECTION('',(1.,1.53063836115601E-16,2.73691106313441E-48)) ;
#111642=DIRECTION('',(0.,0.,1.)) ;
#111643=DIRECTION('center_axis',(-1.53063836115601E-16,1.,0.)) ;
#111644=DIRECTION('ref_axis',(-1.,-1.53063836115601E-16,0.)) ;
#111645=DIRECTION('',(-1.,-1.53063836115601E-16,2.73691106313441E-48)) ;
#111646=DIRECTION('',(0.,0.,-1.)) ;
#111647=DIRECTION('',(1.,1.53063836115601E-16,-1.53236300070382E-33)) ;
#111648=DIRECTION('',(0.,0.,1.)) ;
#111649=DIRECTION('center_axis',(1.99142572374599E-32,-1.30104260698261E-16,
-1.)) ;
#111650=DIRECTION('ref_axis',(0.,1.,-1.30104260698261E-16)) ;
#111651=DIRECTION('',(-1.,-1.53063836115601E-16,2.73691106313441E-48)) ;
#111652=DIRECTION('',(1.53063836115601E-16,-1.,1.30104260698261E-16)) ;
#111653=DIRECTION('',(1.,1.53063836115601E-16,-2.73691106313441E-48)) ;
#111654=DIRECTION('center_axis',(-1.53063836115601E-16,1.,0.)) ;
#111655=DIRECTION('ref_axis',(-1.,-1.53063836115601E-16,0.)) ;
#111656=DIRECTION('',(-1.,-1.53063836115601E-16,-2.73691106313441E-48)) ;
#111657=DIRECTION('',(0.,0.,-1.)) ;
#111658=DIRECTION('',(1.,1.53063836115601E-16,-2.73691106313441E-48)) ;
#111659=DIRECTION('',(0.,0.,1.)) ;
#111660=DIRECTION('center_axis',(1.99142572374599E-32,-1.30104260698261E-16,
1.)) ;
#111661=DIRECTION('ref_axis',(0.,-1.,-1.30104260698261E-16)) ;
#111662=DIRECTION('',(-1.,-1.53063836115601E-16,-2.73691106313441E-48)) ;
#111663=DIRECTION('',(-1.53063836115601E-16,1.,1.30104260698261E-16)) ;
#111664=DIRECTION('',(1.,1.53063836115601E-16,2.73691106313441E-48)) ;
#111665=DIRECTION('',(2.16840434497101E-16,-1.,-1.30104260698261E-16)) ;
#111666=DIRECTION('center_axis',(-1.53063836115601E-16,1.,0.)) ;
#111667=DIRECTION('ref_axis',(-1.,-1.53063836115601E-16,0.)) ;
#111668=DIRECTION('',(-1.,-1.53063836115601E-16,3.06472600140763E-33)) ;
#111669=DIRECTION('',(0.,0.,-1.)) ;
#111670=DIRECTION('',(1.,1.53063836115601E-16,2.73691106313441E-48)) ;
#111671=DIRECTION('',(0.,0.,1.)) ;
#111672=DIRECTION('center_axis',(-1.53063836115601E-16,1.,0.)) ;
#111673=DIRECTION('ref_axis',(-1.,-1.53063836115601E-16,0.)) ;
#111674=DIRECTION('',(-1.,-1.53063836115601E-16,2.73691106313441E-48)) ;
#111675=DIRECTION('',(0.,0.,-1.)) ;
#111676=DIRECTION('',(1.,1.53063836115601E-16,-1.53236300070382E-33)) ;
#111677=DIRECTION('',(0.,0.,1.)) ;
#111678=DIRECTION('center_axis',(1.99142572374599E-32,-1.30104260698261E-16,
-1.)) ;
#111679=DIRECTION('ref_axis',(0.,1.,-1.30104260698261E-16)) ;
#111680=DIRECTION('',(-1.,-1.53063836115601E-16,2.73691106313441E-48)) ;
#111681=DIRECTION('',(1.53063836115601E-16,-1.,1.30104260698261E-16)) ;
#111682=DIRECTION('',(1.,1.53063836115601E-16,-2.73691106313441E-48)) ;
#111683=DIRECTION('center_axis',(-1.53063836115601E-16,1.,0.)) ;
#111684=DIRECTION('ref_axis',(-1.,-1.53063836115601E-16,0.)) ;
#111685=DIRECTION('',(-1.,-1.53063836115601E-16,-2.73691106313441E-48)) ;
#111686=DIRECTION('',(0.,0.,-1.)) ;
#111687=DIRECTION('',(1.,1.53063836115601E-16,-2.73691106313441E-48)) ;
#111688=DIRECTION('',(0.,0.,1.)) ;
#111689=DIRECTION('center_axis',(1.99142572374599E-32,-1.30104260698261E-16,
1.)) ;
#111690=DIRECTION('ref_axis',(0.,-1.,-1.30104260698261E-16)) ;
#111691=DIRECTION('',(-1.,-1.53063836115601E-16,-2.73691106313441E-48)) ;
#111692=DIRECTION('',(-1.53063836115601E-16,1.,1.30104260698261E-16)) ;
#111693=DIRECTION('',(1.,1.53063836115601E-16,2.73691106313441E-48)) ;
#111694=DIRECTION('',(2.16840434497101E-16,-1.,-1.30104260698261E-16)) ;
#111695=DIRECTION('center_axis',(-1.53063836115601E-16,1.,0.)) ;
#111696=DIRECTION('ref_axis',(-1.,-1.53063836115601E-16,0.)) ;
#111697=DIRECTION('',(-1.,-1.53063836115601E-16,3.06472600140763E-33)) ;
#111698=DIRECTION('',(0.,0.,-1.)) ;
#111699=DIRECTION('',(1.,1.53063836115601E-16,2.73691106313441E-48)) ;
#111700=DIRECTION('',(0.,0.,1.)) ;
#111701=DIRECTION('center_axis',(-1.53063836115601E-16,1.,0.)) ;
#111702=DIRECTION('ref_axis',(-1.,-1.53063836115601E-16,0.)) ;
#111703=DIRECTION('',(-1.,-1.53063836115601E-16,2.73691106313441E-48)) ;
#111704=DIRECTION('',(0.,0.,-1.)) ;
#111705=DIRECTION('',(1.,1.53063836115601E-16,-1.53236300070382E-33)) ;
#111706=DIRECTION('',(0.,0.,1.)) ;
#111707=DIRECTION('center_axis',(1.99142572374599E-32,-1.30104260698261E-16,
-1.)) ;
#111708=DIRECTION('ref_axis',(0.,1.,-1.30104260698261E-16)) ;
#111709=DIRECTION('',(-1.,-1.53063836115601E-16,2.73691106313441E-48)) ;
#111710=DIRECTION('',(1.53063836115601E-16,-1.,1.30104260698261E-16)) ;
#111711=DIRECTION('',(1.,1.53063836115601E-16,-2.73691106313441E-48)) ;
#111712=DIRECTION('center_axis',(-1.53063836115601E-16,1.,0.)) ;
#111713=DIRECTION('ref_axis',(-1.,-1.53063836115601E-16,0.)) ;
#111714=DIRECTION('',(-1.,-1.53063836115601E-16,-2.73691106313441E-48)) ;
#111715=DIRECTION('',(0.,0.,-1.)) ;
#111716=DIRECTION('',(1.,1.53063836115601E-16,-2.73691106313441E-48)) ;
#111717=DIRECTION('',(0.,0.,1.)) ;
#111718=DIRECTION('center_axis',(1.99142572374599E-32,-1.30104260698261E-16,
1.)) ;
#111719=DIRECTION('ref_axis',(0.,-1.,-1.30104260698261E-16)) ;
#111720=DIRECTION('',(-1.,-1.53063836115601E-16,-2.73691106313441E-48)) ;
#111721=DIRECTION('',(-1.53063836115601E-16,1.,1.30104260698261E-16)) ;
#111722=DIRECTION('',(1.,1.53063836115601E-16,2.73691106313441E-48)) ;
#111723=DIRECTION('',(2.16840434497101E-16,-1.,-1.30104260698261E-16)) ;
#111724=DIRECTION('center_axis',(-1.53063836115601E-16,1.,0.)) ;
#111725=DIRECTION('ref_axis',(-1.,-1.53063836115601E-16,0.)) ;
#111726=DIRECTION('',(-1.,-1.53063836115601E-16,3.06472600140763E-33)) ;
#111727=DIRECTION('',(0.,0.,-1.)) ;
#111728=DIRECTION('',(1.,1.53063836115601E-16,2.73691106313441E-48)) ;
#111729=DIRECTION('',(0.,0.,1.)) ;
#111730=DIRECTION('center_axis',(-1.53063836115601E-16,1.,0.)) ;
#111731=DIRECTION('ref_axis',(-1.,-1.53063836115601E-16,0.)) ;
#111732=DIRECTION('',(-1.,-1.53063836115601E-16,2.73691106313441E-48)) ;
#111733=DIRECTION('',(0.,0.,-1.)) ;
#111734=DIRECTION('',(1.,1.53063836115601E-16,-1.53236300070382E-33)) ;
#111735=DIRECTION('',(0.,0.,1.)) ;
#111736=DIRECTION('center_axis',(1.99142572374599E-32,-1.30104260698261E-16,
-1.)) ;
#111737=DIRECTION('ref_axis',(0.,1.,-1.30104260698261E-16)) ;
#111738=DIRECTION('',(-1.,-1.53063836115601E-16,2.73691106313441E-48)) ;
#111739=DIRECTION('',(1.53063836115601E-16,-1.,1.30104260698261E-16)) ;
#111740=DIRECTION('',(1.,1.53063836115601E-16,-2.73691106313441E-48)) ;
#111741=DIRECTION('center_axis',(-1.53063836115601E-16,1.,0.)) ;
#111742=DIRECTION('ref_axis',(-1.,-1.53063836115601E-16,0.)) ;
#111743=DIRECTION('',(-1.,-1.53063836115601E-16,-2.73691106313441E-48)) ;
#111744=DIRECTION('',(0.,0.,-1.)) ;
#111745=DIRECTION('',(1.,1.53063836115601E-16,-2.73691106313441E-48)) ;
#111746=DIRECTION('',(0.,0.,1.)) ;
#111747=DIRECTION('center_axis',(1.99142572374599E-32,-1.30104260698261E-16,
1.)) ;
#111748=DIRECTION('ref_axis',(0.,-1.,-1.30104260698261E-16)) ;
#111749=DIRECTION('',(-1.,-1.53063836115601E-16,-2.73691106313441E-48)) ;
#111750=DIRECTION('',(-1.53063836115601E-16,1.,1.30104260698261E-16)) ;
#111751=DIRECTION('',(1.,1.53063836115601E-16,2.73691106313441E-48)) ;
#111752=DIRECTION('',(2.16840434497101E-16,-1.,-1.30104260698261E-16)) ;
#111753=DIRECTION('center_axis',(-1.53063836115601E-16,1.,0.)) ;
#111754=DIRECTION('ref_axis',(-1.,-1.53063836115601E-16,0.)) ;
#111755=DIRECTION('',(-1.,-1.53063836115601E-16,3.06472600140763E-33)) ;
#111756=DIRECTION('',(0.,0.,-1.)) ;
#111757=DIRECTION('',(1.,1.53063836115601E-16,2.73691106313441E-48)) ;
#111758=DIRECTION('',(0.,0.,1.)) ;
#111759=DIRECTION('center_axis',(-1.53063836115601E-16,1.,0.)) ;
#111760=DIRECTION('ref_axis',(-1.,-1.53063836115601E-16,0.)) ;
#111761=DIRECTION('',(-1.,-1.53063836115601E-16,2.73691106313441E-48)) ;
#111762=DIRECTION('',(0.,0.,-1.)) ;
#111763=DIRECTION('',(1.,1.53063836115601E-16,-1.53236300070382E-33)) ;
#111764=DIRECTION('',(0.,0.,1.)) ;
#111765=DIRECTION('center_axis',(1.99142572374599E-32,-1.30104260698261E-16,
-1.)) ;
#111766=DIRECTION('ref_axis',(0.,1.,-1.30104260698261E-16)) ;
#111767=DIRECTION('',(-1.,-1.53063836115601E-16,2.73691106313441E-48)) ;
#111768=DIRECTION('',(1.53063836115601E-16,-1.,1.30104260698261E-16)) ;
#111769=DIRECTION('',(1.,1.53063836115601E-16,-2.73691106313441E-48)) ;
#111770=DIRECTION('center_axis',(-1.53063836115601E-16,1.,0.)) ;
#111771=DIRECTION('ref_axis',(-1.,-1.53063836115601E-16,0.)) ;
#111772=DIRECTION('',(-1.,-1.53063836115601E-16,-2.73691106313441E-48)) ;
#111773=DIRECTION('',(0.,0.,-1.)) ;
#111774=DIRECTION('',(1.,1.53063836115601E-16,-2.73691106313441E-48)) ;
#111775=DIRECTION('',(0.,0.,1.)) ;
#111776=DIRECTION('center_axis',(1.99142572374599E-32,-1.30104260698261E-16,
1.)) ;
#111777=DIRECTION('ref_axis',(0.,-1.,-1.30104260698261E-16)) ;
#111778=DIRECTION('',(-1.,-1.53063836115601E-16,-2.73691106313441E-48)) ;
#111779=DIRECTION('',(-1.53063836115601E-16,1.,1.30104260698261E-16)) ;
#111780=DIRECTION('',(1.,1.53063836115601E-16,2.73691106313441E-48)) ;
#111781=DIRECTION('',(2.16840434497101E-16,-1.,-1.30104260698261E-16)) ;
#111782=DIRECTION('center_axis',(-1.53063836115601E-16,1.,0.)) ;
#111783=DIRECTION('ref_axis',(-1.,-1.53063836115601E-16,0.)) ;
#111784=DIRECTION('',(-1.,-1.53063836115601E-16,3.06472600140763E-33)) ;
#111785=DIRECTION('',(0.,0.,-1.)) ;
#111786=DIRECTION('',(1.,1.53063836115601E-16,2.73691106313441E-48)) ;
#111787=DIRECTION('',(0.,0.,1.)) ;
#111788=DIRECTION('center_axis',(-1.53063836115601E-16,1.,0.)) ;
#111789=DIRECTION('ref_axis',(-1.,-1.53063836115601E-16,0.)) ;
#111790=DIRECTION('',(-1.,-1.53063836115601E-16,2.73691106313441E-48)) ;
#111791=DIRECTION('',(0.,0.,-1.)) ;
#111792=DIRECTION('',(1.,1.53063836115601E-16,-1.53236300070382E-33)) ;
#111793=DIRECTION('',(0.,0.,1.)) ;
#111794=DIRECTION('center_axis',(1.99142572374599E-32,-1.30104260698261E-16,
-1.)) ;
#111795=DIRECTION('ref_axis',(0.,1.,-1.30104260698261E-16)) ;
#111796=DIRECTION('',(-1.,-1.53063836115601E-16,2.73691106313441E-48)) ;
#111797=DIRECTION('',(1.53063836115601E-16,-1.,1.30104260698261E-16)) ;
#111798=DIRECTION('',(1.,1.53063836115601E-16,-2.73691106313441E-48)) ;
#111799=DIRECTION('center_axis',(-1.53063836115601E-16,1.,0.)) ;
#111800=DIRECTION('ref_axis',(-1.,-1.53063836115601E-16,0.)) ;
#111801=DIRECTION('',(-1.,-1.53063836115601E-16,-2.73691106313441E-48)) ;
#111802=DIRECTION('',(0.,0.,-1.)) ;
#111803=DIRECTION('',(1.,1.53063836115601E-16,-2.73691106313441E-48)) ;
#111804=DIRECTION('',(0.,0.,1.)) ;
#111805=DIRECTION('center_axis',(1.99142572374599E-32,-1.30104260698261E-16,
1.)) ;
#111806=DIRECTION('ref_axis',(0.,-1.,-1.30104260698261E-16)) ;
#111807=DIRECTION('',(-1.,-1.53063836115601E-16,-2.73691106313441E-48)) ;
#111808=DIRECTION('',(-1.53063836115601E-16,1.,1.30104260698261E-16)) ;
#111809=DIRECTION('',(1.,1.53063836115601E-16,2.73691106313441E-48)) ;
#111810=DIRECTION('',(2.16840434497101E-16,-1.,-1.30104260698261E-16)) ;
#111811=DIRECTION('center_axis',(-1.53063836115601E-16,1.,0.)) ;
#111812=DIRECTION('ref_axis',(-1.,-1.53063836115601E-16,0.)) ;
#111813=DIRECTION('',(-1.,-1.53063836115601E-16,3.06472600140763E-33)) ;
#111814=DIRECTION('',(0.,0.,-1.)) ;
#111815=DIRECTION('',(1.,1.53063836115601E-16,2.73691106313441E-48)) ;
#111816=DIRECTION('',(0.,0.,1.)) ;
#111817=DIRECTION('center_axis',(1.,0.,0.)) ;
#111818=DIRECTION('ref_axis',(0.,0.,-1.)) ;
#111819=DIRECTION('',(1.,0.,0.)) ;
#111820=DIRECTION('center_axis',(1.,0.,0.)) ;
#111821=DIRECTION('ref_axis',(0.,0.,1.)) ;
#111822=DIRECTION('',(1.,0.,0.)) ;
#111823=DIRECTION('center_axis',(-1.,0.,0.)) ;
#111824=DIRECTION('ref_axis',(0.,0.,-1.)) ;
#111825=DIRECTION('center_axis',(0.,0.,1.)) ;
#111826=DIRECTION('ref_axis',(1.,0.,0.)) ;
#111827=DIRECTION('',(0.,1.,0.)) ;
#111828=DIRECTION('',(1.,0.,0.)) ;
#111829=DIRECTION('',(0.,-1.,0.)) ;
#111830=DIRECTION('center_axis',(1.,0.,0.)) ;
#111831=DIRECTION('ref_axis',(0.,0.,-1.)) ;
#111832=DIRECTION('center_axis',(1.,0.,0.)) ;
#111833=DIRECTION('ref_axis',(0.,0.,1.)) ;
#111834=DIRECTION('',(1.,0.,0.)) ;
#111835=DIRECTION('center_axis',(-1.,0.,0.)) ;
#111836=DIRECTION('ref_axis',(0.,0.,-1.)) ;
#111837=DIRECTION('center_axis',(0.,-1.,3.99416362155027E-15)) ;
#111838=DIRECTION('ref_axis',(0.,-3.99416362155027E-15,-1.)) ;
#111839=DIRECTION('',(0.,3.99416362155027E-15,1.)) ;
#111840=DIRECTION('',(1.,0.,0.)) ;
#111841=DIRECTION('',(0.,-3.99416362155027E-15,-1.)) ;
#111842=DIRECTION('center_axis',(1.,0.,0.)) ;
#111843=DIRECTION('ref_axis',(0.,0.,-1.)) ;
#111844=DIRECTION('center_axis',(-1.,0.,0.)) ;
#111845=DIRECTION('ref_axis',(0.,1.30104260698266E-14,-1.)) ;
#111846=DIRECTION('',(1.,0.,0.)) ;
#111847=DIRECTION('center_axis',(1.,0.,0.)) ;
#111848=DIRECTION('ref_axis',(0.,0.,-1.)) ;
#111849=DIRECTION('center_axis',(0.,-0.707106781186549,0.707106781186546)) ;
#111850=DIRECTION('ref_axis',(0.,-0.707106781186546,-0.707106781186549)) ;
#111851=DIRECTION('',(0.,0.707106781186546,0.707106781186549)) ;
#111852=DIRECTION('',(1.,0.,0.)) ;
#111853=DIRECTION('',(0.,-0.707106781186546,-0.707106781186549)) ;
#111854=DIRECTION('center_axis',(1.,0.,0.)) ;
#111855=DIRECTION('ref_axis',(0.,0.382683432365084,0.923879532511289)) ;
#111856=DIRECTION('',(1.,0.,0.)) ;
#111857=DIRECTION('center_axis',(1.,0.,0.)) ;
#111858=DIRECTION('ref_axis',(0.,0.,-1.)) ;
#111859=DIRECTION('center_axis',(0.,1.,0.)) ;
#111860=DIRECTION('ref_axis',(0.,0.,1.)) ;
#111861=DIRECTION('',(0.,0.,-1.)) ;
#111862=DIRECTION('',(0.,0.,1.)) ;
#111863=DIRECTION('center_axis',(0.,-0.707106781186547,-0.707106781186548)) ;
#111864=DIRECTION('ref_axis',(0.,0.707106781186548,-0.707106781186547)) ;
#111865=DIRECTION('',(0.,-0.707106781186548,0.707106781186547)) ;
#111866=DIRECTION('',(1.,0.,0.)) ;
#111867=DIRECTION('',(0.,0.707106781186548,-0.707106781186547)) ;
#111868=DIRECTION('center_axis',(1.,0.,0.)) ;
#111869=DIRECTION('ref_axis',(0.,0.,-1.)) ;
#111870=DIRECTION('center_axis',(-1.,0.,0.)) ;
#111871=DIRECTION('ref_axis',(0.,1.73472347597676E-14,-1.)) ;
#111872=DIRECTION('',(1.,0.,0.)) ;
#111873=DIRECTION('center_axis',(1.,0.,0.)) ;
#111874=DIRECTION('ref_axis',(0.,0.,-1.)) ;
#111875=DIRECTION('center_axis',(0.,-1.,0.)) ;
#111876=DIRECTION('ref_axis',(0.,0.,-1.)) ;
#111877=DIRECTION('',(0.,0.,1.)) ;
#111878=DIRECTION('',(1.,0.,0.)) ;
#111879=DIRECTION('',(0.,0.,-1.)) ;
#111880=DIRECTION('center_axis',(1.,0.,0.)) ;
#111881=DIRECTION('ref_axis',(0.,0.,-1.)) ;
#111882=DIRECTION('center_axis',(1.,0.,0.)) ;
#111883=DIRECTION('ref_axis',(0.,0.,1.)) ;
#111884=DIRECTION('',(1.,0.,0.)) ;
#111885=DIRECTION('center_axis',(-1.,0.,0.)) ;
#111886=DIRECTION('ref_axis',(0.,0.,-1.)) ;
#111887=DIRECTION('center_axis',(0.,0.,-1.)) ;
#111888=DIRECTION('ref_axis',(-1.,0.,0.)) ;
#111889=DIRECTION('',(0.,-1.,0.)) ;
#111890=DIRECTION('',(1.,0.,0.)) ;
#111891=DIRECTION('',(0.,1.,0.)) ;
#111892=DIRECTION('center_axis',(1.,0.,0.)) ;
#111893=DIRECTION('ref_axis',(0.,0.,-1.)) ;
#111894=DIRECTION('center_axis',(1.,0.,0.)) ;
#111895=DIRECTION('ref_axis',(0.,0.,1.)) ;
#111896=DIRECTION('',(1.,0.,0.)) ;
#111897=DIRECTION('center_axis',(-1.,0.,0.)) ;
#111898=DIRECTION('ref_axis',(0.,0.,-1.)) ;
#111899=DIRECTION('center_axis',(0.,1.,0.)) ;
#111900=DIRECTION('ref_axis',(0.,0.,1.)) ;
#111901=DIRECTION('',(0.,0.,-1.)) ;
#111902=DIRECTION('',(1.,0.,0.)) ;
#111903=DIRECTION('',(0.,0.,1.)) ;
#111904=DIRECTION('center_axis',(1.,0.,0.)) ;
#111905=DIRECTION('ref_axis',(0.,0.,-1.)) ;
#111906=DIRECTION('center_axis',(-1.,0.,0.)) ;
#111907=DIRECTION('ref_axis',(0.,1.95156391047385E-14,-1.)) ;
#111908=DIRECTION('',(1.,0.,0.)) ;
#111909=DIRECTION('center_axis',(1.,0.,0.)) ;
#111910=DIRECTION('ref_axis',(0.,0.,-1.)) ;
#111911=DIRECTION('center_axis',(0.,1.07081696047951E-16,-1.)) ;
#111912=DIRECTION('ref_axis',(0.,1.,1.07081696047951E-16)) ;
#111913=DIRECTION('',(0.,-1.,-1.07081696047951E-16)) ;
#111914=DIRECTION('',(1.,0.,0.)) ;
#111915=DIRECTION('',(0.,1.,1.07081696047951E-16)) ;
#111916=DIRECTION('center_axis',(1.,0.,0.)) ;
#111917=DIRECTION('ref_axis',(0.,0.,-1.)) ;
#111918=DIRECTION('center_axis',(-1.,0.,0.)) ;
#111919=DIRECTION('ref_axis',(0.,0.,-1.)) ;
#111920=DIRECTION('',(1.,0.,0.)) ;
#111921=DIRECTION('center_axis',(1.,0.,0.)) ;
#111922=DIRECTION('ref_axis',(0.,0.,-1.)) ;
#111923=DIRECTION('center_axis',(0.,-1.,0.)) ;
#111924=DIRECTION('ref_axis',(0.,0.,-1.)) ;
#111925=DIRECTION('',(0.,0.,1.)) ;
#111926=DIRECTION('',(1.,0.,0.)) ;
#111927=DIRECTION('',(0.,0.,-1.)) ;
#111928=DIRECTION('center_axis',(1.,0.,0.)) ;
#111929=DIRECTION('ref_axis',(0.,0.,-1.)) ;
#111930=DIRECTION('center_axis',(-1.,0.,0.)) ;
#111931=DIRECTION('ref_axis',(0.,3.03576608295933E-14,-1.)) ;
#111932=DIRECTION('',(1.,0.,0.)) ;
#111933=DIRECTION('center_axis',(1.,0.,0.)) ;
#111934=DIRECTION('ref_axis',(0.,0.,-1.)) ;
#111935=DIRECTION('center_axis',(1.,0.,0.)) ;
#111936=DIRECTION('ref_axis',(0.,0.,-1.)) ;
#111937=DIRECTION('center_axis',(1.,0.,0.)) ;
#111938=DIRECTION('ref_axis',(0.,-7.85535158932895E-16,1.)) ;
#111939=DIRECTION('',(1.,0.,0.)) ;
#111940=DIRECTION('center_axis',(-1.,0.,0.)) ;
#111941=DIRECTION('ref_axis',(0.,-7.85535158932895E-16,-1.)) ;
#111942=DIRECTION('center_axis',(1.,0.,0.)) ;
#111943=DIRECTION('ref_axis',(0.,0.,-1.)) ;
#111944=DIRECTION('center_axis',(-1.,0.,0.)) ;
#111945=DIRECTION('ref_axis',(0.,3.46944695195352E-14,-1.)) ;
#111946=DIRECTION('',(1.,0.,0.)) ;
#111947=DIRECTION('center_axis',(1.,0.,0.)) ;
#111948=DIRECTION('ref_axis',(0.,0.,-1.)) ;
#111949=DIRECTION('center_axis',(0.,-1.,0.)) ;
#111950=DIRECTION('ref_axis',(0.,0.,-1.)) ;
#111951=DIRECTION('',(0.,0.,1.)) ;
#111952=DIRECTION('',(1.,0.,0.)) ;
#111953=DIRECTION('',(0.,0.,-1.)) ;
#111954=DIRECTION('center_axis',(1.,0.,0.)) ;
#111955=DIRECTION('ref_axis',(0.,0.,-1.)) ;
#111956=DIRECTION('center_axis',(-1.,0.,0.)) ;
#111957=DIRECTION('ref_axis',(0.,0.,-1.)) ;
#111958=DIRECTION('',(1.,0.,0.)) ;
#111959=DIRECTION('center_axis',(1.,0.,0.)) ;
#111960=DIRECTION('ref_axis',(0.,0.,-1.)) ;
#111961=DIRECTION('center_axis',(0.,-1.07081696047951E-16,1.)) ;
#111962=DIRECTION('ref_axis',(0.,-1.,-1.07081696047951E-16)) ;
#111963=DIRECTION('',(0.,1.,1.07081696047951E-16)) ;
#111964=DIRECTION('',(1.,0.,0.)) ;
#111965=DIRECTION('',(0.,-1.,-1.07081696047951E-16)) ;
#111966=DIRECTION('center_axis',(1.,0.,0.)) ;
#111967=DIRECTION('ref_axis',(0.,0.,-1.)) ;
#111968=DIRECTION('center_axis',(-1.,0.,0.)) ;
#111969=DIRECTION('ref_axis',(0.,0.,-1.)) ;
#111970=DIRECTION('',(1.,0.,0.)) ;
#111971=DIRECTION('center_axis',(1.,0.,0.)) ;
#111972=DIRECTION('ref_axis',(0.,0.,-1.)) ;
#111973=DIRECTION('center_axis',(0.,1.,0.)) ;
#111974=DIRECTION('ref_axis',(0.,0.,1.)) ;
#111975=DIRECTION('',(0.,0.,-1.)) ;
#111976=DIRECTION('',(0.,0.,1.)) ;
#111977=DIRECTION('center_axis',(-1.,0.,0.)) ;
#111978=DIRECTION('ref_axis',(0.,0.,1.)) ;
#111979=DIRECTION('center_axis',(-1.,0.,0.)) ;
#111980=DIRECTION('ref_axis',(0.,0.,1.)) ;
#111981=DIRECTION('',(0.,-1.,0.)) ;
#111982=DIRECTION('center_axis',(-1.,0.,0.)) ;
#111983=DIRECTION('ref_axis',(0.,0.,1.)) ;
#111984=DIRECTION('',(0.,0.,1.)) ;
#111985=DIRECTION('',(0.,-1.,-1.07081696047951E-16)) ;
#111986=DIRECTION('',(0.,0.,-1.)) ;
#111987=DIRECTION('center_axis',(-1.,0.,0.)) ;
#111988=DIRECTION('ref_axis',(0.,0.,1.)) ;
#111989=DIRECTION('',(0.,0.,-1.)) ;
#111990=DIRECTION('',(0.,1.,1.07081696047951E-16)) ;
#111991=DIRECTION('',(0.,0.,1.)) ;
#111992=DIRECTION('center_axis',(-1.,0.,0.)) ;
#111993=DIRECTION('ref_axis',(0.,0.,1.)) ;
#111994=DIRECTION('',(0.,1.,0.)) ;
#111995=DIRECTION('center_axis',(-1.,0.,0.)) ;
#111996=DIRECTION('ref_axis',(0.,0.,1.)) ;
#111997=DIRECTION('',(0.,0.,-1.)) ;
#111998=DIRECTION('',(0.,0.707106781186548,-0.707106781186547)) ;
#111999=DIRECTION('',(0.,0.,1.)) ;
#112000=DIRECTION('',(0.,-0.707106781186546,-0.707106781186549)) ;
#112001=DIRECTION('',(0.,-3.99416362155027E-15,-1.)) ;
#112002=DIRECTION('center_axis',(1.,0.,0.)) ;
#112003=DIRECTION('ref_axis',(0.,0.,-1.)) ;
#112004=DIRECTION('',(1.,0.,0.)) ;
#112005=DIRECTION('center_axis',(1.,0.,0.)) ;
#112006=DIRECTION('ref_axis',(0.,0.,1.)) ;
#112007=DIRECTION('',(1.,0.,0.)) ;
#112008=DIRECTION('center_axis',(-1.,0.,0.)) ;
#112009=DIRECTION('ref_axis',(0.,0.,-1.)) ;
#112010=DIRECTION('center_axis',(0.,0.,1.)) ;
#112011=DIRECTION('ref_axis',(1.,0.,0.)) ;
#112012=DIRECTION('',(0.,1.,0.)) ;
#112013=DIRECTION('',(1.,0.,0.)) ;
#112014=DIRECTION('',(0.,-1.,0.)) ;
#112015=DIRECTION('center_axis',(1.,0.,0.)) ;
#112016=DIRECTION('ref_axis',(0.,0.,-1.)) ;
#112017=DIRECTION('center_axis',(1.,0.,0.)) ;
#112018=DIRECTION('ref_axis',(0.,0.,1.)) ;
#112019=DIRECTION('',(1.,0.,0.)) ;
#112020=DIRECTION('center_axis',(-1.,0.,0.)) ;
#112021=DIRECTION('ref_axis',(0.,0.,-1.)) ;
#112022=DIRECTION('center_axis',(0.,-1.,3.99416362155027E-15)) ;
#112023=DIRECTION('ref_axis',(0.,-3.99416362155027E-15,-1.)) ;
#112024=DIRECTION('',(0.,3.99416362155027E-15,1.)) ;
#112025=DIRECTION('',(1.,0.,0.)) ;
#112026=DIRECTION('',(0.,-3.99416362155027E-15,-1.)) ;
#112027=DIRECTION('center_axis',(1.,0.,0.)) ;
#112028=DIRECTION('ref_axis',(0.,0.,-1.)) ;
#112029=DIRECTION('center_axis',(-1.,0.,0.)) ;
#112030=DIRECTION('ref_axis',(0.,1.30104260698261E-14,-1.)) ;
#112031=DIRECTION('',(1.,0.,0.)) ;
#112032=DIRECTION('center_axis',(1.,0.,0.)) ;
#112033=DIRECTION('ref_axis',(0.,0.,-1.)) ;
#112034=DIRECTION('center_axis',(0.,-0.707106781186549,0.707106781186546)) ;
#112035=DIRECTION('ref_axis',(0.,-0.707106781186546,-0.707106781186549)) ;
#112036=DIRECTION('',(0.,0.707106781186546,0.707106781186549)) ;
#112037=DIRECTION('',(1.,0.,0.)) ;
#112038=DIRECTION('',(0.,-0.707106781186546,-0.707106781186549)) ;
#112039=DIRECTION('center_axis',(1.,0.,0.)) ;
#112040=DIRECTION('ref_axis',(0.,0.382683432365098,0.923879532511283)) ;
#112041=DIRECTION('',(1.,0.,0.)) ;
#112042=DIRECTION('center_axis',(1.,0.,0.)) ;
#112043=DIRECTION('ref_axis',(0.,0.,-1.)) ;
#112044=DIRECTION('center_axis',(0.,1.,0.)) ;
#112045=DIRECTION('ref_axis',(0.,0.,1.)) ;
#112046=DIRECTION('',(0.,0.,-1.)) ;
#112047=DIRECTION('',(0.,0.,1.)) ;
#112048=DIRECTION('center_axis',(0.,-0.707106781186547,-0.707106781186548)) ;
#112049=DIRECTION('ref_axis',(0.,0.707106781186548,-0.707106781186547)) ;
#112050=DIRECTION('',(0.,-0.707106781186548,0.707106781186547)) ;
#112051=DIRECTION('',(1.,0.,0.)) ;
#112052=DIRECTION('',(0.,0.707106781186548,-0.707106781186547)) ;
#112053=DIRECTION('center_axis',(1.,0.,0.)) ;
#112054=DIRECTION('ref_axis',(0.,0.,-1.)) ;
#112055=DIRECTION('center_axis',(-1.,0.,0.)) ;
#112056=DIRECTION('ref_axis',(0.,1.73472347597676E-14,-1.)) ;
#112057=DIRECTION('',(1.,0.,0.)) ;
#112058=DIRECTION('center_axis',(1.,0.,0.)) ;
#112059=DIRECTION('ref_axis',(0.,0.,-1.)) ;
#112060=DIRECTION('center_axis',(0.,-1.,0.)) ;
#112061=DIRECTION('ref_axis',(0.,0.,-1.)) ;
#112062=DIRECTION('',(0.,0.,1.)) ;
#112063=DIRECTION('',(1.,0.,0.)) ;
#112064=DIRECTION('',(0.,0.,-1.)) ;
#112065=DIRECTION('center_axis',(1.,0.,0.)) ;
#112066=DIRECTION('ref_axis',(0.,0.,-1.)) ;
#112067=DIRECTION('center_axis',(1.,0.,0.)) ;
#112068=DIRECTION('ref_axis',(0.,0.,1.)) ;
#112069=DIRECTION('',(1.,0.,0.)) ;
#112070=DIRECTION('center_axis',(-1.,0.,0.)) ;
#112071=DIRECTION('ref_axis',(0.,0.,-1.)) ;
#112072=DIRECTION('center_axis',(0.,0.,-1.)) ;
#112073=DIRECTION('ref_axis',(-1.,0.,0.)) ;
#112074=DIRECTION('',(0.,-1.,0.)) ;
#112075=DIRECTION('',(1.,0.,0.)) ;
#112076=DIRECTION('',(0.,1.,0.)) ;
#112077=DIRECTION('center_axis',(1.,0.,0.)) ;
#112078=DIRECTION('ref_axis',(0.,0.,-1.)) ;
#112079=DIRECTION('center_axis',(1.,0.,0.)) ;
#112080=DIRECTION('ref_axis',(0.,0.,1.)) ;
#112081=DIRECTION('',(1.,0.,0.)) ;
#112082=DIRECTION('center_axis',(-1.,0.,0.)) ;
#112083=DIRECTION('ref_axis',(0.,0.,-1.)) ;
#112084=DIRECTION('center_axis',(0.,1.,0.)) ;
#112085=DIRECTION('ref_axis',(0.,0.,1.)) ;
#112086=DIRECTION('',(0.,0.,-1.)) ;
#112087=DIRECTION('',(1.,0.,0.)) ;
#112088=DIRECTION('',(0.,0.,1.)) ;
#112089=DIRECTION('center_axis',(1.,0.,0.)) ;
#112090=DIRECTION('ref_axis',(0.,0.,-1.)) ;
#112091=DIRECTION('center_axis',(-1.,0.,0.)) ;
#112092=DIRECTION('ref_axis',(0.,1.95156391047385E-14,-1.)) ;
#112093=DIRECTION('',(1.,0.,0.)) ;
#112094=DIRECTION('center_axis',(1.,0.,0.)) ;
#112095=DIRECTION('ref_axis',(0.,0.,-1.)) ;
#112096=DIRECTION('center_axis',(0.,1.07081696047951E-16,-1.)) ;
#112097=DIRECTION('ref_axis',(0.,1.,1.07081696047951E-16)) ;
#112098=DIRECTION('',(0.,-1.,-1.07081696047951E-16)) ;
#112099=DIRECTION('',(1.,0.,0.)) ;
#112100=DIRECTION('',(0.,1.,1.07081696047951E-16)) ;
#112101=DIRECTION('center_axis',(1.,0.,0.)) ;
#112102=DIRECTION('ref_axis',(0.,0.,-1.)) ;
#112103=DIRECTION('center_axis',(-1.,0.,0.)) ;
#112104=DIRECTION('ref_axis',(0.,0.,-1.)) ;
#112105=DIRECTION('',(1.,0.,0.)) ;
#112106=DIRECTION('center_axis',(1.,0.,0.)) ;
#112107=DIRECTION('ref_axis',(0.,0.,-1.)) ;
#112108=DIRECTION('center_axis',(0.,-1.,0.)) ;
#112109=DIRECTION('ref_axis',(0.,0.,-1.)) ;
#112110=DIRECTION('',(0.,0.,1.)) ;
#112111=DIRECTION('',(1.,0.,0.)) ;
#112112=DIRECTION('',(0.,0.,-1.)) ;
#112113=DIRECTION('center_axis',(1.,0.,0.)) ;
#112114=DIRECTION('ref_axis',(0.,0.,-1.)) ;
#112115=DIRECTION('center_axis',(-1.,0.,0.)) ;
#112116=DIRECTION('ref_axis',(0.,3.03576608295933E-14,-1.)) ;
#112117=DIRECTION('',(1.,0.,0.)) ;
#112118=DIRECTION('center_axis',(1.,0.,0.)) ;
#112119=DIRECTION('ref_axis',(0.,0.,-1.)) ;
#112120=DIRECTION('center_axis',(1.,0.,0.)) ;
#112121=DIRECTION('ref_axis',(0.,0.,-1.)) ;
#112122=DIRECTION('center_axis',(1.,0.,0.)) ;
#112123=DIRECTION('ref_axis',(0.,-7.85535158932895E-16,1.)) ;
#112124=DIRECTION('',(1.,0.,0.)) ;
#112125=DIRECTION('center_axis',(-1.,0.,0.)) ;
#112126=DIRECTION('ref_axis',(0.,-7.85535158932895E-16,-1.)) ;
#112127=DIRECTION('center_axis',(1.,0.,0.)) ;
#112128=DIRECTION('ref_axis',(0.,0.,-1.)) ;
#112129=DIRECTION('center_axis',(-1.,0.,0.)) ;
#112130=DIRECTION('ref_axis',(0.,4.33680868994204E-15,-1.)) ;
#112131=DIRECTION('',(1.,0.,0.)) ;
#112132=DIRECTION('center_axis',(1.,0.,0.)) ;
#112133=DIRECTION('ref_axis',(0.,0.,-1.)) ;
#112134=DIRECTION('center_axis',(0.,-1.,0.)) ;
#112135=DIRECTION('ref_axis',(0.,0.,-1.)) ;
#112136=DIRECTION('',(0.,0.,1.)) ;
#112137=DIRECTION('',(1.,0.,0.)) ;
#112138=DIRECTION('',(0.,0.,-1.)) ;
#112139=DIRECTION('center_axis',(1.,0.,0.)) ;
#112140=DIRECTION('ref_axis',(0.,0.,-1.)) ;
#112141=DIRECTION('center_axis',(-1.,0.,0.)) ;
#112142=DIRECTION('ref_axis',(0.,0.,-1.)) ;
#112143=DIRECTION('',(1.,0.,0.)) ;
#112144=DIRECTION('center_axis',(1.,0.,0.)) ;
#112145=DIRECTION('ref_axis',(0.,0.,-1.)) ;
#112146=DIRECTION('center_axis',(0.,-1.07081696047951E-16,1.)) ;
#112147=DIRECTION('ref_axis',(0.,-1.,-1.07081696047951E-16)) ;
#112148=DIRECTION('',(0.,1.,1.07081696047951E-16)) ;
#112149=DIRECTION('',(1.,0.,0.)) ;
#112150=DIRECTION('',(0.,-1.,-1.07081696047951E-16)) ;
#112151=DIRECTION('center_axis',(1.,0.,0.)) ;
#112152=DIRECTION('ref_axis',(0.,0.,-1.)) ;
#112153=DIRECTION('center_axis',(-1.,0.,0.)) ;
#112154=DIRECTION('ref_axis',(0.,0.,-1.)) ;
#112155=DIRECTION('',(1.,0.,0.)) ;
#112156=DIRECTION('center_axis',(1.,0.,0.)) ;
#112157=DIRECTION('ref_axis',(0.,0.,-1.)) ;
#112158=DIRECTION('center_axis',(0.,1.,0.)) ;
#112159=DIRECTION('ref_axis',(0.,0.,1.)) ;
#112160=DIRECTION('',(0.,0.,-1.)) ;
#112161=DIRECTION('',(0.,0.,1.)) ;
#112162=DIRECTION('center_axis',(-1.,0.,0.)) ;
#112163=DIRECTION('ref_axis',(0.,0.,1.)) ;
#112164=DIRECTION('center_axis',(-1.,0.,0.)) ;
#112165=DIRECTION('ref_axis',(0.,0.,1.)) ;
#112166=DIRECTION('',(0.,-1.,0.)) ;
#112167=DIRECTION('center_axis',(-1.,0.,0.)) ;
#112168=DIRECTION('ref_axis',(0.,0.,1.)) ;
#112169=DIRECTION('',(0.,0.,1.)) ;
#112170=DIRECTION('',(0.,-1.,-1.07081696047951E-16)) ;
#112171=DIRECTION('',(0.,0.,-1.)) ;
#112172=DIRECTION('center_axis',(-1.,0.,0.)) ;
#112173=DIRECTION('ref_axis',(0.,0.,1.)) ;
#112174=DIRECTION('',(0.,0.,-1.)) ;
#112175=DIRECTION('',(0.,1.,1.07081696047951E-16)) ;
#112176=DIRECTION('',(0.,0.,1.)) ;
#112177=DIRECTION('center_axis',(-1.,0.,0.)) ;
#112178=DIRECTION('ref_axis',(0.,0.,1.)) ;
#112179=DIRECTION('',(0.,1.,0.)) ;
#112180=DIRECTION('center_axis',(-1.,0.,0.)) ;
#112181=DIRECTION('ref_axis',(0.,0.,1.)) ;
#112182=DIRECTION('',(0.,0.,-1.)) ;
#112183=DIRECTION('',(0.,0.707106781186548,-0.707106781186547)) ;
#112184=DIRECTION('',(0.,0.,1.)) ;
#112185=DIRECTION('',(0.,-0.707106781186546,-0.707106781186549)) ;
#112186=DIRECTION('',(0.,-3.99416362155027E-15,-1.)) ;
#112187=DIRECTION('center_axis',(1.,0.,0.)) ;
#112188=DIRECTION('ref_axis',(0.,0.,-1.)) ;
#112189=DIRECTION('',(1.,0.,0.)) ;
#112190=DIRECTION('center_axis',(1.,0.,0.)) ;
#112191=DIRECTION('ref_axis',(0.,0.,1.)) ;
#112192=DIRECTION('',(1.,0.,0.)) ;
#112193=DIRECTION('center_axis',(-1.,0.,0.)) ;
#112194=DIRECTION('ref_axis',(0.,0.,-1.)) ;
#112195=DIRECTION('center_axis',(0.,0.,1.)) ;
#112196=DIRECTION('ref_axis',(1.,0.,0.)) ;
#112197=DIRECTION('',(0.,1.,0.)) ;
#112198=DIRECTION('',(1.,0.,0.)) ;
#112199=DIRECTION('',(0.,-1.,0.)) ;
#112200=DIRECTION('center_axis',(1.,0.,0.)) ;
#112201=DIRECTION('ref_axis',(0.,0.,-1.)) ;
#112202=DIRECTION('center_axis',(1.,0.,0.)) ;
#112203=DIRECTION('ref_axis',(0.,0.,1.)) ;
#112204=DIRECTION('',(1.,0.,0.)) ;
#112205=DIRECTION('center_axis',(-1.,0.,0.)) ;
#112206=DIRECTION('ref_axis',(0.,0.,-1.)) ;
#112207=DIRECTION('center_axis',(0.,-1.,3.99416362155027E-15)) ;
#112208=DIRECTION('ref_axis',(0.,-3.99416362155027E-15,-1.)) ;
#112209=DIRECTION('',(0.,3.99416362155027E-15,1.)) ;
#112210=DIRECTION('',(1.,0.,0.)) ;
#112211=DIRECTION('',(0.,-3.99416362155027E-15,-1.)) ;
#112212=DIRECTION('center_axis',(1.,0.,0.)) ;
#112213=DIRECTION('ref_axis',(0.,0.,-1.)) ;
#112214=DIRECTION('center_axis',(-1.,0.,0.)) ;
#112215=DIRECTION('ref_axis',(0.,1.30104260698261E-14,-1.)) ;
#112216=DIRECTION('',(1.,0.,0.)) ;
#112217=DIRECTION('center_axis',(1.,0.,0.)) ;
#112218=DIRECTION('ref_axis',(0.,0.,-1.)) ;
#112219=DIRECTION('center_axis',(0.,-0.707106781186549,0.707106781186546)) ;
#112220=DIRECTION('ref_axis',(0.,-0.707106781186546,-0.707106781186549)) ;
#112221=DIRECTION('',(0.,0.707106781186546,0.707106781186549)) ;
#112222=DIRECTION('',(1.,0.,0.)) ;
#112223=DIRECTION('',(0.,-0.707106781186546,-0.707106781186549)) ;
#112224=DIRECTION('center_axis',(1.,0.,0.)) ;
#112225=DIRECTION('ref_axis',(0.,0.382683432365098,0.923879532511283)) ;
#112226=DIRECTION('',(1.,0.,0.)) ;
#112227=DIRECTION('center_axis',(1.,0.,0.)) ;
#112228=DIRECTION('ref_axis',(0.,0.,-1.)) ;
#112229=DIRECTION('center_axis',(0.,1.,0.)) ;
#112230=DIRECTION('ref_axis',(0.,0.,1.)) ;
#112231=DIRECTION('',(0.,0.,-1.)) ;
#112232=DIRECTION('',(0.,0.,1.)) ;
#112233=DIRECTION('center_axis',(0.,-0.707106781186547,-0.707106781186548)) ;
#112234=DIRECTION('ref_axis',(0.,0.707106781186548,-0.707106781186547)) ;
#112235=DIRECTION('',(0.,-0.707106781186548,0.707106781186547)) ;
#112236=DIRECTION('',(1.,0.,0.)) ;
#112237=DIRECTION('',(0.,0.707106781186548,-0.707106781186547)) ;
#112238=DIRECTION('center_axis',(1.,0.,0.)) ;
#112239=DIRECTION('ref_axis',(0.,0.,-1.)) ;
#112240=DIRECTION('center_axis',(-1.,0.,0.)) ;
#112241=DIRECTION('ref_axis',(0.,-1.73472347597682E-14,-1.)) ;
#112242=DIRECTION('',(1.,0.,0.)) ;
#112243=DIRECTION('center_axis',(1.,0.,0.)) ;
#112244=DIRECTION('ref_axis',(0.,0.,-1.)) ;
#112245=DIRECTION('center_axis',(0.,-1.,0.)) ;
#112246=DIRECTION('ref_axis',(0.,0.,-1.)) ;
#112247=DIRECTION('',(0.,0.,1.)) ;
#112248=DIRECTION('',(1.,0.,0.)) ;
#112249=DIRECTION('',(0.,0.,-1.)) ;
#112250=DIRECTION('center_axis',(1.,0.,0.)) ;
#112251=DIRECTION('ref_axis',(0.,0.,-1.)) ;
#112252=DIRECTION('center_axis',(1.,0.,0.)) ;
#112253=DIRECTION('ref_axis',(0.,0.,1.)) ;
#112254=DIRECTION('',(1.,0.,0.)) ;
#112255=DIRECTION('center_axis',(-1.,0.,0.)) ;
#112256=DIRECTION('ref_axis',(0.,0.,-1.)) ;
#112257=DIRECTION('center_axis',(0.,0.,-1.)) ;
#112258=DIRECTION('ref_axis',(-1.,0.,0.)) ;
#112259=DIRECTION('',(0.,-1.,0.)) ;
#112260=DIRECTION('',(1.,0.,0.)) ;
#112261=DIRECTION('',(0.,1.,0.)) ;
#112262=DIRECTION('center_axis',(1.,0.,0.)) ;
#112263=DIRECTION('ref_axis',(0.,0.,-1.)) ;
#112264=DIRECTION('center_axis',(1.,0.,0.)) ;
#112265=DIRECTION('ref_axis',(0.,0.,1.)) ;
#112266=DIRECTION('',(1.,0.,0.)) ;
#112267=DIRECTION('center_axis',(-1.,0.,0.)) ;
#112268=DIRECTION('ref_axis',(0.,0.,-1.)) ;
#112269=DIRECTION('center_axis',(0.,1.,0.)) ;
#112270=DIRECTION('ref_axis',(0.,0.,1.)) ;
#112271=DIRECTION('',(0.,0.,-1.)) ;
#112272=DIRECTION('',(1.,0.,0.)) ;
#112273=DIRECTION('',(0.,0.,1.)) ;
#112274=DIRECTION('center_axis',(1.,0.,0.)) ;
#112275=DIRECTION('ref_axis',(0.,0.,-1.)) ;
#112276=DIRECTION('center_axis',(-1.,0.,0.)) ;
#112277=DIRECTION('ref_axis',(0.,1.95156391047392E-14,-1.)) ;
#112278=DIRECTION('',(1.,0.,0.)) ;
#112279=DIRECTION('center_axis',(1.,0.,0.)) ;
#112280=DIRECTION('ref_axis',(0.,0.,-1.)) ;
#112281=DIRECTION('center_axis',(0.,1.07081696047951E-16,-1.)) ;
#112282=DIRECTION('ref_axis',(0.,1.,1.07081696047951E-16)) ;
#112283=DIRECTION('',(0.,-1.,-1.07081696047951E-16)) ;
#112284=DIRECTION('',(1.,0.,0.)) ;
#112285=DIRECTION('',(0.,1.,1.07081696047951E-16)) ;
#112286=DIRECTION('center_axis',(1.,0.,0.)) ;
#112287=DIRECTION('ref_axis',(0.,0.,-1.)) ;
#112288=DIRECTION('center_axis',(-1.,0.,0.)) ;
#112289=DIRECTION('ref_axis',(0.,0.,-1.)) ;
#112290=DIRECTION('',(1.,0.,0.)) ;
#112291=DIRECTION('center_axis',(1.,0.,0.)) ;
#112292=DIRECTION('ref_axis',(0.,0.,-1.)) ;
#112293=DIRECTION('center_axis',(0.,-1.,0.)) ;
#112294=DIRECTION('ref_axis',(0.,0.,-1.)) ;
#112295=DIRECTION('',(0.,0.,1.)) ;
#112296=DIRECTION('',(1.,0.,0.)) ;
#112297=DIRECTION('',(0.,0.,-1.)) ;
#112298=DIRECTION('center_axis',(1.,0.,0.)) ;
#112299=DIRECTION('ref_axis',(0.,0.,-1.)) ;
#112300=DIRECTION('center_axis',(-1.,0.,0.)) ;
#112301=DIRECTION('ref_axis',(0.,4.33680868994204E-15,-1.)) ;
#112302=DIRECTION('',(1.,0.,0.)) ;
#112303=DIRECTION('center_axis',(1.,0.,0.)) ;
#112304=DIRECTION('ref_axis',(0.,0.,-1.)) ;
#112305=DIRECTION('center_axis',(1.,0.,0.)) ;
#112306=DIRECTION('ref_axis',(0.,0.,-1.)) ;
#112307=DIRECTION('center_axis',(1.,0.,0.)) ;
#112308=DIRECTION('ref_axis',(0.,-7.85535158932895E-16,1.)) ;
#112309=DIRECTION('',(1.,0.,0.)) ;
#112310=DIRECTION('center_axis',(-1.,0.,0.)) ;
#112311=DIRECTION('ref_axis',(0.,-7.85535158932895E-16,-1.)) ;
#112312=DIRECTION('center_axis',(1.,0.,0.)) ;
#112313=DIRECTION('ref_axis',(0.,0.,-1.)) ;
#112314=DIRECTION('center_axis',(-1.,0.,0.)) ;
#112315=DIRECTION('ref_axis',(0.,4.33680868994204E-15,-1.)) ;
#112316=DIRECTION('',(1.,0.,0.)) ;
#112317=DIRECTION('center_axis',(1.,0.,0.)) ;
#112318=DIRECTION('ref_axis',(0.,0.,-1.)) ;
#112319=DIRECTION('center_axis',(0.,-1.,0.)) ;
#112320=DIRECTION('ref_axis',(0.,0.,-1.)) ;
#112321=DIRECTION('',(0.,0.,1.)) ;
#112322=DIRECTION('',(1.,0.,0.)) ;
#112323=DIRECTION('',(0.,0.,-1.)) ;
#112324=DIRECTION('center_axis',(1.,0.,0.)) ;
#112325=DIRECTION('ref_axis',(0.,0.,-1.)) ;
#112326=DIRECTION('center_axis',(-1.,0.,0.)) ;
#112327=DIRECTION('ref_axis',(0.,0.,-1.)) ;
#112328=DIRECTION('',(1.,0.,0.)) ;
#112329=DIRECTION('center_axis',(1.,0.,0.)) ;
#112330=DIRECTION('ref_axis',(0.,0.,-1.)) ;
#112331=DIRECTION('center_axis',(0.,-1.07081696047951E-16,1.)) ;
#112332=DIRECTION('ref_axis',(0.,-1.,-1.07081696047951E-16)) ;
#112333=DIRECTION('',(0.,1.,1.07081696047951E-16)) ;
#112334=DIRECTION('',(1.,0.,0.)) ;
#112335=DIRECTION('',(0.,-1.,-1.07081696047951E-16)) ;
#112336=DIRECTION('center_axis',(1.,0.,0.)) ;
#112337=DIRECTION('ref_axis',(0.,0.,-1.)) ;
#112338=DIRECTION('center_axis',(-1.,0.,0.)) ;
#112339=DIRECTION('ref_axis',(0.,0.,-1.)) ;
#112340=DIRECTION('',(1.,0.,0.)) ;
#112341=DIRECTION('center_axis',(1.,0.,0.)) ;
#112342=DIRECTION('ref_axis',(0.,0.,-1.)) ;
#112343=DIRECTION('center_axis',(0.,1.,0.)) ;
#112344=DIRECTION('ref_axis',(0.,0.,1.)) ;
#112345=DIRECTION('',(0.,0.,-1.)) ;
#112346=DIRECTION('',(0.,0.,1.)) ;
#112347=DIRECTION('center_axis',(-1.,0.,0.)) ;
#112348=DIRECTION('ref_axis',(0.,0.,1.)) ;
#112349=DIRECTION('center_axis',(-1.,0.,0.)) ;
#112350=DIRECTION('ref_axis',(0.,0.,1.)) ;
#112351=DIRECTION('',(0.,-1.,0.)) ;
#112352=DIRECTION('center_axis',(-1.,0.,0.)) ;
#112353=DIRECTION('ref_axis',(0.,0.,1.)) ;
#112354=DIRECTION('',(0.,0.,1.)) ;
#112355=DIRECTION('',(0.,-1.,-1.07081696047951E-16)) ;
#112356=DIRECTION('',(0.,0.,-1.)) ;
#112357=DIRECTION('center_axis',(-1.,0.,0.)) ;
#112358=DIRECTION('ref_axis',(0.,0.,1.)) ;
#112359=DIRECTION('',(0.,0.,-1.)) ;
#112360=DIRECTION('',(0.,1.,1.07081696047951E-16)) ;
#112361=DIRECTION('',(0.,0.,1.)) ;
#112362=DIRECTION('center_axis',(-1.,0.,0.)) ;
#112363=DIRECTION('ref_axis',(0.,0.,1.)) ;
#112364=DIRECTION('',(0.,1.,0.)) ;
#112365=DIRECTION('center_axis',(-1.,0.,0.)) ;
#112366=DIRECTION('ref_axis',(0.,0.,1.)) ;
#112367=DIRECTION('',(0.,0.,-1.)) ;
#112368=DIRECTION('',(0.,0.707106781186548,-0.707106781186547)) ;
#112369=DIRECTION('',(0.,0.,1.)) ;
#112370=DIRECTION('',(0.,-0.707106781186546,-0.707106781186549)) ;
#112371=DIRECTION('',(0.,-3.99416362155027E-15,-1.)) ;
#112372=DIRECTION('center_axis',(1.,0.,0.)) ;
#112373=DIRECTION('ref_axis',(0.,0.,-1.)) ;
#112374=DIRECTION('',(1.,0.,0.)) ;
#112375=DIRECTION('center_axis',(1.,0.,0.)) ;
#112376=DIRECTION('ref_axis',(0.,0.,1.)) ;
#112377=DIRECTION('',(1.,0.,0.)) ;
#112378=DIRECTION('center_axis',(-1.,0.,0.)) ;
#112379=DIRECTION('ref_axis',(0.,0.,-1.)) ;
#112380=DIRECTION('center_axis',(0.,0.,1.)) ;
#112381=DIRECTION('ref_axis',(1.,0.,0.)) ;
#112382=DIRECTION('',(0.,1.,0.)) ;
#112383=DIRECTION('',(1.,0.,0.)) ;
#112384=DIRECTION('',(0.,-1.,0.)) ;
#112385=DIRECTION('center_axis',(1.,0.,0.)) ;
#112386=DIRECTION('ref_axis',(0.,0.,-1.)) ;
#112387=DIRECTION('center_axis',(1.,0.,0.)) ;
#112388=DIRECTION('ref_axis',(0.,0.,1.)) ;
#112389=DIRECTION('',(1.,0.,0.)) ;
#112390=DIRECTION('center_axis',(-1.,0.,0.)) ;
#112391=DIRECTION('ref_axis',(0.,0.,-1.)) ;
#112392=DIRECTION('center_axis',(0.,-1.,3.99416362155027E-15)) ;
#112393=DIRECTION('ref_axis',(0.,-3.99416362155027E-15,-1.)) ;
#112394=DIRECTION('',(0.,3.99416362155027E-15,1.)) ;
#112395=DIRECTION('',(1.,0.,0.)) ;
#112396=DIRECTION('',(0.,-3.99416362155027E-15,-1.)) ;
#112397=DIRECTION('center_axis',(1.,0.,0.)) ;
#112398=DIRECTION('ref_axis',(0.,0.,-1.)) ;
#112399=DIRECTION('center_axis',(-1.,0.,0.)) ;
#112400=DIRECTION('ref_axis',(0.,1.30104260698261E-14,-1.)) ;
#112401=DIRECTION('',(1.,0.,0.)) ;
#112402=DIRECTION('center_axis',(1.,0.,0.)) ;
#112403=DIRECTION('ref_axis',(0.,0.,-1.)) ;
#112404=DIRECTION('center_axis',(0.,-0.707106781186549,0.707106781186546)) ;
#112405=DIRECTION('ref_axis',(0.,-0.707106781186546,-0.707106781186549)) ;
#112406=DIRECTION('',(0.,0.707106781186546,0.707106781186549)) ;
#112407=DIRECTION('',(1.,0.,0.)) ;
#112408=DIRECTION('',(0.,-0.707106781186546,-0.707106781186549)) ;
#112409=DIRECTION('center_axis',(1.,0.,0.)) ;
#112410=DIRECTION('ref_axis',(0.,0.382683432365098,0.923879532511283)) ;
#112411=DIRECTION('',(1.,0.,0.)) ;
#112412=DIRECTION('center_axis',(1.,0.,0.)) ;
#112413=DIRECTION('ref_axis',(0.,0.,-1.)) ;
#112414=DIRECTION('center_axis',(0.,1.,0.)) ;
#112415=DIRECTION('ref_axis',(0.,0.,1.)) ;
#112416=DIRECTION('',(0.,0.,-1.)) ;
#112417=DIRECTION('',(0.,0.,1.)) ;
#112418=DIRECTION('center_axis',(0.,-0.707106781186547,-0.707106781186548)) ;
#112419=DIRECTION('ref_axis',(0.,0.707106781186548,-0.707106781186547)) ;
#112420=DIRECTION('',(0.,-0.707106781186548,0.707106781186547)) ;
#112421=DIRECTION('',(1.,0.,0.)) ;
#112422=DIRECTION('',(0.,0.707106781186548,-0.707106781186547)) ;
#112423=DIRECTION('center_axis',(1.,0.,0.)) ;
#112424=DIRECTION('ref_axis',(0.,0.,-1.)) ;
#112425=DIRECTION('center_axis',(-1.,0.,0.)) ;
#112426=DIRECTION('ref_axis',(0.,-1.73472347597682E-14,-1.)) ;
#112427=DIRECTION('',(1.,0.,0.)) ;
#112428=DIRECTION('center_axis',(1.,0.,0.)) ;
#112429=DIRECTION('ref_axis',(0.,0.,-1.)) ;
#112430=DIRECTION('center_axis',(0.,-1.,0.)) ;
#112431=DIRECTION('ref_axis',(0.,0.,-1.)) ;
#112432=DIRECTION('',(0.,0.,1.)) ;
#112433=DIRECTION('',(1.,0.,0.)) ;
#112434=DIRECTION('',(0.,0.,-1.)) ;
#112435=DIRECTION('center_axis',(1.,0.,0.)) ;
#112436=DIRECTION('ref_axis',(0.,0.,-1.)) ;
#112437=DIRECTION('center_axis',(1.,0.,0.)) ;
#112438=DIRECTION('ref_axis',(0.,0.,1.)) ;
#112439=DIRECTION('',(1.,0.,0.)) ;
#112440=DIRECTION('center_axis',(-1.,0.,0.)) ;
#112441=DIRECTION('ref_axis',(0.,0.,-1.)) ;
#112442=DIRECTION('center_axis',(0.,0.,-1.)) ;
#112443=DIRECTION('ref_axis',(-1.,0.,0.)) ;
#112444=DIRECTION('',(0.,-1.,0.)) ;
#112445=DIRECTION('',(1.,0.,0.)) ;
#112446=DIRECTION('',(0.,1.,0.)) ;
#112447=DIRECTION('center_axis',(1.,0.,0.)) ;
#112448=DIRECTION('ref_axis',(0.,0.,-1.)) ;
#112449=DIRECTION('center_axis',(1.,0.,0.)) ;
#112450=DIRECTION('ref_axis',(0.,0.,1.)) ;
#112451=DIRECTION('',(1.,0.,0.)) ;
#112452=DIRECTION('center_axis',(-1.,0.,0.)) ;
#112453=DIRECTION('ref_axis',(0.,0.,-1.)) ;
#112454=DIRECTION('center_axis',(0.,1.,0.)) ;
#112455=DIRECTION('ref_axis',(0.,0.,1.)) ;
#112456=DIRECTION('',(0.,0.,-1.)) ;
#112457=DIRECTION('',(1.,0.,0.)) ;
#112458=DIRECTION('',(0.,0.,1.)) ;
#112459=DIRECTION('center_axis',(1.,0.,0.)) ;
#112460=DIRECTION('ref_axis',(0.,0.,-1.)) ;
#112461=DIRECTION('center_axis',(-1.,0.,0.)) ;
#112462=DIRECTION('ref_axis',(0.,1.95156391047392E-14,-1.)) ;
#112463=DIRECTION('',(1.,0.,0.)) ;
#112464=DIRECTION('center_axis',(1.,0.,0.)) ;
#112465=DIRECTION('ref_axis',(0.,0.,-1.)) ;
#112466=DIRECTION('center_axis',(0.,1.07081696047951E-16,-1.)) ;
#112467=DIRECTION('ref_axis',(0.,1.,1.07081696047951E-16)) ;
#112468=DIRECTION('',(0.,-1.,-1.07081696047951E-16)) ;
#112469=DIRECTION('',(1.,0.,0.)) ;
#112470=DIRECTION('',(0.,1.,1.07081696047951E-16)) ;
#112471=DIRECTION('center_axis',(1.,0.,0.)) ;
#112472=DIRECTION('ref_axis',(0.,0.,-1.)) ;
#112473=DIRECTION('center_axis',(-1.,0.,0.)) ;
#112474=DIRECTION('ref_axis',(0.,0.,-1.)) ;
#112475=DIRECTION('',(1.,0.,0.)) ;
#112476=DIRECTION('center_axis',(1.,0.,0.)) ;
#112477=DIRECTION('ref_axis',(0.,0.,-1.)) ;
#112478=DIRECTION('center_axis',(0.,-1.,0.)) ;
#112479=DIRECTION('ref_axis',(0.,0.,-1.)) ;
#112480=DIRECTION('',(0.,0.,1.)) ;
#112481=DIRECTION('',(1.,0.,0.)) ;
#112482=DIRECTION('',(0.,0.,-1.)) ;
#112483=DIRECTION('center_axis',(1.,0.,0.)) ;
#112484=DIRECTION('ref_axis',(0.,0.,-1.)) ;
#112485=DIRECTION('center_axis',(-1.,0.,0.)) ;
#112486=DIRECTION('ref_axis',(0.,4.33680868994204E-15,-1.)) ;
#112487=DIRECTION('',(1.,0.,0.)) ;
#112488=DIRECTION('center_axis',(1.,0.,0.)) ;
#112489=DIRECTION('ref_axis',(0.,0.,-1.)) ;
#112490=DIRECTION('center_axis',(1.,0.,0.)) ;
#112491=DIRECTION('ref_axis',(0.,0.,-1.)) ;
#112492=DIRECTION('center_axis',(1.,0.,0.)) ;
#112493=DIRECTION('ref_axis',(0.,-7.85535158932895E-16,1.)) ;
#112494=DIRECTION('',(1.,0.,0.)) ;
#112495=DIRECTION('center_axis',(-1.,0.,0.)) ;
#112496=DIRECTION('ref_axis',(0.,-7.85535158932895E-16,-1.)) ;
#112497=DIRECTION('center_axis',(1.,0.,0.)) ;
#112498=DIRECTION('ref_axis',(0.,0.,-1.)) ;
#112499=DIRECTION('center_axis',(-1.,0.,0.)) ;
#112500=DIRECTION('ref_axis',(0.,4.33680868994204E-15,-1.)) ;
#112501=DIRECTION('',(1.,0.,0.)) ;
#112502=DIRECTION('center_axis',(1.,0.,0.)) ;
#112503=DIRECTION('ref_axis',(0.,0.,-1.)) ;
#112504=DIRECTION('center_axis',(0.,-1.,0.)) ;
#112505=DIRECTION('ref_axis',(0.,0.,-1.)) ;
#112506=DIRECTION('',(0.,0.,1.)) ;
#112507=DIRECTION('',(1.,0.,0.)) ;
#112508=DIRECTION('',(0.,0.,-1.)) ;
#112509=DIRECTION('center_axis',(1.,0.,0.)) ;
#112510=DIRECTION('ref_axis',(0.,0.,-1.)) ;
#112511=DIRECTION('center_axis',(-1.,0.,0.)) ;
#112512=DIRECTION('ref_axis',(0.,0.,-1.)) ;
#112513=DIRECTION('',(1.,0.,0.)) ;
#112514=DIRECTION('center_axis',(1.,0.,0.)) ;
#112515=DIRECTION('ref_axis',(0.,0.,-1.)) ;
#112516=DIRECTION('center_axis',(0.,-1.07081696047951E-16,1.)) ;
#112517=DIRECTION('ref_axis',(0.,-1.,-1.07081696047951E-16)) ;
#112518=DIRECTION('',(0.,1.,1.07081696047951E-16)) ;
#112519=DIRECTION('',(1.,0.,0.)) ;
#112520=DIRECTION('',(0.,-1.,-1.07081696047951E-16)) ;
#112521=DIRECTION('center_axis',(1.,0.,0.)) ;
#112522=DIRECTION('ref_axis',(0.,0.,-1.)) ;
#112523=DIRECTION('center_axis',(-1.,0.,0.)) ;
#112524=DIRECTION('ref_axis',(0.,0.,-1.)) ;
#112525=DIRECTION('',(1.,0.,0.)) ;
#112526=DIRECTION('center_axis',(1.,0.,0.)) ;
#112527=DIRECTION('ref_axis',(0.,0.,-1.)) ;
#112528=DIRECTION('center_axis',(0.,1.,0.)) ;
#112529=DIRECTION('ref_axis',(0.,0.,1.)) ;
#112530=DIRECTION('',(0.,0.,-1.)) ;
#112531=DIRECTION('',(0.,0.,1.)) ;
#112532=DIRECTION('center_axis',(-1.,0.,0.)) ;
#112533=DIRECTION('ref_axis',(0.,0.,1.)) ;
#112534=DIRECTION('center_axis',(-1.,0.,0.)) ;
#112535=DIRECTION('ref_axis',(0.,0.,1.)) ;
#112536=DIRECTION('',(0.,-1.,0.)) ;
#112537=DIRECTION('center_axis',(-1.,0.,0.)) ;
#112538=DIRECTION('ref_axis',(0.,0.,1.)) ;
#112539=DIRECTION('',(0.,0.,1.)) ;
#112540=DIRECTION('',(0.,-1.,-1.07081696047951E-16)) ;
#112541=DIRECTION('',(0.,0.,-1.)) ;
#112542=DIRECTION('center_axis',(-1.,0.,0.)) ;
#112543=DIRECTION('ref_axis',(0.,0.,1.)) ;
#112544=DIRECTION('',(0.,0.,-1.)) ;
#112545=DIRECTION('',(0.,1.,1.07081696047951E-16)) ;
#112546=DIRECTION('',(0.,0.,1.)) ;
#112547=DIRECTION('center_axis',(-1.,0.,0.)) ;
#112548=DIRECTION('ref_axis',(0.,0.,1.)) ;
#112549=DIRECTION('',(0.,1.,0.)) ;
#112550=DIRECTION('center_axis',(-1.,0.,0.)) ;
#112551=DIRECTION('ref_axis',(0.,0.,1.)) ;
#112552=DIRECTION('',(0.,0.,-1.)) ;
#112553=DIRECTION('',(0.,0.707106781186548,-0.707106781186547)) ;
#112554=DIRECTION('',(0.,0.,1.)) ;
#112555=DIRECTION('',(0.,-0.707106781186546,-0.707106781186549)) ;
#112556=DIRECTION('',(0.,-3.99416362155027E-15,-1.)) ;
#112557=DIRECTION('center_axis',(1.,0.,0.)) ;
#112558=DIRECTION('ref_axis',(0.,0.,-1.)) ;
#112559=DIRECTION('',(1.,0.,0.)) ;
#112560=DIRECTION('center_axis',(1.,0.,0.)) ;
#112561=DIRECTION('ref_axis',(0.,0.,1.)) ;
#112562=DIRECTION('',(1.,0.,0.)) ;
#112563=DIRECTION('center_axis',(-1.,0.,0.)) ;
#112564=DIRECTION('ref_axis',(0.,0.,-1.)) ;
#112565=DIRECTION('center_axis',(0.,0.,1.)) ;
#112566=DIRECTION('ref_axis',(1.,0.,0.)) ;
#112567=DIRECTION('',(0.,1.,0.)) ;
#112568=DIRECTION('',(1.,0.,0.)) ;
#112569=DIRECTION('',(0.,-1.,0.)) ;
#112570=DIRECTION('center_axis',(1.,0.,0.)) ;
#112571=DIRECTION('ref_axis',(0.,0.,-1.)) ;
#112572=DIRECTION('center_axis',(1.,0.,0.)) ;
#112573=DIRECTION('ref_axis',(0.,0.,1.)) ;
#112574=DIRECTION('',(1.,0.,0.)) ;
#112575=DIRECTION('center_axis',(-1.,0.,0.)) ;
#112576=DIRECTION('ref_axis',(0.,0.,-1.)) ;
#112577=DIRECTION('center_axis',(0.,-1.,3.99416362155027E-15)) ;
#112578=DIRECTION('ref_axis',(0.,-3.99416362155027E-15,-1.)) ;
#112579=DIRECTION('',(0.,3.99416362155027E-15,1.)) ;
#112580=DIRECTION('',(1.,0.,0.)) ;
#112581=DIRECTION('',(0.,-3.99416362155027E-15,-1.)) ;
#112582=DIRECTION('center_axis',(1.,0.,0.)) ;
#112583=DIRECTION('ref_axis',(0.,0.,-1.)) ;
#112584=DIRECTION('center_axis',(-1.,0.,0.)) ;
#112585=DIRECTION('ref_axis',(0.,1.30104260698261E-14,-1.)) ;
#112586=DIRECTION('',(1.,0.,0.)) ;
#112587=DIRECTION('center_axis',(1.,0.,0.)) ;
#112588=DIRECTION('ref_axis',(0.,0.,-1.)) ;
#112589=DIRECTION('center_axis',(0.,-0.707106781186549,0.707106781186546)) ;
#112590=DIRECTION('ref_axis',(0.,-0.707106781186546,-0.707106781186549)) ;
#112591=DIRECTION('',(0.,0.707106781186546,0.707106781186549)) ;
#112592=DIRECTION('',(1.,0.,0.)) ;
#112593=DIRECTION('',(0.,-0.707106781186546,-0.707106781186549)) ;
#112594=DIRECTION('center_axis',(1.,0.,0.)) ;
#112595=DIRECTION('ref_axis',(0.,0.38268343236508,0.923879532511291)) ;
#112596=DIRECTION('',(1.,0.,0.)) ;
#112597=DIRECTION('center_axis',(1.,0.,0.)) ;
#112598=DIRECTION('ref_axis',(0.,0.,-1.)) ;
#112599=DIRECTION('center_axis',(0.,1.,0.)) ;
#112600=DIRECTION('ref_axis',(0.,0.,1.)) ;
#112601=DIRECTION('',(0.,0.,-1.)) ;
#112602=DIRECTION('',(0.,0.,1.)) ;
#112603=DIRECTION('center_axis',(0.,-0.707106781186547,-0.707106781186548)) ;
#112604=DIRECTION('ref_axis',(0.,0.707106781186548,-0.707106781186547)) ;
#112605=DIRECTION('',(0.,-0.707106781186548,0.707106781186547)) ;
#112606=DIRECTION('',(1.,0.,0.)) ;
#112607=DIRECTION('',(0.,0.707106781186548,-0.707106781186547)) ;
#112608=DIRECTION('center_axis',(1.,0.,0.)) ;
#112609=DIRECTION('ref_axis',(0.,0.,-1.)) ;
#112610=DIRECTION('center_axis',(-1.,0.,0.)) ;
#112611=DIRECTION('ref_axis',(0.,-1.73472347597682E-14,-1.)) ;
#112612=DIRECTION('',(1.,0.,0.)) ;
#112613=DIRECTION('center_axis',(1.,0.,0.)) ;
#112614=DIRECTION('ref_axis',(0.,0.,-1.)) ;
#112615=DIRECTION('center_axis',(0.,-1.,0.)) ;
#112616=DIRECTION('ref_axis',(0.,0.,-1.)) ;
#112617=DIRECTION('',(0.,0.,1.)) ;
#112618=DIRECTION('',(1.,0.,0.)) ;
#112619=DIRECTION('',(0.,0.,-1.)) ;
#112620=DIRECTION('center_axis',(1.,0.,0.)) ;
#112621=DIRECTION('ref_axis',(0.,0.,-1.)) ;
#112622=DIRECTION('center_axis',(1.,0.,0.)) ;
#112623=DIRECTION('ref_axis',(0.,0.,1.)) ;
#112624=DIRECTION('',(1.,0.,0.)) ;
#112625=DIRECTION('center_axis',(-1.,0.,0.)) ;
#112626=DIRECTION('ref_axis',(0.,0.,-1.)) ;
#112627=DIRECTION('center_axis',(0.,0.,-1.)) ;
#112628=DIRECTION('ref_axis',(-1.,0.,0.)) ;
#112629=DIRECTION('',(0.,-1.,0.)) ;
#112630=DIRECTION('',(1.,0.,0.)) ;
#112631=DIRECTION('',(0.,1.,0.)) ;
#112632=DIRECTION('center_axis',(1.,0.,0.)) ;
#112633=DIRECTION('ref_axis',(0.,0.,-1.)) ;
#112634=DIRECTION('center_axis',(1.,0.,0.)) ;
#112635=DIRECTION('ref_axis',(0.,0.,1.)) ;
#112636=DIRECTION('',(1.,0.,0.)) ;
#112637=DIRECTION('center_axis',(-1.,0.,0.)) ;
#112638=DIRECTION('ref_axis',(0.,0.,-1.)) ;
#112639=DIRECTION('center_axis',(0.,1.,0.)) ;
#112640=DIRECTION('ref_axis',(0.,0.,1.)) ;
#112641=DIRECTION('',(0.,0.,-1.)) ;
#112642=DIRECTION('',(1.,0.,0.)) ;
#112643=DIRECTION('',(0.,0.,1.)) ;
#112644=DIRECTION('center_axis',(1.,0.,0.)) ;
#112645=DIRECTION('ref_axis',(0.,0.,-1.)) ;
#112646=DIRECTION('center_axis',(-1.,0.,0.)) ;
#112647=DIRECTION('ref_axis',(0.,1.95156391047392E-14,-1.)) ;
#112648=DIRECTION('',(1.,0.,0.)) ;
#112649=DIRECTION('center_axis',(1.,0.,0.)) ;
#112650=DIRECTION('ref_axis',(0.,0.,-1.)) ;
#112651=DIRECTION('center_axis',(0.,1.07081696047951E-16,-1.)) ;
#112652=DIRECTION('ref_axis',(0.,1.,1.07081696047951E-16)) ;
#112653=DIRECTION('',(0.,-1.,-1.07081696047951E-16)) ;
#112654=DIRECTION('',(1.,0.,0.)) ;
#112655=DIRECTION('',(0.,1.,1.07081696047951E-16)) ;
#112656=DIRECTION('center_axis',(1.,0.,0.)) ;
#112657=DIRECTION('ref_axis',(0.,0.,-1.)) ;
#112658=DIRECTION('center_axis',(-1.,0.,0.)) ;
#112659=DIRECTION('ref_axis',(0.,0.,-1.)) ;
#112660=DIRECTION('',(1.,0.,0.)) ;
#112661=DIRECTION('center_axis',(1.,0.,0.)) ;
#112662=DIRECTION('ref_axis',(0.,0.,-1.)) ;
#112663=DIRECTION('center_axis',(0.,-1.,0.)) ;
#112664=DIRECTION('ref_axis',(0.,0.,-1.)) ;
#112665=DIRECTION('',(0.,0.,1.)) ;
#112666=DIRECTION('',(1.,0.,0.)) ;
#112667=DIRECTION('',(0.,0.,-1.)) ;
#112668=DIRECTION('center_axis',(1.,0.,0.)) ;
#112669=DIRECTION('ref_axis',(0.,0.,-1.)) ;
#112670=DIRECTION('center_axis',(-1.,0.,0.)) ;
#112671=DIRECTION('ref_axis',(0.,4.33680868994204E-15,-1.)) ;
#112672=DIRECTION('',(1.,0.,0.)) ;
#112673=DIRECTION('center_axis',(1.,0.,0.)) ;
#112674=DIRECTION('ref_axis',(0.,0.,-1.)) ;
#112675=DIRECTION('center_axis',(1.,0.,0.)) ;
#112676=DIRECTION('ref_axis',(0.,0.,-1.)) ;
#112677=DIRECTION('center_axis',(1.,0.,0.)) ;
#112678=DIRECTION('ref_axis',(0.,-7.85535158932895E-16,1.)) ;
#112679=DIRECTION('',(1.,0.,0.)) ;
#112680=DIRECTION('center_axis',(-1.,0.,0.)) ;
#112681=DIRECTION('ref_axis',(0.,-7.85535158932895E-16,-1.)) ;
#112682=DIRECTION('center_axis',(1.,0.,0.)) ;
#112683=DIRECTION('ref_axis',(0.,0.,-1.)) ;
#112684=DIRECTION('center_axis',(-1.,0.,0.)) ;
#112685=DIRECTION('ref_axis',(0.,4.33680868994204E-15,-1.)) ;
#112686=DIRECTION('',(1.,0.,0.)) ;
#112687=DIRECTION('center_axis',(1.,0.,0.)) ;
#112688=DIRECTION('ref_axis',(0.,0.,-1.)) ;
#112689=DIRECTION('center_axis',(0.,-1.,0.)) ;
#112690=DIRECTION('ref_axis',(0.,0.,-1.)) ;
#112691=DIRECTION('',(0.,0.,1.)) ;
#112692=DIRECTION('',(1.,0.,0.)) ;
#112693=DIRECTION('',(0.,0.,-1.)) ;
#112694=DIRECTION('center_axis',(1.,0.,0.)) ;
#112695=DIRECTION('ref_axis',(0.,0.,-1.)) ;
#112696=DIRECTION('center_axis',(-1.,0.,0.)) ;
#112697=DIRECTION('ref_axis',(0.,0.,-1.)) ;
#112698=DIRECTION('',(1.,0.,0.)) ;
#112699=DIRECTION('center_axis',(1.,0.,0.)) ;
#112700=DIRECTION('ref_axis',(0.,0.,-1.)) ;
#112701=DIRECTION('center_axis',(0.,-1.07081696047951E-16,1.)) ;
#112702=DIRECTION('ref_axis',(0.,-1.,-1.07081696047951E-16)) ;
#112703=DIRECTION('',(0.,1.,1.07081696047951E-16)) ;
#112704=DIRECTION('',(1.,0.,0.)) ;
#112705=DIRECTION('',(0.,-1.,-1.07081696047951E-16)) ;
#112706=DIRECTION('center_axis',(1.,0.,0.)) ;
#112707=DIRECTION('ref_axis',(0.,0.,-1.)) ;
#112708=DIRECTION('center_axis',(-1.,0.,0.)) ;
#112709=DIRECTION('ref_axis',(0.,0.,-1.)) ;
#112710=DIRECTION('',(1.,0.,0.)) ;
#112711=DIRECTION('center_axis',(1.,0.,0.)) ;
#112712=DIRECTION('ref_axis',(0.,0.,-1.)) ;
#112713=DIRECTION('center_axis',(0.,1.,0.)) ;
#112714=DIRECTION('ref_axis',(0.,0.,1.)) ;
#112715=DIRECTION('',(0.,0.,-1.)) ;
#112716=DIRECTION('',(0.,0.,1.)) ;
#112717=DIRECTION('center_axis',(-1.,0.,0.)) ;
#112718=DIRECTION('ref_axis',(0.,0.,1.)) ;
#112719=DIRECTION('center_axis',(-1.,0.,0.)) ;
#112720=DIRECTION('ref_axis',(0.,0.,1.)) ;
#112721=DIRECTION('',(0.,-1.,0.)) ;
#112722=DIRECTION('center_axis',(-1.,0.,0.)) ;
#112723=DIRECTION('ref_axis',(0.,0.,1.)) ;
#112724=DIRECTION('',(0.,0.,1.)) ;
#112725=DIRECTION('',(0.,-1.,-1.07081696047951E-16)) ;
#112726=DIRECTION('',(0.,0.,-1.)) ;
#112727=DIRECTION('center_axis',(-1.,0.,0.)) ;
#112728=DIRECTION('ref_axis',(0.,0.,1.)) ;
#112729=DIRECTION('',(0.,0.,-1.)) ;
#112730=DIRECTION('',(0.,1.,1.07081696047951E-16)) ;
#112731=DIRECTION('',(0.,0.,1.)) ;
#112732=DIRECTION('center_axis',(-1.,0.,0.)) ;
#112733=DIRECTION('ref_axis',(0.,0.,1.)) ;
#112734=DIRECTION('',(0.,1.,0.)) ;
#112735=DIRECTION('center_axis',(-1.,0.,0.)) ;
#112736=DIRECTION('ref_axis',(0.,0.,1.)) ;
#112737=DIRECTION('',(0.,0.,-1.)) ;
#112738=DIRECTION('',(0.,0.707106781186548,-0.707106781186547)) ;
#112739=DIRECTION('',(0.,0.,1.)) ;
#112740=DIRECTION('',(0.,-0.707106781186546,-0.707106781186549)) ;
#112741=DIRECTION('',(0.,-3.99416362155027E-15,-1.)) ;
#112742=DIRECTION('center_axis',(1.,0.,0.)) ;
#112743=DIRECTION('ref_axis',(0.,0.,-1.)) ;
#112744=DIRECTION('',(1.,0.,0.)) ;
#112745=DIRECTION('center_axis',(1.,0.,0.)) ;
#112746=DIRECTION('ref_axis',(0.,0.,1.)) ;
#112747=DIRECTION('',(1.,0.,0.)) ;
#112748=DIRECTION('center_axis',(-1.,0.,0.)) ;
#112749=DIRECTION('ref_axis',(0.,0.,-1.)) ;
#112750=DIRECTION('center_axis',(0.,0.,1.)) ;
#112751=DIRECTION('ref_axis',(1.,0.,0.)) ;
#112752=DIRECTION('',(0.,1.,0.)) ;
#112753=DIRECTION('',(1.,0.,0.)) ;
#112754=DIRECTION('',(0.,-1.,0.)) ;
#112755=DIRECTION('center_axis',(1.,0.,0.)) ;
#112756=DIRECTION('ref_axis',(0.,0.,-1.)) ;
#112757=DIRECTION('center_axis',(1.,0.,0.)) ;
#112758=DIRECTION('ref_axis',(0.,0.,1.)) ;
#112759=DIRECTION('',(1.,0.,0.)) ;
#112760=DIRECTION('center_axis',(-1.,0.,0.)) ;
#112761=DIRECTION('ref_axis',(0.,0.,-1.)) ;
#112762=DIRECTION('center_axis',(0.,-1.,3.99416362155027E-15)) ;
#112763=DIRECTION('ref_axis',(0.,-3.99416362155027E-15,-1.)) ;
#112764=DIRECTION('',(0.,3.99416362155027E-15,1.)) ;
#112765=DIRECTION('',(1.,0.,0.)) ;
#112766=DIRECTION('',(0.,-3.99416362155027E-15,-1.)) ;
#112767=DIRECTION('center_axis',(1.,0.,0.)) ;
#112768=DIRECTION('ref_axis',(0.,0.,-1.)) ;
#112769=DIRECTION('center_axis',(-1.,0.,0.)) ;
#112770=DIRECTION('ref_axis',(0.,1.30104260698261E-14,-1.)) ;
#112771=DIRECTION('',(1.,0.,0.)) ;
#112772=DIRECTION('center_axis',(1.,0.,0.)) ;
#112773=DIRECTION('ref_axis',(0.,0.,-1.)) ;
#112774=DIRECTION('center_axis',(0.,-0.707106781186549,0.707106781186546)) ;
#112775=DIRECTION('ref_axis',(0.,-0.707106781186546,-0.707106781186549)) ;
#112776=DIRECTION('',(0.,0.707106781186546,0.707106781186549)) ;
#112777=DIRECTION('',(1.,0.,0.)) ;
#112778=DIRECTION('',(0.,-0.707106781186546,-0.707106781186549)) ;
#112779=DIRECTION('center_axis',(1.,0.,0.)) ;
#112780=DIRECTION('ref_axis',(0.,0.382683432365084,0.923879532511289)) ;
#112781=DIRECTION('',(1.,0.,0.)) ;
#112782=DIRECTION('center_axis',(1.,0.,0.)) ;
#112783=DIRECTION('ref_axis',(0.,0.,-1.)) ;
#112784=DIRECTION('center_axis',(0.,1.,0.)) ;
#112785=DIRECTION('ref_axis',(0.,0.,1.)) ;
#112786=DIRECTION('',(0.,0.,-1.)) ;
#112787=DIRECTION('',(0.,0.,1.)) ;
#112788=DIRECTION('center_axis',(0.,-0.707106781186547,-0.707106781186548)) ;
#112789=DIRECTION('ref_axis',(0.,0.707106781186548,-0.707106781186547)) ;
#112790=DIRECTION('',(0.,-0.707106781186548,0.707106781186547)) ;
#112791=DIRECTION('',(1.,0.,0.)) ;
#112792=DIRECTION('',(0.,0.707106781186548,-0.707106781186547)) ;
#112793=DIRECTION('center_axis',(1.,0.,0.)) ;
#112794=DIRECTION('ref_axis',(0.,0.,-1.)) ;
#112795=DIRECTION('center_axis',(-1.,0.,0.)) ;
#112796=DIRECTION('ref_axis',(0.,-1.73472347597682E-14,-1.)) ;
#112797=DIRECTION('',(1.,0.,0.)) ;
#112798=DIRECTION('center_axis',(1.,0.,0.)) ;
#112799=DIRECTION('ref_axis',(0.,0.,-1.)) ;
#112800=DIRECTION('center_axis',(0.,-1.,0.)) ;
#112801=DIRECTION('ref_axis',(0.,0.,-1.)) ;
#112802=DIRECTION('',(0.,0.,1.)) ;
#112803=DIRECTION('',(1.,0.,0.)) ;
#112804=DIRECTION('',(0.,0.,-1.)) ;
#112805=DIRECTION('center_axis',(1.,0.,0.)) ;
#112806=DIRECTION('ref_axis',(0.,0.,-1.)) ;
#112807=DIRECTION('center_axis',(1.,0.,0.)) ;
#112808=DIRECTION('ref_axis',(0.,0.,1.)) ;
#112809=DIRECTION('',(1.,0.,0.)) ;
#112810=DIRECTION('center_axis',(-1.,0.,0.)) ;
#112811=DIRECTION('ref_axis',(0.,0.,-1.)) ;
#112812=DIRECTION('center_axis',(0.,0.,-1.)) ;
#112813=DIRECTION('ref_axis',(-1.,0.,0.)) ;
#112814=DIRECTION('',(0.,-1.,0.)) ;
#112815=DIRECTION('',(1.,0.,0.)) ;
#112816=DIRECTION('',(0.,1.,0.)) ;
#112817=DIRECTION('center_axis',(1.,0.,0.)) ;
#112818=DIRECTION('ref_axis',(0.,0.,-1.)) ;
#112819=DIRECTION('center_axis',(1.,0.,0.)) ;
#112820=DIRECTION('ref_axis',(0.,0.,1.)) ;
#112821=DIRECTION('',(1.,0.,0.)) ;
#112822=DIRECTION('center_axis',(-1.,0.,0.)) ;
#112823=DIRECTION('ref_axis',(0.,0.,-1.)) ;
#112824=DIRECTION('center_axis',(0.,1.,0.)) ;
#112825=DIRECTION('ref_axis',(0.,0.,1.)) ;
#112826=DIRECTION('',(0.,0.,-1.)) ;
#112827=DIRECTION('',(1.,0.,0.)) ;
#112828=DIRECTION('',(0.,0.,1.)) ;
#112829=DIRECTION('center_axis',(1.,0.,0.)) ;
#112830=DIRECTION('ref_axis',(0.,0.,-1.)) ;
#112831=DIRECTION('center_axis',(-1.,0.,0.)) ;
#112832=DIRECTION('ref_axis',(0.,1.95156391047392E-14,-1.)) ;
#112833=DIRECTION('',(1.,0.,0.)) ;
#112834=DIRECTION('center_axis',(1.,0.,0.)) ;
#112835=DIRECTION('ref_axis',(0.,0.,-1.)) ;
#112836=DIRECTION('center_axis',(0.,1.07081696047951E-16,-1.)) ;
#112837=DIRECTION('ref_axis',(0.,1.,1.07081696047951E-16)) ;
#112838=DIRECTION('',(0.,-1.,-1.07081696047951E-16)) ;
#112839=DIRECTION('',(1.,0.,0.)) ;
#112840=DIRECTION('',(0.,1.,1.07081696047951E-16)) ;
#112841=DIRECTION('center_axis',(1.,0.,0.)) ;
#112842=DIRECTION('ref_axis',(0.,0.,-1.)) ;
#112843=DIRECTION('center_axis',(-1.,0.,0.)) ;
#112844=DIRECTION('ref_axis',(0.,0.,-1.)) ;
#112845=DIRECTION('',(1.,0.,0.)) ;
#112846=DIRECTION('center_axis',(1.,0.,0.)) ;
#112847=DIRECTION('ref_axis',(0.,0.,-1.)) ;
#112848=DIRECTION('center_axis',(0.,-1.,0.)) ;
#112849=DIRECTION('ref_axis',(0.,0.,-1.)) ;
#112850=DIRECTION('',(0.,0.,1.)) ;
#112851=DIRECTION('',(1.,0.,0.)) ;
#112852=DIRECTION('',(0.,0.,-1.)) ;
#112853=DIRECTION('center_axis',(1.,0.,0.)) ;
#112854=DIRECTION('ref_axis',(0.,0.,-1.)) ;
#112855=DIRECTION('center_axis',(-1.,0.,0.)) ;
#112856=DIRECTION('ref_axis',(0.,4.33680868994204E-15,-1.)) ;
#112857=DIRECTION('',(1.,0.,0.)) ;
#112858=DIRECTION('center_axis',(1.,0.,0.)) ;
#112859=DIRECTION('ref_axis',(0.,0.,-1.)) ;
#112860=DIRECTION('center_axis',(1.,0.,0.)) ;
#112861=DIRECTION('ref_axis',(0.,0.,-1.)) ;
#112862=DIRECTION('center_axis',(1.,0.,0.)) ;
#112863=DIRECTION('ref_axis',(0.,-7.85535158932894E-16,1.)) ;
#112864=DIRECTION('',(1.,0.,0.)) ;
#112865=DIRECTION('center_axis',(-1.,0.,0.)) ;
#112866=DIRECTION('ref_axis',(0.,-7.85535158932895E-16,-1.)) ;
#112867=DIRECTION('center_axis',(1.,0.,0.)) ;
#112868=DIRECTION('ref_axis',(0.,0.,-1.)) ;
#112869=DIRECTION('center_axis',(-1.,0.,0.)) ;
#112870=DIRECTION('ref_axis',(0.,-8.67361737988409E-15,-1.)) ;
#112871=DIRECTION('',(1.,0.,0.)) ;
#112872=DIRECTION('center_axis',(1.,0.,0.)) ;
#112873=DIRECTION('ref_axis',(0.,0.,-1.)) ;
#112874=DIRECTION('center_axis',(0.,-1.,0.)) ;
#112875=DIRECTION('ref_axis',(0.,0.,-1.)) ;
#112876=DIRECTION('',(0.,0.,1.)) ;
#112877=DIRECTION('',(1.,0.,0.)) ;
#112878=DIRECTION('',(0.,0.,-1.)) ;
#112879=DIRECTION('center_axis',(1.,0.,0.)) ;
#112880=DIRECTION('ref_axis',(0.,0.,-1.)) ;
#112881=DIRECTION('center_axis',(-1.,0.,0.)) ;
#112882=DIRECTION('ref_axis',(0.,0.,-1.)) ;
#112883=DIRECTION('',(1.,0.,0.)) ;
#112884=DIRECTION('center_axis',(1.,0.,0.)) ;
#112885=DIRECTION('ref_axis',(0.,0.,-1.)) ;
#112886=DIRECTION('center_axis',(0.,-1.07081696047951E-16,1.)) ;
#112887=DIRECTION('ref_axis',(0.,-1.,-1.07081696047951E-16)) ;
#112888=DIRECTION('',(0.,1.,1.07081696047951E-16)) ;
#112889=DIRECTION('',(1.,0.,0.)) ;
#112890=DIRECTION('',(0.,-1.,-1.07081696047951E-16)) ;
#112891=DIRECTION('center_axis',(1.,0.,0.)) ;
#112892=DIRECTION('ref_axis',(0.,0.,-1.)) ;
#112893=DIRECTION('center_axis',(-1.,0.,0.)) ;
#112894=DIRECTION('ref_axis',(0.,0.,-1.)) ;
#112895=DIRECTION('',(1.,0.,0.)) ;
#112896=DIRECTION('center_axis',(1.,0.,0.)) ;
#112897=DIRECTION('ref_axis',(0.,0.,-1.)) ;
#112898=DIRECTION('center_axis',(0.,1.,0.)) ;
#112899=DIRECTION('ref_axis',(0.,0.,1.)) ;
#112900=DIRECTION('',(0.,0.,-1.)) ;
#112901=DIRECTION('',(0.,0.,1.)) ;
#112902=DIRECTION('center_axis',(-1.,0.,0.)) ;
#112903=DIRECTION('ref_axis',(0.,0.,1.)) ;
#112904=DIRECTION('center_axis',(-1.,0.,0.)) ;
#112905=DIRECTION('ref_axis',(0.,0.,1.)) ;
#112906=DIRECTION('',(0.,-1.,0.)) ;
#112907=DIRECTION('center_axis',(-1.,0.,0.)) ;
#112908=DIRECTION('ref_axis',(0.,0.,1.)) ;
#112909=DIRECTION('',(0.,0.,1.)) ;
#112910=DIRECTION('',(0.,-1.,-1.07081696047951E-16)) ;
#112911=DIRECTION('',(0.,0.,-1.)) ;
#112912=DIRECTION('center_axis',(-1.,0.,0.)) ;
#112913=DIRECTION('ref_axis',(0.,0.,1.)) ;
#112914=DIRECTION('',(0.,0.,-1.)) ;
#112915=DIRECTION('',(0.,1.,1.07081696047951E-16)) ;
#112916=DIRECTION('',(0.,0.,1.)) ;
#112917=DIRECTION('center_axis',(-1.,0.,0.)) ;
#112918=DIRECTION('ref_axis',(0.,0.,1.)) ;
#112919=DIRECTION('',(0.,1.,0.)) ;
#112920=DIRECTION('center_axis',(-1.,0.,0.)) ;
#112921=DIRECTION('ref_axis',(0.,0.,1.)) ;
#112922=DIRECTION('',(0.,0.,-1.)) ;
#112923=DIRECTION('',(0.,0.707106781186548,-0.707106781186547)) ;
#112924=DIRECTION('',(0.,0.,1.)) ;
#112925=DIRECTION('',(0.,-0.707106781186546,-0.707106781186549)) ;
#112926=DIRECTION('',(0.,-3.99416362155027E-15,-1.)) ;
#112927=DIRECTION('center_axis',(1.,0.,0.)) ;
#112928=DIRECTION('ref_axis',(0.,0.,-1.)) ;
#112929=DIRECTION('',(1.,0.,0.)) ;
#112930=DIRECTION('center_axis',(1.,0.,0.)) ;
#112931=DIRECTION('ref_axis',(0.,0.,1.)) ;
#112932=DIRECTION('',(1.,0.,0.)) ;
#112933=DIRECTION('center_axis',(-1.,0.,0.)) ;
#112934=DIRECTION('ref_axis',(0.,0.,-1.)) ;
#112935=DIRECTION('center_axis',(0.,0.,1.)) ;
#112936=DIRECTION('ref_axis',(1.,0.,0.)) ;
#112937=DIRECTION('',(0.,1.,0.)) ;
#112938=DIRECTION('',(1.,0.,0.)) ;
#112939=DIRECTION('',(0.,-1.,0.)) ;
#112940=DIRECTION('center_axis',(1.,0.,0.)) ;
#112941=DIRECTION('ref_axis',(0.,0.,-1.)) ;
#112942=DIRECTION('center_axis',(1.,0.,0.)) ;
#112943=DIRECTION('ref_axis',(0.,0.,1.)) ;
#112944=DIRECTION('',(1.,0.,0.)) ;
#112945=DIRECTION('center_axis',(-1.,0.,0.)) ;
#112946=DIRECTION('ref_axis',(0.,0.,-1.)) ;
#112947=DIRECTION('center_axis',(0.,-1.,3.99416362155027E-15)) ;
#112948=DIRECTION('ref_axis',(0.,-3.99416362155027E-15,-1.)) ;
#112949=DIRECTION('',(0.,3.99416362155027E-15,1.)) ;
#112950=DIRECTION('',(1.,0.,0.)) ;
#112951=DIRECTION('',(0.,-3.99416362155027E-15,-1.)) ;
#112952=DIRECTION('center_axis',(1.,0.,0.)) ;
#112953=DIRECTION('ref_axis',(0.,0.,-1.)) ;
#112954=DIRECTION('center_axis',(-1.,0.,0.)) ;
#112955=DIRECTION('ref_axis',(0.,1.30104260698261E-14,-1.)) ;
#112956=DIRECTION('',(1.,0.,0.)) ;
#112957=DIRECTION('center_axis',(1.,0.,0.)) ;
#112958=DIRECTION('ref_axis',(0.,0.,-1.)) ;
#112959=DIRECTION('center_axis',(0.,-0.707106781186549,0.707106781186546)) ;
#112960=DIRECTION('ref_axis',(0.,-0.707106781186546,-0.707106781186549)) ;
#112961=DIRECTION('',(0.,0.707106781186546,0.707106781186549)) ;
#112962=DIRECTION('',(1.,0.,0.)) ;
#112963=DIRECTION('',(0.,-0.707106781186546,-0.707106781186549)) ;
#112964=DIRECTION('center_axis',(1.,0.,0.)) ;
#112965=DIRECTION('ref_axis',(0.,0.382683432365088,0.923879532511288)) ;
#112966=DIRECTION('',(1.,0.,0.)) ;
#112967=DIRECTION('center_axis',(1.,0.,0.)) ;
#112968=DIRECTION('ref_axis',(0.,0.,-1.)) ;
#112969=DIRECTION('center_axis',(0.,1.,0.)) ;
#112970=DIRECTION('ref_axis',(0.,0.,1.)) ;
#112971=DIRECTION('',(0.,0.,-1.)) ;
#112972=DIRECTION('',(0.,0.,1.)) ;
#112973=DIRECTION('center_axis',(0.,-0.707106781186547,-0.707106781186548)) ;
#112974=DIRECTION('ref_axis',(0.,0.707106781186548,-0.707106781186547)) ;
#112975=DIRECTION('',(0.,-0.707106781186548,0.707106781186547)) ;
#112976=DIRECTION('',(1.,0.,0.)) ;
#112977=DIRECTION('',(0.,0.707106781186548,-0.707106781186547)) ;
#112978=DIRECTION('center_axis',(1.,0.,0.)) ;
#112979=DIRECTION('ref_axis',(0.,0.,-1.)) ;
#112980=DIRECTION('center_axis',(-1.,0.,0.)) ;
#112981=DIRECTION('ref_axis',(0.,0.,-1.)) ;
#112982=DIRECTION('',(1.,0.,0.)) ;
#112983=DIRECTION('center_axis',(1.,0.,0.)) ;
#112984=DIRECTION('ref_axis',(0.,0.,-1.)) ;
#112985=DIRECTION('center_axis',(0.,-1.,0.)) ;
#112986=DIRECTION('ref_axis',(0.,0.,-1.)) ;
#112987=DIRECTION('',(0.,0.,1.)) ;
#112988=DIRECTION('',(1.,0.,0.)) ;
#112989=DIRECTION('',(0.,0.,-1.)) ;
#112990=DIRECTION('center_axis',(1.,0.,0.)) ;
#112991=DIRECTION('ref_axis',(0.,0.,-1.)) ;
#112992=DIRECTION('center_axis',(1.,0.,0.)) ;
#112993=DIRECTION('ref_axis',(0.,0.,1.)) ;
#112994=DIRECTION('',(1.,0.,0.)) ;
#112995=DIRECTION('center_axis',(-1.,0.,0.)) ;
#112996=DIRECTION('ref_axis',(0.,0.,-1.)) ;
#112997=DIRECTION('center_axis',(0.,0.,-1.)) ;
#112998=DIRECTION('ref_axis',(-1.,0.,0.)) ;
#112999=DIRECTION('',(0.,-1.,0.)) ;
#113000=DIRECTION('',(1.,0.,0.)) ;
#113001=DIRECTION('',(0.,1.,0.)) ;
#113002=DIRECTION('center_axis',(1.,0.,0.)) ;
#113003=DIRECTION('ref_axis',(0.,0.,-1.)) ;
#113004=DIRECTION('center_axis',(1.,0.,0.)) ;
#113005=DIRECTION('ref_axis',(0.,0.,1.)) ;
#113006=DIRECTION('',(1.,0.,0.)) ;
#113007=DIRECTION('center_axis',(-1.,0.,0.)) ;
#113008=DIRECTION('ref_axis',(0.,0.,-1.)) ;
#113009=DIRECTION('center_axis',(0.,1.,0.)) ;
#113010=DIRECTION('ref_axis',(0.,0.,1.)) ;
#113011=DIRECTION('',(0.,0.,-1.)) ;
#113012=DIRECTION('',(1.,0.,0.)) ;
#113013=DIRECTION('',(0.,0.,1.)) ;
#113014=DIRECTION('center_axis',(1.,0.,0.)) ;
#113015=DIRECTION('ref_axis',(0.,0.,-1.)) ;
#113016=DIRECTION('center_axis',(-1.,0.,0.)) ;
#113017=DIRECTION('ref_axis',(0.,1.95156391047392E-14,-1.)) ;
#113018=DIRECTION('',(1.,0.,0.)) ;
#113019=DIRECTION('center_axis',(1.,0.,0.)) ;
#113020=DIRECTION('ref_axis',(0.,0.,-1.)) ;
#113021=DIRECTION('center_axis',(0.,1.07081696047951E-16,-1.)) ;
#113022=DIRECTION('ref_axis',(0.,1.,1.07081696047951E-16)) ;
#113023=DIRECTION('',(0.,-1.,-1.07081696047951E-16)) ;
#113024=DIRECTION('',(1.,0.,0.)) ;
#113025=DIRECTION('',(0.,1.,1.07081696047951E-16)) ;
#113026=DIRECTION('center_axis',(1.,0.,0.)) ;
#113027=DIRECTION('ref_axis',(0.,0.,-1.)) ;
#113028=DIRECTION('center_axis',(-1.,0.,0.)) ;
#113029=DIRECTION('ref_axis',(0.,0.,-1.)) ;
#113030=DIRECTION('',(1.,0.,0.)) ;
#113031=DIRECTION('center_axis',(1.,0.,0.)) ;
#113032=DIRECTION('ref_axis',(0.,0.,-1.)) ;
#113033=DIRECTION('center_axis',(0.,-1.,0.)) ;
#113034=DIRECTION('ref_axis',(0.,0.,-1.)) ;
#113035=DIRECTION('',(0.,0.,1.)) ;
#113036=DIRECTION('',(1.,0.,0.)) ;
#113037=DIRECTION('',(0.,0.,-1.)) ;
#113038=DIRECTION('center_axis',(1.,0.,0.)) ;
#113039=DIRECTION('ref_axis',(0.,0.,-1.)) ;
#113040=DIRECTION('center_axis',(-1.,0.,0.)) ;
#113041=DIRECTION('ref_axis',(0.,-4.33680868994204E-15,-1.)) ;
#113042=DIRECTION('',(1.,0.,0.)) ;
#113043=DIRECTION('center_axis',(1.,0.,0.)) ;
#113044=DIRECTION('ref_axis',(0.,0.,-1.)) ;
#113045=DIRECTION('center_axis',(1.,0.,0.)) ;
#113046=DIRECTION('ref_axis',(0.,0.,-1.)) ;
#113047=DIRECTION('center_axis',(1.,0.,0.)) ;
#113048=DIRECTION('ref_axis',(0.,-7.85535158932894E-16,1.)) ;
#113049=DIRECTION('',(1.,0.,0.)) ;
#113050=DIRECTION('center_axis',(-1.,0.,0.)) ;
#113051=DIRECTION('ref_axis',(0.,-7.85535158932894E-16,-1.)) ;
#113052=DIRECTION('center_axis',(1.,0.,0.)) ;
#113053=DIRECTION('ref_axis',(0.,0.,-1.)) ;
#113054=DIRECTION('center_axis',(-1.,0.,0.)) ;
#113055=DIRECTION('ref_axis',(0.,-8.67361737988409E-15,-1.)) ;
#113056=DIRECTION('',(1.,0.,0.)) ;
#113057=DIRECTION('center_axis',(1.,0.,0.)) ;
#113058=DIRECTION('ref_axis',(0.,0.,-1.)) ;
#113059=DIRECTION('center_axis',(0.,-1.,0.)) ;
#113060=DIRECTION('ref_axis',(0.,0.,-1.)) ;
#113061=DIRECTION('',(0.,0.,1.)) ;
#113062=DIRECTION('',(1.,0.,0.)) ;
#113063=DIRECTION('',(0.,0.,-1.)) ;
#113064=DIRECTION('center_axis',(1.,0.,0.)) ;
#113065=DIRECTION('ref_axis',(0.,0.,-1.)) ;
#113066=DIRECTION('center_axis',(-1.,0.,0.)) ;
#113067=DIRECTION('ref_axis',(0.,0.,-1.)) ;
#113068=DIRECTION('',(1.,0.,0.)) ;
#113069=DIRECTION('center_axis',(1.,0.,0.)) ;
#113070=DIRECTION('ref_axis',(0.,0.,-1.)) ;
#113071=DIRECTION('center_axis',(0.,-1.07081696047951E-16,1.)) ;
#113072=DIRECTION('ref_axis',(0.,-1.,-1.07081696047951E-16)) ;
#113073=DIRECTION('',(0.,1.,1.07081696047951E-16)) ;
#113074=DIRECTION('',(1.,0.,0.)) ;
#113075=DIRECTION('',(0.,-1.,-1.07081696047951E-16)) ;
#113076=DIRECTION('center_axis',(1.,0.,0.)) ;
#113077=DIRECTION('ref_axis',(0.,0.,-1.)) ;
#113078=DIRECTION('center_axis',(-1.,0.,0.)) ;
#113079=DIRECTION('ref_axis',(0.,0.,-1.)) ;
#113080=DIRECTION('',(1.,0.,0.)) ;
#113081=DIRECTION('center_axis',(1.,0.,0.)) ;
#113082=DIRECTION('ref_axis',(0.,0.,-1.)) ;
#113083=DIRECTION('center_axis',(0.,1.,0.)) ;
#113084=DIRECTION('ref_axis',(0.,0.,1.)) ;
#113085=DIRECTION('',(0.,0.,-1.)) ;
#113086=DIRECTION('',(0.,0.,1.)) ;
#113087=DIRECTION('center_axis',(-1.,0.,0.)) ;
#113088=DIRECTION('ref_axis',(0.,0.,1.)) ;
#113089=DIRECTION('center_axis',(-1.,0.,0.)) ;
#113090=DIRECTION('ref_axis',(0.,0.,1.)) ;
#113091=DIRECTION('',(0.,-1.,0.)) ;
#113092=DIRECTION('center_axis',(-1.,0.,0.)) ;
#113093=DIRECTION('ref_axis',(0.,0.,1.)) ;
#113094=DIRECTION('',(0.,0.,1.)) ;
#113095=DIRECTION('',(0.,-1.,-1.07081696047951E-16)) ;
#113096=DIRECTION('',(0.,0.,-1.)) ;
#113097=DIRECTION('center_axis',(-1.,0.,0.)) ;
#113098=DIRECTION('ref_axis',(0.,0.,1.)) ;
#113099=DIRECTION('',(0.,0.,-1.)) ;
#113100=DIRECTION('',(0.,1.,1.07081696047951E-16)) ;
#113101=DIRECTION('',(0.,0.,1.)) ;
#113102=DIRECTION('center_axis',(-1.,0.,0.)) ;
#113103=DIRECTION('ref_axis',(0.,0.,1.)) ;
#113104=DIRECTION('',(0.,1.,0.)) ;
#113105=DIRECTION('center_axis',(-1.,0.,0.)) ;
#113106=DIRECTION('ref_axis',(0.,0.,1.)) ;
#113107=DIRECTION('',(0.,0.,-1.)) ;
#113108=DIRECTION('',(0.,0.707106781186548,-0.707106781186547)) ;
#113109=DIRECTION('',(0.,0.,1.)) ;
#113110=DIRECTION('',(0.,-0.707106781186546,-0.707106781186549)) ;
#113111=DIRECTION('',(0.,-3.99416362155027E-15,-1.)) ;
#113112=DIRECTION('center_axis',(1.,0.,0.)) ;
#113113=DIRECTION('ref_axis',(0.,0.,-1.)) ;
#113114=DIRECTION('',(1.,0.,0.)) ;
#113115=DIRECTION('center_axis',(1.,0.,0.)) ;
#113116=DIRECTION('ref_axis',(0.,0.,1.)) ;
#113117=DIRECTION('',(1.,0.,0.)) ;
#113118=DIRECTION('center_axis',(-1.,0.,0.)) ;
#113119=DIRECTION('ref_axis',(0.,0.,-1.)) ;
#113120=DIRECTION('center_axis',(0.,0.,1.)) ;
#113121=DIRECTION('ref_axis',(1.,0.,0.)) ;
#113122=DIRECTION('',(0.,1.,0.)) ;
#113123=DIRECTION('',(1.,0.,0.)) ;
#113124=DIRECTION('',(0.,-1.,0.)) ;
#113125=DIRECTION('center_axis',(1.,0.,0.)) ;
#113126=DIRECTION('ref_axis',(0.,0.,-1.)) ;
#113127=DIRECTION('center_axis',(1.,0.,0.)) ;
#113128=DIRECTION('ref_axis',(0.,0.,1.)) ;
#113129=DIRECTION('',(1.,0.,0.)) ;
#113130=DIRECTION('center_axis',(-1.,0.,0.)) ;
#113131=DIRECTION('ref_axis',(0.,0.,-1.)) ;
#113132=DIRECTION('center_axis',(0.,-1.,3.99416362155027E-15)) ;
#113133=DIRECTION('ref_axis',(0.,-3.99416362155027E-15,-1.)) ;
#113134=DIRECTION('',(0.,3.99416362155027E-15,1.)) ;
#113135=DIRECTION('',(1.,0.,0.)) ;
#113136=DIRECTION('',(0.,-3.99416362155027E-15,-1.)) ;
#113137=DIRECTION('center_axis',(1.,0.,0.)) ;
#113138=DIRECTION('ref_axis',(0.,0.,-1.)) ;
#113139=DIRECTION('center_axis',(-1.,0.,0.)) ;
#113140=DIRECTION('ref_axis',(0.,0.,-1.)) ;
#113141=DIRECTION('',(1.,0.,0.)) ;
#113142=DIRECTION('center_axis',(1.,0.,0.)) ;
#113143=DIRECTION('ref_axis',(0.,0.,-1.)) ;
#113144=DIRECTION('center_axis',(0.,-0.707106781186549,0.707106781186546)) ;
#113145=DIRECTION('ref_axis',(0.,-0.707106781186546,-0.707106781186549)) ;
#113146=DIRECTION('',(0.,0.707106781186546,0.707106781186549)) ;
#113147=DIRECTION('',(1.,0.,0.)) ;
#113148=DIRECTION('',(0.,-0.707106781186546,-0.707106781186549)) ;
#113149=DIRECTION('center_axis',(1.,0.,0.)) ;
#113150=DIRECTION('ref_axis',(0.,0.382683432365092,0.923879532511286)) ;
#113151=DIRECTION('',(1.,0.,0.)) ;
#113152=DIRECTION('center_axis',(1.,0.,0.)) ;
#113153=DIRECTION('ref_axis',(0.,0.,-1.)) ;
#113154=DIRECTION('center_axis',(0.,1.,0.)) ;
#113155=DIRECTION('ref_axis',(0.,0.,1.)) ;
#113156=DIRECTION('',(0.,0.,-1.)) ;
#113157=DIRECTION('',(0.,0.,1.)) ;
#113158=DIRECTION('center_axis',(0.,-0.707106781186547,-0.707106781186548)) ;
#113159=DIRECTION('ref_axis',(0.,0.707106781186548,-0.707106781186547)) ;
#113160=DIRECTION('',(0.,-0.707106781186548,0.707106781186547)) ;
#113161=DIRECTION('',(1.,0.,0.)) ;
#113162=DIRECTION('',(0.,0.707106781186548,-0.707106781186547)) ;
#113163=DIRECTION('center_axis',(1.,0.,0.)) ;
#113164=DIRECTION('ref_axis',(0.,0.,-1.)) ;
#113165=DIRECTION('center_axis',(-1.,0.,0.)) ;
#113166=DIRECTION('ref_axis',(0.,0.,-1.)) ;
#113167=DIRECTION('',(1.,0.,0.)) ;
#113168=DIRECTION('center_axis',(1.,0.,0.)) ;
#113169=DIRECTION('ref_axis',(0.,0.,-1.)) ;
#113170=DIRECTION('center_axis',(0.,-1.,0.)) ;
#113171=DIRECTION('ref_axis',(0.,0.,-1.)) ;
#113172=DIRECTION('',(0.,0.,1.)) ;
#113173=DIRECTION('',(1.,0.,0.)) ;
#113174=DIRECTION('',(0.,0.,-1.)) ;
#113175=DIRECTION('center_axis',(1.,0.,0.)) ;
#113176=DIRECTION('ref_axis',(0.,0.,-1.)) ;
#113177=DIRECTION('center_axis',(1.,0.,0.)) ;
#113178=DIRECTION('ref_axis',(0.,0.,1.)) ;
#113179=DIRECTION('',(1.,0.,0.)) ;
#113180=DIRECTION('center_axis',(-1.,0.,0.)) ;
#113181=DIRECTION('ref_axis',(0.,0.,-1.)) ;
#113182=DIRECTION('center_axis',(0.,0.,-1.)) ;
#113183=DIRECTION('ref_axis',(-1.,0.,0.)) ;
#113184=DIRECTION('',(0.,-1.,0.)) ;
#113185=DIRECTION('',(1.,0.,0.)) ;
#113186=DIRECTION('',(0.,1.,0.)) ;
#113187=DIRECTION('center_axis',(1.,0.,0.)) ;
#113188=DIRECTION('ref_axis',(0.,0.,-1.)) ;
#113189=DIRECTION('center_axis',(1.,0.,0.)) ;
#113190=DIRECTION('ref_axis',(0.,0.,1.)) ;
#113191=DIRECTION('',(1.,0.,0.)) ;
#113192=DIRECTION('center_axis',(-1.,0.,0.)) ;
#113193=DIRECTION('ref_axis',(0.,0.,-1.)) ;
#113194=DIRECTION('center_axis',(0.,1.,0.)) ;
#113195=DIRECTION('ref_axis',(0.,0.,1.)) ;
#113196=DIRECTION('',(0.,0.,-1.)) ;
#113197=DIRECTION('',(1.,0.,0.)) ;
#113198=DIRECTION('',(0.,0.,1.)) ;
#113199=DIRECTION('center_axis',(1.,0.,0.)) ;
#113200=DIRECTION('ref_axis',(0.,0.,-1.)) ;
#113201=DIRECTION('center_axis',(-1.,0.,0.)) ;
#113202=DIRECTION('ref_axis',(0.,1.95156391047392E-14,-1.)) ;
#113203=DIRECTION('',(1.,0.,0.)) ;
#113204=DIRECTION('center_axis',(1.,0.,0.)) ;
#113205=DIRECTION('ref_axis',(0.,0.,-1.)) ;
#113206=DIRECTION('center_axis',(0.,1.07081696047951E-16,-1.)) ;
#113207=DIRECTION('ref_axis',(0.,1.,1.07081696047951E-16)) ;
#113208=DIRECTION('',(0.,-1.,-1.07081696047951E-16)) ;
#113209=DIRECTION('',(1.,0.,0.)) ;
#113210=DIRECTION('',(0.,1.,1.07081696047951E-16)) ;
#113211=DIRECTION('center_axis',(1.,0.,0.)) ;
#113212=DIRECTION('ref_axis',(0.,0.,-1.)) ;
#113213=DIRECTION('center_axis',(-1.,0.,0.)) ;
#113214=DIRECTION('ref_axis',(0.,0.,-1.)) ;
#113215=DIRECTION('',(1.,0.,0.)) ;
#113216=DIRECTION('center_axis',(1.,0.,0.)) ;
#113217=DIRECTION('ref_axis',(0.,0.,-1.)) ;
#113218=DIRECTION('center_axis',(0.,-1.,0.)) ;
#113219=DIRECTION('ref_axis',(0.,0.,-1.)) ;
#113220=DIRECTION('',(0.,0.,1.)) ;
#113221=DIRECTION('',(1.,0.,0.)) ;
#113222=DIRECTION('',(0.,0.,-1.)) ;
#113223=DIRECTION('center_axis',(1.,0.,0.)) ;
#113224=DIRECTION('ref_axis',(0.,0.,-1.)) ;
#113225=DIRECTION('center_axis',(-1.,0.,0.)) ;
#113226=DIRECTION('ref_axis',(0.,-4.33680868994204E-15,-1.)) ;
#113227=DIRECTION('',(1.,0.,0.)) ;
#113228=DIRECTION('center_axis',(1.,0.,0.)) ;
#113229=DIRECTION('ref_axis',(0.,0.,-1.)) ;
#113230=DIRECTION('center_axis',(1.,0.,0.)) ;
#113231=DIRECTION('ref_axis',(0.,0.,-1.)) ;
#113232=DIRECTION('center_axis',(1.,0.,0.)) ;
#113233=DIRECTION('ref_axis',(0.,-7.85535158932894E-16,1.)) ;
#113234=DIRECTION('',(1.,0.,0.)) ;
#113235=DIRECTION('center_axis',(-1.,0.,0.)) ;
#113236=DIRECTION('ref_axis',(0.,-7.85535158932894E-16,-1.)) ;
#113237=DIRECTION('center_axis',(1.,0.,0.)) ;
#113238=DIRECTION('ref_axis',(0.,0.,-1.)) ;
#113239=DIRECTION('center_axis',(-1.,0.,0.)) ;
#113240=DIRECTION('ref_axis',(0.,0.,-1.)) ;
#113241=DIRECTION('',(1.,0.,0.)) ;
#113242=DIRECTION('center_axis',(1.,0.,0.)) ;
#113243=DIRECTION('ref_axis',(0.,0.,-1.)) ;
#113244=DIRECTION('center_axis',(0.,-1.,0.)) ;
#113245=DIRECTION('ref_axis',(0.,0.,-1.)) ;
#113246=DIRECTION('',(0.,0.,1.)) ;
#113247=DIRECTION('',(1.,0.,0.)) ;
#113248=DIRECTION('',(0.,0.,-1.)) ;
#113249=DIRECTION('center_axis',(1.,0.,0.)) ;
#113250=DIRECTION('ref_axis',(0.,0.,-1.)) ;
#113251=DIRECTION('center_axis',(-1.,0.,0.)) ;
#113252=DIRECTION('ref_axis',(0.,0.,-1.)) ;
#113253=DIRECTION('',(1.,0.,0.)) ;
#113254=DIRECTION('center_axis',(1.,0.,0.)) ;
#113255=DIRECTION('ref_axis',(0.,0.,-1.)) ;
#113256=DIRECTION('center_axis',(0.,-1.07081696047951E-16,1.)) ;
#113257=DIRECTION('ref_axis',(0.,-1.,-1.07081696047951E-16)) ;
#113258=DIRECTION('',(0.,1.,1.07081696047951E-16)) ;
#113259=DIRECTION('',(1.,0.,0.)) ;
#113260=DIRECTION('',(0.,-1.,-1.07081696047951E-16)) ;
#113261=DIRECTION('center_axis',(1.,0.,0.)) ;
#113262=DIRECTION('ref_axis',(0.,0.,-1.)) ;
#113263=DIRECTION('center_axis',(-1.,0.,0.)) ;
#113264=DIRECTION('ref_axis',(0.,0.,-1.)) ;
#113265=DIRECTION('',(1.,0.,0.)) ;
#113266=DIRECTION('center_axis',(1.,0.,0.)) ;
#113267=DIRECTION('ref_axis',(0.,0.,-1.)) ;
#113268=DIRECTION('center_axis',(0.,1.,0.)) ;
#113269=DIRECTION('ref_axis',(0.,0.,1.)) ;
#113270=DIRECTION('',(0.,0.,-1.)) ;
#113271=DIRECTION('',(0.,0.,1.)) ;
#113272=DIRECTION('center_axis',(-1.,0.,0.)) ;
#113273=DIRECTION('ref_axis',(0.,0.,1.)) ;
#113274=DIRECTION('center_axis',(-1.,0.,0.)) ;
#113275=DIRECTION('ref_axis',(0.,0.,1.)) ;
#113276=DIRECTION('',(0.,-1.,0.)) ;
#113277=DIRECTION('center_axis',(-1.,0.,0.)) ;
#113278=DIRECTION('ref_axis',(0.,0.,1.)) ;
#113279=DIRECTION('',(0.,0.,1.)) ;
#113280=DIRECTION('',(0.,-1.,-1.07081696047951E-16)) ;
#113281=DIRECTION('',(0.,0.,-1.)) ;
#113282=DIRECTION('center_axis',(-1.,0.,0.)) ;
#113283=DIRECTION('ref_axis',(0.,0.,1.)) ;
#113284=DIRECTION('',(0.,0.,-1.)) ;
#113285=DIRECTION('',(0.,1.,1.07081696047951E-16)) ;
#113286=DIRECTION('',(0.,0.,1.)) ;
#113287=DIRECTION('center_axis',(-1.,0.,0.)) ;
#113288=DIRECTION('ref_axis',(0.,0.,1.)) ;
#113289=DIRECTION('',(0.,1.,0.)) ;
#113290=DIRECTION('center_axis',(-1.,0.,0.)) ;
#113291=DIRECTION('ref_axis',(0.,0.,1.)) ;
#113292=DIRECTION('',(0.,0.,-1.)) ;
#113293=DIRECTION('',(0.,0.707106781186548,-0.707106781186547)) ;
#113294=DIRECTION('',(0.,0.,1.)) ;
#113295=DIRECTION('',(0.,-0.707106781186546,-0.707106781186549)) ;
#113296=DIRECTION('',(0.,-3.99416362155027E-15,-1.)) ;
#113297=DIRECTION('center_axis',(1.,0.,0.)) ;
#113298=DIRECTION('ref_axis',(0.,0.,-1.)) ;
#113299=DIRECTION('',(1.,0.,0.)) ;
#113300=DIRECTION('center_axis',(1.,0.,0.)) ;
#113301=DIRECTION('ref_axis',(0.,0.,1.)) ;
#113302=DIRECTION('',(1.,0.,0.)) ;
#113303=DIRECTION('center_axis',(-1.,0.,0.)) ;
#113304=DIRECTION('ref_axis',(0.,0.,-1.)) ;
#113305=DIRECTION('center_axis',(0.,0.,1.)) ;
#113306=DIRECTION('ref_axis',(1.,0.,0.)) ;
#113307=DIRECTION('',(0.,1.,0.)) ;
#113308=DIRECTION('',(1.,0.,0.)) ;
#113309=DIRECTION('',(0.,-1.,0.)) ;
#113310=DIRECTION('center_axis',(1.,0.,0.)) ;
#113311=DIRECTION('ref_axis',(0.,0.,-1.)) ;
#113312=DIRECTION('center_axis',(1.,0.,0.)) ;
#113313=DIRECTION('ref_axis',(0.,0.,1.)) ;
#113314=DIRECTION('',(1.,0.,0.)) ;
#113315=DIRECTION('center_axis',(-1.,0.,0.)) ;
#113316=DIRECTION('ref_axis',(0.,0.,-1.)) ;
#113317=DIRECTION('center_axis',(0.,-1.,3.99416362155027E-15)) ;
#113318=DIRECTION('ref_axis',(0.,-3.99416362155027E-15,-1.)) ;
#113319=DIRECTION('',(0.,3.99416362155027E-15,1.)) ;
#113320=DIRECTION('',(1.,0.,0.)) ;
#113321=DIRECTION('',(0.,-3.99416362155027E-15,-1.)) ;
#113322=DIRECTION('center_axis',(1.,0.,0.)) ;
#113323=DIRECTION('ref_axis',(0.,0.,-1.)) ;
#113324=DIRECTION('center_axis',(-1.,0.,0.)) ;
#113325=DIRECTION('ref_axis',(0.,0.,-1.)) ;
#113326=DIRECTION('',(1.,0.,0.)) ;
#113327=DIRECTION('center_axis',(1.,0.,0.)) ;
#113328=DIRECTION('ref_axis',(0.,0.,-1.)) ;
#113329=DIRECTION('center_axis',(0.,-0.707106781186549,0.707106781186546)) ;
#113330=DIRECTION('ref_axis',(0.,-0.707106781186546,-0.707106781186549)) ;
#113331=DIRECTION('',(0.,0.707106781186546,0.707106781186549)) ;
#113332=DIRECTION('',(1.,0.,0.)) ;
#113333=DIRECTION('',(0.,-0.707106781186546,-0.707106781186549)) ;
#113334=DIRECTION('center_axis',(1.,0.,0.)) ;
#113335=DIRECTION('ref_axis',(0.,0.382683432365092,0.923879532511286)) ;
#113336=DIRECTION('',(1.,0.,0.)) ;
#113337=DIRECTION('center_axis',(1.,0.,0.)) ;
#113338=DIRECTION('ref_axis',(0.,0.,-1.)) ;
#113339=DIRECTION('center_axis',(0.,1.,0.)) ;
#113340=DIRECTION('ref_axis',(0.,0.,1.)) ;
#113341=DIRECTION('',(0.,0.,-1.)) ;
#113342=DIRECTION('',(0.,0.,1.)) ;
#113343=DIRECTION('center_axis',(0.,-0.707106781186547,-0.707106781186548)) ;
#113344=DIRECTION('ref_axis',(0.,0.707106781186548,-0.707106781186547)) ;
#113345=DIRECTION('',(0.,-0.707106781186548,0.707106781186547)) ;
#113346=DIRECTION('',(1.,0.,0.)) ;
#113347=DIRECTION('',(0.,0.707106781186548,-0.707106781186547)) ;
#113348=DIRECTION('center_axis',(1.,0.,0.)) ;
#113349=DIRECTION('ref_axis',(0.,0.,-1.)) ;
#113350=DIRECTION('center_axis',(-1.,0.,0.)) ;
#113351=DIRECTION('ref_axis',(0.,0.,-1.)) ;
#113352=DIRECTION('',(1.,0.,0.)) ;
#113353=DIRECTION('center_axis',(1.,0.,0.)) ;
#113354=DIRECTION('ref_axis',(0.,0.,-1.)) ;
#113355=DIRECTION('center_axis',(0.,-1.,0.)) ;
#113356=DIRECTION('ref_axis',(0.,0.,-1.)) ;
#113357=DIRECTION('',(0.,0.,1.)) ;
#113358=DIRECTION('',(1.,0.,0.)) ;
#113359=DIRECTION('',(0.,0.,-1.)) ;
#113360=DIRECTION('center_axis',(1.,0.,0.)) ;
#113361=DIRECTION('ref_axis',(0.,0.,-1.)) ;
#113362=DIRECTION('center_axis',(1.,0.,0.)) ;
#113363=DIRECTION('ref_axis',(0.,0.,1.)) ;
#113364=DIRECTION('',(1.,0.,0.)) ;
#113365=DIRECTION('center_axis',(-1.,0.,0.)) ;
#113366=DIRECTION('ref_axis',(0.,0.,-1.)) ;
#113367=DIRECTION('center_axis',(0.,0.,-1.)) ;
#113368=DIRECTION('ref_axis',(-1.,0.,0.)) ;
#113369=DIRECTION('',(0.,-1.,0.)) ;
#113370=DIRECTION('',(1.,0.,0.)) ;
#113371=DIRECTION('',(0.,1.,0.)) ;
#113372=DIRECTION('center_axis',(1.,0.,0.)) ;
#113373=DIRECTION('ref_axis',(0.,0.,-1.)) ;
#113374=DIRECTION('center_axis',(1.,0.,0.)) ;
#113375=DIRECTION('ref_axis',(0.,0.,1.)) ;
#113376=DIRECTION('',(1.,0.,0.)) ;
#113377=DIRECTION('center_axis',(-1.,0.,0.)) ;
#113378=DIRECTION('ref_axis',(0.,0.,-1.)) ;
#113379=DIRECTION('center_axis',(0.,1.,0.)) ;
#113380=DIRECTION('ref_axis',(0.,0.,1.)) ;
#113381=DIRECTION('',(0.,0.,-1.)) ;
#113382=DIRECTION('',(1.,0.,0.)) ;
#113383=DIRECTION('',(0.,0.,1.)) ;
#113384=DIRECTION('center_axis',(1.,0.,0.)) ;
#113385=DIRECTION('ref_axis',(0.,0.,-1.)) ;
#113386=DIRECTION('center_axis',(-1.,0.,0.)) ;
#113387=DIRECTION('ref_axis',(0.,1.7347234759768E-14,-1.)) ;
#113388=DIRECTION('',(1.,0.,0.)) ;
#113389=DIRECTION('center_axis',(1.,0.,0.)) ;
#113390=DIRECTION('ref_axis',(0.,0.,-1.)) ;
#113391=DIRECTION('center_axis',(0.,1.07081696047951E-16,-1.)) ;
#113392=DIRECTION('ref_axis',(0.,1.,1.07081696047951E-16)) ;
#113393=DIRECTION('',(0.,-1.,-1.07081696047951E-16)) ;
#113394=DIRECTION('',(1.,0.,0.)) ;
#113395=DIRECTION('',(0.,1.,1.07081696047951E-16)) ;
#113396=DIRECTION('center_axis',(1.,0.,0.)) ;
#113397=DIRECTION('ref_axis',(0.,0.,-1.)) ;
#113398=DIRECTION('center_axis',(-1.,0.,0.)) ;
#113399=DIRECTION('ref_axis',(0.,0.,-1.)) ;
#113400=DIRECTION('',(1.,0.,0.)) ;
#113401=DIRECTION('center_axis',(1.,0.,0.)) ;
#113402=DIRECTION('ref_axis',(0.,0.,-1.)) ;
#113403=DIRECTION('center_axis',(0.,-1.,0.)) ;
#113404=DIRECTION('ref_axis',(0.,0.,-1.)) ;
#113405=DIRECTION('',(0.,0.,1.)) ;
#113406=DIRECTION('',(1.,0.,0.)) ;
#113407=DIRECTION('',(0.,0.,-1.)) ;
#113408=DIRECTION('center_axis',(1.,0.,0.)) ;
#113409=DIRECTION('ref_axis',(0.,0.,-1.)) ;
#113410=DIRECTION('center_axis',(-1.,0.,0.)) ;
#113411=DIRECTION('ref_axis',(0.,0.,-1.)) ;
#113412=DIRECTION('',(1.,0.,0.)) ;
#113413=DIRECTION('center_axis',(1.,0.,0.)) ;
#113414=DIRECTION('ref_axis',(0.,0.,-1.)) ;
#113415=DIRECTION('center_axis',(1.,0.,0.)) ;
#113416=DIRECTION('ref_axis',(0.,0.,-1.)) ;
#113417=DIRECTION('center_axis',(1.,0.,0.)) ;
#113418=DIRECTION('ref_axis',(0.,-7.85535158932894E-16,1.)) ;
#113419=DIRECTION('',(1.,0.,0.)) ;
#113420=DIRECTION('center_axis',(-1.,0.,0.)) ;
#113421=DIRECTION('ref_axis',(0.,-7.85535158932894E-16,-1.)) ;
#113422=DIRECTION('center_axis',(1.,0.,0.)) ;
#113423=DIRECTION('ref_axis',(0.,0.,-1.)) ;
#113424=DIRECTION('center_axis',(-1.,0.,0.)) ;
#113425=DIRECTION('ref_axis',(0.,0.,-1.)) ;
#113426=DIRECTION('',(1.,0.,0.)) ;
#113427=DIRECTION('center_axis',(1.,0.,0.)) ;
#113428=DIRECTION('ref_axis',(0.,0.,-1.)) ;
#113429=DIRECTION('center_axis',(0.,-1.,0.)) ;
#113430=DIRECTION('ref_axis',(0.,0.,-1.)) ;
#113431=DIRECTION('',(0.,0.,1.)) ;
#113432=DIRECTION('',(1.,0.,0.)) ;
#113433=DIRECTION('',(0.,0.,-1.)) ;
#113434=DIRECTION('center_axis',(1.,0.,0.)) ;
#113435=DIRECTION('ref_axis',(0.,0.,-1.)) ;
#113436=DIRECTION('center_axis',(-1.,0.,0.)) ;
#113437=DIRECTION('ref_axis',(0.,0.,-1.)) ;
#113438=DIRECTION('',(1.,0.,0.)) ;
#113439=DIRECTION('center_axis',(1.,0.,0.)) ;
#113440=DIRECTION('ref_axis',(0.,0.,-1.)) ;
#113441=DIRECTION('center_axis',(0.,-1.07081696047951E-16,1.)) ;
#113442=DIRECTION('ref_axis',(0.,-1.,-1.07081696047951E-16)) ;
#113443=DIRECTION('',(0.,1.,1.07081696047951E-16)) ;
#113444=DIRECTION('',(1.,0.,0.)) ;
#113445=DIRECTION('',(0.,-1.,-1.07081696047951E-16)) ;
#113446=DIRECTION('center_axis',(1.,0.,0.)) ;
#113447=DIRECTION('ref_axis',(0.,0.,-1.)) ;
#113448=DIRECTION('center_axis',(-1.,0.,0.)) ;
#113449=DIRECTION('ref_axis',(0.,0.,-1.)) ;
#113450=DIRECTION('',(1.,0.,0.)) ;
#113451=DIRECTION('center_axis',(1.,0.,0.)) ;
#113452=DIRECTION('ref_axis',(0.,0.,-1.)) ;
#113453=DIRECTION('center_axis',(0.,1.,0.)) ;
#113454=DIRECTION('ref_axis',(0.,0.,1.)) ;
#113455=DIRECTION('',(0.,0.,-1.)) ;
#113456=DIRECTION('',(0.,0.,1.)) ;
#113457=DIRECTION('center_axis',(-1.,0.,0.)) ;
#113458=DIRECTION('ref_axis',(0.,0.,1.)) ;
#113459=DIRECTION('center_axis',(-1.,0.,0.)) ;
#113460=DIRECTION('ref_axis',(0.,0.,1.)) ;
#113461=DIRECTION('',(0.,-1.,0.)) ;
#113462=DIRECTION('center_axis',(-1.,0.,0.)) ;
#113463=DIRECTION('ref_axis',(0.,0.,1.)) ;
#113464=DIRECTION('',(0.,0.,1.)) ;
#113465=DIRECTION('',(0.,-1.,-1.07081696047951E-16)) ;
#113466=DIRECTION('',(0.,0.,-1.)) ;
#113467=DIRECTION('center_axis',(-1.,0.,0.)) ;
#113468=DIRECTION('ref_axis',(0.,0.,1.)) ;
#113469=DIRECTION('',(0.,0.,-1.)) ;
#113470=DIRECTION('',(0.,1.,1.07081696047951E-16)) ;
#113471=DIRECTION('',(0.,0.,1.)) ;
#113472=DIRECTION('center_axis',(-1.,0.,0.)) ;
#113473=DIRECTION('ref_axis',(0.,0.,1.)) ;
#113474=DIRECTION('',(0.,1.,0.)) ;
#113475=DIRECTION('center_axis',(-1.,0.,0.)) ;
#113476=DIRECTION('ref_axis',(0.,0.,1.)) ;
#113477=DIRECTION('',(0.,0.,-1.)) ;
#113478=DIRECTION('',(0.,0.707106781186548,-0.707106781186547)) ;
#113479=DIRECTION('',(0.,0.,1.)) ;
#113480=DIRECTION('',(0.,-0.707106781186546,-0.707106781186549)) ;
#113481=DIRECTION('',(0.,-3.99416362155027E-15,-1.)) ;
#113482=DIRECTION('center_axis',(1.,0.,0.)) ;
#113483=DIRECTION('ref_axis',(0.,0.,-1.)) ;
#113484=DIRECTION('',(0.,-1.,0.)) ;
#113485=DIRECTION('center_axis',(-1.,0.,0.)) ;
#113486=DIRECTION('ref_axis',(0.,0.,-1.)) ;
#113487=DIRECTION('',(0.,0.,-1.)) ;
#113488=DIRECTION('center_axis',(-1.,0.,0.)) ;
#113489=DIRECTION('ref_axis',(0.,1.0842021724855E-15,-1.)) ;
#113490=DIRECTION('',(0.,-1.,0.)) ;
#113491=DIRECTION('center_axis',(-1.,0.,0.)) ;
#113492=DIRECTION('ref_axis',(0.,0.,-1.)) ;
#113493=DIRECTION('',(0.,0.,1.)) ;
#113494=DIRECTION('center_axis',(-1.,0.,0.)) ;
#113495=DIRECTION('ref_axis',(0.,0.,-1.)) ;
#113496=DIRECTION('center_axis',(1.,0.,0.)) ;
#113497=DIRECTION('ref_axis',(0.,0.,-1.)) ;
#113498=DIRECTION('',(0.,-1.,0.)) ;
#113499=DIRECTION('center_axis',(-1.,0.,0.)) ;
#113500=DIRECTION('ref_axis',(0.,0.,-1.)) ;
#113501=DIRECTION('',(0.,0.,-1.)) ;
#113502=DIRECTION('center_axis',(-1.,0.,0.)) ;
#113503=DIRECTION('ref_axis',(0.,-1.62630325872827E-15,-1.)) ;
#113504=DIRECTION('',(0.,-1.,0.)) ;
#113505=DIRECTION('center_axis',(-1.,0.,0.)) ;
#113506=DIRECTION('ref_axis',(0.,0.,-1.)) ;
#113507=DIRECTION('',(0.,0.,1.)) ;
#113508=DIRECTION('center_axis',(-1.,0.,0.)) ;
#113509=DIRECTION('ref_axis',(0.,0.,-1.)) ;
#113510=DIRECTION('center_axis',(1.,0.,0.)) ;
#113511=DIRECTION('ref_axis',(0.,0.,-1.)) ;
#113512=DIRECTION('',(0.,-1.,0.)) ;
#113513=DIRECTION('center_axis',(-1.,0.,0.)) ;
#113514=DIRECTION('ref_axis',(0.,0.,-1.)) ;
#113515=DIRECTION('',(0.,0.,-1.)) ;
#113516=DIRECTION('center_axis',(-1.,0.,0.)) ;
#113517=DIRECTION('ref_axis',(0.,0.,-1.)) ;
#113518=DIRECTION('',(0.,-1.,0.)) ;
#113519=DIRECTION('center_axis',(-1.,0.,0.)) ;
#113520=DIRECTION('ref_axis',(0.,0.,-1.)) ;
#113521=DIRECTION('',(0.,0.,1.)) ;
#113522=DIRECTION('center_axis',(-1.,0.,0.)) ;
#113523=DIRECTION('ref_axis',(0.,0.,-1.)) ;
#113524=DIRECTION('center_axis',(1.,0.,0.)) ;
#113525=DIRECTION('ref_axis',(0.,0.,-1.)) ;
#113526=DIRECTION('',(0.,-1.,0.)) ;
#113527=DIRECTION('center_axis',(-1.,0.,0.)) ;
#113528=DIRECTION('ref_axis',(0.,0.,-1.)) ;
#113529=DIRECTION('',(0.,0.,-1.)) ;
#113530=DIRECTION('center_axis',(-1.,0.,0.)) ;
#113531=DIRECTION('ref_axis',(0.,-1.62630325872827E-15,-1.)) ;
#113532=DIRECTION('',(0.,-1.,0.)) ;
#113533=DIRECTION('center_axis',(-1.,0.,0.)) ;
#113534=DIRECTION('ref_axis',(0.,0.,-1.)) ;
#113535=DIRECTION('',(0.,0.,1.)) ;
#113536=DIRECTION('center_axis',(-1.,0.,0.)) ;
#113537=DIRECTION('ref_axis',(0.,0.,-1.)) ;
#113538=DIRECTION('center_axis',(1.,0.,0.)) ;
#113539=DIRECTION('ref_axis',(0.,0.,-1.)) ;
#113540=DIRECTION('',(0.,-1.,0.)) ;
#113541=DIRECTION('center_axis',(-1.,0.,0.)) ;
#113542=DIRECTION('ref_axis',(0.,0.,-1.)) ;
#113543=DIRECTION('',(0.,0.,-1.)) ;
#113544=DIRECTION('center_axis',(-1.,0.,0.)) ;
#113545=DIRECTION('ref_axis',(0.,0.,-1.)) ;
#113546=DIRECTION('',(0.,-1.,0.)) ;
#113547=DIRECTION('center_axis',(-1.,0.,0.)) ;
#113548=DIRECTION('ref_axis',(0.,0.,-1.)) ;
#113549=DIRECTION('',(0.,0.,1.)) ;
#113550=DIRECTION('center_axis',(-1.,0.,0.)) ;
#113551=DIRECTION('ref_axis',(0.,0.,-1.)) ;
#113552=DIRECTION('center_axis',(1.,0.,0.)) ;
#113553=DIRECTION('ref_axis',(0.,0.,-1.)) ;
#113554=DIRECTION('',(0.,-1.,0.)) ;
#113555=DIRECTION('center_axis',(-1.,0.,0.)) ;
#113556=DIRECTION('ref_axis',(0.,0.,-1.)) ;
#113557=DIRECTION('',(0.,0.,-1.)) ;
#113558=DIRECTION('center_axis',(-1.,0.,0.)) ;
#113559=DIRECTION('ref_axis',(0.,0.,-1.)) ;
#113560=DIRECTION('',(0.,-1.,0.)) ;
#113561=DIRECTION('center_axis',(-1.,0.,0.)) ;
#113562=DIRECTION('ref_axis',(0.,0.,-1.)) ;
#113563=DIRECTION('',(0.,0.,1.)) ;
#113564=DIRECTION('center_axis',(-1.,0.,0.)) ;
#113565=DIRECTION('ref_axis',(0.,0.,-1.)) ;
#113566=DIRECTION('center_axis',(1.,0.,0.)) ;
#113567=DIRECTION('ref_axis',(0.,0.,-1.)) ;
#113568=DIRECTION('',(0.,-1.,0.)) ;
#113569=DIRECTION('center_axis',(-1.,0.,0.)) ;
#113570=DIRECTION('ref_axis',(0.,0.,-1.)) ;
#113571=DIRECTION('',(0.,0.,-1.)) ;
#113572=DIRECTION('center_axis',(-1.,0.,0.)) ;
#113573=DIRECTION('ref_axis',(0.,0.,-1.)) ;
#113574=DIRECTION('',(0.,-1.,0.)) ;
#113575=DIRECTION('center_axis',(-1.,0.,0.)) ;
#113576=DIRECTION('ref_axis',(0.,0.,-1.)) ;
#113577=DIRECTION('',(0.,0.,1.)) ;
#113578=DIRECTION('center_axis',(-1.,0.,0.)) ;
#113579=DIRECTION('ref_axis',(0.,0.,-1.)) ;
#113580=DIRECTION('center_axis',(1.,0.,0.)) ;
#113581=DIRECTION('ref_axis',(0.,0.,-1.)) ;
#113582=DIRECTION('',(0.,-1.,0.)) ;
#113583=DIRECTION('center_axis',(-1.,0.,0.)) ;
#113584=DIRECTION('ref_axis',(0.,0.,-1.)) ;
#113585=DIRECTION('',(0.,0.,-1.)) ;
#113586=DIRECTION('center_axis',(-1.,0.,0.)) ;
#113587=DIRECTION('ref_axis',(0.,0.,-1.)) ;
#113588=DIRECTION('',(0.,-1.,0.)) ;
#113589=DIRECTION('center_axis',(-1.,0.,0.)) ;
#113590=DIRECTION('ref_axis',(0.,0.,-1.)) ;
#113591=DIRECTION('',(0.,0.,1.)) ;
#113592=DIRECTION('center_axis',(-1.,0.,0.)) ;
#113593=DIRECTION('ref_axis',(0.,0.,-1.)) ;
#113594=DIRECTION('center_axis',(1.,0.,0.)) ;
#113595=DIRECTION('ref_axis',(0.,0.,-1.)) ;
#113596=DIRECTION('',(0.,-1.,0.)) ;
#113597=DIRECTION('center_axis',(-1.,0.,0.)) ;
#113598=DIRECTION('ref_axis',(0.,0.,-1.)) ;
#113599=DIRECTION('',(0.,0.,-1.)) ;
#113600=DIRECTION('center_axis',(-1.,0.,0.)) ;
#113601=DIRECTION('ref_axis',(0.,0.,-1.)) ;
#113602=DIRECTION('',(0.,-1.,0.)) ;
#113603=DIRECTION('center_axis',(-1.,0.,0.)) ;
#113604=DIRECTION('ref_axis',(0.,0.,-1.)) ;
#113605=DIRECTION('',(0.,0.,1.)) ;
#113606=DIRECTION('center_axis',(-1.,0.,0.)) ;
#113607=DIRECTION('ref_axis',(0.,0.,-1.)) ;
#113608=DIRECTION('center_axis',(1.53063836115601E-16,-1.,-1.30104260698261E-16)) ;
#113609=DIRECTION('ref_axis',(1.,1.53063836115601E-16,1.99142572374599E-32)) ;
#113610=DIRECTION('center_axis',(0.,1.,0.)) ;
#113611=DIRECTION('ref_axis',(0.,0.,1.)) ;
#113612=DIRECTION('center_axis',(0.,-1.,0.)) ;
#113613=DIRECTION('ref_axis',(0.,0.,-1.)) ;
#113614=DIRECTION('center_axis',(1.,1.53063836115601E-16,2.73691106313441E-48)) ;
#113615=DIRECTION('ref_axis',(-1.53063836115601E-16,1.,-4.18922106430579E-64)) ;
#113616=DIRECTION('center_axis',(-1.,0.,0.)) ;
#113617=DIRECTION('ref_axis',(0.,0.,1.)) ;
#113618=DIRECTION('center_axis',(1.,1.53063836115601E-16,0.)) ;
#113619=DIRECTION('ref_axis',(1.53063836115601E-16,-1.,0.)) ;
#113620=DIRECTION('center_axis',(0.,1.,0.)) ;
#113621=DIRECTION('ref_axis',(1.,0.,0.)) ;
#113622=DIRECTION('center_axis',(0.,1.,0.)) ;
#113623=DIRECTION('ref_axis',(0.,0.,-1.)) ;
#113624=DIRECTION('center_axis',(0.,0.,1.)) ;
#113625=DIRECTION('ref_axis',(-1.,0.,0.)) ;
#113626=DIRECTION('center_axis',(0.,1.,0.)) ;
#113627=DIRECTION('ref_axis',(1.,0.,0.)) ;
#113628=DIRECTION('center_axis',(0.,0.,1.)) ;
#113629=DIRECTION('ref_axis',(-1.,0.,0.)) ;
#113630=DIRECTION('center_axis',(1.,1.0842021724855E-15,0.)) ;
#113631=DIRECTION('ref_axis',(1.0842021724855E-15,-1.,0.)) ;
#113632=DIRECTION('center_axis',(-1.,-1.53063836115601E-16,0.)) ;
#113633=DIRECTION('ref_axis',(0.,-1.,0.)) ;
#113634=DIRECTION('center_axis',(0.,0.,-1.)) ;
#113635=DIRECTION('ref_axis',(1.,0.,0.)) ;
#113636=DIRECTION('center_axis',(0.,0.,-1.)) ;
#113637=DIRECTION('ref_axis',(0.804034447892617,0.594582716366709,0.)) ;
#113638=DIRECTION('center_axis',(0.,0.,1.)) ;
#113639=DIRECTION('ref_axis',(1.,0.,0.)) ;
#113640=DIRECTION('',(0.,0.,-1.)) ;
#113641=DIRECTION('center_axis',(-2.16840434497101E-16,1.,1.30104260698261E-16)) ;
#113642=DIRECTION('ref_axis',(1.,2.16840434497101E-16,1.22464679914735E-16)) ;
#113643=DIRECTION('',(-2.16840434497101E-16,1.,1.30104260698261E-16)) ;
#113644=DIRECTION('center_axis',(0.,1.,0.)) ;
#113645=DIRECTION('ref_axis',(0.,0.,1.)) ;
#113646=DIRECTION('center_axis',(-1.,-1.53063836115601E-16,-2.73691106313441E-48)) ;
#113647=DIRECTION('ref_axis',(1.53063836115601E-16,-1.,4.18922106430579E-64)) ;
#113648=DIRECTION('center_axis',(1.,2.16840434497101E-16,0.)) ;
#113649=DIRECTION('ref_axis',(2.16840434497101E-16,-1.,0.)) ;
#113650=DIRECTION('center_axis',(0.,0.,1.)) ;
#113651=DIRECTION('ref_axis',(1.,0.,0.)) ;
#113652=DIRECTION('center_axis',(-1.25542992828747E-32,1.020425574104E-16,
1.)) ;
#113653=DIRECTION('ref_axis',(-1.28107280532009E-48,-1.,1.020425574104E-16)) ;
#113654=DIRECTION('center_axis',(0.,0.,1.)) ;
#113655=DIRECTION('ref_axis',(1.,0.,0.)) ;
#113656=DIRECTION('center_axis',(0.,0.,-1.)) ;
#113657=DIRECTION('ref_axis',(-1.,0.,0.)) ;
#113658=DIRECTION('center_axis',(1.,1.53063836115601E-16,-2.73691106313441E-48)) ;
#113659=DIRECTION('ref_axis',(-1.53063836115601E-16,1.,4.18922106430579E-64)) ;
#113660=DIRECTION('center_axis',(-1.,0.,0.)) ;
#113661=DIRECTION('ref_axis',(0.,0.,1.)) ;
#113662=DIRECTION('center_axis',(1.,1.53063836115601E-16,0.)) ;
#113663=DIRECTION('ref_axis',(1.53063836115601E-16,-1.,0.)) ;
#113664=DIRECTION('center_axis',(0.,1.,0.)) ;
#113665=DIRECTION('ref_axis',(1.,0.,0.)) ;
#113666=DIRECTION('center_axis',(-1.,-2.16840434497101E-16,0.)) ;
#113667=DIRECTION('ref_axis',(0.,-1.,0.)) ;
#113668=DIRECTION('center_axis',(0.,0.,-1.)) ;
#113669=DIRECTION('ref_axis',(1.,0.,0.)) ;
#113670=DIRECTION('center_axis',(-1.25542992828747E-32,1.020425574104E-16,
1.)) ;
#113671=DIRECTION('ref_axis',(0.,-1.,0.)) ;
#113672=DIRECTION('center_axis',(0.,-1.,0.)) ;
#113673=DIRECTION('ref_axis',(-6.50521303491304E-15,0.,1.)) ;
#113674=DIRECTION('center_axis',(-1.,0.,0.)) ;
#113675=DIRECTION('ref_axis',(0.,0.,-1.)) ;
#113676=DIRECTION('center_axis',(-1.,-1.53063836115601E-16,0.)) ;
#113677=DIRECTION('ref_axis',(0.,-1.,0.)) ;
#113678=DIRECTION('center_axis',(0.,-1.,0.)) ;
#113679=DIRECTION('ref_axis',(0.,0.,1.)) ;
#113680=DIRECTION('center_axis',(0.,0.,-1.)) ;
#113681=DIRECTION('ref_axis',(-1.,0.,0.)) ;
#113682=DIRECTION('center_axis',(-4.33680868994202E-15,0.,-1.)) ;
#113683=DIRECTION('ref_axis',(-1.,0.,4.33680868994202E-15)) ;
#113684=DIRECTION('center_axis',(1.,1.53063836115601E-16,-3.06472600140763E-33)) ;
#113685=DIRECTION('ref_axis',(-1.53063836115601E-16,1.,4.69098718418678E-49)) ;
#113686=DIRECTION('center_axis',(-1.,0.,0.)) ;
#113687=DIRECTION('ref_axis',(0.,0.,1.)) ;
#113688=DIRECTION('center_axis',(-1.53063836115601E-16,1.,-1.020425574104E-16)) ;
#113689=DIRECTION('ref_axis',(-1.,-1.53063836115601E-16,1.3684555315672E-47)) ;
#113690=DIRECTION('',(1.53063836115601E-16,-1.,1.020425574104E-16)) ;
#113691=DIRECTION('center_axis',(0.,-1.,0.)) ;
#113692=DIRECTION('ref_axis',(0.,0.,-1.)) ;
#113693=DIRECTION('center_axis',(-1.53063836115601E-16,1.,-1.30104260698261E-16)) ;
#113694=DIRECTION('ref_axis',(-1.,-1.53063836115601E-16,1.99142572374599E-32)) ;
#113695=DIRECTION('center_axis',(0.,-1.,0.)) ;
#113696=DIRECTION('ref_axis',(0.,0.,-1.)) ;
#113697=DIRECTION('center_axis',(-1.,-1.53063836115601E-16,2.73691106313441E-48)) ;
#113698=DIRECTION('ref_axis',(1.53063836115601E-16,-1.,-4.18922106430579E-64)) ;
#113699=DIRECTION('center_axis',(1.,2.16840434497101E-16,0.)) ;
#113700=DIRECTION('ref_axis',(2.16840434497101E-16,-1.,0.)) ;
#113701=DIRECTION('center_axis',(-1.,0.,2.168404344971E-15)) ;
#113702=DIRECTION('ref_axis',(2.168404344971E-15,0.,1.)) ;
#113703=DIRECTION('center_axis',(-1.,-2.16840434497101E-16,0.)) ;
#113704=DIRECTION('ref_axis',(0.,-1.,0.)) ;
#113705=DIRECTION('center_axis',(0.,0.,1.)) ;
#113706=DIRECTION('ref_axis',(-1.,0.,0.)) ;
#113707=DIRECTION('center_axis',(0.,1.,0.)) ;
#113708=DIRECTION('ref_axis',(1.,0.,0.)) ;
#113709=DIRECTION('center_axis',(0.,1.,0.)) ;
#113710=DIRECTION('ref_axis',(0.,0.,-1.)) ;
#113711=DIRECTION('center_axis',(1.,0.,0.)) ;
#113712=DIRECTION('ref_axis',(0.,-1.,0.)) ;
#113713=DIRECTION('center_axis',(1.,6.50521303491304E-15,0.)) ;
#113714=DIRECTION('ref_axis',(-6.50521303491304E-15,1.,0.)) ;
#113715=DIRECTION('center_axis',(8.67361737988403E-15,1.,0.)) ;
#113716=DIRECTION('ref_axis',(-1.,8.67361737988403E-15,0.)) ;
#113717=DIRECTION('center_axis',(1.2303003375722E-16,-1.,1.020425574104E-16)) ;
#113718=DIRECTION('ref_axis',(1.,1.2303003375722E-16,-1.25542992828747E-32)) ;
#113719=DIRECTION('center_axis',(0.,1.,0.)) ;
#113720=DIRECTION('ref_axis',(0.,0.,1.)) ;
#113721=DIRECTION('center_axis',(0.,1.,0.)) ;
#113722=DIRECTION('ref_axis',(1.,0.,0.)) ;
#113723=DIRECTION('center_axis',(1.,1.2303003375722E-16,0.)) ;
#113724=DIRECTION('ref_axis',(1.2303003375722E-16,-1.,0.)) ;
#113725=DIRECTION('center_axis',(0.,0.,1.)) ;
#113726=DIRECTION('ref_axis',(-1.,0.,0.)) ;
#113727=DIRECTION('center_axis',(0.,1.,0.)) ;
#113728=DIRECTION('ref_axis',(1.,0.,0.)) ;
#113729=DIRECTION('center_axis',(0.,0.,-1.)) ;
#113730=DIRECTION('ref_axis',(1.,0.,0.)) ;
#113731=DIRECTION('center_axis',(0.,0.,-1.)) ;
#113732=DIRECTION('ref_axis',(-1.,0.,0.)) ;
#113733=DIRECTION('center_axis',(0.,0.,1.)) ;
#113734=DIRECTION('ref_axis',(1.,0.,0.)) ;
#113735=DIRECTION('center_axis',(-2.16840434497101E-16,1.,-1.020425574104E-16)) ;
#113736=DIRECTION('ref_axis',(-1.,-2.16840434497101E-16,5.47382212626882E-48)) ;
#113737=DIRECTION('center_axis',(0.,1.,0.)) ;
#113738=DIRECTION('ref_axis',(0.,0.,-1.)) ;
#113739=DIRECTION('center_axis',(1.,0.,1.25542992828747E-32)) ;
#113740=DIRECTION('ref_axis',(1.25542992828747E-32,0.,-1.)) ;
#113741=DIRECTION('center_axis',(1.,0.,0.)) ;
#113742=DIRECTION('ref_axis',(0.,0.,-1.)) ;
#113743=DIRECTION('center_axis',(-1.,-1.2303003375722E-16,0.)) ;
#113744=DIRECTION('ref_axis',(0.,-1.,0.)) ;
#113745=DIRECTION('center_axis',(0.,0.,-1.)) ;
#113746=DIRECTION('ref_axis',(1.,0.,0.)) ;
#113747=DIRECTION('center_axis',(0.,0.,-1.)) ;
#113748=DIRECTION('ref_axis',(-1.,0.,0.)) ;
#113749=DIRECTION('',(0.,0.,1.)) ;
#113750=DIRECTION('center_axis',(0.,0.,1.)) ;
#113751=DIRECTION('ref_axis',(1.,0.,0.)) ;
#113752=DIRECTION('center_axis',(0.,0.,1.)) ;
#113753=DIRECTION('ref_axis',(1.,0.,0.)) ;
#113754=DIRECTION('center_axis',(6.27714964143733E-33,-5.10212787052002E-17,
-1.)) ;
#113755=DIRECTION('ref_axis',(3.20268201330022E-49,1.,-5.10212787052002E-17)) ;
#113756=DIRECTION('center_axis',(1.,1.53063836115601E-16,-1.53236300070382E-33)) ;
#113757=DIRECTION('ref_axis',(-1.53063836115601E-16,1.,2.34549359209339E-49)) ;
#113758=DIRECTION('center_axis',(-1.,0.,0.)) ;
#113759=DIRECTION('ref_axis',(0.,0.,1.)) ;
#113760=DIRECTION('center_axis',(1.,0.,0.)) ;
#113761=DIRECTION('ref_axis',(0.,0.,-1.)) ;
#113762=DIRECTION('center_axis',(0.,1.,0.)) ;
#113763=DIRECTION('ref_axis',(1.,0.,0.)) ;
#113764=DIRECTION('center_axis',(-4.33680868994202E-15,1.,0.)) ;
#113765=DIRECTION('ref_axis',(1.,4.33680868994202E-15,0.)) ;
#113766=DIRECTION('center_axis',(0.,-1.,0.)) ;
#113767=DIRECTION('ref_axis',(0.,0.,-1.)) ;
#113768=DIRECTION('center_axis',(0.,0.,-1.)) ;
#113769=DIRECTION('ref_axis',(1.,0.,0.)) ;
#113770=DIRECTION('center_axis',(0.,0.,1.)) ;
#113771=DIRECTION('ref_axis',(1.,0.,0.)) ;
#113772=DIRECTION('center_axis',(0.,0.,-1.)) ;
#113773=DIRECTION('ref_axis',(-1.,0.,0.)) ;
#113774=DIRECTION('center_axis',(0.,1.,0.)) ;
#113775=DIRECTION('ref_axis',(1.,0.,0.)) ;
#113776=DIRECTION('center_axis',(1.,1.2303003375722E-16,0.)) ;
#113777=DIRECTION('ref_axis',(1.2303003375722E-16,-1.,0.)) ;
#113778=DIRECTION('center_axis',(0.,1.,0.)) ;
#113779=DIRECTION('ref_axis',(-6.50521303491301E-15,0.,-1.)) ;
#113780=DIRECTION('center_axis',(6.27714964143733E-33,-5.10212787052002E-17,
-1.)) ;
#113781=DIRECTION('ref_axis',(0.,1.,0.)) ;
#113782=DIRECTION('center_axis',(0.,-1.,0.)) ;
#113783=DIRECTION('ref_axis',(0.,0.,1.)) ;
#113784=DIRECTION('center_axis',(2.16840434497101E-16,-1.,5.10212787052002E-17)) ;
#113785=DIRECTION('ref_axis',(1.,2.16840434497101E-16,-5.47382212626882E-48)) ;
#113786=DIRECTION('center_axis',(0.,1.,0.)) ;
#113787=DIRECTION('ref_axis',(0.,0.,-1.)) ;
#113788=DIRECTION('center_axis',(0.,0.,1.)) ;
#113789=DIRECTION('ref_axis',(1.,0.,0.)) ;
#113790=DIRECTION('center_axis',(0.,0.,-1.)) ;
#113791=DIRECTION('ref_axis',(-1.,0.,0.)) ;
#113792=DIRECTION('center_axis',(-1.,-1.2303003375722E-16,0.)) ;
#113793=DIRECTION('ref_axis',(0.,-1.,0.)) ;
#113794=DIRECTION('center_axis',(0.,-1.,0.)) ;
#113795=DIRECTION('ref_axis',(0.,0.,1.)) ;
#113796=DIRECTION('center_axis',(1.53063836115601E-16,-1.,5.10212787052002E-17)) ;
#113797=DIRECTION('ref_axis',(1.,1.53063836115601E-16,-6.84227765783602E-48)) ;
#113798=DIRECTION('',(-1.53063836115601E-16,1.,-5.10212787052002E-17)) ;
#113799=DIRECTION('center_axis',(0.,-1.,0.)) ;
#113800=DIRECTION('ref_axis',(0.,0.,-1.)) ;
#113801=DIRECTION('center_axis',(-1.,0.,0.)) ;
#113802=DIRECTION('ref_axis',(0.,0.,-1.)) ;
#113803=DIRECTION('center_axis',(-1.2303003375722E-16,1.,-5.10212787052002E-17)) ;
#113804=DIRECTION('ref_axis',(-1.,-1.2303003375722E-16,6.27714964143733E-33)) ;
#113805=DIRECTION('center_axis',(-8.67361737988403E-15,-1.,0.)) ;
#113806=DIRECTION('ref_axis',(1.,-8.67361737988403E-15,0.)) ;
#113807=DIRECTION('center_axis',(1.,0.,6.27714964143733E-33)) ;
#113808=DIRECTION('ref_axis',(6.27714964143733E-33,0.,-1.)) ;
#113809=DIRECTION('center_axis',(-1.,0.,-6.50521303491318E-15)) ;
#113810=DIRECTION('ref_axis',(-6.50521303491318E-15,0.,1.)) ;
#113811=DIRECTION('center_axis',(1.,0.,0.)) ;
#113812=DIRECTION('ref_axis',(0.,1.,0.)) ;
#113813=DIRECTION('center_axis',(0.,0.,-1.)) ;
#113814=DIRECTION('ref_axis',(-1.,0.,0.)) ;
#113815=DIRECTION('center_axis',(0.,0.,1.)) ;
#113816=DIRECTION('ref_axis',(1.,0.,0.)) ;
#113817=DIRECTION('center_axis',(0.,0.,-1.)) ;
#113818=DIRECTION('ref_axis',(-1.,0.,0.)) ;
#113819=DIRECTION('center_axis',(-1.,0.,0.)) ;
#113820=DIRECTION('ref_axis',(0.,0.,1.)) ;
#113821=DIRECTION('center_axis',(0.,-1.,0.)) ;
#113822=DIRECTION('ref_axis',(0.,0.,-1.)) ;
#113823=DIRECTION('center_axis',(0.,1.,0.)) ;
#113824=DIRECTION('ref_axis',(0.,0.,1.)) ;
#113825=DIRECTION('center_axis',(0.,1.,-6.50521303491301E-15)) ;
#113826=DIRECTION('ref_axis',(0.,6.50521303491301E-15,1.)) ;
#113827=DIRECTION('center_axis',(0.,-1.,0.)) ;
#113828=DIRECTION('ref_axis',(0.,0.,-1.)) ;
#113829=DIRECTION('center_axis',(0.,-1.,0.)) ;
#113830=DIRECTION('ref_axis',(0.,0.,-1.)) ;
#113831=DIRECTION('center_axis',(0.,-1.,-1.07081696047951E-16)) ;
#113832=DIRECTION('ref_axis',(0.,1.07081696047951E-16,-1.)) ;
#113833=DIRECTION('center_axis',(0.,1.,0.)) ;
#113834=DIRECTION('ref_axis',(0.,0.,1.)) ;
#113835=DIRECTION('center_axis',(-1.,0.,0.)) ;
#113836=DIRECTION('ref_axis',(0.,0.,1.)) ;
#113837=DIRECTION('center_axis',(0.,0.,1.)) ;
#113838=DIRECTION('ref_axis',(1.,0.,0.)) ;
#113839=DIRECTION('center_axis',(0.,1.,0.)) ;
#113840=DIRECTION('ref_axis',(0.,0.,1.)) ;
#113841=DIRECTION('center_axis',(0.,0.,-1.)) ;
#113842=DIRECTION('ref_axis',(-1.,0.,0.)) ;
#113843=DIRECTION('center_axis',(0.,0.,1.)) ;
#113844=DIRECTION('ref_axis',(1.,0.,0.)) ;
#113845=DIRECTION('center_axis',(0.,0.,1.)) ;
#113846=DIRECTION('ref_axis',(1.,0.,0.)) ;
#113847=DIRECTION('center_axis',(0.,0.,1.)) ;
#113848=DIRECTION('ref_axis',(1.,0.,0.)) ;
#113849=DIRECTION('center_axis',(0.,0.,-1.)) ;
#113850=DIRECTION('ref_axis',(-1.,0.,0.)) ;
#113851=DIRECTION('center_axis',(0.,1.,0.)) ;
#113852=DIRECTION('ref_axis',(0.,0.,1.)) ;
#113853=DIRECTION('center_axis',(0.,-0.707106781186545,0.70710678118655)) ;
#113854=DIRECTION('ref_axis',(0.,-0.70710678118655,-0.707106781186545)) ;
#113855=DIRECTION('center_axis',(0.,1.,0.)) ;
#113856=DIRECTION('ref_axis',(0.,0.,1.)) ;
#113857=DIRECTION('center_axis',(0.,-0.514231796959101,-0.857651245551602)) ;
#113858=DIRECTION('ref_axis',(0.,0.857651245551602,-0.514231796959101)) ;
#113859=DIRECTION('center_axis',(0.,-0.707106781186548,0.707106781186547)) ;
#113860=DIRECTION('ref_axis',(0.,-0.707106781186547,-0.707106781186548)) ;
#113861=DIRECTION('center_axis',(0.,-0.707106781186552,0.707106781186543)) ;
#113862=DIRECTION('ref_axis',(0.,-0.707106781186543,-0.707106781186552)) ;
#113863=DIRECTION('center_axis',(-1.,0.,0.)) ;
#113864=DIRECTION('ref_axis',(0.,0.,1.)) ;
#113865=DIRECTION('center_axis',(0.,0.514231796959101,-0.857651245551602)) ;
#113866=DIRECTION('ref_axis',(0.,0.857651245551602,0.514231796959101)) ;
#113867=DIRECTION('center_axis',(0.,1.,0.)) ;
#113868=DIRECTION('ref_axis',(0.,0.,1.)) ;
#113869=DIRECTION('center_axis',(0.,0.,-1.)) ;
#113870=DIRECTION('ref_axis',(-1.,0.,0.)) ;
#113871=DIRECTION('center_axis',(0.,1.,0.)) ;
#113872=DIRECTION('ref_axis',(0.,0.,1.)) ;
#113873=DIRECTION('center_axis',(0.,0.,-1.)) ;
#113874=DIRECTION('ref_axis',(-1.,0.,0.)) ;
#113875=DIRECTION('center_axis',(0.,0.,-1.)) ;
#113876=DIRECTION('ref_axis',(-1.,0.,0.)) ;
#113877=DIRECTION('center_axis',(0.,0.,1.)) ;
#113878=DIRECTION('ref_axis',(1.,0.,0.)) ;
#113879=DIRECTION('center_axis',(0.,0.,-1.)) ;
#113880=DIRECTION('ref_axis',(-1.,0.,0.)) ;
#113881=DIRECTION('center_axis',(0.,1.,0.)) ;
#113882=DIRECTION('ref_axis',(0.,0.,1.)) ;
#113883=DIRECTION('center_axis',(0.,-1.,8.67361737988405E-15)) ;
#113884=DIRECTION('ref_axis',(0.,-8.67361737988405E-15,-1.)) ;
#113885=DIRECTION('center_axis',(0.,0.707106781186546,0.707106781186549)) ;
#113886=DIRECTION('ref_axis',(0.,-0.707106781186549,0.707106781186546)) ;
#113887=DIRECTION('center_axis',(0.,0.707106781186545,0.70710678118655)) ;
#113888=DIRECTION('ref_axis',(0.,-0.70710678118655,0.707106781186545)) ;
#113889=DIRECTION('center_axis',(0.,1.,1.07081696047951E-16)) ;
#113890=DIRECTION('ref_axis',(0.,-1.07081696047951E-16,1.)) ;
#113891=DIRECTION('center_axis',(0.,-1.,0.)) ;
#113892=DIRECTION('ref_axis',(0.,0.,-1.)) ;
#113893=DIRECTION('center_axis',(0.,1.,0.)) ;
#113894=DIRECTION('ref_axis',(0.,0.,1.)) ;
#113895=DIRECTION('center_axis',(0.,0.,1.)) ;
#113896=DIRECTION('ref_axis',(1.,0.,0.)) ;
#113897=DIRECTION('center_axis',(0.,1.,0.)) ;
#113898=DIRECTION('ref_axis',(0.,0.,1.)) ;
#113899=DIRECTION('center_axis',(0.,8.67361737988403E-15,1.)) ;
#113900=DIRECTION('ref_axis',(0.,-1.,8.67361737988403E-15)) ;
#113901=DIRECTION('center_axis',(0.,3.99416362155027E-15,1.)) ;
#113902=DIRECTION('ref_axis',(0.,-1.,3.99416362155027E-15)) ;
#113903=DIRECTION('center_axis',(0.,0.,1.)) ;
#113904=DIRECTION('ref_axis',(1.,0.,0.)) ;
#113905=DIRECTION('center_axis',(0.,0.,-1.)) ;
#113906=DIRECTION('ref_axis',(-1.,0.,0.)) ;
#113907=DIRECTION('center_axis',(0.,0.,1.)) ;
#113908=DIRECTION('ref_axis',(1.,0.,0.)) ;
#113909=DIRECTION('center_axis',(-1.,0.,0.)) ;
#113910=DIRECTION('ref_axis',(0.,0.,1.)) ;
#113911=DIRECTION('center_axis',(0.,1.,0.)) ;
#113912=DIRECTION('ref_axis',(0.,0.,1.)) ;
#113913=DIRECTION('center_axis',(-1.,0.,0.)) ;
#113914=DIRECTION('ref_axis',(0.,0.,1.)) ;
#113915=DIRECTION('center_axis',(0.,-1.,0.)) ;
#113916=DIRECTION('ref_axis',(0.,0.,-1.)) ;
#113917=DIRECTION('center_axis',(0.,1.,0.)) ;
#113918=DIRECTION('ref_axis',(0.,0.,1.)) ;
#113919=DIRECTION('center_axis',(0.,-1.,0.)) ;
#113920=DIRECTION('ref_axis',(0.,0.,-1.)) ;
#113921=DIRECTION('center_axis',(0.,1.,0.)) ;
#113922=DIRECTION('ref_axis',(0.,0.,1.)) ;
#113923=DIRECTION('center_axis',(0.,-1.,0.)) ;
#113924=DIRECTION('ref_axis',(0.,0.,-1.)) ;
#113925=DIRECTION('center_axis',(0.,1.,0.)) ;
#113926=DIRECTION('ref_axis',(0.,0.,-1.)) ;
#113927=DIRECTION('center_axis',(0.,0.,-1.)) ;
#113928=DIRECTION('ref_axis',(-1.,0.,0.)) ;
#113929=DIRECTION('center_axis',(0.,1.,0.)) ;
#113930=DIRECTION('ref_axis',(0.,0.,-1.)) ;
#113931=DIRECTION('center_axis',(0.,0.,-1.)) ;
#113932=DIRECTION('ref_axis',(-1.,0.,0.)) ;
#113933=DIRECTION('center_axis',(0.,0.,1.)) ;
#113934=DIRECTION('ref_axis',(1.,0.,0.)) ;
#113935=DIRECTION('center_axis',(0.,0.,-1.)) ;
#113936=DIRECTION('ref_axis',(-1.,0.,0.)) ;
#113937=DIRECTION('center_axis',(0.,0.,-1.)) ;
#113938=DIRECTION('ref_axis',(-1.,0.,0.)) ;
#113939=DIRECTION('center_axis',(0.,6.93889390390724E-14,-1.)) ;
#113940=DIRECTION('ref_axis',(0.,1.,6.93889390390724E-14)) ;
#113941=DIRECTION('center_axis',(1.,0.,0.)) ;
#113942=DIRECTION('ref_axis',(0.,0.,-1.)) ;
#113943=DIRECTION('center_axis',(3.0665868333667E-15,0.707106781186532,
-0.707106781186563)) ;
#113944=DIRECTION('ref_axis',(-5.39294103027656E-31,0.707106781186563,0.707106781186532)) ;
#113945=DIRECTION('center_axis',(1.,0.,0.)) ;
#113946=DIRECTION('ref_axis',(0.,0.,-1.)) ;
#113947=DIRECTION('center_axis',(0.,-1.,0.)) ;
#113948=DIRECTION('ref_axis',(0.,0.,-1.)) ;
#113949=DIRECTION('center_axis',(0.,-0.707106781186548,0.707106781186547)) ;
#113950=DIRECTION('ref_axis',(0.,-0.707106781186547,-0.707106781186548)) ;
#113951=DIRECTION('center_axis',(0.,-1.,-1.07081696047951E-16)) ;
#113952=DIRECTION('ref_axis',(0.,1.07081696047951E-16,-1.)) ;
#113953=DIRECTION('center_axis',(0.,-1.,-8.67361737988379E-15)) ;
#113954=DIRECTION('ref_axis',(0.,8.67361737988379E-15,-1.)) ;
#113955=DIRECTION('center_axis',(1.,0.,0.)) ;
#113956=DIRECTION('ref_axis',(0.,0.,-1.)) ;
#113957=DIRECTION('center_axis',(0.,0.,1.)) ;
#113958=DIRECTION('ref_axis',(1.,0.,0.)) ;
#113959=DIRECTION('center_axis',(0.,0.,-1.)) ;
#113960=DIRECTION('ref_axis',(-1.,0.,0.)) ;
#113961=DIRECTION('center_axis',(0.,0.,1.)) ;
#113962=DIRECTION('ref_axis',(1.,0.,0.)) ;
#113963=DIRECTION('center_axis',(0.,0.,1.)) ;
#113964=DIRECTION('ref_axis',(1.,0.,0.)) ;
#113965=DIRECTION('center_axis',(0.,0.,1.)) ;
#113966=DIRECTION('ref_axis',(1.,0.,0.)) ;
#113967=DIRECTION('center_axis',(1.,0.,0.)) ;
#113968=DIRECTION('ref_axis',(0.,0.382683432365085,0.923879532511289)) ;
#113969=DIRECTION('center_axis',(-3.0665868333667E-15,-0.707106781186532,
-0.707106781186563)) ;
#113970=DIRECTION('ref_axis',(-5.39294103027656E-31,0.707106781186563,-0.707106781186532)) ;
#113971=DIRECTION('center_axis',(1.,0.,0.)) ;
#113972=DIRECTION('ref_axis',(0.,0.,-1.)) ;
#113973=DIRECTION('center_axis',(0.,0.514231796959126,0.857651245551587)) ;
#113974=DIRECTION('ref_axis',(0.,-0.857651245551587,0.514231796959126)) ;
#113975=DIRECTION('center_axis',(0.,0.707106781186546,0.707106781186549)) ;
#113976=DIRECTION('ref_axis',(0.,-0.707106781186549,0.707106781186546)) ;
#113977=DIRECTION('center_axis',(3.06658683336673E-15,-0.707106781186539,
-0.707106781186556)) ;
#113978=DIRECTION('ref_axis',(1.90456316695698E-29,0.707106781186556,-0.707106781186539)) ;
#113979=DIRECTION('center_axis',(1.,0.,0.)) ;
#113980=DIRECTION('ref_axis',(0.,0.,-1.)) ;
#113981=DIRECTION('center_axis',(0.,-0.514231796959058,0.857651245551628)) ;
#113982=DIRECTION('ref_axis',(0.,-0.857651245551628,-0.514231796959058)) ;
#113983=DIRECTION('center_axis',(1.,0.,0.)) ;
#113984=DIRECTION('ref_axis',(0.,0.,-1.)) ;
#113985=DIRECTION('center_axis',(0.,0.,-1.)) ;
#113986=DIRECTION('ref_axis',(-1.,0.,0.)) ;
#113987=DIRECTION('center_axis',(1.,0.,0.)) ;
#113988=DIRECTION('ref_axis',(0.,0.,-1.)) ;
#113989=DIRECTION('center_axis',(0.,0.,1.)) ;
#113990=DIRECTION('ref_axis',(1.,0.,0.)) ;
#113991=DIRECTION('center_axis',(0.,3.99416362155027E-15,1.)) ;
#113992=DIRECTION('ref_axis',(0.,-1.,3.99416362155027E-15)) ;
#113993=DIRECTION('center_axis',(0.,0.,-1.)) ;
#113994=DIRECTION('ref_axis',(-1.,0.,0.)) ;
#113995=DIRECTION('center_axis',(0.,0.,1.)) ;
#113996=DIRECTION('ref_axis',(1.,0.,0.)) ;
#113997=DIRECTION('center_axis',(0.,-6.93889390390724E-14,1.)) ;
#113998=DIRECTION('ref_axis',(0.,-1.,-6.93889390390724E-14)) ;
#113999=DIRECTION('center_axis',(0.,1.,0.)) ;
#114000=DIRECTION('ref_axis',(0.,0.,-1.)) ;
#114001=DIRECTION('center_axis',(0.,-1.,0.)) ;
#114002=DIRECTION('ref_axis',(0.,0.,-1.)) ;
#114003=DIRECTION('center_axis',(1.,0.,0.)) ;
#114004=DIRECTION('ref_axis',(0.,0.,-1.)) ;
#114005=DIRECTION('center_axis',(0.,1.,0.)) ;
#114006=DIRECTION('ref_axis',(0.,0.,1.)) ;
#114007=DIRECTION('center_axis',(0.,1.,0.)) ;
#114008=DIRECTION('ref_axis',(0.,0.,1.)) ;
#114009=DIRECTION('center_axis',(0.,-1.,0.)) ;
#114010=DIRECTION('ref_axis',(0.,0.,-1.)) ;
#114011=DIRECTION('center_axis',(0.,1.,1.07081696047951E-16)) ;
#114012=DIRECTION('ref_axis',(0.,-1.07081696047951E-16,1.)) ;
#114013=DIRECTION('center_axis',(0.,1.,6.50521303491284E-15)) ;
#114014=DIRECTION('ref_axis',(0.,-6.50521303491284E-15,1.)) ;
#114015=DIRECTION('center_axis',(0.,1.,0.)) ;
#114016=DIRECTION('ref_axis',(0.,0.,-1.)) ;
#114017=DIRECTION('center_axis',(0.,0.,1.)) ;
#114018=DIRECTION('ref_axis',(1.,0.,0.)) ;
#114019=DIRECTION('center_axis',(1.,0.,0.)) ;
#114020=DIRECTION('ref_axis',(0.,0.,-1.)) ;
#114021=DIRECTION('center_axis',(0.,0.,-1.)) ;
#114022=DIRECTION('ref_axis',(-1.,0.,0.)) ;
#114023=DIRECTION('center_axis',(0.,0.,-1.)) ;
#114024=DIRECTION('ref_axis',(-1.,0.,0.)) ;
#114025=DIRECTION('center_axis',(0.,-1.,0.)) ;
#114026=DIRECTION('ref_axis',(0.,0.,-1.)) ;
#114027=DIRECTION('center_axis',(0.,1.,0.)) ;
#114028=DIRECTION('ref_axis',(0.,0.,1.)) ;
#114029=DIRECTION('center_axis',(0.,-1.,0.)) ;
#114030=DIRECTION('ref_axis',(0.,0.,-1.)) ;
#114031=DIRECTION('center_axis',(0.,1.,0.)) ;
#114032=DIRECTION('ref_axis',(0.,0.,-1.)) ;
#114033=DIRECTION('center_axis',(0.,0.,-1.)) ;
#114034=DIRECTION('ref_axis',(-1.,0.,0.)) ;
#114035=DIRECTION('center_axis',(0.,1.,0.)) ;
#114036=DIRECTION('ref_axis',(0.,0.,-1.)) ;
#114037=DIRECTION('center_axis',(0.,0.,-1.)) ;
#114038=DIRECTION('ref_axis',(-1.,0.,0.)) ;
#114039=DIRECTION('center_axis',(0.,0.,1.)) ;
#114040=DIRECTION('ref_axis',(1.,0.,0.)) ;
#114041=DIRECTION('center_axis',(0.,0.,-1.)) ;
#114042=DIRECTION('ref_axis',(-1.,0.,0.)) ;
#114043=DIRECTION('center_axis',(0.,0.,-1.)) ;
#114044=DIRECTION('ref_axis',(-1.,0.,0.)) ;
#114045=DIRECTION('center_axis',(0.,0.,-1.)) ;
#114046=DIRECTION('ref_axis',(-1.,0.,0.)) ;
#114047=DIRECTION('center_axis',(1.,0.,0.)) ;
#114048=DIRECTION('ref_axis',(0.,0.,-1.)) ;
#114049=DIRECTION('center_axis',(3.0665868333667E-15,0.707106781186532,
-0.707106781186563)) ;
#114050=DIRECTION('ref_axis',(-5.39294103027656E-31,0.707106781186563,0.707106781186532)) ;
#114051=DIRECTION('center_axis',(1.,0.,0.)) ;
#114052=DIRECTION('ref_axis',(0.,0.,-1.)) ;
#114053=DIRECTION('center_axis',(0.,-1.,0.)) ;
#114054=DIRECTION('ref_axis',(0.,0.,-1.)) ;
#114055=DIRECTION('center_axis',(0.,-0.707106781186548,0.707106781186547)) ;
#114056=DIRECTION('ref_axis',(0.,-0.707106781186547,-0.707106781186548)) ;
#114057=DIRECTION('center_axis',(0.,-1.,-1.07081696047951E-16)) ;
#114058=DIRECTION('ref_axis',(0.,1.07081696047951E-16,-1.)) ;
#114059=DIRECTION('center_axis',(0.,-1.,-8.67361737988379E-15)) ;
#114060=DIRECTION('ref_axis',(0.,8.67361737988379E-15,-1.)) ;
#114061=DIRECTION('center_axis',(1.,0.,0.)) ;
#114062=DIRECTION('ref_axis',(0.,0.,-1.)) ;
#114063=DIRECTION('center_axis',(0.,0.,1.)) ;
#114064=DIRECTION('ref_axis',(1.,0.,0.)) ;
#114065=DIRECTION('center_axis',(0.,0.,-1.)) ;
#114066=DIRECTION('ref_axis',(-1.,0.,0.)) ;
#114067=DIRECTION('center_axis',(0.,0.,1.)) ;
#114068=DIRECTION('ref_axis',(1.,0.,0.)) ;
#114069=DIRECTION('center_axis',(0.,0.,1.)) ;
#114070=DIRECTION('ref_axis',(1.,0.,0.)) ;
#114071=DIRECTION('center_axis',(0.,0.,1.)) ;
#114072=DIRECTION('ref_axis',(1.,0.,0.)) ;
#114073=DIRECTION('center_axis',(1.,0.,0.)) ;
#114074=DIRECTION('ref_axis',(0.,0.382683432365093,0.923879532511286)) ;
#114075=DIRECTION('center_axis',(6.13317366673366E-15,-0.707106781186563,
-0.707106781186532)) ;
#114076=DIRECTION('ref_axis',(-1.7381816909424E-29,0.707106781186532,-0.707106781186563)) ;
#114077=DIRECTION('center_axis',(1.,0.,0.)) ;
#114078=DIRECTION('ref_axis',(0.,0.,-1.)) ;
#114079=DIRECTION('center_axis',(0.,0.514231796959126,0.857651245551587)) ;
#114080=DIRECTION('ref_axis',(0.,-0.857651245551587,0.514231796959126)) ;
#114081=DIRECTION('center_axis',(0.,0.707106781186546,0.707106781186549)) ;
#114082=DIRECTION('ref_axis',(0.,-0.707106781186549,0.707106781186546)) ;
#114083=DIRECTION('center_axis',(3.06658683336673E-15,-0.707106781186539,
-0.707106781186556)) ;
#114084=DIRECTION('ref_axis',(1.90456316695698E-29,0.707106781186556,-0.707106781186539)) ;
#114085=DIRECTION('center_axis',(1.,0.,0.)) ;
#114086=DIRECTION('ref_axis',(0.,0.,-1.)) ;
#114087=DIRECTION('center_axis',(0.,-0.514231796959091,0.857651245551608)) ;
#114088=DIRECTION('ref_axis',(0.,-0.857651245551608,-0.514231796959091)) ;
#114089=DIRECTION('center_axis',(1.,0.,0.)) ;
#114090=DIRECTION('ref_axis',(0.,0.,-1.)) ;
#114091=DIRECTION('center_axis',(0.,0.,-1.)) ;
#114092=DIRECTION('ref_axis',(-1.,0.,0.)) ;
#114093=DIRECTION('center_axis',(1.,0.,0.)) ;
#114094=DIRECTION('ref_axis',(0.,0.,-1.)) ;
#114095=DIRECTION('center_axis',(0.,0.,1.)) ;
#114096=DIRECTION('ref_axis',(1.,0.,0.)) ;
#114097=DIRECTION('center_axis',(0.,3.99416362155027E-15,1.)) ;
#114098=DIRECTION('ref_axis',(0.,-1.,3.99416362155027E-15)) ;
#114099=DIRECTION('center_axis',(0.,0.,-1.)) ;
#114100=DIRECTION('ref_axis',(-1.,0.,0.)) ;
#114101=DIRECTION('center_axis',(0.,0.,1.)) ;
#114102=DIRECTION('ref_axis',(1.,0.,0.)) ;
#114103=DIRECTION('center_axis',(0.,0.,1.)) ;
#114104=DIRECTION('ref_axis',(1.,0.,0.)) ;
#114105=DIRECTION('center_axis',(0.,1.,0.)) ;
#114106=DIRECTION('ref_axis',(0.,0.,-1.)) ;
#114107=DIRECTION('center_axis',(0.,-1.,0.)) ;
#114108=DIRECTION('ref_axis',(0.,0.,-1.)) ;
#114109=DIRECTION('center_axis',(1.,0.,0.)) ;
#114110=DIRECTION('ref_axis',(0.,0.,-1.)) ;
#114111=DIRECTION('center_axis',(0.,1.,0.)) ;
#114112=DIRECTION('ref_axis',(0.,0.,1.)) ;
#114113=DIRECTION('center_axis',(0.,1.,0.)) ;
#114114=DIRECTION('ref_axis',(0.,0.,1.)) ;
#114115=DIRECTION('center_axis',(0.,-1.,0.)) ;
#114116=DIRECTION('ref_axis',(0.,0.,-1.)) ;
#114117=DIRECTION('center_axis',(0.,1.,1.07081696047951E-16)) ;
#114118=DIRECTION('ref_axis',(0.,-1.07081696047951E-16,1.)) ;
#114119=DIRECTION('center_axis',(0.,1.,6.50521303491307E-15)) ;
#114120=DIRECTION('ref_axis',(0.,-6.50521303491307E-15,1.)) ;
#114121=DIRECTION('center_axis',(0.,1.,0.)) ;
#114122=DIRECTION('ref_axis',(0.,0.,-1.)) ;
#114123=DIRECTION('center_axis',(0.,0.,1.)) ;
#114124=DIRECTION('ref_axis',(1.,0.,0.)) ;
#114125=DIRECTION('center_axis',(1.,0.,0.)) ;
#114126=DIRECTION('ref_axis',(0.,0.,-1.)) ;
#114127=DIRECTION('center_axis',(0.,0.,-1.)) ;
#114128=DIRECTION('ref_axis',(-1.,0.,0.)) ;
#114129=DIRECTION('center_axis',(0.,0.,-1.)) ;
#114130=DIRECTION('ref_axis',(-1.,0.,0.)) ;
#114131=DIRECTION('center_axis',(0.,-1.,0.)) ;
#114132=DIRECTION('ref_axis',(0.,0.,-1.)) ;
#114133=DIRECTION('center_axis',(0.,1.,0.)) ;
#114134=DIRECTION('ref_axis',(0.,0.,1.)) ;
#114135=DIRECTION('center_axis',(0.,-1.,0.)) ;
#114136=DIRECTION('ref_axis',(0.,0.,-1.)) ;
#114137=DIRECTION('center_axis',(0.,1.,0.)) ;
#114138=DIRECTION('ref_axis',(0.,0.,-1.)) ;
#114139=DIRECTION('center_axis',(0.,0.,-1.)) ;
#114140=DIRECTION('ref_axis',(-1.,0.,0.)) ;
#114141=DIRECTION('center_axis',(0.,1.,0.)) ;
#114142=DIRECTION('ref_axis',(0.,0.,-1.)) ;
#114143=DIRECTION('center_axis',(0.,0.,-1.)) ;
#114144=DIRECTION('ref_axis',(-1.,0.,0.)) ;
#114145=DIRECTION('center_axis',(0.,0.,1.)) ;
#114146=DIRECTION('ref_axis',(1.,0.,0.)) ;
#114147=DIRECTION('center_axis',(0.,0.,-1.)) ;
#114148=DIRECTION('ref_axis',(-1.,0.,0.)) ;
#114149=DIRECTION('center_axis',(0.,0.,-1.)) ;
#114150=DIRECTION('ref_axis',(-1.,0.,0.)) ;
#114151=DIRECTION('center_axis',(0.,0.,-1.)) ;
#114152=DIRECTION('ref_axis',(-1.,0.,0.)) ;
#114153=DIRECTION('center_axis',(1.,0.,0.)) ;
#114154=DIRECTION('ref_axis',(0.,0.,-1.)) ;
#114155=DIRECTION('center_axis',(-6.13317366673366E-15,0.707106781186563,
-0.707106781186532)) ;
#114156=DIRECTION('ref_axis',(-1.7381816909424E-29,0.707106781186532,0.707106781186563)) ;
#114157=DIRECTION('center_axis',(1.,0.,0.)) ;
#114158=DIRECTION('ref_axis',(0.,0.,-1.)) ;
#114159=DIRECTION('center_axis',(0.,-1.,0.)) ;
#114160=DIRECTION('ref_axis',(0.,0.,-1.)) ;
#114161=DIRECTION('center_axis',(0.,-0.707106781186548,0.707106781186547)) ;
#114162=DIRECTION('ref_axis',(0.,-0.707106781186547,-0.707106781186548)) ;
#114163=DIRECTION('center_axis',(0.,-1.,-1.07081696047951E-16)) ;
#114164=DIRECTION('ref_axis',(0.,1.07081696047951E-16,-1.)) ;
#114165=DIRECTION('center_axis',(0.,-1.,-8.67361737988409E-15)) ;
#114166=DIRECTION('ref_axis',(0.,8.67361737988409E-15,-1.)) ;
#114167=DIRECTION('center_axis',(1.,0.,0.)) ;
#114168=DIRECTION('ref_axis',(0.,0.,-1.)) ;
#114169=DIRECTION('center_axis',(0.,0.,1.)) ;
#114170=DIRECTION('ref_axis',(1.,0.,0.)) ;
#114171=DIRECTION('center_axis',(0.,0.,-1.)) ;
#114172=DIRECTION('ref_axis',(-1.,0.,0.)) ;
#114173=DIRECTION('center_axis',(0.,0.,1.)) ;
#114174=DIRECTION('ref_axis',(1.,0.,0.)) ;
#114175=DIRECTION('center_axis',(0.,0.,1.)) ;
#114176=DIRECTION('ref_axis',(1.,0.,0.)) ;
#114177=DIRECTION('center_axis',(0.,0.,1.)) ;
#114178=DIRECTION('ref_axis',(1.,0.,0.)) ;
#114179=DIRECTION('center_axis',(1.,0.,0.)) ;
#114180=DIRECTION('ref_axis',(0.,0.382683432365093,0.923879532511286)) ;
#114181=DIRECTION('center_axis',(6.13317366673366E-15,-0.707106781186563,
-0.707106781186532)) ;
#114182=DIRECTION('ref_axis',(-1.7381816909424E-29,0.707106781186532,-0.707106781186563)) ;
#114183=DIRECTION('center_axis',(1.,0.,0.)) ;
#114184=DIRECTION('ref_axis',(0.,0.,-1.)) ;
#114185=DIRECTION('center_axis',(0.,0.514231796959093,0.857651245551607)) ;
#114186=DIRECTION('ref_axis',(0.,-0.857651245551607,0.514231796959093)) ;
#114187=DIRECTION('center_axis',(0.,0.707106781186546,0.707106781186549)) ;
#114188=DIRECTION('ref_axis',(0.,-0.707106781186549,0.707106781186546)) ;
#114189=DIRECTION('center_axis',(3.06658683336673E-15,-0.707106781186539,
-0.707106781186556)) ;
#114190=DIRECTION('ref_axis',(1.90456316695698E-29,0.707106781186556,-0.707106781186539)) ;
#114191=DIRECTION('center_axis',(1.,0.,0.)) ;
#114192=DIRECTION('ref_axis',(0.,0.,-1.)) ;
#114193=DIRECTION('center_axis',(0.,-0.514231796959091,0.857651245551608)) ;
#114194=DIRECTION('ref_axis',(0.,-0.857651245551608,-0.514231796959091)) ;
#114195=DIRECTION('center_axis',(1.,0.,0.)) ;
#114196=DIRECTION('ref_axis',(0.,0.,-1.)) ;
#114197=DIRECTION('center_axis',(0.,0.,-1.)) ;
#114198=DIRECTION('ref_axis',(-1.,0.,0.)) ;
#114199=DIRECTION('center_axis',(1.,0.,0.)) ;
#114200=DIRECTION('ref_axis',(0.,0.,-1.)) ;
#114201=DIRECTION('center_axis',(0.,0.,1.)) ;
#114202=DIRECTION('ref_axis',(1.,0.,0.)) ;
#114203=DIRECTION('center_axis',(0.,3.99416362155027E-15,1.)) ;
#114204=DIRECTION('ref_axis',(0.,-1.,3.99416362155027E-15)) ;
#114205=DIRECTION('center_axis',(0.,0.,-1.)) ;
#114206=DIRECTION('ref_axis',(-1.,0.,0.)) ;
#114207=DIRECTION('center_axis',(0.,0.,1.)) ;
#114208=DIRECTION('ref_axis',(1.,0.,0.)) ;
#114209=DIRECTION('center_axis',(0.,0.,1.)) ;
#114210=DIRECTION('ref_axis',(1.,0.,0.)) ;
#114211=DIRECTION('center_axis',(0.,1.,0.)) ;
#114212=DIRECTION('ref_axis',(0.,0.,-1.)) ;
#114213=DIRECTION('center_axis',(0.,-1.,0.)) ;
#114214=DIRECTION('ref_axis',(0.,0.,-1.)) ;
#114215=DIRECTION('center_axis',(1.,0.,0.)) ;
#114216=DIRECTION('ref_axis',(0.,0.,-1.)) ;
#114217=DIRECTION('center_axis',(0.,1.,0.)) ;
#114218=DIRECTION('ref_axis',(0.,0.,1.)) ;
#114219=DIRECTION('center_axis',(0.,1.,0.)) ;
#114220=DIRECTION('ref_axis',(0.,0.,1.)) ;
#114221=DIRECTION('center_axis',(0.,-1.,0.)) ;
#114222=DIRECTION('ref_axis',(0.,0.,-1.)) ;
#114223=DIRECTION('center_axis',(0.,1.,1.07081696047951E-16)) ;
#114224=DIRECTION('ref_axis',(0.,-1.07081696047951E-16,1.)) ;
#114225=DIRECTION('center_axis',(0.,1.,6.50521303491307E-15)) ;
#114226=DIRECTION('ref_axis',(0.,-6.50521303491307E-15,1.)) ;
#114227=DIRECTION('center_axis',(0.,1.,0.)) ;
#114228=DIRECTION('ref_axis',(0.,0.,-1.)) ;
#114229=DIRECTION('center_axis',(0.,0.,1.)) ;
#114230=DIRECTION('ref_axis',(1.,0.,0.)) ;
#114231=DIRECTION('center_axis',(1.,0.,0.)) ;
#114232=DIRECTION('ref_axis',(0.,0.,-1.)) ;
#114233=DIRECTION('center_axis',(0.,0.,-1.)) ;
#114234=DIRECTION('ref_axis',(-1.,0.,0.)) ;
#114235=DIRECTION('center_axis',(0.,0.,-1.)) ;
#114236=DIRECTION('ref_axis',(-1.,0.,0.)) ;
#114237=DIRECTION('center_axis',(0.,-1.,0.)) ;
#114238=DIRECTION('ref_axis',(0.,0.,-1.)) ;
#114239=DIRECTION('center_axis',(0.,1.,0.)) ;
#114240=DIRECTION('ref_axis',(0.,0.,1.)) ;
#114241=DIRECTION('center_axis',(0.,-1.,0.)) ;
#114242=DIRECTION('ref_axis',(0.,0.,-1.)) ;
#114243=DIRECTION('center_axis',(0.,1.,0.)) ;
#114244=DIRECTION('ref_axis',(0.,0.,-1.)) ;
#114245=DIRECTION('center_axis',(0.,0.,-1.)) ;
#114246=DIRECTION('ref_axis',(-1.,0.,0.)) ;
#114247=DIRECTION('center_axis',(0.,1.,0.)) ;
#114248=DIRECTION('ref_axis',(0.,0.,-1.)) ;
#114249=DIRECTION('center_axis',(0.,0.,-1.)) ;
#114250=DIRECTION('ref_axis',(-1.,0.,0.)) ;
#114251=DIRECTION('center_axis',(0.,0.,1.)) ;
#114252=DIRECTION('ref_axis',(1.,0.,0.)) ;
#114253=DIRECTION('center_axis',(0.,0.,-1.)) ;
#114254=DIRECTION('ref_axis',(-1.,0.,0.)) ;
#114255=DIRECTION('center_axis',(0.,0.,-1.)) ;
#114256=DIRECTION('ref_axis',(-1.,0.,0.)) ;
#114257=DIRECTION('center_axis',(0.,0.,-1.)) ;
#114258=DIRECTION('ref_axis',(-1.,0.,0.)) ;
#114259=DIRECTION('center_axis',(1.,0.,0.)) ;
#114260=DIRECTION('ref_axis',(0.,0.,-1.)) ;
#114261=DIRECTION('center_axis',(-6.13317366673366E-15,0.707106781186563,
-0.707106781186532)) ;
#114262=DIRECTION('ref_axis',(-1.7381816909424E-29,0.707106781186532,0.707106781186563)) ;
#114263=DIRECTION('center_axis',(1.,0.,0.)) ;
#114264=DIRECTION('ref_axis',(0.,0.,-1.)) ;
#114265=DIRECTION('center_axis',(0.,-1.,0.)) ;
#114266=DIRECTION('ref_axis',(0.,0.,-1.)) ;
#114267=DIRECTION('center_axis',(0.,-0.707106781186548,0.707106781186547)) ;
#114268=DIRECTION('ref_axis',(0.,-0.707106781186547,-0.707106781186548)) ;
#114269=DIRECTION('center_axis',(0.,-1.,-1.07081696047951E-16)) ;
#114270=DIRECTION('ref_axis',(0.,1.07081696047951E-16,-1.)) ;
#114271=DIRECTION('center_axis',(0.,-1.,-8.67361737988409E-15)) ;
#114272=DIRECTION('ref_axis',(0.,8.67361737988409E-15,-1.)) ;
#114273=DIRECTION('center_axis',(1.,0.,0.)) ;
#114274=DIRECTION('ref_axis',(0.,0.,-1.)) ;
#114275=DIRECTION('center_axis',(0.,0.,1.)) ;
#114276=DIRECTION('ref_axis',(1.,0.,0.)) ;
#114277=DIRECTION('center_axis',(0.,0.,-1.)) ;
#114278=DIRECTION('ref_axis',(-1.,0.,0.)) ;
#114279=DIRECTION('center_axis',(0.,0.,1.)) ;
#114280=DIRECTION('ref_axis',(1.,0.,0.)) ;
#114281=DIRECTION('center_axis',(0.,0.,1.)) ;
#114282=DIRECTION('ref_axis',(1.,0.,0.)) ;
#114283=DIRECTION('center_axis',(0.,0.,1.)) ;
#114284=DIRECTION('ref_axis',(1.,0.,0.)) ;
#114285=DIRECTION('center_axis',(1.,0.,0.)) ;
#114286=DIRECTION('ref_axis',(0.,0.382683432365092,0.923879532511286)) ;
#114287=DIRECTION('center_axis',(6.13317366673366E-15,-0.707106781186563,
-0.707106781186532)) ;
#114288=DIRECTION('ref_axis',(-1.7381816909424E-29,0.707106781186532,-0.707106781186563)) ;
#114289=DIRECTION('center_axis',(1.,0.,0.)) ;
#114290=DIRECTION('ref_axis',(0.,0.,-1.)) ;
#114291=DIRECTION('center_axis',(0.,0.514231796959093,0.857651245551607)) ;
#114292=DIRECTION('ref_axis',(0.,-0.857651245551607,0.514231796959093)) ;
#114293=DIRECTION('center_axis',(0.,0.707106781186546,0.707106781186549)) ;
#114294=DIRECTION('ref_axis',(0.,-0.707106781186549,0.707106781186546)) ;
#114295=DIRECTION('center_axis',(3.06658683336673E-15,-0.707106781186539,
-0.707106781186556)) ;
#114296=DIRECTION('ref_axis',(1.90456316695698E-29,0.707106781186556,-0.707106781186539)) ;
#114297=DIRECTION('center_axis',(1.,0.,0.)) ;
#114298=DIRECTION('ref_axis',(0.,0.,-1.)) ;
#114299=DIRECTION('center_axis',(0.,-0.514231796959091,0.857651245551608)) ;
#114300=DIRECTION('ref_axis',(0.,-0.857651245551608,-0.514231796959091)) ;
#114301=DIRECTION('center_axis',(1.,0.,0.)) ;
#114302=DIRECTION('ref_axis',(0.,0.,-1.)) ;
#114303=DIRECTION('center_axis',(0.,0.,-1.)) ;
#114304=DIRECTION('ref_axis',(-1.,0.,0.)) ;
#114305=DIRECTION('center_axis',(1.,0.,0.)) ;
#114306=DIRECTION('ref_axis',(0.,0.,-1.)) ;
#114307=DIRECTION('center_axis',(0.,0.,1.)) ;
#114308=DIRECTION('ref_axis',(1.,0.,0.)) ;
#114309=DIRECTION('center_axis',(0.,3.99416362155027E-15,1.)) ;
#114310=DIRECTION('ref_axis',(0.,-1.,3.99416362155027E-15)) ;
#114311=DIRECTION('center_axis',(0.,0.,-1.)) ;
#114312=DIRECTION('ref_axis',(-1.,0.,0.)) ;
#114313=DIRECTION('center_axis',(0.,0.,1.)) ;
#114314=DIRECTION('ref_axis',(1.,0.,0.)) ;
#114315=DIRECTION('center_axis',(0.,0.,1.)) ;
#114316=DIRECTION('ref_axis',(1.,0.,0.)) ;
#114317=DIRECTION('center_axis',(0.,1.,0.)) ;
#114318=DIRECTION('ref_axis',(0.,0.,-1.)) ;
#114319=DIRECTION('center_axis',(0.,-1.,0.)) ;
#114320=DIRECTION('ref_axis',(0.,0.,-1.)) ;
#114321=DIRECTION('center_axis',(1.,0.,0.)) ;
#114322=DIRECTION('ref_axis',(0.,0.,-1.)) ;
#114323=DIRECTION('center_axis',(0.,1.,0.)) ;
#114324=DIRECTION('ref_axis',(0.,0.,1.)) ;
#114325=DIRECTION('center_axis',(0.,1.,0.)) ;
#114326=DIRECTION('ref_axis',(0.,0.,1.)) ;
#114327=DIRECTION('center_axis',(0.,-1.,0.)) ;
#114328=DIRECTION('ref_axis',(0.,0.,-1.)) ;
#114329=DIRECTION('center_axis',(0.,1.,1.07081696047951E-16)) ;
#114330=DIRECTION('ref_axis',(0.,-1.07081696047951E-16,1.)) ;
#114331=DIRECTION('center_axis',(0.,1.,6.50521303491307E-15)) ;
#114332=DIRECTION('ref_axis',(0.,-6.50521303491307E-15,1.)) ;
#114333=DIRECTION('center_axis',(0.,1.,0.)) ;
#114334=DIRECTION('ref_axis',(0.,0.,-1.)) ;
#114335=DIRECTION('center_axis',(0.,0.,1.)) ;
#114336=DIRECTION('ref_axis',(1.,0.,0.)) ;
#114337=DIRECTION('center_axis',(1.,0.,0.)) ;
#114338=DIRECTION('ref_axis',(0.,0.,-1.)) ;
#114339=DIRECTION('center_axis',(0.,0.,-1.)) ;
#114340=DIRECTION('ref_axis',(-1.,0.,0.)) ;
#114341=DIRECTION('center_axis',(0.,0.,-1.)) ;
#114342=DIRECTION('ref_axis',(-1.,0.,0.)) ;
#114343=DIRECTION('center_axis',(0.,-1.,0.)) ;
#114344=DIRECTION('ref_axis',(0.,0.,-1.)) ;
#114345=DIRECTION('center_axis',(0.,1.,0.)) ;
#114346=DIRECTION('ref_axis',(0.,0.,1.)) ;
#114347=DIRECTION('center_axis',(0.,-1.,0.)) ;
#114348=DIRECTION('ref_axis',(0.,0.,-1.)) ;
#114349=DIRECTION('center_axis',(0.,1.,0.)) ;
#114350=DIRECTION('ref_axis',(0.,0.,-1.)) ;
#114351=DIRECTION('center_axis',(0.,0.,-1.)) ;
#114352=DIRECTION('ref_axis',(-1.,0.,0.)) ;
#114353=DIRECTION('center_axis',(0.,1.,0.)) ;
#114354=DIRECTION('ref_axis',(0.,0.,-1.)) ;
#114355=DIRECTION('center_axis',(0.,0.,-1.)) ;
#114356=DIRECTION('ref_axis',(-1.,0.,0.)) ;
#114357=DIRECTION('center_axis',(0.,0.,1.)) ;
#114358=DIRECTION('ref_axis',(1.,0.,0.)) ;
#114359=DIRECTION('center_axis',(0.,0.,-1.)) ;
#114360=DIRECTION('ref_axis',(-1.,0.,0.)) ;
#114361=DIRECTION('center_axis',(0.,0.,-1.)) ;
#114362=DIRECTION('ref_axis',(-1.,0.,0.)) ;
#114363=DIRECTION('center_axis',(0.,0.,-1.)) ;
#114364=DIRECTION('ref_axis',(-1.,0.,0.)) ;
#114365=DIRECTION('center_axis',(1.,0.,0.)) ;
#114366=DIRECTION('ref_axis',(0.,0.,-1.)) ;
#114367=DIRECTION('center_axis',(-6.13317366673366E-15,0.707106781186563,
-0.707106781186532)) ;
#114368=DIRECTION('ref_axis',(-1.7381816909424E-29,0.707106781186532,0.707106781186563)) ;
#114369=DIRECTION('center_axis',(1.,0.,0.)) ;
#114370=DIRECTION('ref_axis',(0.,0.,-1.)) ;
#114371=DIRECTION('center_axis',(0.,-1.,0.)) ;
#114372=DIRECTION('ref_axis',(0.,0.,-1.)) ;
#114373=DIRECTION('center_axis',(0.,-0.707106781186548,0.707106781186547)) ;
#114374=DIRECTION('ref_axis',(0.,-0.707106781186547,-0.707106781186548)) ;
#114375=DIRECTION('center_axis',(0.,-1.,-1.07081696047951E-16)) ;
#114376=DIRECTION('ref_axis',(0.,1.07081696047951E-16,-1.)) ;
#114377=DIRECTION('center_axis',(0.,-1.,-8.67361737988409E-15)) ;
#114378=DIRECTION('ref_axis',(0.,8.67361737988409E-15,-1.)) ;
#114379=DIRECTION('center_axis',(1.,0.,0.)) ;
#114380=DIRECTION('ref_axis',(0.,0.,-1.)) ;
#114381=DIRECTION('center_axis',(0.,0.,1.)) ;
#114382=DIRECTION('ref_axis',(1.,0.,0.)) ;
#114383=DIRECTION('center_axis',(0.,0.,-1.)) ;
#114384=DIRECTION('ref_axis',(-1.,0.,0.)) ;
#114385=DIRECTION('center_axis',(0.,0.,1.)) ;
#114386=DIRECTION('ref_axis',(1.,0.,0.)) ;
#114387=DIRECTION('center_axis',(0.,0.,1.)) ;
#114388=DIRECTION('ref_axis',(1.,0.,0.)) ;
#114389=DIRECTION('center_axis',(0.,0.,1.)) ;
#114390=DIRECTION('ref_axis',(1.,0.,0.)) ;
#114391=DIRECTION('center_axis',(1.,0.,0.)) ;
#114392=DIRECTION('ref_axis',(0.,0.382683432365085,0.923879532511289)) ;
#114393=DIRECTION('center_axis',(6.13317366673366E-15,-0.707106781186563,
-0.707106781186532)) ;
#114394=DIRECTION('ref_axis',(-1.7381816909424E-29,0.707106781186532,-0.707106781186563)) ;
#114395=DIRECTION('center_axis',(1.,0.,0.)) ;
#114396=DIRECTION('ref_axis',(0.,0.,-1.)) ;
#114397=DIRECTION('center_axis',(0.,0.514231796959093,0.857651245551607)) ;
#114398=DIRECTION('ref_axis',(0.,-0.857651245551607,0.514231796959093)) ;
#114399=DIRECTION('center_axis',(0.,0.707106781186546,0.707106781186549)) ;
#114400=DIRECTION('ref_axis',(0.,-0.707106781186549,0.707106781186546)) ;
#114401=DIRECTION('center_axis',(3.06658683336673E-15,-0.707106781186539,
-0.707106781186556)) ;
#114402=DIRECTION('ref_axis',(1.90456316695698E-29,0.707106781186556,-0.707106781186539)) ;
#114403=DIRECTION('center_axis',(1.,0.,0.)) ;
#114404=DIRECTION('ref_axis',(0.,0.,-1.)) ;
#114405=DIRECTION('center_axis',(0.,-0.514231796959091,0.857651245551608)) ;
#114406=DIRECTION('ref_axis',(0.,-0.857651245551608,-0.514231796959091)) ;
#114407=DIRECTION('center_axis',(1.,0.,0.)) ;
#114408=DIRECTION('ref_axis',(0.,0.,-1.)) ;
#114409=DIRECTION('center_axis',(0.,0.,-1.)) ;
#114410=DIRECTION('ref_axis',(-1.,0.,0.)) ;
#114411=DIRECTION('center_axis',(1.,0.,0.)) ;
#114412=DIRECTION('ref_axis',(0.,0.,-1.)) ;
#114413=DIRECTION('center_axis',(0.,0.,1.)) ;
#114414=DIRECTION('ref_axis',(1.,0.,0.)) ;
#114415=DIRECTION('center_axis',(0.,3.99416362155027E-15,1.)) ;
#114416=DIRECTION('ref_axis',(0.,-1.,3.99416362155027E-15)) ;
#114417=DIRECTION('center_axis',(0.,0.,-1.)) ;
#114418=DIRECTION('ref_axis',(-1.,0.,0.)) ;
#114419=DIRECTION('center_axis',(0.,0.,1.)) ;
#114420=DIRECTION('ref_axis',(1.,0.,0.)) ;
#114421=DIRECTION('center_axis',(0.,0.,1.)) ;
#114422=DIRECTION('ref_axis',(1.,0.,0.)) ;
#114423=DIRECTION('center_axis',(0.,1.,0.)) ;
#114424=DIRECTION('ref_axis',(0.,0.,-1.)) ;
#114425=DIRECTION('center_axis',(0.,-1.,0.)) ;
#114426=DIRECTION('ref_axis',(0.,0.,-1.)) ;
#114427=DIRECTION('center_axis',(1.,0.,0.)) ;
#114428=DIRECTION('ref_axis',(0.,0.,-1.)) ;
#114429=DIRECTION('center_axis',(0.,1.,0.)) ;
#114430=DIRECTION('ref_axis',(0.,0.,1.)) ;
#114431=DIRECTION('center_axis',(0.,1.,0.)) ;
#114432=DIRECTION('ref_axis',(0.,0.,1.)) ;
#114433=DIRECTION('center_axis',(0.,-1.,0.)) ;
#114434=DIRECTION('ref_axis',(0.,0.,-1.)) ;
#114435=DIRECTION('center_axis',(0.,1.,1.07081696047951E-16)) ;
#114436=DIRECTION('ref_axis',(0.,-1.07081696047951E-16,1.)) ;
#114437=DIRECTION('center_axis',(0.,1.,6.50521303491307E-15)) ;
#114438=DIRECTION('ref_axis',(0.,-6.50521303491307E-15,1.)) ;
#114439=DIRECTION('center_axis',(0.,1.,0.)) ;
#114440=DIRECTION('ref_axis',(0.,0.,-1.)) ;
#114441=DIRECTION('center_axis',(0.,0.,1.)) ;
#114442=DIRECTION('ref_axis',(1.,0.,0.)) ;
#114443=DIRECTION('center_axis',(1.,0.,0.)) ;
#114444=DIRECTION('ref_axis',(0.,0.,-1.)) ;
#114445=DIRECTION('center_axis',(0.,0.,-1.)) ;
#114446=DIRECTION('ref_axis',(-1.,0.,0.)) ;
#114447=DIRECTION('center_axis',(0.,0.,-1.)) ;
#114448=DIRECTION('ref_axis',(-1.,0.,0.)) ;
#114449=DIRECTION('center_axis',(0.,-1.,0.)) ;
#114450=DIRECTION('ref_axis',(0.,0.,-1.)) ;
#114451=DIRECTION('center_axis',(0.,1.,0.)) ;
#114452=DIRECTION('ref_axis',(0.,0.,1.)) ;
#114453=DIRECTION('center_axis',(0.,-1.,0.)) ;
#114454=DIRECTION('ref_axis',(0.,0.,-1.)) ;
#114455=DIRECTION('center_axis',(0.,1.,0.)) ;
#114456=DIRECTION('ref_axis',(0.,0.,-1.)) ;
#114457=DIRECTION('center_axis',(0.,0.,-1.)) ;
#114458=DIRECTION('ref_axis',(-1.,0.,0.)) ;
#114459=DIRECTION('center_axis',(0.,1.,0.)) ;
#114460=DIRECTION('ref_axis',(0.,0.,-1.)) ;
#114461=DIRECTION('center_axis',(0.,0.,-1.)) ;
#114462=DIRECTION('ref_axis',(-1.,0.,0.)) ;
#114463=DIRECTION('center_axis',(0.,0.,1.)) ;
#114464=DIRECTION('ref_axis',(1.,0.,0.)) ;
#114465=DIRECTION('center_axis',(0.,0.,-1.)) ;
#114466=DIRECTION('ref_axis',(-1.,0.,0.)) ;
#114467=DIRECTION('center_axis',(0.,0.,-1.)) ;
#114468=DIRECTION('ref_axis',(-1.,0.,0.)) ;
#114469=DIRECTION('center_axis',(0.,0.,-1.)) ;
#114470=DIRECTION('ref_axis',(-1.,0.,0.)) ;
#114471=DIRECTION('center_axis',(1.,0.,0.)) ;
#114472=DIRECTION('ref_axis',(0.,0.,-1.)) ;
#114473=DIRECTION('center_axis',(-6.13317366673366E-15,0.707106781186563,
-0.707106781186532)) ;
#114474=DIRECTION('ref_axis',(-1.7381816909424E-29,0.707106781186532,0.707106781186563)) ;
#114475=DIRECTION('center_axis',(1.,0.,0.)) ;
#114476=DIRECTION('ref_axis',(0.,0.,-1.)) ;
#114477=DIRECTION('center_axis',(0.,-1.,0.)) ;
#114478=DIRECTION('ref_axis',(0.,0.,-1.)) ;
#114479=DIRECTION('center_axis',(0.,-0.707106781186548,0.707106781186547)) ;
#114480=DIRECTION('ref_axis',(0.,-0.707106781186547,-0.707106781186548)) ;
#114481=DIRECTION('center_axis',(0.,-1.,-1.07081696047951E-16)) ;
#114482=DIRECTION('ref_axis',(0.,1.07081696047951E-16,-1.)) ;
#114483=DIRECTION('center_axis',(0.,-1.,-8.67361737988409E-15)) ;
#114484=DIRECTION('ref_axis',(0.,8.67361737988409E-15,-1.)) ;
#114485=DIRECTION('center_axis',(1.,0.,0.)) ;
#114486=DIRECTION('ref_axis',(0.,0.,-1.)) ;
#114487=DIRECTION('center_axis',(0.,0.,1.)) ;
#114488=DIRECTION('ref_axis',(1.,0.,0.)) ;
#114489=DIRECTION('center_axis',(0.,0.,-1.)) ;
#114490=DIRECTION('ref_axis',(-1.,0.,0.)) ;
#114491=DIRECTION('center_axis',(0.,0.,1.)) ;
#114492=DIRECTION('ref_axis',(1.,0.,0.)) ;
#114493=DIRECTION('center_axis',(0.,0.,1.)) ;
#114494=DIRECTION('ref_axis',(1.,0.,0.)) ;
#114495=DIRECTION('center_axis',(0.,0.,1.)) ;
#114496=DIRECTION('ref_axis',(1.,0.,0.)) ;
#114497=DIRECTION('center_axis',(1.,0.,0.)) ;
#114498=DIRECTION('ref_axis',(0.,0.382683432365081,0.92387953251129)) ;
#114499=DIRECTION('center_axis',(0.,-0.707106781186548,-0.707106781186548)) ;
#114500=DIRECTION('ref_axis',(0.,0.707106781186548,-0.707106781186548)) ;
#114501=DIRECTION('center_axis',(1.,0.,0.)) ;
#114502=DIRECTION('ref_axis',(0.,0.,-1.)) ;
#114503=DIRECTION('center_axis',(0.,0.514231796959093,0.857651245551607)) ;
#114504=DIRECTION('ref_axis',(0.,-0.857651245551607,0.514231796959093)) ;
#114505=DIRECTION('center_axis',(0.,0.707106781186546,0.707106781186549)) ;
#114506=DIRECTION('ref_axis',(0.,-0.707106781186549,0.707106781186546)) ;
#114507=DIRECTION('center_axis',(0.,-0.707106781186548,-0.707106781186548)) ;
#114508=DIRECTION('ref_axis',(0.,0.707106781186548,-0.707106781186548)) ;
#114509=DIRECTION('center_axis',(1.,0.,0.)) ;
#114510=DIRECTION('ref_axis',(0.,0.,-1.)) ;
#114511=DIRECTION('center_axis',(0.,-0.514231796959109,0.857651245551597)) ;
#114512=DIRECTION('ref_axis',(0.,-0.857651245551597,-0.514231796959109)) ;
#114513=DIRECTION('center_axis',(1.,0.,0.)) ;
#114514=DIRECTION('ref_axis',(0.,0.,-1.)) ;
#114515=DIRECTION('center_axis',(0.,0.,-1.)) ;
#114516=DIRECTION('ref_axis',(-1.,0.,0.)) ;
#114517=DIRECTION('center_axis',(1.,0.,0.)) ;
#114518=DIRECTION('ref_axis',(0.,0.,-1.)) ;
#114519=DIRECTION('center_axis',(0.,0.,1.)) ;
#114520=DIRECTION('ref_axis',(1.,0.,0.)) ;
#114521=DIRECTION('center_axis',(0.,3.99416362155027E-15,1.)) ;
#114522=DIRECTION('ref_axis',(0.,-1.,3.99416362155027E-15)) ;
#114523=DIRECTION('center_axis',(0.,0.,-1.)) ;
#114524=DIRECTION('ref_axis',(-1.,0.,0.)) ;
#114525=DIRECTION('center_axis',(0.,0.,1.)) ;
#114526=DIRECTION('ref_axis',(1.,0.,0.)) ;
#114527=DIRECTION('center_axis',(0.,0.,1.)) ;
#114528=DIRECTION('ref_axis',(1.,0.,0.)) ;
#114529=DIRECTION('center_axis',(0.,1.,0.)) ;
#114530=DIRECTION('ref_axis',(0.,0.,-1.)) ;
#114531=DIRECTION('center_axis',(0.,-1.,0.)) ;
#114532=DIRECTION('ref_axis',(0.,0.,-1.)) ;
#114533=DIRECTION('center_axis',(1.,0.,0.)) ;
#114534=DIRECTION('ref_axis',(0.,0.,-1.)) ;
#114535=DIRECTION('center_axis',(0.,1.,0.)) ;
#114536=DIRECTION('ref_axis',(0.,0.,1.)) ;
#114537=DIRECTION('center_axis',(0.,1.,0.)) ;
#114538=DIRECTION('ref_axis',(0.,0.,1.)) ;
#114539=DIRECTION('center_axis',(0.,-1.,0.)) ;
#114540=DIRECTION('ref_axis',(0.,0.,-1.)) ;
#114541=DIRECTION('center_axis',(0.,1.,1.07081696047951E-16)) ;
#114542=DIRECTION('ref_axis',(0.,-1.07081696047951E-16,1.)) ;
#114543=DIRECTION('center_axis',(0.,1.,6.50521303491307E-15)) ;
#114544=DIRECTION('ref_axis',(0.,-6.50521303491307E-15,1.)) ;
#114545=DIRECTION('center_axis',(0.,1.,0.)) ;
#114546=DIRECTION('ref_axis',(0.,0.,-1.)) ;
#114547=DIRECTION('center_axis',(0.,0.,1.)) ;
#114548=DIRECTION('ref_axis',(1.,0.,0.)) ;
#114549=DIRECTION('center_axis',(1.,0.,0.)) ;
#114550=DIRECTION('ref_axis',(0.,0.,-1.)) ;
#114551=DIRECTION('center_axis',(0.,0.,-1.)) ;
#114552=DIRECTION('ref_axis',(-1.,0.,0.)) ;
#114553=DIRECTION('center_axis',(0.,0.,-1.)) ;
#114554=DIRECTION('ref_axis',(-1.,0.,0.)) ;
#114555=DIRECTION('center_axis',(0.,-1.,0.)) ;
#114556=DIRECTION('ref_axis',(0.,0.,-1.)) ;
#114557=DIRECTION('center_axis',(0.,1.,0.)) ;
#114558=DIRECTION('ref_axis',(0.,0.,1.)) ;
#114559=DIRECTION('center_axis',(0.,-1.,0.)) ;
#114560=DIRECTION('ref_axis',(0.,0.,-1.)) ;
#114561=DIRECTION('center_axis',(0.,1.,0.)) ;
#114562=DIRECTION('ref_axis',(0.,0.,-1.)) ;
#114563=DIRECTION('center_axis',(0.,0.,-1.)) ;
#114564=DIRECTION('ref_axis',(-1.,0.,0.)) ;
#114565=DIRECTION('center_axis',(0.,1.,0.)) ;
#114566=DIRECTION('ref_axis',(0.,0.,-1.)) ;
#114567=DIRECTION('center_axis',(0.,0.,-1.)) ;
#114568=DIRECTION('ref_axis',(-1.,0.,0.)) ;
#114569=DIRECTION('center_axis',(0.,0.,1.)) ;
#114570=DIRECTION('ref_axis',(1.,0.,0.)) ;
#114571=DIRECTION('center_axis',(0.,0.,-1.)) ;
#114572=DIRECTION('ref_axis',(-1.,0.,0.)) ;
#114573=DIRECTION('center_axis',(0.,0.,-1.)) ;
#114574=DIRECTION('ref_axis',(-1.,0.,0.)) ;
#114575=DIRECTION('center_axis',(0.,0.,-1.)) ;
#114576=DIRECTION('ref_axis',(-1.,0.,0.)) ;
#114577=DIRECTION('center_axis',(1.,0.,0.)) ;
#114578=DIRECTION('ref_axis',(0.,0.,-1.)) ;
#114579=DIRECTION('center_axis',(0.,0.707106781186548,-0.707106781186548)) ;
#114580=DIRECTION('ref_axis',(0.,0.707106781186548,0.707106781186548)) ;
#114581=DIRECTION('center_axis',(1.,0.,0.)) ;
#114582=DIRECTION('ref_axis',(0.,0.,-1.)) ;
#114583=DIRECTION('center_axis',(0.,-1.,0.)) ;
#114584=DIRECTION('ref_axis',(0.,0.,-1.)) ;
#114585=DIRECTION('center_axis',(0.,-0.707106781186548,0.707106781186547)) ;
#114586=DIRECTION('ref_axis',(0.,-0.707106781186547,-0.707106781186548)) ;
#114587=DIRECTION('center_axis',(0.,-1.,-1.07081696047951E-16)) ;
#114588=DIRECTION('ref_axis',(0.,1.07081696047951E-16,-1.)) ;
#114589=DIRECTION('center_axis',(0.,-1.,-8.67361737988409E-15)) ;
#114590=DIRECTION('ref_axis',(0.,8.67361737988409E-15,-1.)) ;
#114591=DIRECTION('center_axis',(1.,0.,0.)) ;
#114592=DIRECTION('ref_axis',(0.,0.,-1.)) ;
#114593=DIRECTION('center_axis',(0.,0.,1.)) ;
#114594=DIRECTION('ref_axis',(1.,0.,0.)) ;
#114595=DIRECTION('center_axis',(0.,0.,-1.)) ;
#114596=DIRECTION('ref_axis',(-1.,0.,0.)) ;
#114597=DIRECTION('center_axis',(0.,0.,1.)) ;
#114598=DIRECTION('ref_axis',(1.,0.,0.)) ;
#114599=DIRECTION('center_axis',(0.,0.,1.)) ;
#114600=DIRECTION('ref_axis',(1.,0.,0.)) ;
#114601=DIRECTION('center_axis',(0.,0.,1.)) ;
#114602=DIRECTION('ref_axis',(1.,0.,0.)) ;
#114603=DIRECTION('center_axis',(1.,0.,0.)) ;
#114604=DIRECTION('ref_axis',(0.,0.382683432365087,0.923879532511288)) ;
#114605=DIRECTION('center_axis',(0.,-0.707106781186548,-0.707106781186548)) ;
#114606=DIRECTION('ref_axis',(0.,0.707106781186548,-0.707106781186548)) ;
#114607=DIRECTION('center_axis',(1.,0.,0.)) ;
#114608=DIRECTION('ref_axis',(0.,0.,-1.)) ;
#114609=DIRECTION('center_axis',(0.,0.514231796959109,0.857651245551597)) ;
#114610=DIRECTION('ref_axis',(0.,-0.857651245551597,0.514231796959109)) ;
#114611=DIRECTION('center_axis',(0.,0.707106781186546,0.707106781186549)) ;
#114612=DIRECTION('ref_axis',(0.,-0.707106781186549,0.707106781186546)) ;
#114613=DIRECTION('center_axis',(0.,-0.707106781186548,-0.707106781186548)) ;
#114614=DIRECTION('ref_axis',(0.,0.707106781186548,-0.707106781186548)) ;
#114615=DIRECTION('center_axis',(1.,0.,0.)) ;
#114616=DIRECTION('ref_axis',(0.,0.,-1.)) ;
#114617=DIRECTION('center_axis',(0.,-0.514231796959109,0.857651245551597)) ;
#114618=DIRECTION('ref_axis',(0.,-0.857651245551597,-0.514231796959109)) ;
#114619=DIRECTION('center_axis',(1.,0.,0.)) ;
#114620=DIRECTION('ref_axis',(0.,0.,-1.)) ;
#114621=DIRECTION('center_axis',(0.,0.,-1.)) ;
#114622=DIRECTION('ref_axis',(-1.,0.,0.)) ;
#114623=DIRECTION('center_axis',(1.,0.,0.)) ;
#114624=DIRECTION('ref_axis',(0.,0.,-1.)) ;
#114625=DIRECTION('center_axis',(0.,0.,1.)) ;
#114626=DIRECTION('ref_axis',(1.,0.,0.)) ;
#114627=DIRECTION('center_axis',(0.,3.99416362155027E-15,1.)) ;
#114628=DIRECTION('ref_axis',(0.,-1.,3.99416362155027E-15)) ;
#114629=DIRECTION('center_axis',(0.,0.,-1.)) ;
#114630=DIRECTION('ref_axis',(-1.,0.,0.)) ;
#114631=DIRECTION('center_axis',(0.,0.,1.)) ;
#114632=DIRECTION('ref_axis',(1.,0.,0.)) ;
#114633=DIRECTION('center_axis',(0.,0.,1.)) ;
#114634=DIRECTION('ref_axis',(1.,0.,0.)) ;
#114635=DIRECTION('center_axis',(0.,1.,0.)) ;
#114636=DIRECTION('ref_axis',(0.,0.,-1.)) ;
#114637=DIRECTION('center_axis',(0.,-1.,0.)) ;
#114638=DIRECTION('ref_axis',(0.,0.,-1.)) ;
#114639=DIRECTION('center_axis',(1.,0.,0.)) ;
#114640=DIRECTION('ref_axis',(0.,0.,-1.)) ;
#114641=DIRECTION('center_axis',(0.,1.,0.)) ;
#114642=DIRECTION('ref_axis',(0.,0.,1.)) ;
#114643=DIRECTION('center_axis',(0.,1.,0.)) ;
#114644=DIRECTION('ref_axis',(0.,0.,1.)) ;
#114645=DIRECTION('center_axis',(0.,-1.,0.)) ;
#114646=DIRECTION('ref_axis',(0.,0.,-1.)) ;
#114647=DIRECTION('center_axis',(0.,1.,1.07081696047951E-16)) ;
#114648=DIRECTION('ref_axis',(0.,-1.07081696047951E-16,1.)) ;
#114649=DIRECTION('center_axis',(0.,1.,6.50521303491307E-15)) ;
#114650=DIRECTION('ref_axis',(0.,-6.50521303491307E-15,1.)) ;
#114651=DIRECTION('center_axis',(0.,1.,0.)) ;
#114652=DIRECTION('ref_axis',(0.,0.,-1.)) ;
#114653=DIRECTION('center_axis',(0.,0.,1.)) ;
#114654=DIRECTION('ref_axis',(1.,0.,0.)) ;
#114655=DIRECTION('center_axis',(1.,0.,0.)) ;
#114656=DIRECTION('ref_axis',(0.,0.,-1.)) ;
#114657=DIRECTION('center_axis',(0.,0.,-1.)) ;
#114658=DIRECTION('ref_axis',(-1.,0.,0.)) ;
#114659=DIRECTION('center_axis',(0.,0.,-1.)) ;
#114660=DIRECTION('ref_axis',(-1.,0.,0.)) ;
#114661=DIRECTION('center_axis',(0.,-1.,0.)) ;
#114662=DIRECTION('ref_axis',(0.,0.,-1.)) ;
#114663=DIRECTION('center_axis',(0.,1.,0.)) ;
#114664=DIRECTION('ref_axis',(0.,0.,1.)) ;
#114665=DIRECTION('center_axis',(0.,-1.,0.)) ;
#114666=DIRECTION('ref_axis',(0.,0.,-1.)) ;
#114667=DIRECTION('center_axis',(0.,1.,0.)) ;
#114668=DIRECTION('ref_axis',(0.,0.,-1.)) ;
#114669=DIRECTION('center_axis',(0.,0.,-1.)) ;
#114670=DIRECTION('ref_axis',(-1.,0.,0.)) ;
#114671=DIRECTION('center_axis',(0.,1.,0.)) ;
#114672=DIRECTION('ref_axis',(0.,0.,-1.)) ;
#114673=DIRECTION('center_axis',(0.,0.,-1.)) ;
#114674=DIRECTION('ref_axis',(-1.,0.,0.)) ;
#114675=DIRECTION('center_axis',(0.,0.,1.)) ;
#114676=DIRECTION('ref_axis',(1.,0.,0.)) ;
#114677=DIRECTION('center_axis',(0.,0.,-1.)) ;
#114678=DIRECTION('ref_axis',(-1.,0.,0.)) ;
#114679=DIRECTION('center_axis',(0.,0.,-1.)) ;
#114680=DIRECTION('ref_axis',(-1.,0.,0.)) ;
#114681=DIRECTION('center_axis',(0.,0.,-1.)) ;
#114682=DIRECTION('ref_axis',(-1.,0.,0.)) ;
#114683=DIRECTION('center_axis',(1.,0.,0.)) ;
#114684=DIRECTION('ref_axis',(0.,0.,-1.)) ;
#114685=DIRECTION('center_axis',(0.,0.707106781186548,-0.707106781186548)) ;
#114686=DIRECTION('ref_axis',(0.,0.707106781186548,0.707106781186548)) ;
#114687=DIRECTION('center_axis',(1.,0.,0.)) ;
#114688=DIRECTION('ref_axis',(0.,0.,-1.)) ;
#114689=DIRECTION('center_axis',(0.,-1.,0.)) ;
#114690=DIRECTION('ref_axis',(0.,0.,-1.)) ;
#114691=DIRECTION('center_axis',(0.,-0.707106781186548,0.707106781186547)) ;
#114692=DIRECTION('ref_axis',(0.,-0.707106781186547,-0.707106781186548)) ;
#114693=DIRECTION('center_axis',(0.,-1.,-1.07081696047951E-16)) ;
#114694=DIRECTION('ref_axis',(0.,1.07081696047951E-16,-1.)) ;
#114695=DIRECTION('center_axis',(0.,-1.,-8.67361737988409E-15)) ;
#114696=DIRECTION('ref_axis',(0.,8.67361737988409E-15,-1.)) ;
#114697=DIRECTION('center_axis',(1.,0.,0.)) ;
#114698=DIRECTION('ref_axis',(0.,0.,-1.)) ;
#114699=DIRECTION('center_axis',(0.,0.,1.)) ;
#114700=DIRECTION('ref_axis',(1.,0.,0.)) ;
#114701=DIRECTION('center_axis',(0.,0.,-1.)) ;
#114702=DIRECTION('ref_axis',(-1.,0.,0.)) ;
#114703=DIRECTION('center_axis',(0.,0.,1.)) ;
#114704=DIRECTION('ref_axis',(1.,0.,0.)) ;
#114705=DIRECTION('center_axis',(0.,0.,1.)) ;
#114706=DIRECTION('ref_axis',(1.,0.,0.)) ;
#114707=DIRECTION('center_axis',(0.,0.,1.)) ;
#114708=DIRECTION('ref_axis',(1.,0.,0.)) ;
#114709=DIRECTION('center_axis',(1.,0.,0.)) ;
#114710=DIRECTION('ref_axis',(0.,0.382683432365088,0.923879532511288)) ;
#114711=DIRECTION('center_axis',(0.,-0.707106781186548,-0.707106781186548)) ;
#114712=DIRECTION('ref_axis',(0.,0.707106781186548,-0.707106781186548)) ;
#114713=DIRECTION('center_axis',(1.,0.,0.)) ;
#114714=DIRECTION('ref_axis',(0.,0.,-1.)) ;
#114715=DIRECTION('center_axis',(0.,0.514231796959109,0.857651245551597)) ;
#114716=DIRECTION('ref_axis',(0.,-0.857651245551597,0.514231796959109)) ;
#114717=DIRECTION('center_axis',(0.,0.707106781186546,0.707106781186549)) ;
#114718=DIRECTION('ref_axis',(0.,-0.707106781186549,0.707106781186546)) ;
#114719=DIRECTION('center_axis',(0.,-0.707106781186548,-0.707106781186548)) ;
#114720=DIRECTION('ref_axis',(0.,0.707106781186548,-0.707106781186548)) ;
#114721=DIRECTION('center_axis',(1.,0.,0.)) ;
#114722=DIRECTION('ref_axis',(0.,0.,-1.)) ;
#114723=DIRECTION('center_axis',(0.,-0.514231796959101,0.857651245551602)) ;
#114724=DIRECTION('ref_axis',(0.,-0.857651245551602,-0.514231796959101)) ;
#114725=DIRECTION('center_axis',(1.,0.,0.)) ;
#114726=DIRECTION('ref_axis',(0.,0.,-1.)) ;
#114727=DIRECTION('center_axis',(0.,8.67361737988405E-15,-1.)) ;
#114728=DIRECTION('ref_axis',(0.,1.,8.67361737988405E-15)) ;
#114729=DIRECTION('center_axis',(1.,0.,0.)) ;
#114730=DIRECTION('ref_axis',(0.,0.,-1.)) ;
#114731=DIRECTION('center_axis',(0.,0.,1.)) ;
#114732=DIRECTION('ref_axis',(1.,0.,0.)) ;
#114733=DIRECTION('center_axis',(0.,3.99416362155027E-15,1.)) ;
#114734=DIRECTION('ref_axis',(0.,-1.,3.99416362155027E-15)) ;
#114735=DIRECTION('center_axis',(0.,0.,-1.)) ;
#114736=DIRECTION('ref_axis',(-1.,0.,0.)) ;
#114737=DIRECTION('center_axis',(0.,0.,1.)) ;
#114738=DIRECTION('ref_axis',(1.,0.,0.)) ;
#114739=DIRECTION('center_axis',(0.,0.,1.)) ;
#114740=DIRECTION('ref_axis',(1.,0.,0.)) ;
#114741=DIRECTION('center_axis',(0.,1.,0.)) ;
#114742=DIRECTION('ref_axis',(0.,0.,-1.)) ;
#114743=DIRECTION('center_axis',(0.,-1.,0.)) ;
#114744=DIRECTION('ref_axis',(0.,0.,-1.)) ;
#114745=DIRECTION('center_axis',(1.,0.,0.)) ;
#114746=DIRECTION('ref_axis',(0.,0.,-1.)) ;
#114747=DIRECTION('center_axis',(0.,1.,0.)) ;
#114748=DIRECTION('ref_axis',(0.,0.,1.)) ;
#114749=DIRECTION('center_axis',(0.,1.,0.)) ;
#114750=DIRECTION('ref_axis',(0.,0.,1.)) ;
#114751=DIRECTION('center_axis',(0.,-1.,0.)) ;
#114752=DIRECTION('ref_axis',(0.,0.,-1.)) ;
#114753=DIRECTION('center_axis',(0.,1.,1.07081696047951E-16)) ;
#114754=DIRECTION('ref_axis',(0.,-1.07081696047951E-16,1.)) ;
#114755=DIRECTION('center_axis',(0.,1.,6.50521303491301E-15)) ;
#114756=DIRECTION('ref_axis',(0.,-6.50521303491301E-15,1.)) ;
#114757=DIRECTION('center_axis',(0.,1.,0.)) ;
#114758=DIRECTION('ref_axis',(0.,0.,-1.)) ;
#114759=DIRECTION('center_axis',(0.,0.,1.)) ;
#114760=DIRECTION('ref_axis',(1.,0.,0.)) ;
#114761=DIRECTION('center_axis',(1.,0.,0.)) ;
#114762=DIRECTION('ref_axis',(0.,0.,-1.)) ;
#114763=DIRECTION('center_axis',(0.,0.,-1.)) ;
#114764=DIRECTION('ref_axis',(-1.,0.,0.)) ;
#114765=DIRECTION('center_axis',(0.,0.,-1.)) ;
#114766=DIRECTION('ref_axis',(-1.,0.,0.)) ;
#114767=DIRECTION('center_axis',(0.,-1.,0.)) ;
#114768=DIRECTION('ref_axis',(0.,0.,-1.)) ;
#114769=DIRECTION('center_axis',(0.,1.,0.)) ;
#114770=DIRECTION('ref_axis',(0.,0.,1.)) ;
#114771=DIRECTION('center_axis',(0.,-1.,0.)) ;
#114772=DIRECTION('ref_axis',(0.,0.,-1.)) ;
#114773=DIRECTION('center_axis',(0.,1.,0.)) ;
#114774=DIRECTION('ref_axis',(0.,0.,-1.)) ;
#114775=DIRECTION('center_axis',(0.,0.,-1.)) ;
#114776=DIRECTION('ref_axis',(-1.,0.,0.)) ;
#114777=DIRECTION('center_axis',(0.,1.,0.)) ;
#114778=DIRECTION('ref_axis',(0.,0.,-1.)) ;
#114779=DIRECTION('center_axis',(0.,0.,-1.)) ;
#114780=DIRECTION('ref_axis',(-1.,0.,0.)) ;
#114781=DIRECTION('center_axis',(0.,0.,1.)) ;
#114782=DIRECTION('ref_axis',(1.,0.,0.)) ;
#114783=DIRECTION('center_axis',(0.,0.,-1.)) ;
#114784=DIRECTION('ref_axis',(-1.,0.,0.)) ;
#114785=DIRECTION('center_axis',(0.,0.,-1.)) ;
#114786=DIRECTION('ref_axis',(-1.,0.,0.)) ;
#114787=DIRECTION('center_axis',(0.,8.67361737988405E-15,-1.)) ;
#114788=DIRECTION('ref_axis',(0.,1.,8.67361737988405E-15)) ;
#114789=DIRECTION('center_axis',(1.,0.,0.)) ;
#114790=DIRECTION('ref_axis',(0.,0.,-1.)) ;
#114791=DIRECTION('center_axis',(0.,0.707106781186548,-0.707106781186548)) ;
#114792=DIRECTION('ref_axis',(0.,0.707106781186548,0.707106781186548)) ;
#114793=DIRECTION('center_axis',(1.,0.,0.)) ;
#114794=DIRECTION('ref_axis',(0.,0.,-1.)) ;
#114795=DIRECTION('center_axis',(0.,-1.,0.)) ;
#114796=DIRECTION('ref_axis',(0.,0.,-1.)) ;
#114797=DIRECTION('center_axis',(0.,-0.707106781186548,0.707106781186547)) ;
#114798=DIRECTION('ref_axis',(0.,-0.707106781186547,-0.707106781186548)) ;
#114799=DIRECTION('center_axis',(0.,-1.,-1.07081696047951E-16)) ;
#114800=DIRECTION('ref_axis',(0.,1.07081696047951E-16,-1.)) ;
#114801=DIRECTION('center_axis',(0.,-1.,-8.67361737988401E-15)) ;
#114802=DIRECTION('ref_axis',(0.,8.67361737988401E-15,-1.)) ;
#114803=DIRECTION('center_axis',(1.,0.,0.)) ;
#114804=DIRECTION('ref_axis',(0.,0.,-1.)) ;
#114805=DIRECTION('center_axis',(0.,0.,1.)) ;
#114806=DIRECTION('ref_axis',(1.,0.,0.)) ;
#114807=DIRECTION('center_axis',(0.,0.,-1.)) ;
#114808=DIRECTION('ref_axis',(-1.,0.,0.)) ;
#114809=DIRECTION('center_axis',(0.,0.,1.)) ;
#114810=DIRECTION('ref_axis',(1.,0.,0.)) ;
#114811=DIRECTION('center_axis',(0.,0.,1.)) ;
#114812=DIRECTION('ref_axis',(1.,0.,0.)) ;
#114813=DIRECTION('center_axis',(0.,0.,1.)) ;
#114814=DIRECTION('ref_axis',(1.,0.,0.)) ;
#114815=DIRECTION('center_axis',(1.,0.,0.)) ;
#114816=DIRECTION('ref_axis',(0.,0.38268343236509,0.923879532511287)) ;
#114817=DIRECTION('center_axis',(0.,-0.70710678118655,-0.707106781186545)) ;
#114818=DIRECTION('ref_axis',(0.,0.707106781186545,-0.70710678118655)) ;
#114819=DIRECTION('center_axis',(1.,0.,0.)) ;
#114820=DIRECTION('ref_axis',(0.,0.,-1.)) ;
#114821=DIRECTION('center_axis',(0.,0.514231796959101,0.857651245551602)) ;
#114822=DIRECTION('ref_axis',(0.,-0.857651245551602,0.514231796959101)) ;
#114823=DIRECTION('center_axis',(0.,0.707106781186546,0.707106781186549)) ;
#114824=DIRECTION('ref_axis',(0.,-0.707106781186549,0.707106781186546)) ;
#114825=DIRECTION('center_axis',(1.88079096131567E-29,-0.707106781186545,
-0.70710678118655)) ;
#114826=DIRECTION('ref_axis',(7.62257770433106E-46,0.70710678118655,-0.707106781186545)) ;
#114827=DIRECTION('center_axis',(1.,0.,0.)) ;
#114828=DIRECTION('ref_axis',(0.,0.,-1.)) ;
#114829=DIRECTION('center_axis',(0.,-0.514231796959101,0.857651245551602)) ;
#114830=DIRECTION('ref_axis',(0.,-0.857651245551602,-0.514231796959101)) ;
#114831=DIRECTION('center_axis',(1.,0.,0.)) ;
#114832=DIRECTION('ref_axis',(0.,0.,-1.)) ;
#114833=DIRECTION('center_axis',(0.,0.,-1.)) ;
#114834=DIRECTION('ref_axis',(-1.,0.,0.)) ;
#114835=DIRECTION('center_axis',(1.,0.,0.)) ;
#114836=DIRECTION('ref_axis',(0.,0.,-1.)) ;
#114837=DIRECTION('center_axis',(0.,0.,1.)) ;
#114838=DIRECTION('ref_axis',(1.,0.,0.)) ;
#114839=DIRECTION('center_axis',(0.,3.99416362155027E-15,1.)) ;
#114840=DIRECTION('ref_axis',(0.,-1.,3.99416362155027E-15)) ;
#114841=DIRECTION('center_axis',(0.,-4.33680868994202E-15,-1.)) ;
#114842=DIRECTION('ref_axis',(0.,1.,-4.33680868994202E-15)) ;
#114843=DIRECTION('center_axis',(0.,0.,1.)) ;
#114844=DIRECTION('ref_axis',(1.,0.,0.)) ;
#114845=DIRECTION('center_axis',(0.,-4.33680868994202E-15,1.)) ;
#114846=DIRECTION('ref_axis',(0.,-1.,-4.33680868994202E-15)) ;
#114847=DIRECTION('center_axis',(0.,1.,0.)) ;
#114848=DIRECTION('ref_axis',(0.,0.,-1.)) ;
#114849=DIRECTION('center_axis',(0.,-1.,0.)) ;
#114850=DIRECTION('ref_axis',(0.,0.,-1.)) ;
#114851=DIRECTION('center_axis',(1.,0.,0.)) ;
#114852=DIRECTION('ref_axis',(0.,0.,-1.)) ;
#114853=DIRECTION('center_axis',(0.,1.,0.)) ;
#114854=DIRECTION('ref_axis',(0.,0.,1.)) ;
#114855=DIRECTION('center_axis',(0.,1.,0.)) ;
#114856=DIRECTION('ref_axis',(0.,0.,1.)) ;
#114857=DIRECTION('center_axis',(0.,-1.,0.)) ;
#114858=DIRECTION('ref_axis',(0.,0.,-1.)) ;
#114859=DIRECTION('center_axis',(0.,1.,1.07081696047951E-16)) ;
#114860=DIRECTION('ref_axis',(0.,-1.07081696047951E-16,1.)) ;
#114861=DIRECTION('center_axis',(0.,1.,6.50521303491304E-15)) ;
#114862=DIRECTION('ref_axis',(0.,-6.50521303491304E-15,1.)) ;
#114863=DIRECTION('center_axis',(0.,1.,0.)) ;
#114864=DIRECTION('ref_axis',(0.,0.,-1.)) ;
#114865=DIRECTION('center_axis',(0.,0.,1.)) ;
#114866=DIRECTION('ref_axis',(1.,0.,0.)) ;
#114867=DIRECTION('center_axis',(1.,0.,0.)) ;
#114868=DIRECTION('ref_axis',(0.,0.,-1.)) ;
#114869=DIRECTION('center_axis',(0.,0.,-1.)) ;
#114870=DIRECTION('ref_axis',(-1.,0.,0.)) ;
#114871=DIRECTION('center_axis',(0.,0.,-1.)) ;
#114872=DIRECTION('ref_axis',(-1.,0.,0.)) ;
#114873=DIRECTION('center_axis',(1.53063836115601E-16,-1.,-1.30104260698261E-16)) ;
#114874=DIRECTION('ref_axis',(1.,1.53063836115601E-16,1.99142572374599E-32)) ;
#114875=DIRECTION('center_axis',(0.,1.,0.)) ;
#114876=DIRECTION('ref_axis',(0.,0.,1.)) ;
#114877=DIRECTION('center_axis',(0.,-1.,0.)) ;
#114878=DIRECTION('ref_axis',(0.,0.,-1.)) ;
#114879=DIRECTION('center_axis',(1.,1.53063836115601E-16,2.73691106313441E-48)) ;
#114880=DIRECTION('ref_axis',(-1.53063836115601E-16,1.,-4.18922106430579E-64)) ;
#114881=DIRECTION('center_axis',(-1.,0.,0.)) ;
#114882=DIRECTION('ref_axis',(0.,0.,1.)) ;
#114883=DIRECTION('center_axis',(1.,1.53063836115601E-16,0.)) ;
#114884=DIRECTION('ref_axis',(1.53063836115601E-16,-1.,0.)) ;
#114885=DIRECTION('center_axis',(0.,1.,0.)) ;
#114886=DIRECTION('ref_axis',(1.,0.,0.)) ;
#114887=DIRECTION('center_axis',(0.,1.,0.)) ;
#114888=DIRECTION('ref_axis',(0.,0.,-1.)) ;
#114889=DIRECTION('center_axis',(0.,0.,1.)) ;
#114890=DIRECTION('ref_axis',(-1.,0.,0.)) ;
#114891=DIRECTION('center_axis',(0.,1.,0.)) ;
#114892=DIRECTION('ref_axis',(1.,0.,0.)) ;
#114893=DIRECTION('center_axis',(0.,0.,1.)) ;
#114894=DIRECTION('ref_axis',(-1.,0.,0.)) ;
#114895=DIRECTION('center_axis',(1.,1.0842021724855E-15,0.)) ;
#114896=DIRECTION('ref_axis',(1.0842021724855E-15,-1.,0.)) ;
#114897=DIRECTION('center_axis',(-1.,-1.53063836115601E-16,0.)) ;
#114898=DIRECTION('ref_axis',(0.,-1.,0.)) ;
#114899=DIRECTION('center_axis',(0.,0.,-1.)) ;
#114900=DIRECTION('ref_axis',(1.,0.,0.)) ;
#114901=DIRECTION('center_axis',(0.,0.,-1.)) ;
#114902=DIRECTION('ref_axis',(0.804034447892619,0.594582716366707,0.)) ;
#114903=DIRECTION('center_axis',(0.,0.,1.)) ;
#114904=DIRECTION('ref_axis',(1.,0.,0.)) ;
#114905=DIRECTION('',(0.,0.,-1.)) ;
#114906=DIRECTION('center_axis',(-2.16840434497101E-16,1.,1.30104260698261E-16)) ;
#114907=DIRECTION('ref_axis',(1.,2.16840434497101E-16,1.22464679914735E-16)) ;
#114908=DIRECTION('',(-2.16840434497101E-16,1.,1.30104260698261E-16)) ;
#114909=DIRECTION('center_axis',(0.,1.,0.)) ;
#114910=DIRECTION('ref_axis',(0.,0.,1.)) ;
#114911=DIRECTION('center_axis',(-1.,-1.53063836115601E-16,-2.73691106313441E-48)) ;
#114912=DIRECTION('ref_axis',(1.53063836115601E-16,-1.,4.18922106430579E-64)) ;
#114913=DIRECTION('center_axis',(1.,2.16840434497101E-16,0.)) ;
#114914=DIRECTION('ref_axis',(2.16840434497101E-16,-1.,0.)) ;
#114915=DIRECTION('center_axis',(0.,0.,1.)) ;
#114916=DIRECTION('ref_axis',(1.,0.,0.)) ;
#114917=DIRECTION('center_axis',(-1.25542992828747E-32,1.020425574104E-16,
1.)) ;
#114918=DIRECTION('ref_axis',(-1.28107280532009E-48,-1.,1.020425574104E-16)) ;
#114919=DIRECTION('center_axis',(0.,0.,1.)) ;
#114920=DIRECTION('ref_axis',(1.,0.,0.)) ;
#114921=DIRECTION('center_axis',(0.,0.,-1.)) ;
#114922=DIRECTION('ref_axis',(-1.,0.,0.)) ;
#114923=DIRECTION('center_axis',(1.,1.53063836115601E-16,-2.73691106313441E-48)) ;
#114924=DIRECTION('ref_axis',(-1.53063836115601E-16,1.,4.18922106430579E-64)) ;
#114925=DIRECTION('center_axis',(-1.,0.,0.)) ;
#114926=DIRECTION('ref_axis',(0.,0.,1.)) ;
#114927=DIRECTION('center_axis',(1.,1.53063836115601E-16,0.)) ;
#114928=DIRECTION('ref_axis',(1.53063836115601E-16,-1.,0.)) ;
#114929=DIRECTION('center_axis',(0.,1.,0.)) ;
#114930=DIRECTION('ref_axis',(1.,0.,0.)) ;
#114931=DIRECTION('center_axis',(-1.,-2.16840434497101E-16,0.)) ;
#114932=DIRECTION('ref_axis',(0.,-1.,0.)) ;
#114933=DIRECTION('center_axis',(0.,0.,-1.)) ;
#114934=DIRECTION('ref_axis',(1.,0.,0.)) ;
#114935=DIRECTION('center_axis',(-1.25542992828747E-32,1.020425574104E-16,
1.)) ;
#114936=DIRECTION('ref_axis',(0.,-1.,0.)) ;
#114937=DIRECTION('center_axis',(0.,-1.,0.)) ;
#114938=DIRECTION('ref_axis',(-6.50521303491301E-15,0.,1.)) ;
#114939=DIRECTION('center_axis',(-1.,0.,0.)) ;
#114940=DIRECTION('ref_axis',(0.,0.,-1.)) ;
#114941=DIRECTION('center_axis',(-1.,-1.53063836115601E-16,0.)) ;
#114942=DIRECTION('ref_axis',(0.,-1.,0.)) ;
#114943=DIRECTION('center_axis',(0.,-1.,0.)) ;
#114944=DIRECTION('ref_axis',(0.,0.,1.)) ;
#114945=DIRECTION('center_axis',(0.,0.,-1.)) ;
#114946=DIRECTION('ref_axis',(-1.,0.,0.)) ;
#114947=DIRECTION('center_axis',(0.,0.,-1.)) ;
#114948=DIRECTION('ref_axis',(-1.,0.,0.)) ;
#114949=DIRECTION('center_axis',(1.,1.53063836115601E-16,-3.06472600140763E-33)) ;
#114950=DIRECTION('ref_axis',(-1.53063836115601E-16,1.,4.69098718418678E-49)) ;
#114951=DIRECTION('center_axis',(-1.,0.,0.)) ;
#114952=DIRECTION('ref_axis',(0.,0.,1.)) ;
#114953=DIRECTION('center_axis',(-1.53063836115601E-16,1.,-1.020425574104E-16)) ;
#114954=DIRECTION('ref_axis',(-1.,-1.53063836115601E-16,1.3684555315672E-47)) ;
#114955=DIRECTION('',(1.53063836115601E-16,-1.,1.020425574104E-16)) ;
#114956=DIRECTION('center_axis',(0.,-1.,0.)) ;
#114957=DIRECTION('ref_axis',(0.,0.,-1.)) ;
#114958=DIRECTION('center_axis',(-1.53063836115601E-16,1.,-1.30104260698261E-16)) ;
#114959=DIRECTION('ref_axis',(-1.,-1.53063836115601E-16,1.99142572374599E-32)) ;
#114960=DIRECTION('center_axis',(0.,-1.,0.)) ;
#114961=DIRECTION('ref_axis',(0.,0.,-1.)) ;
#114962=DIRECTION('center_axis',(-1.,-1.53063836115601E-16,2.73691106313441E-48)) ;
#114963=DIRECTION('ref_axis',(1.53063836115601E-16,-1.,-4.18922106430579E-64)) ;
#114964=DIRECTION('center_axis',(1.,2.16840434497101E-16,0.)) ;
#114965=DIRECTION('ref_axis',(2.16840434497101E-16,-1.,0.)) ;
#114966=DIRECTION('center_axis',(-1.,0.,2.16840434497102E-15)) ;
#114967=DIRECTION('ref_axis',(2.16840434497102E-15,0.,1.)) ;
#114968=DIRECTION('center_axis',(-1.,-2.16840434497101E-16,0.)) ;
#114969=DIRECTION('ref_axis',(0.,-1.,0.)) ;
#114970=DIRECTION('center_axis',(0.,0.,1.)) ;
#114971=DIRECTION('ref_axis',(-1.,0.,0.)) ;
#114972=DIRECTION('center_axis',(0.,1.,0.)) ;
#114973=DIRECTION('ref_axis',(1.,0.,0.)) ;
#114974=DIRECTION('center_axis',(0.,1.,0.)) ;
#114975=DIRECTION('ref_axis',(0.,0.,-1.)) ;
#114976=DIRECTION('center_axis',(1.,0.,0.)) ;
#114977=DIRECTION('ref_axis',(0.,-1.,0.)) ;
#114978=DIRECTION('center_axis',(1.,6.50521303491304E-15,0.)) ;
#114979=DIRECTION('ref_axis',(-6.50521303491304E-15,1.,0.)) ;
#114980=DIRECTION('center_axis',(8.67361737988403E-15,1.,0.)) ;
#114981=DIRECTION('ref_axis',(-1.,8.67361737988403E-15,0.)) ;
#114982=DIRECTION('center_axis',(1.2303003375722E-16,-1.,1.020425574104E-16)) ;
#114983=DIRECTION('ref_axis',(1.,1.2303003375722E-16,-1.25542992828747E-32)) ;
#114984=DIRECTION('center_axis',(0.,1.,0.)) ;
#114985=DIRECTION('ref_axis',(0.,0.,1.)) ;
#114986=DIRECTION('center_axis',(0.,1.,0.)) ;
#114987=DIRECTION('ref_axis',(1.,0.,0.)) ;
#114988=DIRECTION('center_axis',(1.,1.2303003375722E-16,0.)) ;
#114989=DIRECTION('ref_axis',(1.2303003375722E-16,-1.,0.)) ;
#114990=DIRECTION('center_axis',(0.,0.,1.)) ;
#114991=DIRECTION('ref_axis',(-1.,0.,0.)) ;
#114992=DIRECTION('center_axis',(0.,1.,0.)) ;
#114993=DIRECTION('ref_axis',(1.,0.,0.)) ;
#114994=DIRECTION('center_axis',(0.,0.,-1.)) ;
#114995=DIRECTION('ref_axis',(1.,0.,0.)) ;
#114996=DIRECTION('center_axis',(0.,0.,-1.)) ;
#114997=DIRECTION('ref_axis',(-1.,0.,0.)) ;
#114998=DIRECTION('center_axis',(0.,0.,1.)) ;
#114999=DIRECTION('ref_axis',(1.,0.,0.)) ;
#115000=DIRECTION('center_axis',(-2.16840434497101E-16,1.,-1.020425574104E-16)) ;
#115001=DIRECTION('ref_axis',(-1.,-2.16840434497101E-16,5.47382212626882E-48)) ;
#115002=DIRECTION('center_axis',(0.,1.,0.)) ;
#115003=DIRECTION('ref_axis',(0.,0.,-1.)) ;
#115004=DIRECTION('center_axis',(1.,0.,1.25542992828747E-32)) ;
#115005=DIRECTION('ref_axis',(1.25542992828747E-32,0.,-1.)) ;
#115006=DIRECTION('center_axis',(1.,0.,0.)) ;
#115007=DIRECTION('ref_axis',(0.,0.,-1.)) ;
#115008=DIRECTION('center_axis',(-1.,-1.2303003375722E-16,0.)) ;
#115009=DIRECTION('ref_axis',(0.,-1.,0.)) ;
#115010=DIRECTION('center_axis',(0.,0.,-1.)) ;
#115011=DIRECTION('ref_axis',(1.,0.,0.)) ;
#115012=DIRECTION('center_axis',(0.,0.,-1.)) ;
#115013=DIRECTION('ref_axis',(-1.,0.,0.)) ;
#115014=DIRECTION('',(0.,0.,1.)) ;
#115015=DIRECTION('center_axis',(0.,0.,1.)) ;
#115016=DIRECTION('ref_axis',(1.,0.,0.)) ;
#115017=DIRECTION('center_axis',(0.,0.,1.)) ;
#115018=DIRECTION('ref_axis',(1.,0.,0.)) ;
#115019=DIRECTION('center_axis',(6.27714964143733E-33,-5.10212787052002E-17,
-1.)) ;
#115020=DIRECTION('ref_axis',(3.20268201330022E-49,1.,-5.10212787052002E-17)) ;
#115021=DIRECTION('center_axis',(1.,1.53063836115601E-16,-1.53236300070382E-33)) ;
#115022=DIRECTION('ref_axis',(-1.53063836115601E-16,1.,2.34549359209339E-49)) ;
#115023=DIRECTION('center_axis',(-1.,0.,0.)) ;
#115024=DIRECTION('ref_axis',(0.,0.,1.)) ;
#115025=DIRECTION('center_axis',(1.,0.,0.)) ;
#115026=DIRECTION('ref_axis',(0.,0.,-1.)) ;
#115027=DIRECTION('center_axis',(0.,1.,0.)) ;
#115028=DIRECTION('ref_axis',(1.,0.,0.)) ;
#115029=DIRECTION('center_axis',(-4.33680868994202E-15,1.,0.)) ;
#115030=DIRECTION('ref_axis',(1.,4.33680868994202E-15,0.)) ;
#115031=DIRECTION('center_axis',(0.,-1.,0.)) ;
#115032=DIRECTION('ref_axis',(0.,0.,-1.)) ;
#115033=DIRECTION('center_axis',(0.,0.,-1.)) ;
#115034=DIRECTION('ref_axis',(1.,0.,0.)) ;
#115035=DIRECTION('center_axis',(0.,0.,1.)) ;
#115036=DIRECTION('ref_axis',(1.,0.,0.)) ;
#115037=DIRECTION('center_axis',(0.,0.,-1.)) ;
#115038=DIRECTION('ref_axis',(-1.,0.,0.)) ;
#115039=DIRECTION('center_axis',(0.,1.,0.)) ;
#115040=DIRECTION('ref_axis',(1.,0.,0.)) ;
#115041=DIRECTION('center_axis',(1.,1.2303003375722E-16,0.)) ;
#115042=DIRECTION('ref_axis',(1.2303003375722E-16,-1.,0.)) ;
#115043=DIRECTION('center_axis',(0.,1.,0.)) ;
#115044=DIRECTION('ref_axis',(-6.50521303491307E-15,0.,-1.)) ;
#115045=DIRECTION('center_axis',(6.27714964143733E-33,-5.10212787052002E-17,
-1.)) ;
#115046=DIRECTION('ref_axis',(0.,1.,0.)) ;
#115047=DIRECTION('center_axis',(0.,-1.,0.)) ;
#115048=DIRECTION('ref_axis',(0.,0.,1.)) ;
#115049=DIRECTION('center_axis',(2.16840434497101E-16,-1.,5.10212787052002E-17)) ;
#115050=DIRECTION('ref_axis',(1.,2.16840434497101E-16,-5.47382212626882E-48)) ;
#115051=DIRECTION('center_axis',(0.,1.,0.)) ;
#115052=DIRECTION('ref_axis',(0.,0.,-1.)) ;
#115053=DIRECTION('center_axis',(0.,0.,1.)) ;
#115054=DIRECTION('ref_axis',(1.,0.,0.)) ;
#115055=DIRECTION('center_axis',(0.,0.,-1.)) ;
#115056=DIRECTION('ref_axis',(-1.,0.,0.)) ;
#115057=DIRECTION('center_axis',(-1.,-1.2303003375722E-16,0.)) ;
#115058=DIRECTION('ref_axis',(0.,-1.,0.)) ;
#115059=DIRECTION('center_axis',(0.,-1.,0.)) ;
#115060=DIRECTION('ref_axis',(0.,0.,1.)) ;
#115061=DIRECTION('center_axis',(1.53063836115601E-16,-1.,5.10212787052002E-17)) ;
#115062=DIRECTION('ref_axis',(1.,1.53063836115601E-16,-6.84227765783602E-48)) ;
#115063=DIRECTION('',(-1.53063836115601E-16,1.,-5.10212787052002E-17)) ;
#115064=DIRECTION('center_axis',(0.,-1.,0.)) ;
#115065=DIRECTION('ref_axis',(0.,0.,-1.)) ;
#115066=DIRECTION('center_axis',(-1.,0.,0.)) ;
#115067=DIRECTION('ref_axis',(0.,0.,-1.)) ;
#115068=DIRECTION('center_axis',(-1.2303003375722E-16,1.,-5.10212787052002E-17)) ;
#115069=DIRECTION('ref_axis',(-1.,-1.2303003375722E-16,6.27714964143733E-33)) ;
#115070=DIRECTION('center_axis',(-8.67361737988403E-15,-1.,0.)) ;
#115071=DIRECTION('ref_axis',(1.,-8.67361737988403E-15,0.)) ;
#115072=DIRECTION('center_axis',(1.,0.,6.27714964143733E-33)) ;
#115073=DIRECTION('ref_axis',(6.27714964143733E-33,0.,-1.)) ;
#115074=DIRECTION('center_axis',(-1.,0.,-6.50521303491318E-15)) ;
#115075=DIRECTION('ref_axis',(-6.50521303491318E-15,0.,1.)) ;
#115076=DIRECTION('center_axis',(1.,0.,0.)) ;
#115077=DIRECTION('ref_axis',(0.,1.,0.)) ;
#115078=DIRECTION('center_axis',(0.,0.,-1.)) ;
#115079=DIRECTION('ref_axis',(-1.,0.,0.)) ;
#115080=DIRECTION('center_axis',(0.,0.,1.)) ;
#115081=DIRECTION('ref_axis',(1.,0.,0.)) ;
#115082=DIRECTION('center_axis',(0.,0.,-1.)) ;
#115083=DIRECTION('ref_axis',(-1.,0.,0.)) ;
#115084=DIRECTION('center_axis',(-1.,0.,0.)) ;
#115085=DIRECTION('ref_axis',(0.,0.,1.)) ;
#115086=DIRECTION('center_axis',(0.,-1.,0.)) ;
#115087=DIRECTION('ref_axis',(0.,0.,-1.)) ;
#115088=DIRECTION('center_axis',(0.,1.,0.)) ;
#115089=DIRECTION('ref_axis',(0.,0.,1.)) ;
#115090=DIRECTION('center_axis',(0.,1.,-6.50521303491307E-15)) ;
#115091=DIRECTION('ref_axis',(0.,6.50521303491307E-15,1.)) ;
#115092=DIRECTION('center_axis',(0.,-1.,0.)) ;
#115093=DIRECTION('ref_axis',(0.,0.,-1.)) ;
#115094=DIRECTION('center_axis',(0.,-1.,0.)) ;
#115095=DIRECTION('ref_axis',(0.,0.,-1.)) ;
#115096=DIRECTION('center_axis',(0.,-1.,-1.07081696047951E-16)) ;
#115097=DIRECTION('ref_axis',(0.,1.07081696047951E-16,-1.)) ;
#115098=DIRECTION('center_axis',(0.,1.,0.)) ;
#115099=DIRECTION('ref_axis',(0.,0.,1.)) ;
#115100=DIRECTION('center_axis',(-1.,0.,0.)) ;
#115101=DIRECTION('ref_axis',(0.,0.,1.)) ;
#115102=DIRECTION('center_axis',(0.,0.,1.)) ;
#115103=DIRECTION('ref_axis',(1.,0.,0.)) ;
#115104=DIRECTION('center_axis',(0.,1.,0.)) ;
#115105=DIRECTION('ref_axis',(0.,0.,1.)) ;
#115106=DIRECTION('center_axis',(0.,-1.73472347597681E-14,-1.)) ;
#115107=DIRECTION('ref_axis',(0.,1.,-1.73472347597681E-14)) ;
#115108=DIRECTION('center_axis',(0.,0.,1.)) ;
#115109=DIRECTION('ref_axis',(1.,0.,0.)) ;
#115110=DIRECTION('center_axis',(0.,0.,1.)) ;
#115111=DIRECTION('ref_axis',(1.,0.,0.)) ;
#115112=DIRECTION('center_axis',(0.,0.,1.)) ;
#115113=DIRECTION('ref_axis',(1.,0.,0.)) ;
#115114=DIRECTION('center_axis',(0.,0.,-1.)) ;
#115115=DIRECTION('ref_axis',(-1.,0.,0.)) ;
#115116=DIRECTION('center_axis',(0.,1.,0.)) ;
#115117=DIRECTION('ref_axis',(0.,0.,1.)) ;
#115118=DIRECTION('center_axis',(0.,-0.707106781186545,0.70710678118655)) ;
#115119=DIRECTION('ref_axis',(0.,-0.70710678118655,-0.707106781186545)) ;
#115120=DIRECTION('center_axis',(0.,1.,0.)) ;
#115121=DIRECTION('ref_axis',(0.,0.,1.)) ;
#115122=DIRECTION('center_axis',(0.,-0.514231796959109,-0.857651245551597)) ;
#115123=DIRECTION('ref_axis',(0.,0.857651245551597,-0.514231796959109)) ;
#115124=DIRECTION('center_axis',(0.,-0.707106781186548,0.707106781186547)) ;
#115125=DIRECTION('ref_axis',(0.,-0.707106781186547,-0.707106781186548)) ;
#115126=DIRECTION('center_axis',(0.,-0.707106781186548,0.707106781186548)) ;
#115127=DIRECTION('ref_axis',(0.,-0.707106781186548,-0.707106781186548)) ;
#115128=DIRECTION('center_axis',(-1.,0.,0.)) ;
#115129=DIRECTION('ref_axis',(0.,0.,1.)) ;
#115130=DIRECTION('center_axis',(0.,0.514231796959101,-0.857651245551602)) ;
#115131=DIRECTION('ref_axis',(0.,0.857651245551602,0.514231796959101)) ;
#115132=DIRECTION('center_axis',(0.,1.,0.)) ;
#115133=DIRECTION('ref_axis',(0.,0.,1.)) ;
#115134=DIRECTION('center_axis',(0.,0.,-1.)) ;
#115135=DIRECTION('ref_axis',(-1.,0.,0.)) ;
#115136=DIRECTION('center_axis',(0.,1.,0.)) ;
#115137=DIRECTION('ref_axis',(0.,0.,1.)) ;
#115138=DIRECTION('center_axis',(0.,0.,-1.)) ;
#115139=DIRECTION('ref_axis',(-1.,0.,0.)) ;
#115140=DIRECTION('center_axis',(0.,0.,-1.)) ;
#115141=DIRECTION('ref_axis',(-1.,0.,0.)) ;
#115142=DIRECTION('center_axis',(0.,0.,1.)) ;
#115143=DIRECTION('ref_axis',(1.,0.,0.)) ;
#115144=DIRECTION('center_axis',(0.,0.,-1.)) ;
#115145=DIRECTION('ref_axis',(-1.,0.,0.)) ;
#115146=DIRECTION('center_axis',(0.,1.,0.)) ;
#115147=DIRECTION('ref_axis',(0.,0.,1.)) ;
#115148=DIRECTION('center_axis',(0.,-1.,8.67361737988401E-15)) ;
#115149=DIRECTION('ref_axis',(0.,-8.67361737988401E-15,-1.)) ;
#115150=DIRECTION('center_axis',(0.,0.707106781186546,0.707106781186549)) ;
#115151=DIRECTION('ref_axis',(0.,-0.707106781186549,0.707106781186546)) ;
#115152=DIRECTION('center_axis',(0.,0.707106781186548,0.707106781186548)) ;
#115153=DIRECTION('ref_axis',(0.,-0.707106781186548,0.707106781186548)) ;
#115154=DIRECTION('center_axis',(0.,1.,1.07081696047951E-16)) ;
#115155=DIRECTION('ref_axis',(0.,-1.07081696047951E-16,1.)) ;
#115156=DIRECTION('center_axis',(0.,-1.,0.)) ;
#115157=DIRECTION('ref_axis',(0.,0.,-1.)) ;
#115158=DIRECTION('center_axis',(0.,1.,0.)) ;
#115159=DIRECTION('ref_axis',(0.,0.,1.)) ;
#115160=DIRECTION('center_axis',(0.,-8.67361737988409E-15,1.)) ;
#115161=DIRECTION('ref_axis',(0.,-1.,-8.67361737988409E-15)) ;
#115162=DIRECTION('center_axis',(0.,1.,0.)) ;
#115163=DIRECTION('ref_axis',(0.,0.,1.)) ;
#115164=DIRECTION('center_axis',(0.,8.67361737988403E-15,1.)) ;
#115165=DIRECTION('ref_axis',(0.,-1.,8.67361737988403E-15)) ;
#115166=DIRECTION('center_axis',(0.,3.99416362155027E-15,1.)) ;
#115167=DIRECTION('ref_axis',(0.,-1.,3.99416362155027E-15)) ;
#115168=DIRECTION('center_axis',(0.,0.,1.)) ;
#115169=DIRECTION('ref_axis',(1.,0.,0.)) ;
#115170=DIRECTION('center_axis',(0.,0.,-1.)) ;
#115171=DIRECTION('ref_axis',(-1.,0.,0.)) ;
#115172=DIRECTION('center_axis',(0.,0.,1.)) ;
#115173=DIRECTION('ref_axis',(1.,0.,0.)) ;
#115174=DIRECTION('center_axis',(-1.,0.,0.)) ;
#115175=DIRECTION('ref_axis',(0.,0.,1.)) ;
#115176=DIRECTION('center_axis',(0.,1.,0.)) ;
#115177=DIRECTION('ref_axis',(0.,0.,1.)) ;
#115178=DIRECTION('center_axis',(-1.,0.,0.)) ;
#115179=DIRECTION('ref_axis',(0.,0.,1.)) ;
#115180=DIRECTION('center_axis',(0.,-1.,0.)) ;
#115181=DIRECTION('ref_axis',(0.,0.,-1.)) ;
#115182=DIRECTION('center_axis',(0.,1.,0.)) ;
#115183=DIRECTION('ref_axis',(0.,0.,1.)) ;
#115184=DIRECTION('center_axis',(1.53063836115601E-16,-1.,-1.30104260698261E-16)) ;
#115185=DIRECTION('ref_axis',(1.,1.53063836115601E-16,1.99142572374599E-32)) ;
#115186=DIRECTION('center_axis',(0.,1.,0.)) ;
#115187=DIRECTION('ref_axis',(0.,0.,1.)) ;
#115188=DIRECTION('center_axis',(0.,-1.,0.)) ;
#115189=DIRECTION('ref_axis',(0.,0.,-1.)) ;
#115190=DIRECTION('center_axis',(1.,1.53063836115601E-16,2.73691106313441E-48)) ;
#115191=DIRECTION('ref_axis',(-1.53063836115601E-16,1.,-4.18922106430579E-64)) ;
#115192=DIRECTION('center_axis',(-1.,0.,0.)) ;
#115193=DIRECTION('ref_axis',(0.,0.,1.)) ;
#115194=DIRECTION('center_axis',(1.,1.53063836115601E-16,0.)) ;
#115195=DIRECTION('ref_axis',(1.53063836115601E-16,-1.,0.)) ;
#115196=DIRECTION('center_axis',(0.,1.,0.)) ;
#115197=DIRECTION('ref_axis',(1.,0.,0.)) ;
#115198=DIRECTION('center_axis',(0.,1.,0.)) ;
#115199=DIRECTION('ref_axis',(0.,0.,-1.)) ;
#115200=DIRECTION('center_axis',(0.,0.,1.)) ;
#115201=DIRECTION('ref_axis',(-1.,0.,0.)) ;
#115202=DIRECTION('center_axis',(0.,1.,0.)) ;
#115203=DIRECTION('ref_axis',(1.,0.,0.)) ;
#115204=DIRECTION('center_axis',(0.,0.,1.)) ;
#115205=DIRECTION('ref_axis',(-1.,0.,0.)) ;
#115206=DIRECTION('center_axis',(1.,1.0842021724855E-15,0.)) ;
#115207=DIRECTION('ref_axis',(1.0842021724855E-15,-1.,0.)) ;
#115208=DIRECTION('center_axis',(-1.,-1.53063836115601E-16,0.)) ;
#115209=DIRECTION('ref_axis',(0.,-1.,0.)) ;
#115210=DIRECTION('center_axis',(0.,0.,-1.)) ;
#115211=DIRECTION('ref_axis',(1.,0.,0.)) ;
#115212=DIRECTION('center_axis',(0.,0.,-1.)) ;
#115213=DIRECTION('ref_axis',(0.804034447892625,0.594582716366698,0.)) ;
#115214=DIRECTION('center_axis',(0.,0.,1.)) ;
#115215=DIRECTION('ref_axis',(1.,0.,0.)) ;
#115216=DIRECTION('',(0.,0.,-1.)) ;
#115217=DIRECTION('center_axis',(-2.16840434497101E-16,1.,1.30104260698261E-16)) ;
#115218=DIRECTION('ref_axis',(1.,2.16840434497101E-16,1.22464679914735E-16)) ;
#115219=DIRECTION('',(-2.16840434497101E-16,1.,1.30104260698261E-16)) ;
#115220=DIRECTION('center_axis',(0.,1.,0.)) ;
#115221=DIRECTION('ref_axis',(0.,0.,1.)) ;
#115222=DIRECTION('center_axis',(-1.,-1.53063836115601E-16,-2.73691106313441E-48)) ;
#115223=DIRECTION('ref_axis',(1.53063836115601E-16,-1.,4.18922106430579E-64)) ;
#115224=DIRECTION('center_axis',(1.,2.16840434497101E-16,0.)) ;
#115225=DIRECTION('ref_axis',(2.16840434497101E-16,-1.,0.)) ;
#115226=DIRECTION('center_axis',(0.,0.,1.)) ;
#115227=DIRECTION('ref_axis',(1.,0.,0.)) ;
#115228=DIRECTION('center_axis',(-1.25542992828747E-32,1.020425574104E-16,
1.)) ;
#115229=DIRECTION('ref_axis',(-1.28107280532009E-48,-1.,1.020425574104E-16)) ;
#115230=DIRECTION('center_axis',(0.,0.,1.)) ;
#115231=DIRECTION('ref_axis',(1.,0.,0.)) ;
#115232=DIRECTION('center_axis',(0.,0.,-1.)) ;
#115233=DIRECTION('ref_axis',(-1.,0.,0.)) ;
#115234=DIRECTION('center_axis',(1.,1.53063836115601E-16,-2.73691106313441E-48)) ;
#115235=DIRECTION('ref_axis',(-1.53063836115601E-16,1.,4.18922106430579E-64)) ;
#115236=DIRECTION('center_axis',(-1.,0.,0.)) ;
#115237=DIRECTION('ref_axis',(0.,0.,1.)) ;
#115238=DIRECTION('center_axis',(1.,1.53063836115601E-16,0.)) ;
#115239=DIRECTION('ref_axis',(1.53063836115601E-16,-1.,0.)) ;
#115240=DIRECTION('center_axis',(0.,1.,0.)) ;
#115241=DIRECTION('ref_axis',(1.,0.,0.)) ;
#115242=DIRECTION('center_axis',(-1.,-2.16840434497101E-16,0.)) ;
#115243=DIRECTION('ref_axis',(0.,-1.,0.)) ;
#115244=DIRECTION('center_axis',(0.,0.,-1.)) ;
#115245=DIRECTION('ref_axis',(1.,0.,0.)) ;
#115246=DIRECTION('center_axis',(-1.25542992828747E-32,1.020425574104E-16,
1.)) ;
#115247=DIRECTION('ref_axis',(0.,-1.,0.)) ;
#115248=DIRECTION('center_axis',(0.,-1.,0.)) ;
#115249=DIRECTION('ref_axis',(-6.50521303491307E-15,0.,1.)) ;
#115250=DIRECTION('center_axis',(-1.,0.,0.)) ;
#115251=DIRECTION('ref_axis',(0.,0.,-1.)) ;
#115252=DIRECTION('center_axis',(-1.,-1.53063836115601E-16,0.)) ;
#115253=DIRECTION('ref_axis',(0.,-1.,0.)) ;
#115254=DIRECTION('center_axis',(0.,-1.,0.)) ;
#115255=DIRECTION('ref_axis',(0.,0.,1.)) ;
#115256=DIRECTION('center_axis',(0.,0.,-1.)) ;
#115257=DIRECTION('ref_axis',(-1.,0.,0.)) ;
#115258=DIRECTION('center_axis',(0.,0.,-1.)) ;
#115259=DIRECTION('ref_axis',(-1.,0.,0.)) ;
#115260=DIRECTION('center_axis',(1.,1.53063836115601E-16,-3.06472600140763E-33)) ;
#115261=DIRECTION('ref_axis',(-1.53063836115601E-16,1.,4.69098718418678E-49)) ;
#115262=DIRECTION('center_axis',(-1.,0.,0.)) ;
#115263=DIRECTION('ref_axis',(0.,0.,1.)) ;
#115264=DIRECTION('center_axis',(-1.53063836115601E-16,1.,-1.020425574104E-16)) ;
#115265=DIRECTION('ref_axis',(-1.,-1.53063836115601E-16,1.3684555315672E-47)) ;
#115266=DIRECTION('',(1.53063836115601E-16,-1.,1.020425574104E-16)) ;
#115267=DIRECTION('center_axis',(0.,-1.,0.)) ;
#115268=DIRECTION('ref_axis',(0.,0.,-1.)) ;
#115269=DIRECTION('center_axis',(-1.53063836115601E-16,1.,-1.30104260698261E-16)) ;
#115270=DIRECTION('ref_axis',(-1.,-1.53063836115601E-16,1.99142572374599E-32)) ;
#115271=DIRECTION('center_axis',(0.,-1.,0.)) ;
#115272=DIRECTION('ref_axis',(0.,0.,-1.)) ;
#115273=DIRECTION('center_axis',(-1.,-1.53063836115601E-16,2.73691106313441E-48)) ;
#115274=DIRECTION('ref_axis',(1.53063836115601E-16,-1.,-4.18922106430579E-64)) ;
#115275=DIRECTION('center_axis',(1.,2.16840434497101E-16,0.)) ;
#115276=DIRECTION('ref_axis',(2.16840434497101E-16,-1.,0.)) ;
#115277=DIRECTION('center_axis',(-1.,0.,2.16840434497102E-15)) ;
#115278=DIRECTION('ref_axis',(2.16840434497102E-15,0.,1.)) ;
#115279=DIRECTION('center_axis',(-1.,-2.16840434497101E-16,0.)) ;
#115280=DIRECTION('ref_axis',(0.,-1.,0.)) ;
#115281=DIRECTION('center_axis',(0.,0.,1.)) ;
#115282=DIRECTION('ref_axis',(-1.,0.,0.)) ;
#115283=DIRECTION('center_axis',(0.,1.,0.)) ;
#115284=DIRECTION('ref_axis',(1.,0.,0.)) ;
#115285=DIRECTION('center_axis',(0.,1.,0.)) ;
#115286=DIRECTION('ref_axis',(0.,0.,-1.)) ;
#115287=DIRECTION('center_axis',(1.,0.,0.)) ;
#115288=DIRECTION('ref_axis',(0.,-1.,0.)) ;
#115289=DIRECTION('center_axis',(1.,6.50521303491304E-15,0.)) ;
#115290=DIRECTION('ref_axis',(-6.50521303491304E-15,1.,0.)) ;
#115291=DIRECTION('center_axis',(8.67361737988403E-15,1.,0.)) ;
#115292=DIRECTION('ref_axis',(-1.,8.67361737988403E-15,0.)) ;
#115293=DIRECTION('center_axis',(1.2303003375722E-16,-1.,1.020425574104E-16)) ;
#115294=DIRECTION('ref_axis',(1.,1.2303003375722E-16,-1.25542992828747E-32)) ;
#115295=DIRECTION('center_axis',(0.,1.,0.)) ;
#115296=DIRECTION('ref_axis',(0.,0.,1.)) ;
#115297=DIRECTION('center_axis',(0.,1.,0.)) ;
#115298=DIRECTION('ref_axis',(1.,0.,0.)) ;
#115299=DIRECTION('center_axis',(1.,1.2303003375722E-16,0.)) ;
#115300=DIRECTION('ref_axis',(1.2303003375722E-16,-1.,0.)) ;
#115301=DIRECTION('center_axis',(0.,0.,1.)) ;
#115302=DIRECTION('ref_axis',(-1.,0.,0.)) ;
#115303=DIRECTION('center_axis',(0.,1.,0.)) ;
#115304=DIRECTION('ref_axis',(1.,0.,0.)) ;
#115305=DIRECTION('center_axis',(0.,0.,-1.)) ;
#115306=DIRECTION('ref_axis',(1.,0.,0.)) ;
#115307=DIRECTION('center_axis',(0.,0.,-1.)) ;
#115308=DIRECTION('ref_axis',(-1.,0.,0.)) ;
#115309=DIRECTION('center_axis',(0.,0.,1.)) ;
#115310=DIRECTION('ref_axis',(1.,0.,0.)) ;
#115311=DIRECTION('center_axis',(-2.16840434497101E-16,1.,-1.020425574104E-16)) ;
#115312=DIRECTION('ref_axis',(-1.,-2.16840434497101E-16,5.47382212626882E-48)) ;
#115313=DIRECTION('center_axis',(0.,1.,0.)) ;
#115314=DIRECTION('ref_axis',(0.,0.,-1.)) ;
#115315=DIRECTION('center_axis',(1.,0.,1.25542992828747E-32)) ;
#115316=DIRECTION('ref_axis',(1.25542992828747E-32,0.,-1.)) ;
#115317=DIRECTION('center_axis',(1.,0.,0.)) ;
#115318=DIRECTION('ref_axis',(0.,0.,-1.)) ;
#115319=DIRECTION('center_axis',(-1.,-1.2303003375722E-16,0.)) ;
#115320=DIRECTION('ref_axis',(0.,-1.,0.)) ;
#115321=DIRECTION('center_axis',(0.,0.,-1.)) ;
#115322=DIRECTION('ref_axis',(1.,0.,0.)) ;
#115323=DIRECTION('center_axis',(0.,0.,-1.)) ;
#115324=DIRECTION('ref_axis',(-1.,0.,0.)) ;
#115325=DIRECTION('',(0.,0.,1.)) ;
#115326=DIRECTION('center_axis',(0.,0.,1.)) ;
#115327=DIRECTION('ref_axis',(1.,0.,0.)) ;
#115328=DIRECTION('center_axis',(0.,0.,1.)) ;
#115329=DIRECTION('ref_axis',(1.,0.,0.)) ;
#115330=DIRECTION('center_axis',(6.27714964143733E-33,-5.10212787052002E-17,
-1.)) ;
#115331=DIRECTION('ref_axis',(3.20268201330022E-49,1.,-5.10212787052002E-17)) ;
#115332=DIRECTION('center_axis',(1.,1.53063836115601E-16,-1.53236300070382E-33)) ;
#115333=DIRECTION('ref_axis',(-1.53063836115601E-16,1.,2.34549359209339E-49)) ;
#115334=DIRECTION('center_axis',(-1.,0.,0.)) ;
#115335=DIRECTION('ref_axis',(0.,0.,1.)) ;
#115336=DIRECTION('center_axis',(1.,0.,0.)) ;
#115337=DIRECTION('ref_axis',(0.,0.,-1.)) ;
#115338=DIRECTION('center_axis',(0.,1.,0.)) ;
#115339=DIRECTION('ref_axis',(1.,0.,0.)) ;
#115340=DIRECTION('center_axis',(-4.33680868994202E-15,1.,0.)) ;
#115341=DIRECTION('ref_axis',(1.,4.33680868994202E-15,0.)) ;
#115342=DIRECTION('center_axis',(0.,-1.,0.)) ;
#115343=DIRECTION('ref_axis',(0.,0.,-1.)) ;
#115344=DIRECTION('center_axis',(0.,0.,-1.)) ;
#115345=DIRECTION('ref_axis',(1.,0.,0.)) ;
#115346=DIRECTION('center_axis',(0.,0.,1.)) ;
#115347=DIRECTION('ref_axis',(1.,0.,0.)) ;
#115348=DIRECTION('center_axis',(0.,0.,-1.)) ;
#115349=DIRECTION('ref_axis',(-1.,0.,0.)) ;
#115350=DIRECTION('center_axis',(0.,1.,0.)) ;
#115351=DIRECTION('ref_axis',(1.,0.,0.)) ;
#115352=DIRECTION('center_axis',(1.,1.2303003375722E-16,0.)) ;
#115353=DIRECTION('ref_axis',(1.2303003375722E-16,-1.,0.)) ;
#115354=DIRECTION('center_axis',(0.,1.,0.)) ;
#115355=DIRECTION('ref_axis',(-6.50521303491307E-15,0.,-1.)) ;
#115356=DIRECTION('center_axis',(6.27714964143733E-33,-5.10212787052002E-17,
-1.)) ;
#115357=DIRECTION('ref_axis',(0.,1.,0.)) ;
#115358=DIRECTION('center_axis',(0.,-1.,0.)) ;
#115359=DIRECTION('ref_axis',(0.,0.,1.)) ;
#115360=DIRECTION('center_axis',(2.16840434497101E-16,-1.,5.10212787052002E-17)) ;
#115361=DIRECTION('ref_axis',(1.,2.16840434497101E-16,-5.47382212626882E-48)) ;
#115362=DIRECTION('center_axis',(0.,1.,0.)) ;
#115363=DIRECTION('ref_axis',(0.,0.,-1.)) ;
#115364=DIRECTION('center_axis',(0.,0.,1.)) ;
#115365=DIRECTION('ref_axis',(1.,0.,0.)) ;
#115366=DIRECTION('center_axis',(0.,0.,-1.)) ;
#115367=DIRECTION('ref_axis',(-1.,0.,0.)) ;
#115368=DIRECTION('center_axis',(-1.,-1.2303003375722E-16,0.)) ;
#115369=DIRECTION('ref_axis',(0.,-1.,0.)) ;
#115370=DIRECTION('center_axis',(0.,-1.,0.)) ;
#115371=DIRECTION('ref_axis',(0.,0.,1.)) ;
#115372=DIRECTION('center_axis',(1.53063836115601E-16,-1.,5.10212787052002E-17)) ;
#115373=DIRECTION('ref_axis',(1.,1.53063836115601E-16,-6.84227765783602E-48)) ;
#115374=DIRECTION('',(-1.53063836115601E-16,1.,-5.10212787052002E-17)) ;
#115375=DIRECTION('center_axis',(0.,-1.,0.)) ;
#115376=DIRECTION('ref_axis',(0.,0.,-1.)) ;
#115377=DIRECTION('center_axis',(-1.,0.,0.)) ;
#115378=DIRECTION('ref_axis',(0.,0.,-1.)) ;
#115379=DIRECTION('center_axis',(-1.2303003375722E-16,1.,-5.10212787052002E-17)) ;
#115380=DIRECTION('ref_axis',(-1.,-1.2303003375722E-16,6.27714964143733E-33)) ;
#115381=DIRECTION('center_axis',(-8.67361737988403E-15,-1.,0.)) ;
#115382=DIRECTION('ref_axis',(1.,-8.67361737988403E-15,0.)) ;
#115383=DIRECTION('center_axis',(1.,0.,6.27714964143733E-33)) ;
#115384=DIRECTION('ref_axis',(6.27714964143733E-33,0.,-1.)) ;
#115385=DIRECTION('center_axis',(-1.,0.,-6.50521303491307E-15)) ;
#115386=DIRECTION('ref_axis',(-6.50521303491307E-15,0.,1.)) ;
#115387=DIRECTION('center_axis',(1.,0.,0.)) ;
#115388=DIRECTION('ref_axis',(0.,1.,0.)) ;
#115389=DIRECTION('center_axis',(0.,0.,-1.)) ;
#115390=DIRECTION('ref_axis',(-1.,0.,0.)) ;
#115391=DIRECTION('center_axis',(0.,0.,1.)) ;
#115392=DIRECTION('ref_axis',(1.,0.,0.)) ;
#115393=DIRECTION('center_axis',(0.,0.,-1.)) ;
#115394=DIRECTION('ref_axis',(-1.,0.,0.)) ;
#115395=DIRECTION('center_axis',(-1.,0.,0.)) ;
#115396=DIRECTION('ref_axis',(0.,0.,1.)) ;
#115397=DIRECTION('center_axis',(0.,-1.,0.)) ;
#115398=DIRECTION('ref_axis',(0.,0.,-1.)) ;
#115399=DIRECTION('center_axis',(0.,1.,0.)) ;
#115400=DIRECTION('ref_axis',(0.,0.,1.)) ;
#115401=DIRECTION('center_axis',(0.,1.,-6.50521303491307E-15)) ;
#115402=DIRECTION('ref_axis',(0.,6.50521303491307E-15,1.)) ;
#115403=DIRECTION('center_axis',(0.,-1.,0.)) ;
#115404=DIRECTION('ref_axis',(0.,0.,-1.)) ;
#115405=DIRECTION('center_axis',(0.,-1.,0.)) ;
#115406=DIRECTION('ref_axis',(0.,0.,-1.)) ;
#115407=DIRECTION('center_axis',(0.,-1.,-1.07081696047951E-16)) ;
#115408=DIRECTION('ref_axis',(0.,1.07081696047951E-16,-1.)) ;
#115409=DIRECTION('center_axis',(0.,1.,0.)) ;
#115410=DIRECTION('ref_axis',(0.,0.,1.)) ;
#115411=DIRECTION('center_axis',(-1.,0.,0.)) ;
#115412=DIRECTION('ref_axis',(0.,0.,1.)) ;
#115413=DIRECTION('center_axis',(0.,0.,1.)) ;
#115414=DIRECTION('ref_axis',(1.,0.,0.)) ;
#115415=DIRECTION('center_axis',(0.,1.,0.)) ;
#115416=DIRECTION('ref_axis',(0.,0.,1.)) ;
#115417=DIRECTION('center_axis',(0.,-1.73472347597681E-14,-1.)) ;
#115418=DIRECTION('ref_axis',(0.,1.,-1.73472347597681E-14)) ;
#115419=DIRECTION('center_axis',(0.,0.,1.)) ;
#115420=DIRECTION('ref_axis',(1.,0.,0.)) ;
#115421=DIRECTION('center_axis',(0.,0.,1.)) ;
#115422=DIRECTION('ref_axis',(1.,0.,0.)) ;
#115423=DIRECTION('center_axis',(0.,0.,1.)) ;
#115424=DIRECTION('ref_axis',(1.,0.,0.)) ;
#115425=DIRECTION('center_axis',(0.,0.,-1.)) ;
#115426=DIRECTION('ref_axis',(-1.,0.,0.)) ;
#115427=DIRECTION('center_axis',(0.,1.,0.)) ;
#115428=DIRECTION('ref_axis',(0.,0.,1.)) ;
#115429=DIRECTION('center_axis',(0.,-0.707106781186545,0.70710678118655)) ;
#115430=DIRECTION('ref_axis',(0.,-0.70710678118655,-0.707106781186545)) ;
#115431=DIRECTION('center_axis',(0.,1.,0.)) ;
#115432=DIRECTION('ref_axis',(0.,0.,1.)) ;
#115433=DIRECTION('center_axis',(0.,-0.514231796959109,-0.857651245551597)) ;
#115434=DIRECTION('ref_axis',(0.,0.857651245551597,-0.514231796959109)) ;
#115435=DIRECTION('center_axis',(0.,-0.707106781186548,0.707106781186547)) ;
#115436=DIRECTION('ref_axis',(0.,-0.707106781186547,-0.707106781186548)) ;
#115437=DIRECTION('center_axis',(0.,-0.707106781186548,0.707106781186548)) ;
#115438=DIRECTION('ref_axis',(0.,-0.707106781186548,-0.707106781186548)) ;
#115439=DIRECTION('center_axis',(-1.,0.,0.)) ;
#115440=DIRECTION('ref_axis',(0.,0.,1.)) ;
#115441=DIRECTION('center_axis',(-2.23012492569676E-15,0.514231796959107,
-0.857651245551598)) ;
#115442=DIRECTION('ref_axis',(-5.69910941180089E-30,0.857651245551598,0.514231796959107)) ;
#115443=DIRECTION('center_axis',(0.,1.,0.)) ;
#115444=DIRECTION('ref_axis',(0.,0.,1.)) ;
#115445=DIRECTION('center_axis',(0.,0.,-1.)) ;
#115446=DIRECTION('ref_axis',(-1.,0.,0.)) ;
#115447=DIRECTION('center_axis',(0.,1.,0.)) ;
#115448=DIRECTION('ref_axis',(0.,0.,1.)) ;
#115449=DIRECTION('center_axis',(0.,0.,-1.)) ;
#115450=DIRECTION('ref_axis',(-1.,0.,0.)) ;
#115451=DIRECTION('center_axis',(0.,0.,-1.)) ;
#115452=DIRECTION('ref_axis',(-1.,0.,0.)) ;
#115453=DIRECTION('center_axis',(0.,0.,1.)) ;
#115454=DIRECTION('ref_axis',(1.,0.,0.)) ;
#115455=DIRECTION('center_axis',(0.,0.,-1.)) ;
#115456=DIRECTION('ref_axis',(-1.,0.,0.)) ;
#115457=DIRECTION('center_axis',(0.,1.,0.)) ;
#115458=DIRECTION('ref_axis',(0.,0.,1.)) ;
#115459=DIRECTION('center_axis',(0.,-1.,8.67361737988409E-15)) ;
#115460=DIRECTION('ref_axis',(0.,-8.67361737988409E-15,-1.)) ;
#115461=DIRECTION('center_axis',(0.,0.707106781186546,0.707106781186549)) ;
#115462=DIRECTION('ref_axis',(0.,-0.707106781186549,0.707106781186546)) ;
#115463=DIRECTION('center_axis',(0.,0.707106781186541,0.707106781186554)) ;
#115464=DIRECTION('ref_axis',(0.,-0.707106781186554,0.707106781186541)) ;
#115465=DIRECTION('center_axis',(0.,1.,1.07081696047951E-16)) ;
#115466=DIRECTION('ref_axis',(0.,-1.07081696047951E-16,1.)) ;
#115467=DIRECTION('center_axis',(0.,-1.,0.)) ;
#115468=DIRECTION('ref_axis',(0.,0.,-1.)) ;
#115469=DIRECTION('center_axis',(0.,1.,0.)) ;
#115470=DIRECTION('ref_axis',(0.,0.,1.)) ;
#115471=DIRECTION('center_axis',(0.,0.,1.)) ;
#115472=DIRECTION('ref_axis',(1.,0.,0.)) ;
#115473=DIRECTION('center_axis',(0.,1.,0.)) ;
#115474=DIRECTION('ref_axis',(0.,0.,1.)) ;
#115475=DIRECTION('center_axis',(0.,0.,1.)) ;
#115476=DIRECTION('ref_axis',(1.,0.,0.)) ;
#115477=DIRECTION('center_axis',(0.,3.99416362155027E-15,1.)) ;
#115478=DIRECTION('ref_axis',(0.,-1.,3.99416362155027E-15)) ;
#115479=DIRECTION('center_axis',(0.,0.,1.)) ;
#115480=DIRECTION('ref_axis',(1.,0.,0.)) ;
#115481=DIRECTION('center_axis',(0.,0.,-1.)) ;
#115482=DIRECTION('ref_axis',(-1.,0.,0.)) ;
#115483=DIRECTION('center_axis',(0.,0.,1.)) ;
#115484=DIRECTION('ref_axis',(1.,0.,0.)) ;
#115485=DIRECTION('center_axis',(-1.,0.,0.)) ;
#115486=DIRECTION('ref_axis',(0.,0.,1.)) ;
#115487=DIRECTION('center_axis',(0.,1.,0.)) ;
#115488=DIRECTION('ref_axis',(0.,0.,1.)) ;
#115489=DIRECTION('center_axis',(-1.,0.,0.)) ;
#115490=DIRECTION('ref_axis',(0.,0.,1.)) ;
#115491=DIRECTION('center_axis',(0.,-1.,0.)) ;
#115492=DIRECTION('ref_axis',(0.,0.,-1.)) ;
#115493=DIRECTION('center_axis',(0.,1.,0.)) ;
#115494=DIRECTION('ref_axis',(0.,0.,1.)) ;
#115495=DIRECTION('center_axis',(1.53063836115601E-16,-1.,-1.30104260698261E-16)) ;
#115496=DIRECTION('ref_axis',(1.,1.53063836115601E-16,1.99142572374599E-32)) ;
#115497=DIRECTION('center_axis',(0.,1.,0.)) ;
#115498=DIRECTION('ref_axis',(0.,0.,1.)) ;
#115499=DIRECTION('center_axis',(0.,-1.,0.)) ;
#115500=DIRECTION('ref_axis',(0.,0.,-1.)) ;
#115501=DIRECTION('center_axis',(1.,1.53063836115601E-16,2.73691106313441E-48)) ;
#115502=DIRECTION('ref_axis',(-1.53063836115601E-16,1.,-4.18922106430579E-64)) ;
#115503=DIRECTION('center_axis',(-1.,0.,0.)) ;
#115504=DIRECTION('ref_axis',(0.,0.,1.)) ;
#115505=DIRECTION('center_axis',(1.,1.53063836115601E-16,0.)) ;
#115506=DIRECTION('ref_axis',(1.53063836115601E-16,-1.,0.)) ;
#115507=DIRECTION('center_axis',(0.,1.,0.)) ;
#115508=DIRECTION('ref_axis',(1.,0.,0.)) ;
#115509=DIRECTION('center_axis',(0.,1.,0.)) ;
#115510=DIRECTION('ref_axis',(0.,0.,-1.)) ;
#115511=DIRECTION('center_axis',(0.,0.,1.)) ;
#115512=DIRECTION('ref_axis',(-1.,0.,0.)) ;
#115513=DIRECTION('center_axis',(0.,1.,0.)) ;
#115514=DIRECTION('ref_axis',(1.,0.,0.)) ;
#115515=DIRECTION('center_axis',(0.,0.,1.)) ;
#115516=DIRECTION('ref_axis',(-1.,0.,0.)) ;
#115517=DIRECTION('center_axis',(1.,1.0842021724855E-15,0.)) ;
#115518=DIRECTION('ref_axis',(1.0842021724855E-15,-1.,0.)) ;
#115519=DIRECTION('center_axis',(-1.,-1.53063836115601E-16,0.)) ;
#115520=DIRECTION('ref_axis',(0.,-1.,0.)) ;
#115521=DIRECTION('center_axis',(0.,0.,-1.)) ;
#115522=DIRECTION('ref_axis',(1.,0.,0.)) ;
#115523=DIRECTION('center_axis',(0.,0.,-1.)) ;
#115524=DIRECTION('ref_axis',(0.804034447892618,0.594582716366708,0.)) ;
#115525=DIRECTION('center_axis',(0.,0.,1.)) ;
#115526=DIRECTION('ref_axis',(1.,0.,0.)) ;
#115527=DIRECTION('',(0.,0.,-1.)) ;
#115528=DIRECTION('center_axis',(-2.16840434497101E-16,1.,1.30104260698261E-16)) ;
#115529=DIRECTION('ref_axis',(1.,2.16840434497101E-16,1.22464679914735E-16)) ;
#115530=DIRECTION('',(-2.16840434497101E-16,1.,1.30104260698261E-16)) ;
#115531=DIRECTION('center_axis',(0.,1.,0.)) ;
#115532=DIRECTION('ref_axis',(0.,0.,1.)) ;
#115533=DIRECTION('center_axis',(-1.,-1.53063836115601E-16,-2.73691106313441E-48)) ;
#115534=DIRECTION('ref_axis',(1.53063836115601E-16,-1.,4.18922106430579E-64)) ;
#115535=DIRECTION('center_axis',(1.,2.16840434497101E-16,0.)) ;
#115536=DIRECTION('ref_axis',(2.16840434497101E-16,-1.,0.)) ;
#115537=DIRECTION('center_axis',(0.,0.,1.)) ;
#115538=DIRECTION('ref_axis',(1.,0.,0.)) ;
#115539=DIRECTION('center_axis',(-1.25542992828747E-32,1.020425574104E-16,
1.)) ;
#115540=DIRECTION('ref_axis',(-1.28107280532009E-48,-1.,1.020425574104E-16)) ;
#115541=DIRECTION('center_axis',(0.,0.,1.)) ;
#115542=DIRECTION('ref_axis',(1.,0.,0.)) ;
#115543=DIRECTION('center_axis',(0.,0.,-1.)) ;
#115544=DIRECTION('ref_axis',(-1.,0.,0.)) ;
#115545=DIRECTION('center_axis',(1.,1.53063836115601E-16,-2.73691106313441E-48)) ;
#115546=DIRECTION('ref_axis',(-1.53063836115601E-16,1.,4.18922106430579E-64)) ;
#115547=DIRECTION('center_axis',(-1.,0.,0.)) ;
#115548=DIRECTION('ref_axis',(0.,0.,1.)) ;
#115549=DIRECTION('center_axis',(1.,1.53063836115601E-16,0.)) ;
#115550=DIRECTION('ref_axis',(1.53063836115601E-16,-1.,0.)) ;
#115551=DIRECTION('center_axis',(0.,1.,0.)) ;
#115552=DIRECTION('ref_axis',(1.,0.,0.)) ;
#115553=DIRECTION('center_axis',(-1.,-2.16840434497101E-16,0.)) ;
#115554=DIRECTION('ref_axis',(0.,-1.,0.)) ;
#115555=DIRECTION('center_axis',(0.,0.,-1.)) ;
#115556=DIRECTION('ref_axis',(1.,0.,0.)) ;
#115557=DIRECTION('center_axis',(-1.25542992828747E-32,1.020425574104E-16,
1.)) ;
#115558=DIRECTION('ref_axis',(0.,-1.,0.)) ;
#115559=DIRECTION('center_axis',(0.,-1.,0.)) ;
#115560=DIRECTION('ref_axis',(-6.50521303491307E-15,0.,1.)) ;
#115561=DIRECTION('center_axis',(-1.,0.,0.)) ;
#115562=DIRECTION('ref_axis',(0.,0.,-1.)) ;
#115563=DIRECTION('center_axis',(-1.,-1.53063836115601E-16,0.)) ;
#115564=DIRECTION('ref_axis',(0.,-1.,0.)) ;
#115565=DIRECTION('center_axis',(0.,-1.,0.)) ;
#115566=DIRECTION('ref_axis',(0.,0.,1.)) ;
#115567=DIRECTION('center_axis',(0.,0.,-1.)) ;
#115568=DIRECTION('ref_axis',(-1.,0.,0.)) ;
#115569=DIRECTION('center_axis',(0.,0.,-1.)) ;
#115570=DIRECTION('ref_axis',(-1.,0.,0.)) ;
#115571=DIRECTION('center_axis',(1.,1.53063836115601E-16,-3.06472600140763E-33)) ;
#115572=DIRECTION('ref_axis',(-1.53063836115601E-16,1.,4.69098718418678E-49)) ;
#115573=DIRECTION('center_axis',(-1.,0.,0.)) ;
#115574=DIRECTION('ref_axis',(0.,0.,1.)) ;
#115575=DIRECTION('center_axis',(-1.53063836115601E-16,1.,-1.020425574104E-16)) ;
#115576=DIRECTION('ref_axis',(-1.,-1.53063836115601E-16,1.3684555315672E-47)) ;
#115577=DIRECTION('',(1.53063836115601E-16,-1.,1.020425574104E-16)) ;
#115578=DIRECTION('center_axis',(0.,-1.,0.)) ;
#115579=DIRECTION('ref_axis',(0.,0.,-1.)) ;
#115580=DIRECTION('center_axis',(-1.53063836115601E-16,1.,-1.30104260698261E-16)) ;
#115581=DIRECTION('ref_axis',(-1.,-1.53063836115601E-16,1.99142572374599E-32)) ;
#115582=DIRECTION('center_axis',(0.,-1.,0.)) ;
#115583=DIRECTION('ref_axis',(0.,0.,-1.)) ;
#115584=DIRECTION('center_axis',(-1.,-1.53063836115601E-16,2.73691106313441E-48)) ;
#115585=DIRECTION('ref_axis',(1.53063836115601E-16,-1.,-4.18922106430579E-64)) ;
#115586=DIRECTION('center_axis',(1.,2.16840434497101E-16,0.)) ;
#115587=DIRECTION('ref_axis',(2.16840434497101E-16,-1.,0.)) ;
#115588=DIRECTION('center_axis',(-1.,0.,2.16840434497102E-15)) ;
#115589=DIRECTION('ref_axis',(2.16840434497102E-15,0.,1.)) ;
#115590=DIRECTION('center_axis',(-1.,-2.16840434497101E-16,0.)) ;
#115591=DIRECTION('ref_axis',(0.,-1.,0.)) ;
#115592=DIRECTION('center_axis',(0.,0.,1.)) ;
#115593=DIRECTION('ref_axis',(-1.,0.,0.)) ;
#115594=DIRECTION('center_axis',(0.,1.,0.)) ;
#115595=DIRECTION('ref_axis',(1.,0.,0.)) ;
#115596=DIRECTION('center_axis',(0.,1.,0.)) ;
#115597=DIRECTION('ref_axis',(0.,0.,-1.)) ;
#115598=DIRECTION('center_axis',(1.,0.,0.)) ;
#115599=DIRECTION('ref_axis',(0.,-1.,0.)) ;
#115600=DIRECTION('center_axis',(1.,6.50521303491304E-15,0.)) ;
#115601=DIRECTION('ref_axis',(-6.50521303491304E-15,1.,0.)) ;
#115602=DIRECTION('center_axis',(8.67361737988403E-15,1.,0.)) ;
#115603=DIRECTION('ref_axis',(-1.,8.67361737988403E-15,0.)) ;
#115604=DIRECTION('center_axis',(1.2303003375722E-16,-1.,1.020425574104E-16)) ;
#115605=DIRECTION('ref_axis',(1.,1.2303003375722E-16,-1.25542992828747E-32)) ;
#115606=DIRECTION('center_axis',(0.,1.,0.)) ;
#115607=DIRECTION('ref_axis',(0.,0.,1.)) ;
#115608=DIRECTION('center_axis',(0.,1.,0.)) ;
#115609=DIRECTION('ref_axis',(1.,0.,0.)) ;
#115610=DIRECTION('center_axis',(1.,1.2303003375722E-16,0.)) ;
#115611=DIRECTION('ref_axis',(1.2303003375722E-16,-1.,0.)) ;
#115612=DIRECTION('center_axis',(0.,0.,1.)) ;
#115613=DIRECTION('ref_axis',(-1.,0.,0.)) ;
#115614=DIRECTION('center_axis',(0.,1.,0.)) ;
#115615=DIRECTION('ref_axis',(1.,0.,0.)) ;
#115616=DIRECTION('center_axis',(0.,0.,-1.)) ;
#115617=DIRECTION('ref_axis',(1.,0.,0.)) ;
#115618=DIRECTION('center_axis',(0.,0.,-1.)) ;
#115619=DIRECTION('ref_axis',(-1.,0.,0.)) ;
#115620=DIRECTION('center_axis',(0.,0.,1.)) ;
#115621=DIRECTION('ref_axis',(1.,0.,0.)) ;
#115622=DIRECTION('center_axis',(-2.16840434497101E-16,1.,-1.020425574104E-16)) ;
#115623=DIRECTION('ref_axis',(-1.,-2.16840434497101E-16,5.47382212626882E-48)) ;
#115624=DIRECTION('center_axis',(0.,1.,0.)) ;
#115625=DIRECTION('ref_axis',(0.,0.,-1.)) ;
#115626=DIRECTION('center_axis',(1.,0.,1.25542992828747E-32)) ;
#115627=DIRECTION('ref_axis',(1.25542992828747E-32,0.,-1.)) ;
#115628=DIRECTION('center_axis',(1.,0.,0.)) ;
#115629=DIRECTION('ref_axis',(0.,0.,-1.)) ;
#115630=DIRECTION('center_axis',(-1.,-1.2303003375722E-16,0.)) ;
#115631=DIRECTION('ref_axis',(0.,-1.,0.)) ;
#115632=DIRECTION('center_axis',(0.,0.,-1.)) ;
#115633=DIRECTION('ref_axis',(1.,0.,0.)) ;
#115634=DIRECTION('center_axis',(0.,0.,-1.)) ;
#115635=DIRECTION('ref_axis',(-1.,0.,0.)) ;
#115636=DIRECTION('',(0.,0.,1.)) ;
#115637=DIRECTION('center_axis',(0.,0.,1.)) ;
#115638=DIRECTION('ref_axis',(1.,0.,0.)) ;
#115639=DIRECTION('center_axis',(0.,0.,1.)) ;
#115640=DIRECTION('ref_axis',(1.,0.,0.)) ;
#115641=DIRECTION('center_axis',(6.27714964143733E-33,-5.10212787052002E-17,
-1.)) ;
#115642=DIRECTION('ref_axis',(3.20268201330022E-49,1.,-5.10212787052002E-17)) ;
#115643=DIRECTION('center_axis',(1.,1.53063836115601E-16,-1.53236300070382E-33)) ;
#115644=DIRECTION('ref_axis',(-1.53063836115601E-16,1.,2.34549359209339E-49)) ;
#115645=DIRECTION('center_axis',(-1.,0.,0.)) ;
#115646=DIRECTION('ref_axis',(0.,0.,1.)) ;
#115647=DIRECTION('center_axis',(1.,0.,0.)) ;
#115648=DIRECTION('ref_axis',(0.,0.,-1.)) ;
#115649=DIRECTION('center_axis',(0.,1.,0.)) ;
#115650=DIRECTION('ref_axis',(1.,0.,0.)) ;
#115651=DIRECTION('center_axis',(-4.33680868994202E-15,1.,0.)) ;
#115652=DIRECTION('ref_axis',(1.,4.33680868994202E-15,0.)) ;
#115653=DIRECTION('center_axis',(0.,-1.,0.)) ;
#115654=DIRECTION('ref_axis',(0.,0.,-1.)) ;
#115655=DIRECTION('center_axis',(0.,0.,-1.)) ;
#115656=DIRECTION('ref_axis',(1.,0.,0.)) ;
#115657=DIRECTION('center_axis',(0.,0.,1.)) ;
#115658=DIRECTION('ref_axis',(1.,0.,0.)) ;
#115659=DIRECTION('center_axis',(0.,0.,-1.)) ;
#115660=DIRECTION('ref_axis',(-1.,0.,0.)) ;
#115661=DIRECTION('center_axis',(0.,1.,0.)) ;
#115662=DIRECTION('ref_axis',(1.,0.,0.)) ;
#115663=DIRECTION('center_axis',(1.,1.2303003375722E-16,0.)) ;
#115664=DIRECTION('ref_axis',(1.2303003375722E-16,-1.,0.)) ;
#115665=DIRECTION('center_axis',(0.,1.,0.)) ;
#115666=DIRECTION('ref_axis',(-6.50521303491307E-15,0.,-1.)) ;
#115667=DIRECTION('center_axis',(6.27714964143733E-33,-5.10212787052002E-17,
-1.)) ;
#115668=DIRECTION('ref_axis',(0.,1.,0.)) ;
#115669=DIRECTION('center_axis',(0.,-1.,0.)) ;
#115670=DIRECTION('ref_axis',(0.,0.,1.)) ;
#115671=DIRECTION('center_axis',(2.16840434497101E-16,-1.,5.10212787052002E-17)) ;
#115672=DIRECTION('ref_axis',(1.,2.16840434497101E-16,-5.47382212626882E-48)) ;
#115673=DIRECTION('center_axis',(0.,1.,0.)) ;
#115674=DIRECTION('ref_axis',(0.,0.,-1.)) ;
#115675=DIRECTION('center_axis',(0.,0.,1.)) ;
#115676=DIRECTION('ref_axis',(1.,0.,0.)) ;
#115677=DIRECTION('center_axis',(0.,0.,-1.)) ;
#115678=DIRECTION('ref_axis',(-1.,0.,0.)) ;
#115679=DIRECTION('center_axis',(-1.,-1.2303003375722E-16,0.)) ;
#115680=DIRECTION('ref_axis',(0.,-1.,0.)) ;
#115681=DIRECTION('center_axis',(0.,-1.,0.)) ;
#115682=DIRECTION('ref_axis',(0.,0.,1.)) ;
#115683=DIRECTION('center_axis',(1.53063836115601E-16,-1.,5.10212787052002E-17)) ;
#115684=DIRECTION('ref_axis',(1.,1.53063836115601E-16,-6.84227765783602E-48)) ;
#115685=DIRECTION('',(-1.53063836115601E-16,1.,-5.10212787052002E-17)) ;
#115686=DIRECTION('center_axis',(0.,-1.,0.)) ;
#115687=DIRECTION('ref_axis',(0.,0.,-1.)) ;
#115688=DIRECTION('center_axis',(-1.,0.,0.)) ;
#115689=DIRECTION('ref_axis',(0.,0.,-1.)) ;
#115690=DIRECTION('center_axis',(-1.2303003375722E-16,1.,-5.10212787052002E-17)) ;
#115691=DIRECTION('ref_axis',(-1.,-1.2303003375722E-16,6.27714964143733E-33)) ;
#115692=DIRECTION('center_axis',(-8.67361737988403E-15,-1.,0.)) ;
#115693=DIRECTION('ref_axis',(1.,-8.67361737988403E-15,0.)) ;
#115694=DIRECTION('center_axis',(1.,0.,6.27714964143733E-33)) ;
#115695=DIRECTION('ref_axis',(6.27714964143733E-33,0.,-1.)) ;
#115696=DIRECTION('center_axis',(-1.,0.,-6.50521303491307E-15)) ;
#115697=DIRECTION('ref_axis',(-6.50521303491307E-15,0.,1.)) ;
#115698=DIRECTION('center_axis',(1.,0.,0.)) ;
#115699=DIRECTION('ref_axis',(0.,1.,0.)) ;
#115700=DIRECTION('center_axis',(0.,0.,-1.)) ;
#115701=DIRECTION('ref_axis',(-1.,0.,0.)) ;
#115702=DIRECTION('center_axis',(0.,0.,1.)) ;
#115703=DIRECTION('ref_axis',(1.,0.,0.)) ;
#115704=DIRECTION('center_axis',(0.,0.,-1.)) ;
#115705=DIRECTION('ref_axis',(-1.,0.,0.)) ;
#115706=DIRECTION('center_axis',(-1.,0.,0.)) ;
#115707=DIRECTION('ref_axis',(0.,0.,1.)) ;
#115708=DIRECTION('center_axis',(0.,-1.,0.)) ;
#115709=DIRECTION('ref_axis',(0.,0.,-1.)) ;
#115710=DIRECTION('center_axis',(0.,1.,0.)) ;
#115711=DIRECTION('ref_axis',(0.,0.,1.)) ;
#115712=DIRECTION('center_axis',(0.,1.,-6.50521303491307E-15)) ;
#115713=DIRECTION('ref_axis',(0.,6.50521303491307E-15,1.)) ;
#115714=DIRECTION('center_axis',(0.,-1.,0.)) ;
#115715=DIRECTION('ref_axis',(0.,0.,-1.)) ;
#115716=DIRECTION('center_axis',(0.,-1.,0.)) ;
#115717=DIRECTION('ref_axis',(0.,0.,-1.)) ;
#115718=DIRECTION('center_axis',(0.,-1.,-1.07081696047951E-16)) ;
#115719=DIRECTION('ref_axis',(0.,1.07081696047951E-16,-1.)) ;
#115720=DIRECTION('center_axis',(0.,1.,0.)) ;
#115721=DIRECTION('ref_axis',(0.,0.,1.)) ;
#115722=DIRECTION('center_axis',(-1.,0.,0.)) ;
#115723=DIRECTION('ref_axis',(0.,0.,1.)) ;
#115724=DIRECTION('center_axis',(0.,0.,1.)) ;
#115725=DIRECTION('ref_axis',(1.,0.,0.)) ;
#115726=DIRECTION('center_axis',(0.,1.,0.)) ;
#115727=DIRECTION('ref_axis',(0.,0.,1.)) ;
#115728=DIRECTION('center_axis',(0.,0.,-1.)) ;
#115729=DIRECTION('ref_axis',(-1.,0.,0.)) ;
#115730=DIRECTION('center_axis',(0.,0.,1.)) ;
#115731=DIRECTION('ref_axis',(1.,0.,0.)) ;
#115732=DIRECTION('center_axis',(0.,0.,1.)) ;
#115733=DIRECTION('ref_axis',(1.,0.,0.)) ;
#115734=DIRECTION('center_axis',(0.,0.,1.)) ;
#115735=DIRECTION('ref_axis',(1.,0.,0.)) ;
#115736=DIRECTION('center_axis',(0.,0.,-1.)) ;
#115737=DIRECTION('ref_axis',(-1.,0.,0.)) ;
#115738=DIRECTION('center_axis',(0.,1.,0.)) ;
#115739=DIRECTION('ref_axis',(0.,0.,1.)) ;
#115740=DIRECTION('center_axis',(0.,-0.707106781186558,0.707106781186537)) ;
#115741=DIRECTION('ref_axis',(0.,-0.707106781186537,-0.707106781186558)) ;
#115742=DIRECTION('center_axis',(0.,1.,0.)) ;
#115743=DIRECTION('ref_axis',(0.,0.,1.)) ;
#115744=DIRECTION('center_axis',(0.,-0.514231796959093,-0.857651245551607)) ;
#115745=DIRECTION('ref_axis',(0.,0.857651245551607,-0.514231796959093)) ;
#115746=DIRECTION('center_axis',(0.,-0.707106781186548,0.707106781186547)) ;
#115747=DIRECTION('ref_axis',(0.,-0.707106781186547,-0.707106781186548)) ;
#115748=DIRECTION('center_axis',(0.,-0.70710678118655,0.707106781186545)) ;
#115749=DIRECTION('ref_axis',(0.,-0.707106781186545,-0.70710678118655)) ;
#115750=DIRECTION('center_axis',(-1.,0.,0.)) ;
#115751=DIRECTION('ref_axis',(0.,0.,1.)) ;
#115752=DIRECTION('center_axis',(-2.23012492569676E-15,0.514231796959107,
-0.857651245551598)) ;
#115753=DIRECTION('ref_axis',(-5.69910941180089E-30,0.857651245551598,0.514231796959107)) ;
#115754=DIRECTION('center_axis',(0.,1.,0.)) ;
#115755=DIRECTION('ref_axis',(0.,0.,1.)) ;
#115756=DIRECTION('center_axis',(0.,0.,-1.)) ;
#115757=DIRECTION('ref_axis',(-1.,0.,0.)) ;
#115758=DIRECTION('center_axis',(0.,1.,0.)) ;
#115759=DIRECTION('ref_axis',(0.,0.,1.)) ;
#115760=DIRECTION('center_axis',(0.,0.,-1.)) ;
#115761=DIRECTION('ref_axis',(-1.,0.,0.)) ;
#115762=DIRECTION('center_axis',(0.,0.,-1.)) ;
#115763=DIRECTION('ref_axis',(-1.,0.,0.)) ;
#115764=DIRECTION('center_axis',(0.,0.,1.)) ;
#115765=DIRECTION('ref_axis',(1.,0.,0.)) ;
#115766=DIRECTION('center_axis',(0.,0.,-1.)) ;
#115767=DIRECTION('ref_axis',(-1.,0.,0.)) ;
#115768=DIRECTION('center_axis',(0.,1.,0.)) ;
#115769=DIRECTION('ref_axis',(0.,0.,1.)) ;
#115770=DIRECTION('center_axis',(0.,-1.,8.67361737988409E-15)) ;
#115771=DIRECTION('ref_axis',(0.,-8.67361737988409E-15,-1.)) ;
#115772=DIRECTION('center_axis',(0.,0.707106781186546,0.707106781186549)) ;
#115773=DIRECTION('ref_axis',(0.,-0.707106781186549,0.707106781186546)) ;
#115774=DIRECTION('center_axis',(0.,0.707106781186541,0.707106781186554)) ;
#115775=DIRECTION('ref_axis',(0.,-0.707106781186554,0.707106781186541)) ;
#115776=DIRECTION('center_axis',(0.,1.,1.07081696047951E-16)) ;
#115777=DIRECTION('ref_axis',(0.,-1.07081696047951E-16,1.)) ;
#115778=DIRECTION('center_axis',(0.,-1.,0.)) ;
#115779=DIRECTION('ref_axis',(0.,0.,-1.)) ;
#115780=DIRECTION('center_axis',(0.,1.,0.)) ;
#115781=DIRECTION('ref_axis',(0.,0.,1.)) ;
#115782=DIRECTION('center_axis',(0.,0.,1.)) ;
#115783=DIRECTION('ref_axis',(1.,0.,0.)) ;
#115784=DIRECTION('center_axis',(0.,1.,0.)) ;
#115785=DIRECTION('ref_axis',(0.,0.,1.)) ;
#115786=DIRECTION('center_axis',(0.,0.,1.)) ;
#115787=DIRECTION('ref_axis',(1.,0.,0.)) ;
#115788=DIRECTION('center_axis',(0.,3.99416362155027E-15,1.)) ;
#115789=DIRECTION('ref_axis',(0.,-1.,3.99416362155027E-15)) ;
#115790=DIRECTION('center_axis',(0.,0.,1.)) ;
#115791=DIRECTION('ref_axis',(1.,0.,0.)) ;
#115792=DIRECTION('center_axis',(0.,0.,-1.)) ;
#115793=DIRECTION('ref_axis',(-1.,0.,0.)) ;
#115794=DIRECTION('center_axis',(0.,0.,1.)) ;
#115795=DIRECTION('ref_axis',(1.,0.,0.)) ;
#115796=DIRECTION('center_axis',(-1.,0.,0.)) ;
#115797=DIRECTION('ref_axis',(0.,0.,1.)) ;
#115798=DIRECTION('center_axis',(0.,1.,0.)) ;
#115799=DIRECTION('ref_axis',(0.,0.,1.)) ;
#115800=DIRECTION('center_axis',(-1.,0.,0.)) ;
#115801=DIRECTION('ref_axis',(0.,0.,1.)) ;
#115802=DIRECTION('center_axis',(0.,-1.,0.)) ;
#115803=DIRECTION('ref_axis',(0.,0.,-1.)) ;
#115804=DIRECTION('center_axis',(0.,1.,0.)) ;
#115805=DIRECTION('ref_axis',(0.,0.,1.)) ;
#115806=DIRECTION('center_axis',(1.53063836115601E-16,-1.,-1.30104260698261E-16)) ;
#115807=DIRECTION('ref_axis',(1.,1.53063836115601E-16,1.99142572374599E-32)) ;
#115808=DIRECTION('center_axis',(0.,1.,0.)) ;
#115809=DIRECTION('ref_axis',(0.,0.,1.)) ;
#115810=DIRECTION('center_axis',(0.,-1.,0.)) ;
#115811=DIRECTION('ref_axis',(0.,0.,-1.)) ;
#115812=DIRECTION('center_axis',(1.,1.53063836115601E-16,2.73691106313441E-48)) ;
#115813=DIRECTION('ref_axis',(-1.53063836115601E-16,1.,-4.18922106430579E-64)) ;
#115814=DIRECTION('center_axis',(-1.,0.,0.)) ;
#115815=DIRECTION('ref_axis',(0.,0.,1.)) ;
#115816=DIRECTION('center_axis',(1.,1.53063836115601E-16,0.)) ;
#115817=DIRECTION('ref_axis',(1.53063836115601E-16,-1.,0.)) ;
#115818=DIRECTION('center_axis',(0.,1.,0.)) ;
#115819=DIRECTION('ref_axis',(1.,0.,0.)) ;
#115820=DIRECTION('center_axis',(0.,1.,0.)) ;
#115821=DIRECTION('ref_axis',(0.,0.,-1.)) ;
#115822=DIRECTION('center_axis',(0.,0.,1.)) ;
#115823=DIRECTION('ref_axis',(-1.,0.,0.)) ;
#115824=DIRECTION('center_axis',(0.,1.,0.)) ;
#115825=DIRECTION('ref_axis',(1.,0.,0.)) ;
#115826=DIRECTION('center_axis',(0.,0.,1.)) ;
#115827=DIRECTION('ref_axis',(-1.,0.,0.)) ;
#115828=DIRECTION('center_axis',(1.,1.0842021724855E-15,0.)) ;
#115829=DIRECTION('ref_axis',(1.0842021724855E-15,-1.,0.)) ;
#115830=DIRECTION('center_axis',(-1.,-1.53063836115601E-16,0.)) ;
#115831=DIRECTION('ref_axis',(0.,-1.,0.)) ;
#115832=DIRECTION('center_axis',(0.,0.,-1.)) ;
#115833=DIRECTION('ref_axis',(1.,0.,0.)) ;
#115834=DIRECTION('center_axis',(0.,0.,-1.)) ;
#115835=DIRECTION('ref_axis',(0.804034447892622,0.594582716366702,0.)) ;
#115836=DIRECTION('center_axis',(0.,0.,1.)) ;
#115837=DIRECTION('ref_axis',(1.,0.,0.)) ;
#115838=DIRECTION('',(0.,0.,-1.)) ;
#115839=DIRECTION('center_axis',(-2.16840434497101E-16,1.,1.30104260698261E-16)) ;
#115840=DIRECTION('ref_axis',(1.,2.16840434497101E-16,1.22464679914735E-16)) ;
#115841=DIRECTION('',(-2.16840434497101E-16,1.,1.30104260698261E-16)) ;
#115842=DIRECTION('center_axis',(0.,1.,0.)) ;
#115843=DIRECTION('ref_axis',(0.,0.,1.)) ;
#115844=DIRECTION('center_axis',(-1.,-1.53063836115601E-16,-2.73691106313441E-48)) ;
#115845=DIRECTION('ref_axis',(1.53063836115601E-16,-1.,4.18922106430579E-64)) ;
#115846=DIRECTION('center_axis',(1.,2.16840434497101E-16,0.)) ;
#115847=DIRECTION('ref_axis',(2.16840434497101E-16,-1.,0.)) ;
#115848=DIRECTION('center_axis',(0.,0.,1.)) ;
#115849=DIRECTION('ref_axis',(1.,0.,0.)) ;
#115850=DIRECTION('center_axis',(-1.25542992828747E-32,1.020425574104E-16,
1.)) ;
#115851=DIRECTION('ref_axis',(-1.28107280532009E-48,-1.,1.020425574104E-16)) ;
#115852=DIRECTION('center_axis',(0.,0.,1.)) ;
#115853=DIRECTION('ref_axis',(1.,0.,0.)) ;
#115854=DIRECTION('center_axis',(0.,0.,-1.)) ;
#115855=DIRECTION('ref_axis',(-1.,0.,0.)) ;
#115856=DIRECTION('center_axis',(1.,1.53063836115601E-16,-2.73691106313441E-48)) ;
#115857=DIRECTION('ref_axis',(-1.53063836115601E-16,1.,4.18922106430579E-64)) ;
#115858=DIRECTION('center_axis',(-1.,0.,0.)) ;
#115859=DIRECTION('ref_axis',(0.,0.,1.)) ;
#115860=DIRECTION('center_axis',(1.,1.53063836115601E-16,0.)) ;
#115861=DIRECTION('ref_axis',(1.53063836115601E-16,-1.,0.)) ;
#115862=DIRECTION('center_axis',(0.,1.,0.)) ;
#115863=DIRECTION('ref_axis',(1.,0.,0.)) ;
#115864=DIRECTION('center_axis',(-1.,-2.16840434497101E-16,0.)) ;
#115865=DIRECTION('ref_axis',(0.,-1.,0.)) ;
#115866=DIRECTION('center_axis',(0.,0.,-1.)) ;
#115867=DIRECTION('ref_axis',(1.,0.,0.)) ;
#115868=DIRECTION('center_axis',(-1.25542992828747E-32,1.020425574104E-16,
1.)) ;
#115869=DIRECTION('ref_axis',(0.,-1.,0.)) ;
#115870=DIRECTION('center_axis',(0.,-1.,0.)) ;
#115871=DIRECTION('ref_axis',(-6.50521303491307E-15,0.,1.)) ;
#115872=DIRECTION('center_axis',(-1.,0.,0.)) ;
#115873=DIRECTION('ref_axis',(0.,0.,-1.)) ;
#115874=DIRECTION('center_axis',(-1.,-1.53063836115601E-16,0.)) ;
#115875=DIRECTION('ref_axis',(0.,-1.,0.)) ;
#115876=DIRECTION('center_axis',(0.,-1.,0.)) ;
#115877=DIRECTION('ref_axis',(0.,0.,1.)) ;
#115878=DIRECTION('center_axis',(0.,0.,-1.)) ;
#115879=DIRECTION('ref_axis',(-1.,0.,0.)) ;
#115880=DIRECTION('center_axis',(0.,0.,-1.)) ;
#115881=DIRECTION('ref_axis',(-1.,0.,0.)) ;
#115882=DIRECTION('center_axis',(1.,1.53063836115601E-16,-3.06472600140763E-33)) ;
#115883=DIRECTION('ref_axis',(-1.53063836115601E-16,1.,4.69098718418678E-49)) ;
#115884=DIRECTION('center_axis',(-1.,0.,0.)) ;
#115885=DIRECTION('ref_axis',(0.,0.,1.)) ;
#115886=DIRECTION('center_axis',(-1.53063836115601E-16,1.,-1.020425574104E-16)) ;
#115887=DIRECTION('ref_axis',(-1.,-1.53063836115601E-16,1.3684555315672E-47)) ;
#115888=DIRECTION('',(1.53063836115601E-16,-1.,1.020425574104E-16)) ;
#115889=DIRECTION('center_axis',(0.,-1.,0.)) ;
#115890=DIRECTION('ref_axis',(0.,0.,-1.)) ;
#115891=DIRECTION('center_axis',(-1.53063836115601E-16,1.,-1.30104260698261E-16)) ;
#115892=DIRECTION('ref_axis',(-1.,-1.53063836115601E-16,1.99142572374599E-32)) ;
#115893=DIRECTION('center_axis',(0.,-1.,0.)) ;
#115894=DIRECTION('ref_axis',(0.,0.,-1.)) ;
#115895=DIRECTION('center_axis',(-1.,-1.53063836115601E-16,2.73691106313441E-48)) ;
#115896=DIRECTION('ref_axis',(1.53063836115601E-16,-1.,-4.18922106430579E-64)) ;
#115897=DIRECTION('center_axis',(1.,2.16840434497101E-16,0.)) ;
#115898=DIRECTION('ref_axis',(2.16840434497101E-16,-1.,0.)) ;
#115899=DIRECTION('center_axis',(-1.,0.,2.16840434497102E-15)) ;
#115900=DIRECTION('ref_axis',(2.16840434497102E-15,0.,1.)) ;
#115901=DIRECTION('center_axis',(-1.,-2.16840434497101E-16,0.)) ;
#115902=DIRECTION('ref_axis',(0.,-1.,0.)) ;
#115903=DIRECTION('center_axis',(0.,0.,1.)) ;
#115904=DIRECTION('ref_axis',(-1.,0.,0.)) ;
#115905=DIRECTION('center_axis',(0.,1.,0.)) ;
#115906=DIRECTION('ref_axis',(1.,0.,0.)) ;
#115907=DIRECTION('center_axis',(0.,1.,0.)) ;
#115908=DIRECTION('ref_axis',(0.,0.,-1.)) ;
#115909=DIRECTION('center_axis',(1.,0.,0.)) ;
#115910=DIRECTION('ref_axis',(0.,-1.,0.)) ;
#115911=DIRECTION('center_axis',(1.,6.50521303491304E-15,0.)) ;
#115912=DIRECTION('ref_axis',(-6.50521303491304E-15,1.,0.)) ;
#115913=DIRECTION('center_axis',(8.67361737988403E-15,1.,0.)) ;
#115914=DIRECTION('ref_axis',(-1.,8.67361737988403E-15,0.)) ;
#115915=DIRECTION('center_axis',(1.2303003375722E-16,-1.,1.020425574104E-16)) ;
#115916=DIRECTION('ref_axis',(1.,1.2303003375722E-16,-1.25542992828747E-32)) ;
#115917=DIRECTION('center_axis',(0.,1.,0.)) ;
#115918=DIRECTION('ref_axis',(0.,0.,1.)) ;
#115919=DIRECTION('center_axis',(0.,1.,0.)) ;
#115920=DIRECTION('ref_axis',(1.,0.,0.)) ;
#115921=DIRECTION('center_axis',(1.,1.2303003375722E-16,0.)) ;
#115922=DIRECTION('ref_axis',(1.2303003375722E-16,-1.,0.)) ;
#115923=DIRECTION('center_axis',(0.,0.,1.)) ;
#115924=DIRECTION('ref_axis',(-1.,0.,0.)) ;
#115925=DIRECTION('center_axis',(0.,1.,0.)) ;
#115926=DIRECTION('ref_axis',(1.,0.,0.)) ;
#115927=DIRECTION('center_axis',(0.,0.,-1.)) ;
#115928=DIRECTION('ref_axis',(1.,0.,0.)) ;
#115929=DIRECTION('center_axis',(0.,0.,-1.)) ;
#115930=DIRECTION('ref_axis',(-1.,0.,0.)) ;
#115931=DIRECTION('center_axis',(0.,0.,1.)) ;
#115932=DIRECTION('ref_axis',(1.,0.,0.)) ;
#115933=DIRECTION('center_axis',(-2.16840434497101E-16,1.,-1.020425574104E-16)) ;
#115934=DIRECTION('ref_axis',(-1.,-2.16840434497101E-16,5.47382212626882E-48)) ;
#115935=DIRECTION('center_axis',(0.,1.,0.)) ;
#115936=DIRECTION('ref_axis',(0.,0.,-1.)) ;
#115937=DIRECTION('center_axis',(1.,0.,1.25542992828747E-32)) ;
#115938=DIRECTION('ref_axis',(1.25542992828747E-32,0.,-1.)) ;
#115939=DIRECTION('center_axis',(1.,0.,0.)) ;
#115940=DIRECTION('ref_axis',(0.,0.,-1.)) ;
#115941=DIRECTION('center_axis',(-1.,-1.2303003375722E-16,0.)) ;
#115942=DIRECTION('ref_axis',(0.,-1.,0.)) ;
#115943=DIRECTION('center_axis',(0.,0.,-1.)) ;
#115944=DIRECTION('ref_axis',(1.,0.,0.)) ;
#115945=DIRECTION('center_axis',(0.,0.,-1.)) ;
#115946=DIRECTION('ref_axis',(-1.,0.,0.)) ;
#115947=DIRECTION('',(0.,0.,1.)) ;
#115948=DIRECTION('center_axis',(0.,0.,1.)) ;
#115949=DIRECTION('ref_axis',(1.,0.,0.)) ;
#115950=DIRECTION('center_axis',(0.,0.,1.)) ;
#115951=DIRECTION('ref_axis',(1.,0.,0.)) ;
#115952=DIRECTION('center_axis',(6.27714964143733E-33,-5.10212787052002E-17,
-1.)) ;
#115953=DIRECTION('ref_axis',(3.20268201330022E-49,1.,-5.10212787052002E-17)) ;
#115954=DIRECTION('center_axis',(1.,1.53063836115601E-16,-1.53236300070382E-33)) ;
#115955=DIRECTION('ref_axis',(-1.53063836115601E-16,1.,2.34549359209339E-49)) ;
#115956=DIRECTION('center_axis',(-1.,0.,0.)) ;
#115957=DIRECTION('ref_axis',(0.,0.,1.)) ;
#115958=DIRECTION('center_axis',(1.,0.,0.)) ;
#115959=DIRECTION('ref_axis',(0.,0.,-1.)) ;
#115960=DIRECTION('center_axis',(0.,1.,0.)) ;
#115961=DIRECTION('ref_axis',(1.,0.,0.)) ;
#115962=DIRECTION('center_axis',(-4.33680868994202E-15,1.,0.)) ;
#115963=DIRECTION('ref_axis',(1.,4.33680868994202E-15,0.)) ;
#115964=DIRECTION('center_axis',(0.,-1.,0.)) ;
#115965=DIRECTION('ref_axis',(0.,0.,-1.)) ;
#115966=DIRECTION('center_axis',(0.,0.,-1.)) ;
#115967=DIRECTION('ref_axis',(1.,0.,0.)) ;
#115968=DIRECTION('center_axis',(0.,0.,1.)) ;
#115969=DIRECTION('ref_axis',(1.,0.,0.)) ;
#115970=DIRECTION('center_axis',(0.,0.,-1.)) ;
#115971=DIRECTION('ref_axis',(-1.,0.,0.)) ;
#115972=DIRECTION('center_axis',(0.,1.,0.)) ;
#115973=DIRECTION('ref_axis',(1.,0.,0.)) ;
#115974=DIRECTION('center_axis',(1.,1.2303003375722E-16,0.)) ;
#115975=DIRECTION('ref_axis',(1.2303003375722E-16,-1.,0.)) ;
#115976=DIRECTION('center_axis',(0.,1.,0.)) ;
#115977=DIRECTION('ref_axis',(-6.50521303491307E-15,0.,-1.)) ;
#115978=DIRECTION('center_axis',(6.27714964143733E-33,-5.10212787052002E-17,
-1.)) ;
#115979=DIRECTION('ref_axis',(0.,1.,0.)) ;
#115980=DIRECTION('center_axis',(0.,-1.,0.)) ;
#115981=DIRECTION('ref_axis',(0.,0.,1.)) ;
#115982=DIRECTION('center_axis',(2.16840434497101E-16,-1.,5.10212787052002E-17)) ;
#115983=DIRECTION('ref_axis',(1.,2.16840434497101E-16,-5.47382212626882E-48)) ;
#115984=DIRECTION('center_axis',(0.,1.,0.)) ;
#115985=DIRECTION('ref_axis',(0.,0.,-1.)) ;
#115986=DIRECTION('center_axis',(0.,0.,1.)) ;
#115987=DIRECTION('ref_axis',(1.,0.,0.)) ;
#115988=DIRECTION('center_axis',(0.,0.,-1.)) ;
#115989=DIRECTION('ref_axis',(-1.,0.,0.)) ;
#115990=DIRECTION('center_axis',(-1.,-1.2303003375722E-16,0.)) ;
#115991=DIRECTION('ref_axis',(0.,-1.,0.)) ;
#115992=DIRECTION('center_axis',(0.,-1.,0.)) ;
#115993=DIRECTION('ref_axis',(0.,0.,1.)) ;
#115994=DIRECTION('center_axis',(1.53063836115601E-16,-1.,5.10212787052002E-17)) ;
#115995=DIRECTION('ref_axis',(1.,1.53063836115601E-16,-6.84227765783602E-48)) ;
#115996=DIRECTION('',(-1.53063836115601E-16,1.,-5.10212787052002E-17)) ;
#115997=DIRECTION('center_axis',(0.,-1.,0.)) ;
#115998=DIRECTION('ref_axis',(0.,0.,-1.)) ;
#115999=DIRECTION('center_axis',(-1.,0.,0.)) ;
#116000=DIRECTION('ref_axis',(0.,0.,-1.)) ;
#116001=DIRECTION('center_axis',(-1.2303003375722E-16,1.,-5.10212787052002E-17)) ;
#116002=DIRECTION('ref_axis',(-1.,-1.2303003375722E-16,6.27714964143733E-33)) ;
#116003=DIRECTION('center_axis',(-8.67361737988403E-15,-1.,0.)) ;
#116004=DIRECTION('ref_axis',(1.,-8.67361737988403E-15,0.)) ;
#116005=DIRECTION('center_axis',(1.,0.,6.27714964143733E-33)) ;
#116006=DIRECTION('ref_axis',(6.27714964143733E-33,0.,-1.)) ;
#116007=DIRECTION('center_axis',(-1.,0.,-6.50521303491307E-15)) ;
#116008=DIRECTION('ref_axis',(-6.50521303491307E-15,0.,1.)) ;
#116009=DIRECTION('center_axis',(1.,0.,0.)) ;
#116010=DIRECTION('ref_axis',(0.,1.,0.)) ;
#116011=DIRECTION('center_axis',(0.,0.,-1.)) ;
#116012=DIRECTION('ref_axis',(-1.,0.,0.)) ;
#116013=DIRECTION('center_axis',(0.,0.,1.)) ;
#116014=DIRECTION('ref_axis',(1.,0.,0.)) ;
#116015=DIRECTION('center_axis',(0.,0.,-1.)) ;
#116016=DIRECTION('ref_axis',(-1.,0.,0.)) ;
#116017=DIRECTION('center_axis',(-1.,0.,0.)) ;
#116018=DIRECTION('ref_axis',(0.,0.,1.)) ;
#116019=DIRECTION('center_axis',(0.,-1.,0.)) ;
#116020=DIRECTION('ref_axis',(0.,0.,-1.)) ;
#116021=DIRECTION('center_axis',(0.,1.,0.)) ;
#116022=DIRECTION('ref_axis',(0.,0.,1.)) ;
#116023=DIRECTION('center_axis',(0.,1.,-6.50521303491307E-15)) ;
#116024=DIRECTION('ref_axis',(0.,6.50521303491307E-15,1.)) ;
#116025=DIRECTION('center_axis',(0.,-1.,0.)) ;
#116026=DIRECTION('ref_axis',(0.,0.,-1.)) ;
#116027=DIRECTION('center_axis',(0.,-1.,0.)) ;
#116028=DIRECTION('ref_axis',(0.,0.,-1.)) ;
#116029=DIRECTION('center_axis',(0.,-1.,-1.07081696047951E-16)) ;
#116030=DIRECTION('ref_axis',(0.,1.07081696047951E-16,-1.)) ;
#116031=DIRECTION('center_axis',(0.,1.,0.)) ;
#116032=DIRECTION('ref_axis',(0.,0.,1.)) ;
#116033=DIRECTION('center_axis',(-1.,0.,0.)) ;
#116034=DIRECTION('ref_axis',(0.,0.,1.)) ;
#116035=DIRECTION('center_axis',(0.,0.,1.)) ;
#116036=DIRECTION('ref_axis',(1.,0.,0.)) ;
#116037=DIRECTION('center_axis',(0.,1.,0.)) ;
#116038=DIRECTION('ref_axis',(0.,0.,1.)) ;
#116039=DIRECTION('center_axis',(0.,0.,-1.)) ;
#116040=DIRECTION('ref_axis',(-1.,0.,0.)) ;
#116041=DIRECTION('center_axis',(0.,0.,1.)) ;
#116042=DIRECTION('ref_axis',(1.,0.,0.)) ;
#116043=DIRECTION('center_axis',(0.,0.,1.)) ;
#116044=DIRECTION('ref_axis',(1.,0.,0.)) ;
#116045=DIRECTION('center_axis',(0.,0.,1.)) ;
#116046=DIRECTION('ref_axis',(1.,0.,0.)) ;
#116047=DIRECTION('center_axis',(0.,0.,-1.)) ;
#116048=DIRECTION('ref_axis',(-1.,0.,0.)) ;
#116049=DIRECTION('center_axis',(0.,1.,0.)) ;
#116050=DIRECTION('ref_axis',(0.,0.,1.)) ;
#116051=DIRECTION('center_axis',(0.,-0.707106781186558,0.707106781186537)) ;
#116052=DIRECTION('ref_axis',(0.,-0.707106781186537,-0.707106781186558)) ;
#116053=DIRECTION('center_axis',(0.,1.,0.)) ;
#116054=DIRECTION('ref_axis',(0.,0.,1.)) ;
#116055=DIRECTION('center_axis',(0.,-0.514231796959093,-0.857651245551607)) ;
#116056=DIRECTION('ref_axis',(0.,0.857651245551607,-0.514231796959093)) ;
#116057=DIRECTION('center_axis',(0.,-0.707106781186548,0.707106781186547)) ;
#116058=DIRECTION('ref_axis',(0.,-0.707106781186547,-0.707106781186548)) ;
#116059=DIRECTION('center_axis',(0.,-0.707106781186548,0.707106781186548)) ;
#116060=DIRECTION('ref_axis',(0.,-0.707106781186548,-0.707106781186548)) ;
#116061=DIRECTION('center_axis',(-1.,0.,0.)) ;
#116062=DIRECTION('ref_axis',(0.,0.,1.)) ;
#116063=DIRECTION('center_axis',(0.,0.514231796959095,-0.857651245551606)) ;
#116064=DIRECTION('ref_axis',(0.,0.857651245551606,0.514231796959095)) ;
#116065=DIRECTION('center_axis',(0.,1.,0.)) ;
#116066=DIRECTION('ref_axis',(0.,0.,1.)) ;
#116067=DIRECTION('center_axis',(0.,0.,-1.)) ;
#116068=DIRECTION('ref_axis',(-1.,0.,0.)) ;
#116069=DIRECTION('center_axis',(0.,1.,0.)) ;
#116070=DIRECTION('ref_axis',(0.,0.,1.)) ;
#116071=DIRECTION('center_axis',(0.,0.,-1.)) ;
#116072=DIRECTION('ref_axis',(-1.,0.,0.)) ;
#116073=DIRECTION('center_axis',(0.,0.,-1.)) ;
#116074=DIRECTION('ref_axis',(-1.,0.,0.)) ;
#116075=DIRECTION('center_axis',(0.,0.,1.)) ;
#116076=DIRECTION('ref_axis',(1.,0.,0.)) ;
#116077=DIRECTION('center_axis',(0.,0.,-1.)) ;
#116078=DIRECTION('ref_axis',(-1.,0.,0.)) ;
#116079=DIRECTION('center_axis',(0.,1.,0.)) ;
#116080=DIRECTION('ref_axis',(0.,0.,1.)) ;
#116081=DIRECTION('center_axis',(0.,-1.,8.67361737988409E-15)) ;
#116082=DIRECTION('ref_axis',(0.,-8.67361737988409E-15,-1.)) ;
#116083=DIRECTION('center_axis',(0.,0.707106781186546,0.707106781186549)) ;
#116084=DIRECTION('ref_axis',(0.,-0.707106781186549,0.707106781186546)) ;
#116085=DIRECTION('center_axis',(0.,0.707106781186537,0.707106781186558)) ;
#116086=DIRECTION('ref_axis',(0.,-0.707106781186558,0.707106781186537)) ;
#116087=DIRECTION('center_axis',(0.,1.,1.07081696047951E-16)) ;
#116088=DIRECTION('ref_axis',(0.,-1.07081696047951E-16,1.)) ;
#116089=DIRECTION('center_axis',(0.,-1.,0.)) ;
#116090=DIRECTION('ref_axis',(0.,0.,-1.)) ;
#116091=DIRECTION('center_axis',(0.,1.,0.)) ;
#116092=DIRECTION('ref_axis',(0.,0.,1.)) ;
#116093=DIRECTION('center_axis',(0.,0.,1.)) ;
#116094=DIRECTION('ref_axis',(1.,0.,0.)) ;
#116095=DIRECTION('center_axis',(0.,1.,0.)) ;
#116096=DIRECTION('ref_axis',(0.,0.,1.)) ;
#116097=DIRECTION('center_axis',(0.,0.,1.)) ;
#116098=DIRECTION('ref_axis',(1.,0.,0.)) ;
#116099=DIRECTION('center_axis',(0.,3.99416362155027E-15,1.)) ;
#116100=DIRECTION('ref_axis',(0.,-1.,3.99416362155027E-15)) ;
#116101=DIRECTION('center_axis',(0.,0.,1.)) ;
#116102=DIRECTION('ref_axis',(1.,0.,0.)) ;
#116103=DIRECTION('center_axis',(0.,0.,-1.)) ;
#116104=DIRECTION('ref_axis',(-1.,0.,0.)) ;
#116105=DIRECTION('center_axis',(0.,0.,1.)) ;
#116106=DIRECTION('ref_axis',(1.,0.,0.)) ;
#116107=DIRECTION('center_axis',(-1.,0.,0.)) ;
#116108=DIRECTION('ref_axis',(0.,0.,1.)) ;
#116109=DIRECTION('center_axis',(0.,1.,0.)) ;
#116110=DIRECTION('ref_axis',(0.,0.,1.)) ;
#116111=DIRECTION('center_axis',(-1.,0.,0.)) ;
#116112=DIRECTION('ref_axis',(0.,0.,1.)) ;
#116113=DIRECTION('center_axis',(0.,-1.,0.)) ;
#116114=DIRECTION('ref_axis',(0.,0.,-1.)) ;
#116115=DIRECTION('center_axis',(0.,1.,0.)) ;
#116116=DIRECTION('ref_axis',(0.,0.,1.)) ;
#116117=DIRECTION('center_axis',(1.53063836115601E-16,-1.,-1.30104260698261E-16)) ;
#116118=DIRECTION('ref_axis',(1.,1.53063836115601E-16,1.99142572374599E-32)) ;
#116119=DIRECTION('center_axis',(0.,1.,0.)) ;
#116120=DIRECTION('ref_axis',(0.,0.,1.)) ;
#116121=DIRECTION('center_axis',(0.,-1.,0.)) ;
#116122=DIRECTION('ref_axis',(0.,0.,-1.)) ;
#116123=DIRECTION('center_axis',(1.,1.53063836115601E-16,2.73691106313441E-48)) ;
#116124=DIRECTION('ref_axis',(-1.53063836115601E-16,1.,-4.18922106430579E-64)) ;
#116125=DIRECTION('center_axis',(-1.,0.,0.)) ;
#116126=DIRECTION('ref_axis',(0.,0.,1.)) ;
#116127=DIRECTION('center_axis',(1.,1.53063836115601E-16,0.)) ;
#116128=DIRECTION('ref_axis',(1.53063836115601E-16,-1.,0.)) ;
#116129=DIRECTION('center_axis',(0.,1.,0.)) ;
#116130=DIRECTION('ref_axis',(1.,0.,0.)) ;
#116131=DIRECTION('center_axis',(0.,1.,0.)) ;
#116132=DIRECTION('ref_axis',(0.,0.,-1.)) ;
#116133=DIRECTION('center_axis',(0.,0.,1.)) ;
#116134=DIRECTION('ref_axis',(-1.,0.,0.)) ;
#116135=DIRECTION('center_axis',(0.,1.,0.)) ;
#116136=DIRECTION('ref_axis',(1.,0.,0.)) ;
#116137=DIRECTION('center_axis',(0.,0.,1.)) ;
#116138=DIRECTION('ref_axis',(-1.,0.,0.)) ;
#116139=DIRECTION('center_axis',(1.,1.0842021724855E-15,0.)) ;
#116140=DIRECTION('ref_axis',(1.0842021724855E-15,-1.,0.)) ;
#116141=DIRECTION('center_axis',(-1.,-1.53063836115601E-16,0.)) ;
#116142=DIRECTION('ref_axis',(0.,-1.,0.)) ;
#116143=DIRECTION('center_axis',(0.,0.,-1.)) ;
#116144=DIRECTION('ref_axis',(1.,0.,0.)) ;
#116145=DIRECTION('center_axis',(0.,0.,-1.)) ;
#116146=DIRECTION('ref_axis',(0.804034447892617,0.594582716366709,0.)) ;
#116147=DIRECTION('center_axis',(0.,0.,1.)) ;
#116148=DIRECTION('ref_axis',(1.,0.,0.)) ;
#116149=DIRECTION('',(0.,0.,-1.)) ;
#116150=DIRECTION('center_axis',(-2.16840434497101E-16,1.,1.30104260698261E-16)) ;
#116151=DIRECTION('ref_axis',(1.,2.16840434497101E-16,1.22464679914735E-16)) ;
#116152=DIRECTION('',(-2.16840434497101E-16,1.,1.30104260698261E-16)) ;
#116153=DIRECTION('center_axis',(0.,1.,0.)) ;
#116154=DIRECTION('ref_axis',(0.,0.,1.)) ;
#116155=DIRECTION('center_axis',(-1.,-1.53063836115601E-16,-2.73691106313441E-48)) ;
#116156=DIRECTION('ref_axis',(1.53063836115601E-16,-1.,4.18922106430579E-64)) ;
#116157=DIRECTION('center_axis',(1.,2.16840434497101E-16,0.)) ;
#116158=DIRECTION('ref_axis',(2.16840434497101E-16,-1.,0.)) ;
#116159=DIRECTION('center_axis',(0.,0.,1.)) ;
#116160=DIRECTION('ref_axis',(1.,0.,0.)) ;
#116161=DIRECTION('center_axis',(-1.25542992828747E-32,1.020425574104E-16,
1.)) ;
#116162=DIRECTION('ref_axis',(-1.28107280532009E-48,-1.,1.020425574104E-16)) ;
#116163=DIRECTION('center_axis',(0.,0.,1.)) ;
#116164=DIRECTION('ref_axis',(1.,0.,0.)) ;
#116165=DIRECTION('center_axis',(0.,0.,-1.)) ;
#116166=DIRECTION('ref_axis',(-1.,0.,0.)) ;
#116167=DIRECTION('center_axis',(1.,1.53063836115601E-16,-2.73691106313441E-48)) ;
#116168=DIRECTION('ref_axis',(-1.53063836115601E-16,1.,4.18922106430579E-64)) ;
#116169=DIRECTION('center_axis',(-1.,0.,0.)) ;
#116170=DIRECTION('ref_axis',(0.,0.,1.)) ;
#116171=DIRECTION('center_axis',(1.,1.53063836115601E-16,0.)) ;
#116172=DIRECTION('ref_axis',(1.53063836115601E-16,-1.,0.)) ;
#116173=DIRECTION('center_axis',(0.,1.,0.)) ;
#116174=DIRECTION('ref_axis',(1.,0.,0.)) ;
#116175=DIRECTION('center_axis',(-1.,-2.16840434497101E-16,0.)) ;
#116176=DIRECTION('ref_axis',(0.,-1.,0.)) ;
#116177=DIRECTION('center_axis',(0.,0.,-1.)) ;
#116178=DIRECTION('ref_axis',(1.,0.,0.)) ;
#116179=DIRECTION('center_axis',(-1.25542992828747E-32,1.020425574104E-16,
1.)) ;
#116180=DIRECTION('ref_axis',(0.,-1.,0.)) ;
#116181=DIRECTION('center_axis',(0.,-1.,0.)) ;
#116182=DIRECTION('ref_axis',(-6.50521303491307E-15,0.,1.)) ;
#116183=DIRECTION('center_axis',(-1.,0.,0.)) ;
#116184=DIRECTION('ref_axis',(0.,0.,-1.)) ;
#116185=DIRECTION('center_axis',(-1.,-1.53063836115601E-16,0.)) ;
#116186=DIRECTION('ref_axis',(0.,-1.,0.)) ;
#116187=DIRECTION('center_axis',(0.,-1.,0.)) ;
#116188=DIRECTION('ref_axis',(0.,0.,1.)) ;
#116189=DIRECTION('center_axis',(0.,0.,-1.)) ;
#116190=DIRECTION('ref_axis',(-1.,0.,0.)) ;
#116191=DIRECTION('center_axis',(0.,0.,-1.)) ;
#116192=DIRECTION('ref_axis',(-1.,0.,0.)) ;
#116193=DIRECTION('center_axis',(1.,1.53063836115601E-16,-3.06472600140763E-33)) ;
#116194=DIRECTION('ref_axis',(-1.53063836115601E-16,1.,4.69098718418678E-49)) ;
#116195=DIRECTION('center_axis',(-1.,0.,0.)) ;
#116196=DIRECTION('ref_axis',(0.,0.,1.)) ;
#116197=DIRECTION('center_axis',(-1.53063836115601E-16,1.,-1.020425574104E-16)) ;
#116198=DIRECTION('ref_axis',(-1.,-1.53063836115601E-16,1.3684555315672E-47)) ;
#116199=DIRECTION('',(1.53063836115601E-16,-1.,1.020425574104E-16)) ;
#116200=DIRECTION('center_axis',(0.,-1.,0.)) ;
#116201=DIRECTION('ref_axis',(0.,0.,-1.)) ;
#116202=DIRECTION('center_axis',(-1.53063836115601E-16,1.,-1.30104260698261E-16)) ;
#116203=DIRECTION('ref_axis',(-1.,-1.53063836115601E-16,1.99142572374599E-32)) ;
#116204=DIRECTION('center_axis',(0.,-1.,0.)) ;
#116205=DIRECTION('ref_axis',(0.,0.,-1.)) ;
#116206=DIRECTION('center_axis',(-1.,-1.53063836115601E-16,2.73691106313441E-48)) ;
#116207=DIRECTION('ref_axis',(1.53063836115601E-16,-1.,-4.18922106430579E-64)) ;
#116208=DIRECTION('center_axis',(1.,2.16840434497101E-16,0.)) ;
#116209=DIRECTION('ref_axis',(2.16840434497101E-16,-1.,0.)) ;
#116210=DIRECTION('center_axis',(-1.,0.,2.16840434497102E-15)) ;
#116211=DIRECTION('ref_axis',(2.16840434497102E-15,0.,1.)) ;
#116212=DIRECTION('center_axis',(-1.,-2.16840434497101E-16,0.)) ;
#116213=DIRECTION('ref_axis',(0.,-1.,0.)) ;
#116214=DIRECTION('center_axis',(0.,0.,1.)) ;
#116215=DIRECTION('ref_axis',(-1.,0.,0.)) ;
#116216=DIRECTION('center_axis',(0.,1.,0.)) ;
#116217=DIRECTION('ref_axis',(1.,0.,0.)) ;
#116218=DIRECTION('center_axis',(0.,1.,0.)) ;
#116219=DIRECTION('ref_axis',(0.,0.,-1.)) ;
#116220=DIRECTION('center_axis',(1.,0.,0.)) ;
#116221=DIRECTION('ref_axis',(0.,-1.,0.)) ;
#116222=DIRECTION('center_axis',(1.,6.50521303491304E-15,0.)) ;
#116223=DIRECTION('ref_axis',(-6.50521303491304E-15,1.,0.)) ;
#116224=DIRECTION('center_axis',(8.67361737988403E-15,1.,0.)) ;
#116225=DIRECTION('ref_axis',(-1.,8.67361737988403E-15,0.)) ;
#116226=DIRECTION('center_axis',(1.2303003375722E-16,-1.,1.020425574104E-16)) ;
#116227=DIRECTION('ref_axis',(1.,1.2303003375722E-16,-1.25542992828747E-32)) ;
#116228=DIRECTION('center_axis',(0.,1.,0.)) ;
#116229=DIRECTION('ref_axis',(0.,0.,1.)) ;
#116230=DIRECTION('center_axis',(0.,1.,0.)) ;
#116231=DIRECTION('ref_axis',(1.,0.,0.)) ;
#116232=DIRECTION('center_axis',(1.,1.2303003375722E-16,0.)) ;
#116233=DIRECTION('ref_axis',(1.2303003375722E-16,-1.,0.)) ;
#116234=DIRECTION('center_axis',(0.,0.,1.)) ;
#116235=DIRECTION('ref_axis',(-1.,0.,0.)) ;
#116236=DIRECTION('center_axis',(0.,1.,0.)) ;
#116237=DIRECTION('ref_axis',(1.,0.,0.)) ;
#116238=DIRECTION('center_axis',(0.,0.,-1.)) ;
#116239=DIRECTION('ref_axis',(1.,0.,0.)) ;
#116240=DIRECTION('center_axis',(0.,0.,-1.)) ;
#116241=DIRECTION('ref_axis',(-1.,0.,0.)) ;
#116242=DIRECTION('center_axis',(0.,0.,1.)) ;
#116243=DIRECTION('ref_axis',(1.,0.,0.)) ;
#116244=DIRECTION('center_axis',(-2.16840434497101E-16,1.,-1.020425574104E-16)) ;
#116245=DIRECTION('ref_axis',(-1.,-2.16840434497101E-16,5.47382212626882E-48)) ;
#116246=DIRECTION('center_axis',(0.,1.,0.)) ;
#116247=DIRECTION('ref_axis',(0.,0.,-1.)) ;
#116248=DIRECTION('center_axis',(1.,0.,1.25542992828747E-32)) ;
#116249=DIRECTION('ref_axis',(1.25542992828747E-32,0.,-1.)) ;
#116250=DIRECTION('center_axis',(1.,0.,0.)) ;
#116251=DIRECTION('ref_axis',(0.,0.,-1.)) ;
#116252=DIRECTION('center_axis',(-1.,-1.2303003375722E-16,0.)) ;
#116253=DIRECTION('ref_axis',(0.,-1.,0.)) ;
#116254=DIRECTION('center_axis',(0.,0.,-1.)) ;
#116255=DIRECTION('ref_axis',(1.,0.,0.)) ;
#116256=DIRECTION('center_axis',(0.,0.,-1.)) ;
#116257=DIRECTION('ref_axis',(-1.,0.,0.)) ;
#116258=DIRECTION('',(0.,0.,1.)) ;
#116259=DIRECTION('center_axis',(0.,0.,1.)) ;
#116260=DIRECTION('ref_axis',(1.,0.,0.)) ;
#116261=DIRECTION('center_axis',(0.,0.,1.)) ;
#116262=DIRECTION('ref_axis',(1.,0.,0.)) ;
#116263=DIRECTION('center_axis',(6.27714964143733E-33,-5.10212787052002E-17,
-1.)) ;
#116264=DIRECTION('ref_axis',(3.20268201330022E-49,1.,-5.10212787052002E-17)) ;
#116265=DIRECTION('center_axis',(1.,1.53063836115601E-16,-1.53236300070382E-33)) ;
#116266=DIRECTION('ref_axis',(-1.53063836115601E-16,1.,2.34549359209339E-49)) ;
#116267=DIRECTION('center_axis',(-1.,0.,0.)) ;
#116268=DIRECTION('ref_axis',(0.,0.,1.)) ;
#116269=DIRECTION('center_axis',(1.,0.,0.)) ;
#116270=DIRECTION('ref_axis',(0.,0.,-1.)) ;
#116271=DIRECTION('center_axis',(0.,1.,0.)) ;
#116272=DIRECTION('ref_axis',(1.,0.,0.)) ;
#116273=DIRECTION('center_axis',(-4.33680868994202E-15,1.,0.)) ;
#116274=DIRECTION('ref_axis',(1.,4.33680868994202E-15,0.)) ;
#116275=DIRECTION('center_axis',(0.,-1.,0.)) ;
#116276=DIRECTION('ref_axis',(0.,0.,-1.)) ;
#116277=DIRECTION('center_axis',(0.,0.,-1.)) ;
#116278=DIRECTION('ref_axis',(1.,0.,0.)) ;
#116279=DIRECTION('center_axis',(0.,0.,1.)) ;
#116280=DIRECTION('ref_axis',(1.,0.,0.)) ;
#116281=DIRECTION('center_axis',(0.,0.,-1.)) ;
#116282=DIRECTION('ref_axis',(-1.,0.,0.)) ;
#116283=DIRECTION('center_axis',(0.,1.,0.)) ;
#116284=DIRECTION('ref_axis',(1.,0.,0.)) ;
#116285=DIRECTION('center_axis',(1.,1.2303003375722E-16,0.)) ;
#116286=DIRECTION('ref_axis',(1.2303003375722E-16,-1.,0.)) ;
#116287=DIRECTION('center_axis',(0.,1.,0.)) ;
#116288=DIRECTION('ref_axis',(-6.50521303491307E-15,0.,-1.)) ;
#116289=DIRECTION('center_axis',(6.27714964143733E-33,-5.10212787052002E-17,
-1.)) ;
#116290=DIRECTION('ref_axis',(0.,1.,0.)) ;
#116291=DIRECTION('center_axis',(0.,-1.,0.)) ;
#116292=DIRECTION('ref_axis',(0.,0.,1.)) ;
#116293=DIRECTION('center_axis',(2.16840434497101E-16,-1.,5.10212787052002E-17)) ;
#116294=DIRECTION('ref_axis',(1.,2.16840434497101E-16,-5.47382212626882E-48)) ;
#116295=DIRECTION('center_axis',(0.,1.,0.)) ;
#116296=DIRECTION('ref_axis',(0.,0.,-1.)) ;
#116297=DIRECTION('center_axis',(0.,0.,1.)) ;
#116298=DIRECTION('ref_axis',(1.,0.,0.)) ;
#116299=DIRECTION('center_axis',(0.,0.,-1.)) ;
#116300=DIRECTION('ref_axis',(-1.,0.,0.)) ;
#116301=DIRECTION('center_axis',(-1.,-1.2303003375722E-16,0.)) ;
#116302=DIRECTION('ref_axis',(0.,-1.,0.)) ;
#116303=DIRECTION('center_axis',(0.,-1.,0.)) ;
#116304=DIRECTION('ref_axis',(0.,0.,1.)) ;
#116305=DIRECTION('center_axis',(1.53063836115601E-16,-1.,5.10212787052002E-17)) ;
#116306=DIRECTION('ref_axis',(1.,1.53063836115601E-16,-6.84227765783602E-48)) ;
#116307=DIRECTION('',(-1.53063836115601E-16,1.,-5.10212787052002E-17)) ;
#116308=DIRECTION('center_axis',(0.,-1.,0.)) ;
#116309=DIRECTION('ref_axis',(0.,0.,-1.)) ;
#116310=DIRECTION('center_axis',(-1.,0.,0.)) ;
#116311=DIRECTION('ref_axis',(0.,0.,-1.)) ;
#116312=DIRECTION('center_axis',(-1.2303003375722E-16,1.,-5.10212787052002E-17)) ;
#116313=DIRECTION('ref_axis',(-1.,-1.2303003375722E-16,6.27714964143733E-33)) ;
#116314=DIRECTION('center_axis',(-8.67361737988403E-15,-1.,0.)) ;
#116315=DIRECTION('ref_axis',(1.,-8.67361737988403E-15,0.)) ;
#116316=DIRECTION('center_axis',(1.,0.,6.27714964143733E-33)) ;
#116317=DIRECTION('ref_axis',(6.27714964143733E-33,0.,-1.)) ;
#116318=DIRECTION('center_axis',(-1.,0.,-6.50521303491307E-15)) ;
#116319=DIRECTION('ref_axis',(-6.50521303491307E-15,0.,1.)) ;
#116320=DIRECTION('center_axis',(1.,0.,0.)) ;
#116321=DIRECTION('ref_axis',(0.,1.,0.)) ;
#116322=DIRECTION('center_axis',(0.,0.,-1.)) ;
#116323=DIRECTION('ref_axis',(-1.,0.,0.)) ;
#116324=DIRECTION('center_axis',(0.,0.,1.)) ;
#116325=DIRECTION('ref_axis',(1.,0.,0.)) ;
#116326=DIRECTION('center_axis',(0.,0.,-1.)) ;
#116327=DIRECTION('ref_axis',(-1.,0.,0.)) ;
#116328=DIRECTION('center_axis',(-1.,0.,0.)) ;
#116329=DIRECTION('ref_axis',(0.,0.,1.)) ;
#116330=DIRECTION('center_axis',(0.,-1.,0.)) ;
#116331=DIRECTION('ref_axis',(0.,0.,-1.)) ;
#116332=DIRECTION('center_axis',(0.,1.,0.)) ;
#116333=DIRECTION('ref_axis',(0.,0.,1.)) ;
#116334=DIRECTION('center_axis',(0.,1.,-6.50521303491307E-15)) ;
#116335=DIRECTION('ref_axis',(0.,6.50521303491307E-15,1.)) ;
#116336=DIRECTION('center_axis',(0.,-1.,0.)) ;
#116337=DIRECTION('ref_axis',(0.,0.,-1.)) ;
#116338=DIRECTION('center_axis',(0.,-1.,0.)) ;
#116339=DIRECTION('ref_axis',(0.,0.,-1.)) ;
#116340=DIRECTION('center_axis',(0.,-1.,-1.07081696047951E-16)) ;
#116341=DIRECTION('ref_axis',(0.,1.07081696047951E-16,-1.)) ;
#116342=DIRECTION('center_axis',(0.,1.,0.)) ;
#116343=DIRECTION('ref_axis',(0.,0.,1.)) ;
#116344=DIRECTION('center_axis',(-1.,0.,0.)) ;
#116345=DIRECTION('ref_axis',(0.,0.,1.)) ;
#116346=DIRECTION('center_axis',(0.,0.,1.)) ;
#116347=DIRECTION('ref_axis',(1.,0.,0.)) ;
#116348=DIRECTION('center_axis',(0.,1.,0.)) ;
#116349=DIRECTION('ref_axis',(0.,0.,1.)) ;
#116350=DIRECTION('center_axis',(0.,0.,-1.)) ;
#116351=DIRECTION('ref_axis',(-1.,0.,0.)) ;
#116352=DIRECTION('center_axis',(0.,0.,1.)) ;
#116353=DIRECTION('ref_axis',(1.,0.,0.)) ;
#116354=DIRECTION('center_axis',(0.,0.,1.)) ;
#116355=DIRECTION('ref_axis',(1.,0.,0.)) ;
#116356=DIRECTION('center_axis',(0.,0.,1.)) ;
#116357=DIRECTION('ref_axis',(1.,0.,0.)) ;
#116358=DIRECTION('center_axis',(0.,0.,-1.)) ;
#116359=DIRECTION('ref_axis',(-1.,0.,0.)) ;
#116360=DIRECTION('center_axis',(0.,1.,0.)) ;
#116361=DIRECTION('ref_axis',(0.,0.,1.)) ;
#116362=DIRECTION('center_axis',(0.,-0.707106781186558,0.707106781186537)) ;
#116363=DIRECTION('ref_axis',(0.,-0.707106781186537,-0.707106781186558)) ;
#116364=DIRECTION('center_axis',(0.,1.,0.)) ;
#116365=DIRECTION('ref_axis',(0.,0.,1.)) ;
#116366=DIRECTION('center_axis',(0.,-0.514231796959093,-0.857651245551607)) ;
#116367=DIRECTION('ref_axis',(0.,0.857651245551607,-0.514231796959093)) ;
#116368=DIRECTION('center_axis',(0.,-0.707106781186548,0.707106781186547)) ;
#116369=DIRECTION('ref_axis',(0.,-0.707106781186547,-0.707106781186548)) ;
#116370=DIRECTION('center_axis',(0.,-0.707106781186548,0.707106781186548)) ;
#116371=DIRECTION('ref_axis',(0.,-0.707106781186548,-0.707106781186548)) ;
#116372=DIRECTION('center_axis',(-1.,0.,0.)) ;
#116373=DIRECTION('ref_axis',(0.,0.,1.)) ;
#116374=DIRECTION('center_axis',(0.,0.514231796959095,-0.857651245551606)) ;
#116375=DIRECTION('ref_axis',(0.,0.857651245551606,0.514231796959095)) ;
#116376=DIRECTION('center_axis',(0.,1.,0.)) ;
#116377=DIRECTION('ref_axis',(0.,0.,1.)) ;
#116378=DIRECTION('center_axis',(0.,0.,-1.)) ;
#116379=DIRECTION('ref_axis',(-1.,0.,0.)) ;
#116380=DIRECTION('center_axis',(0.,1.,0.)) ;
#116381=DIRECTION('ref_axis',(0.,0.,1.)) ;
#116382=DIRECTION('center_axis',(0.,0.,-1.)) ;
#116383=DIRECTION('ref_axis',(-1.,0.,0.)) ;
#116384=DIRECTION('center_axis',(0.,0.,-1.)) ;
#116385=DIRECTION('ref_axis',(-1.,0.,0.)) ;
#116386=DIRECTION('center_axis',(0.,0.,1.)) ;
#116387=DIRECTION('ref_axis',(1.,0.,0.)) ;
#116388=DIRECTION('center_axis',(0.,0.,-1.)) ;
#116389=DIRECTION('ref_axis',(-1.,0.,0.)) ;
#116390=DIRECTION('center_axis',(0.,1.,0.)) ;
#116391=DIRECTION('ref_axis',(0.,0.,1.)) ;
#116392=DIRECTION('center_axis',(0.,-1.,8.67361737988409E-15)) ;
#116393=DIRECTION('ref_axis',(0.,-8.67361737988409E-15,-1.)) ;
#116394=DIRECTION('center_axis',(0.,0.707106781186546,0.707106781186549)) ;
#116395=DIRECTION('ref_axis',(0.,-0.707106781186549,0.707106781186546)) ;
#116396=DIRECTION('center_axis',(0.,0.707106781186537,0.707106781186558)) ;
#116397=DIRECTION('ref_axis',(0.,-0.707106781186558,0.707106781186537)) ;
#116398=DIRECTION('center_axis',(0.,1.,1.07081696047951E-16)) ;
#116399=DIRECTION('ref_axis',(0.,-1.07081696047951E-16,1.)) ;
#116400=DIRECTION('center_axis',(0.,-1.,0.)) ;
#116401=DIRECTION('ref_axis',(0.,0.,-1.)) ;
#116402=DIRECTION('center_axis',(0.,1.,0.)) ;
#116403=DIRECTION('ref_axis',(0.,0.,1.)) ;
#116404=DIRECTION('center_axis',(0.,0.,1.)) ;
#116405=DIRECTION('ref_axis',(1.,0.,0.)) ;
#116406=DIRECTION('center_axis',(0.,1.,0.)) ;
#116407=DIRECTION('ref_axis',(0.,0.,1.)) ;
#116408=DIRECTION('center_axis',(0.,0.,1.)) ;
#116409=DIRECTION('ref_axis',(1.,0.,0.)) ;
#116410=DIRECTION('center_axis',(0.,3.99416362155027E-15,1.)) ;
#116411=DIRECTION('ref_axis',(0.,-1.,3.99416362155027E-15)) ;
#116412=DIRECTION('center_axis',(0.,0.,1.)) ;
#116413=DIRECTION('ref_axis',(1.,0.,0.)) ;
#116414=DIRECTION('center_axis',(0.,0.,-1.)) ;
#116415=DIRECTION('ref_axis',(-1.,0.,0.)) ;
#116416=DIRECTION('center_axis',(0.,0.,1.)) ;
#116417=DIRECTION('ref_axis',(1.,0.,0.)) ;
#116418=DIRECTION('center_axis',(-1.,0.,0.)) ;
#116419=DIRECTION('ref_axis',(0.,0.,1.)) ;
#116420=DIRECTION('center_axis',(0.,1.,0.)) ;
#116421=DIRECTION('ref_axis',(0.,0.,1.)) ;
#116422=DIRECTION('center_axis',(-1.,0.,0.)) ;
#116423=DIRECTION('ref_axis',(0.,0.,1.)) ;
#116424=DIRECTION('center_axis',(0.,-1.,0.)) ;
#116425=DIRECTION('ref_axis',(0.,0.,-1.)) ;
#116426=DIRECTION('center_axis',(0.,1.,0.)) ;
#116427=DIRECTION('ref_axis',(0.,0.,1.)) ;
#116428=DIRECTION('center_axis',(1.53063836115601E-16,-1.,-1.30104260698261E-16)) ;
#116429=DIRECTION('ref_axis',(1.,1.53063836115601E-16,1.99142572374599E-32)) ;
#116430=DIRECTION('center_axis',(0.,1.,0.)) ;
#116431=DIRECTION('ref_axis',(0.,0.,1.)) ;
#116432=DIRECTION('center_axis',(0.,-1.,0.)) ;
#116433=DIRECTION('ref_axis',(0.,0.,-1.)) ;
#116434=DIRECTION('center_axis',(1.,1.53063836115601E-16,2.73691106313441E-48)) ;
#116435=DIRECTION('ref_axis',(-1.53063836115601E-16,1.,-4.18922106430579E-64)) ;
#116436=DIRECTION('center_axis',(-1.,0.,0.)) ;
#116437=DIRECTION('ref_axis',(0.,0.,1.)) ;
#116438=DIRECTION('center_axis',(1.,1.53063836115601E-16,0.)) ;
#116439=DIRECTION('ref_axis',(1.53063836115601E-16,-1.,0.)) ;
#116440=DIRECTION('center_axis',(0.,1.,0.)) ;
#116441=DIRECTION('ref_axis',(1.,0.,0.)) ;
#116442=DIRECTION('center_axis',(0.,1.,0.)) ;
#116443=DIRECTION('ref_axis',(0.,0.,-1.)) ;
#116444=DIRECTION('center_axis',(0.,0.,1.)) ;
#116445=DIRECTION('ref_axis',(-1.,0.,0.)) ;
#116446=DIRECTION('center_axis',(0.,1.,0.)) ;
#116447=DIRECTION('ref_axis',(1.,0.,0.)) ;
#116448=DIRECTION('center_axis',(0.,0.,1.)) ;
#116449=DIRECTION('ref_axis',(-1.,0.,0.)) ;
#116450=DIRECTION('center_axis',(1.,1.0842021724855E-15,0.)) ;
#116451=DIRECTION('ref_axis',(1.0842021724855E-15,-1.,0.)) ;
#116452=DIRECTION('center_axis',(-1.,-1.53063836115601E-16,0.)) ;
#116453=DIRECTION('ref_axis',(0.,-1.,0.)) ;
#116454=DIRECTION('center_axis',(0.,0.,-1.)) ;
#116455=DIRECTION('ref_axis',(1.,0.,0.)) ;
#116456=DIRECTION('center_axis',(0.,0.,-1.)) ;
#116457=DIRECTION('ref_axis',(0.804034447892626,0.594582716366697,0.)) ;
#116458=DIRECTION('center_axis',(0.,0.,1.)) ;
#116459=DIRECTION('ref_axis',(1.,0.,0.)) ;
#116460=DIRECTION('',(0.,0.,-1.)) ;
#116461=DIRECTION('center_axis',(-2.16840434497101E-16,1.,1.30104260698261E-16)) ;
#116462=DIRECTION('ref_axis',(1.,2.16840434497101E-16,1.22464679914735E-16)) ;
#116463=DIRECTION('',(-2.16840434497101E-16,1.,1.30104260698261E-16)) ;
#116464=DIRECTION('center_axis',(0.,1.,0.)) ;
#116465=DIRECTION('ref_axis',(0.,0.,1.)) ;
#116466=DIRECTION('center_axis',(-1.,-1.53063836115601E-16,-2.73691106313441E-48)) ;
#116467=DIRECTION('ref_axis',(1.53063836115601E-16,-1.,4.18922106430579E-64)) ;
#116468=DIRECTION('center_axis',(1.,2.16840434497101E-16,0.)) ;
#116469=DIRECTION('ref_axis',(2.16840434497101E-16,-1.,0.)) ;
#116470=DIRECTION('center_axis',(0.,0.,1.)) ;
#116471=DIRECTION('ref_axis',(1.,0.,0.)) ;
#116472=DIRECTION('center_axis',(-1.25542992828747E-32,1.020425574104E-16,
1.)) ;
#116473=DIRECTION('ref_axis',(-1.28107280532009E-48,-1.,1.020425574104E-16)) ;
#116474=DIRECTION('center_axis',(0.,0.,1.)) ;
#116475=DIRECTION('ref_axis',(1.,0.,0.)) ;
#116476=DIRECTION('center_axis',(0.,0.,-1.)) ;
#116477=DIRECTION('ref_axis',(-1.,0.,0.)) ;
#116478=DIRECTION('center_axis',(1.,1.53063836115601E-16,-2.73691106313441E-48)) ;
#116479=DIRECTION('ref_axis',(-1.53063836115601E-16,1.,4.18922106430579E-64)) ;
#116480=DIRECTION('center_axis',(-1.,0.,0.)) ;
#116481=DIRECTION('ref_axis',(0.,0.,1.)) ;
#116482=DIRECTION('center_axis',(1.,1.53063836115601E-16,0.)) ;
#116483=DIRECTION('ref_axis',(1.53063836115601E-16,-1.,0.)) ;
#116484=DIRECTION('center_axis',(0.,1.,0.)) ;
#116485=DIRECTION('ref_axis',(1.,0.,0.)) ;
#116486=DIRECTION('center_axis',(-1.,-2.16840434497101E-16,0.)) ;
#116487=DIRECTION('ref_axis',(0.,-1.,0.)) ;
#116488=DIRECTION('center_axis',(0.,0.,-1.)) ;
#116489=DIRECTION('ref_axis',(1.,0.,0.)) ;
#116490=DIRECTION('center_axis',(-1.25542992828747E-32,1.020425574104E-16,
1.)) ;
#116491=DIRECTION('ref_axis',(0.,-1.,0.)) ;
#116492=DIRECTION('center_axis',(0.,-1.,0.)) ;
#116493=DIRECTION('ref_axis',(-6.50521303491307E-15,0.,1.)) ;
#116494=DIRECTION('center_axis',(-1.,0.,0.)) ;
#116495=DIRECTION('ref_axis',(0.,0.,-1.)) ;
#116496=DIRECTION('center_axis',(-1.,-1.53063836115601E-16,0.)) ;
#116497=DIRECTION('ref_axis',(0.,-1.,0.)) ;
#116498=DIRECTION('center_axis',(0.,-1.,0.)) ;
#116499=DIRECTION('ref_axis',(0.,0.,1.)) ;
#116500=DIRECTION('center_axis',(0.,0.,-1.)) ;
#116501=DIRECTION('ref_axis',(-1.,0.,0.)) ;
#116502=DIRECTION('center_axis',(0.,0.,-1.)) ;
#116503=DIRECTION('ref_axis',(-1.,0.,0.)) ;
#116504=DIRECTION('center_axis',(1.,1.53063836115601E-16,-3.06472600140763E-33)) ;
#116505=DIRECTION('ref_axis',(-1.53063836115601E-16,1.,4.69098718418678E-49)) ;
#116506=DIRECTION('center_axis',(-1.,0.,0.)) ;
#116507=DIRECTION('ref_axis',(0.,0.,1.)) ;
#116508=DIRECTION('center_axis',(-1.53063836115601E-16,1.,-1.020425574104E-16)) ;
#116509=DIRECTION('ref_axis',(-1.,-1.53063836115601E-16,1.3684555315672E-47)) ;
#116510=DIRECTION('',(1.53063836115601E-16,-1.,1.020425574104E-16)) ;
#116511=DIRECTION('center_axis',(0.,-1.,0.)) ;
#116512=DIRECTION('ref_axis',(0.,0.,-1.)) ;
#116513=DIRECTION('center_axis',(-1.53063836115601E-16,1.,-1.30104260698261E-16)) ;
#116514=DIRECTION('ref_axis',(-1.,-1.53063836115601E-16,1.99142572374599E-32)) ;
#116515=DIRECTION('center_axis',(0.,-1.,0.)) ;
#116516=DIRECTION('ref_axis',(0.,0.,-1.)) ;
#116517=DIRECTION('center_axis',(-1.,-1.53063836115601E-16,2.73691106313441E-48)) ;
#116518=DIRECTION('ref_axis',(1.53063836115601E-16,-1.,-4.18922106430579E-64)) ;
#116519=DIRECTION('center_axis',(1.,2.16840434497101E-16,0.)) ;
#116520=DIRECTION('ref_axis',(2.16840434497101E-16,-1.,0.)) ;
#116521=DIRECTION('center_axis',(-1.,0.,2.16840434497102E-15)) ;
#116522=DIRECTION('ref_axis',(2.16840434497102E-15,0.,1.)) ;
#116523=DIRECTION('center_axis',(-1.,-2.16840434497101E-16,0.)) ;
#116524=DIRECTION('ref_axis',(0.,-1.,0.)) ;
#116525=DIRECTION('center_axis',(0.,0.,1.)) ;
#116526=DIRECTION('ref_axis',(-1.,0.,0.)) ;
#116527=DIRECTION('center_axis',(0.,1.,0.)) ;
#116528=DIRECTION('ref_axis',(1.,0.,0.)) ;
#116529=DIRECTION('center_axis',(0.,1.,0.)) ;
#116530=DIRECTION('ref_axis',(0.,0.,-1.)) ;
#116531=DIRECTION('center_axis',(1.,0.,0.)) ;
#116532=DIRECTION('ref_axis',(0.,-1.,0.)) ;
#116533=DIRECTION('center_axis',(1.,6.50521303491304E-15,0.)) ;
#116534=DIRECTION('ref_axis',(-6.50521303491304E-15,1.,0.)) ;
#116535=DIRECTION('center_axis',(8.67361737988403E-15,1.,0.)) ;
#116536=DIRECTION('ref_axis',(-1.,8.67361737988403E-15,0.)) ;
#116537=DIRECTION('center_axis',(1.2303003375722E-16,-1.,1.020425574104E-16)) ;
#116538=DIRECTION('ref_axis',(1.,1.2303003375722E-16,-1.25542992828747E-32)) ;
#116539=DIRECTION('center_axis',(0.,1.,0.)) ;
#116540=DIRECTION('ref_axis',(0.,0.,1.)) ;
#116541=DIRECTION('center_axis',(0.,1.,0.)) ;
#116542=DIRECTION('ref_axis',(1.,0.,0.)) ;
#116543=DIRECTION('center_axis',(1.,1.2303003375722E-16,0.)) ;
#116544=DIRECTION('ref_axis',(1.2303003375722E-16,-1.,0.)) ;
#116545=DIRECTION('center_axis',(0.,0.,1.)) ;
#116546=DIRECTION('ref_axis',(-1.,0.,0.)) ;
#116547=DIRECTION('center_axis',(0.,1.,0.)) ;
#116548=DIRECTION('ref_axis',(1.,0.,0.)) ;
#116549=DIRECTION('center_axis',(0.,0.,-1.)) ;
#116550=DIRECTION('ref_axis',(1.,0.,0.)) ;
#116551=DIRECTION('center_axis',(0.,0.,-1.)) ;
#116552=DIRECTION('ref_axis',(-1.,0.,0.)) ;
#116553=DIRECTION('center_axis',(0.,0.,1.)) ;
#116554=DIRECTION('ref_axis',(1.,0.,0.)) ;
#116555=DIRECTION('center_axis',(-2.16840434497101E-16,1.,-1.020425574104E-16)) ;
#116556=DIRECTION('ref_axis',(-1.,-2.16840434497101E-16,5.47382212626882E-48)) ;
#116557=DIRECTION('center_axis',(0.,1.,0.)) ;
#116558=DIRECTION('ref_axis',(0.,0.,-1.)) ;
#116559=DIRECTION('center_axis',(1.,0.,1.25542992828747E-32)) ;
#116560=DIRECTION('ref_axis',(1.25542992828747E-32,0.,-1.)) ;
#116561=DIRECTION('center_axis',(1.,0.,0.)) ;
#116562=DIRECTION('ref_axis',(0.,0.,-1.)) ;
#116563=DIRECTION('center_axis',(-1.,-1.2303003375722E-16,0.)) ;
#116564=DIRECTION('ref_axis',(0.,-1.,0.)) ;
#116565=DIRECTION('center_axis',(0.,0.,-1.)) ;
#116566=DIRECTION('ref_axis',(1.,0.,0.)) ;
#116567=DIRECTION('center_axis',(0.,0.,-1.)) ;
#116568=DIRECTION('ref_axis',(-1.,0.,0.)) ;
#116569=DIRECTION('',(0.,0.,1.)) ;
#116570=DIRECTION('center_axis',(0.,0.,1.)) ;
#116571=DIRECTION('ref_axis',(1.,0.,0.)) ;
#116572=DIRECTION('center_axis',(0.,0.,1.)) ;
#116573=DIRECTION('ref_axis',(1.,0.,0.)) ;
#116574=DIRECTION('center_axis',(6.27714964143733E-33,-5.10212787052002E-17,
-1.)) ;
#116575=DIRECTION('ref_axis',(3.20268201330022E-49,1.,-5.10212787052002E-17)) ;
#116576=DIRECTION('center_axis',(1.,1.53063836115601E-16,-1.53236300070382E-33)) ;
#116577=DIRECTION('ref_axis',(-1.53063836115601E-16,1.,2.34549359209339E-49)) ;
#116578=DIRECTION('center_axis',(-1.,0.,0.)) ;
#116579=DIRECTION('ref_axis',(0.,0.,1.)) ;
#116580=DIRECTION('center_axis',(1.,0.,0.)) ;
#116581=DIRECTION('ref_axis',(0.,0.,-1.)) ;
#116582=DIRECTION('center_axis',(0.,1.,0.)) ;
#116583=DIRECTION('ref_axis',(1.,0.,0.)) ;
#116584=DIRECTION('center_axis',(-4.33680868994202E-15,1.,0.)) ;
#116585=DIRECTION('ref_axis',(1.,4.33680868994202E-15,0.)) ;
#116586=DIRECTION('center_axis',(0.,-1.,0.)) ;
#116587=DIRECTION('ref_axis',(0.,0.,-1.)) ;
#116588=DIRECTION('center_axis',(0.,0.,-1.)) ;
#116589=DIRECTION('ref_axis',(1.,0.,0.)) ;
#116590=DIRECTION('center_axis',(0.,0.,1.)) ;
#116591=DIRECTION('ref_axis',(1.,0.,0.)) ;
#116592=DIRECTION('center_axis',(0.,0.,-1.)) ;
#116593=DIRECTION('ref_axis',(-1.,0.,0.)) ;
#116594=DIRECTION('center_axis',(0.,1.,0.)) ;
#116595=DIRECTION('ref_axis',(1.,0.,0.)) ;
#116596=DIRECTION('center_axis',(1.,1.2303003375722E-16,0.)) ;
#116597=DIRECTION('ref_axis',(1.2303003375722E-16,-1.,0.)) ;
#116598=DIRECTION('center_axis',(0.,1.,0.)) ;
#116599=DIRECTION('ref_axis',(-6.50521303491307E-15,0.,-1.)) ;
#116600=DIRECTION('center_axis',(6.27714964143733E-33,-5.10212787052002E-17,
-1.)) ;
#116601=DIRECTION('ref_axis',(0.,1.,0.)) ;
#116602=DIRECTION('center_axis',(0.,-1.,0.)) ;
#116603=DIRECTION('ref_axis',(0.,0.,1.)) ;
#116604=DIRECTION('center_axis',(2.16840434497101E-16,-1.,5.10212787052002E-17)) ;
#116605=DIRECTION('ref_axis',(1.,2.16840434497101E-16,-5.47382212626882E-48)) ;
#116606=DIRECTION('center_axis',(0.,1.,0.)) ;
#116607=DIRECTION('ref_axis',(0.,0.,-1.)) ;
#116608=DIRECTION('center_axis',(0.,0.,1.)) ;
#116609=DIRECTION('ref_axis',(1.,0.,0.)) ;
#116610=DIRECTION('center_axis',(0.,0.,-1.)) ;
#116611=DIRECTION('ref_axis',(-1.,0.,0.)) ;
#116612=DIRECTION('center_axis',(-1.,-1.2303003375722E-16,0.)) ;
#116613=DIRECTION('ref_axis',(0.,-1.,0.)) ;
#116614=DIRECTION('center_axis',(0.,-1.,0.)) ;
#116615=DIRECTION('ref_axis',(0.,0.,1.)) ;
#116616=DIRECTION('center_axis',(1.53063836115601E-16,-1.,5.10212787052002E-17)) ;
#116617=DIRECTION('ref_axis',(1.,1.53063836115601E-16,-6.84227765783602E-48)) ;
#116618=DIRECTION('',(-1.53063836115601E-16,1.,-5.10212787052002E-17)) ;
#116619=DIRECTION('center_axis',(0.,-1.,0.)) ;
#116620=DIRECTION('ref_axis',(0.,0.,-1.)) ;
#116621=DIRECTION('center_axis',(-1.,0.,0.)) ;
#116622=DIRECTION('ref_axis',(0.,0.,-1.)) ;
#116623=DIRECTION('center_axis',(-1.2303003375722E-16,1.,-5.10212787052002E-17)) ;
#116624=DIRECTION('ref_axis',(-1.,-1.2303003375722E-16,6.27714964143733E-33)) ;
#116625=DIRECTION('center_axis',(-8.67361737988403E-15,-1.,0.)) ;
#116626=DIRECTION('ref_axis',(1.,-8.67361737988403E-15,0.)) ;
#116627=DIRECTION('center_axis',(1.,0.,6.27714964143733E-33)) ;
#116628=DIRECTION('ref_axis',(6.27714964143733E-33,0.,-1.)) ;
#116629=DIRECTION('center_axis',(-1.,0.,-6.50521303491307E-15)) ;
#116630=DIRECTION('ref_axis',(-6.50521303491307E-15,0.,1.)) ;
#116631=DIRECTION('center_axis',(1.,0.,0.)) ;
#116632=DIRECTION('ref_axis',(0.,1.,0.)) ;
#116633=DIRECTION('center_axis',(0.,0.,-1.)) ;
#116634=DIRECTION('ref_axis',(-1.,0.,0.)) ;
#116635=DIRECTION('center_axis',(0.,0.,1.)) ;
#116636=DIRECTION('ref_axis',(1.,0.,0.)) ;
#116637=DIRECTION('center_axis',(0.,0.,-1.)) ;
#116638=DIRECTION('ref_axis',(-1.,0.,0.)) ;
#116639=DIRECTION('center_axis',(-1.,0.,0.)) ;
#116640=DIRECTION('ref_axis',(0.,0.,1.)) ;
#116641=DIRECTION('center_axis',(0.,-1.,0.)) ;
#116642=DIRECTION('ref_axis',(0.,0.,-1.)) ;
#116643=DIRECTION('center_axis',(0.,1.,0.)) ;
#116644=DIRECTION('ref_axis',(0.,0.,1.)) ;
#116645=DIRECTION('center_axis',(0.,1.,-6.50521303491307E-15)) ;
#116646=DIRECTION('ref_axis',(0.,6.50521303491307E-15,1.)) ;
#116647=DIRECTION('center_axis',(0.,-1.,0.)) ;
#116648=DIRECTION('ref_axis',(0.,0.,-1.)) ;
#116649=DIRECTION('center_axis',(0.,-1.,0.)) ;
#116650=DIRECTION('ref_axis',(0.,0.,-1.)) ;
#116651=DIRECTION('center_axis',(0.,-1.,-1.07081696047951E-16)) ;
#116652=DIRECTION('ref_axis',(0.,1.07081696047951E-16,-1.)) ;
#116653=DIRECTION('center_axis',(0.,1.,0.)) ;
#116654=DIRECTION('ref_axis',(0.,0.,1.)) ;
#116655=DIRECTION('center_axis',(-1.,0.,0.)) ;
#116656=DIRECTION('ref_axis',(0.,0.,1.)) ;
#116657=DIRECTION('center_axis',(0.,0.,1.)) ;
#116658=DIRECTION('ref_axis',(1.,0.,0.)) ;
#116659=DIRECTION('center_axis',(0.,1.,0.)) ;
#116660=DIRECTION('ref_axis',(0.,0.,1.)) ;
#116661=DIRECTION('center_axis',(0.,0.,-1.)) ;
#116662=DIRECTION('ref_axis',(-1.,0.,0.)) ;
#116663=DIRECTION('center_axis',(0.,0.,1.)) ;
#116664=DIRECTION('ref_axis',(1.,0.,0.)) ;
#116665=DIRECTION('center_axis',(0.,0.,1.)) ;
#116666=DIRECTION('ref_axis',(1.,0.,0.)) ;
#116667=DIRECTION('center_axis',(0.,0.,1.)) ;
#116668=DIRECTION('ref_axis',(1.,0.,0.)) ;
#116669=DIRECTION('center_axis',(0.,0.,-1.)) ;
#116670=DIRECTION('ref_axis',(-1.,0.,0.)) ;
#116671=DIRECTION('center_axis',(0.,1.,0.)) ;
#116672=DIRECTION('ref_axis',(0.,0.,1.)) ;
#116673=DIRECTION('center_axis',(0.,-0.707106781186558,0.707106781186537)) ;
#116674=DIRECTION('ref_axis',(0.,-0.707106781186537,-0.707106781186558)) ;
#116675=DIRECTION('center_axis',(0.,1.,0.)) ;
#116676=DIRECTION('ref_axis',(0.,0.,1.)) ;
#116677=DIRECTION('center_axis',(0.,-0.514231796959093,-0.857651245551607)) ;
#116678=DIRECTION('ref_axis',(0.,0.857651245551607,-0.514231796959093)) ;
#116679=DIRECTION('center_axis',(0.,-0.707106781186548,0.707106781186547)) ;
#116680=DIRECTION('ref_axis',(0.,-0.707106781186547,-0.707106781186548)) ;
#116681=DIRECTION('center_axis',(0.,-0.707106781186548,0.707106781186548)) ;
#116682=DIRECTION('ref_axis',(0.,-0.707106781186548,-0.707106781186548)) ;
#116683=DIRECTION('center_axis',(-1.,0.,0.)) ;
#116684=DIRECTION('ref_axis',(0.,0.,1.)) ;
#116685=DIRECTION('center_axis',(0.,0.514231796959095,-0.857651245551606)) ;
#116686=DIRECTION('ref_axis',(0.,0.857651245551606,0.514231796959095)) ;
#116687=DIRECTION('center_axis',(0.,1.,0.)) ;
#116688=DIRECTION('ref_axis',(0.,0.,1.)) ;
#116689=DIRECTION('center_axis',(0.,0.,-1.)) ;
#116690=DIRECTION('ref_axis',(-1.,0.,0.)) ;
#116691=DIRECTION('center_axis',(0.,1.,0.)) ;
#116692=DIRECTION('ref_axis',(0.,0.,1.)) ;
#116693=DIRECTION('center_axis',(0.,0.,-1.)) ;
#116694=DIRECTION('ref_axis',(-1.,0.,0.)) ;
#116695=DIRECTION('center_axis',(0.,0.,-1.)) ;
#116696=DIRECTION('ref_axis',(-1.,0.,0.)) ;
#116697=DIRECTION('center_axis',(0.,0.,1.)) ;
#116698=DIRECTION('ref_axis',(1.,0.,0.)) ;
#116699=DIRECTION('center_axis',(0.,0.,-1.)) ;
#116700=DIRECTION('ref_axis',(-1.,0.,0.)) ;
#116701=DIRECTION('center_axis',(0.,1.,0.)) ;
#116702=DIRECTION('ref_axis',(0.,0.,1.)) ;
#116703=DIRECTION('center_axis',(0.,-1.,8.67361737988409E-15)) ;
#116704=DIRECTION('ref_axis',(0.,-8.67361737988409E-15,-1.)) ;
#116705=DIRECTION('center_axis',(0.,0.707106781186546,0.707106781186549)) ;
#116706=DIRECTION('ref_axis',(0.,-0.707106781186549,0.707106781186546)) ;
#116707=DIRECTION('center_axis',(0.,0.707106781186537,0.707106781186558)) ;
#116708=DIRECTION('ref_axis',(0.,-0.707106781186558,0.707106781186537)) ;
#116709=DIRECTION('center_axis',(0.,1.,1.07081696047951E-16)) ;
#116710=DIRECTION('ref_axis',(0.,-1.07081696047951E-16,1.)) ;
#116711=DIRECTION('center_axis',(0.,-1.,0.)) ;
#116712=DIRECTION('ref_axis',(0.,0.,-1.)) ;
#116713=DIRECTION('center_axis',(0.,1.,0.)) ;
#116714=DIRECTION('ref_axis',(0.,0.,1.)) ;
#116715=DIRECTION('center_axis',(0.,0.,1.)) ;
#116716=DIRECTION('ref_axis',(1.,0.,0.)) ;
#116717=DIRECTION('center_axis',(0.,1.,0.)) ;
#116718=DIRECTION('ref_axis',(0.,0.,1.)) ;
#116719=DIRECTION('center_axis',(0.,0.,1.)) ;
#116720=DIRECTION('ref_axis',(1.,0.,0.)) ;
#116721=DIRECTION('center_axis',(0.,3.99416362155027E-15,1.)) ;
#116722=DIRECTION('ref_axis',(0.,-1.,3.99416362155027E-15)) ;
#116723=DIRECTION('center_axis',(0.,0.,1.)) ;
#116724=DIRECTION('ref_axis',(1.,0.,0.)) ;
#116725=DIRECTION('center_axis',(0.,0.,-1.)) ;
#116726=DIRECTION('ref_axis',(-1.,0.,0.)) ;
#116727=DIRECTION('center_axis',(0.,0.,1.)) ;
#116728=DIRECTION('ref_axis',(1.,0.,0.)) ;
#116729=DIRECTION('center_axis',(-1.,0.,0.)) ;
#116730=DIRECTION('ref_axis',(0.,0.,1.)) ;
#116731=DIRECTION('center_axis',(0.,1.,0.)) ;
#116732=DIRECTION('ref_axis',(0.,0.,1.)) ;
#116733=DIRECTION('center_axis',(-1.,0.,0.)) ;
#116734=DIRECTION('ref_axis',(0.,0.,1.)) ;
#116735=DIRECTION('center_axis',(0.,-1.,0.)) ;
#116736=DIRECTION('ref_axis',(0.,0.,-1.)) ;
#116737=DIRECTION('center_axis',(0.,1.,0.)) ;
#116738=DIRECTION('ref_axis',(0.,0.,1.)) ;
#116739=DIRECTION('center_axis',(1.53063836115601E-16,-1.,-1.30104260698261E-16)) ;
#116740=DIRECTION('ref_axis',(1.,1.53063836115601E-16,1.99142572374599E-32)) ;
#116741=DIRECTION('center_axis',(0.,1.,0.)) ;
#116742=DIRECTION('ref_axis',(0.,0.,1.)) ;
#116743=DIRECTION('center_axis',(0.,-1.,0.)) ;
#116744=DIRECTION('ref_axis',(0.,0.,-1.)) ;
#116745=DIRECTION('center_axis',(1.,1.53063836115601E-16,2.73691106313441E-48)) ;
#116746=DIRECTION('ref_axis',(-1.53063836115601E-16,1.,-4.18922106430579E-64)) ;
#116747=DIRECTION('center_axis',(-1.,0.,0.)) ;
#116748=DIRECTION('ref_axis',(0.,0.,1.)) ;
#116749=DIRECTION('center_axis',(1.,1.53063836115601E-16,0.)) ;
#116750=DIRECTION('ref_axis',(1.53063836115601E-16,-1.,0.)) ;
#116751=DIRECTION('center_axis',(0.,1.,0.)) ;
#116752=DIRECTION('ref_axis',(1.,0.,0.)) ;
#116753=DIRECTION('center_axis',(0.,1.,0.)) ;
#116754=DIRECTION('ref_axis',(0.,0.,-1.)) ;
#116755=DIRECTION('center_axis',(0.,0.,1.)) ;
#116756=DIRECTION('ref_axis',(-1.,0.,0.)) ;
#116757=DIRECTION('center_axis',(0.,1.,0.)) ;
#116758=DIRECTION('ref_axis',(1.,0.,0.)) ;
#116759=DIRECTION('center_axis',(0.,0.,1.)) ;
#116760=DIRECTION('ref_axis',(-1.,0.,0.)) ;
#116761=DIRECTION('center_axis',(1.,1.0842021724855E-15,0.)) ;
#116762=DIRECTION('ref_axis',(1.0842021724855E-15,-1.,0.)) ;
#116763=DIRECTION('center_axis',(-1.,-1.53063836115601E-16,0.)) ;
#116764=DIRECTION('ref_axis',(0.,-1.,0.)) ;
#116765=DIRECTION('center_axis',(0.,0.,-1.)) ;
#116766=DIRECTION('ref_axis',(1.,0.,0.)) ;
#116767=DIRECTION('center_axis',(0.,0.,-1.)) ;
#116768=DIRECTION('ref_axis',(0.804034447892627,0.594582716366695,0.)) ;
#116769=DIRECTION('center_axis',(0.,0.,1.)) ;
#116770=DIRECTION('ref_axis',(1.,0.,0.)) ;
#116771=DIRECTION('',(0.,0.,-1.)) ;
#116772=DIRECTION('center_axis',(-2.16840434497101E-16,1.,1.30104260698261E-16)) ;
#116773=DIRECTION('ref_axis',(1.,2.16840434497101E-16,1.22464679914735E-16)) ;
#116774=DIRECTION('',(-2.16840434497101E-16,1.,1.30104260698261E-16)) ;
#116775=DIRECTION('center_axis',(0.,1.,0.)) ;
#116776=DIRECTION('ref_axis',(0.,0.,1.)) ;
#116777=DIRECTION('center_axis',(-1.,-1.53063836115601E-16,-2.73691106313441E-48)) ;
#116778=DIRECTION('ref_axis',(1.53063836115601E-16,-1.,4.18922106430579E-64)) ;
#116779=DIRECTION('center_axis',(1.,2.16840434497101E-16,0.)) ;
#116780=DIRECTION('ref_axis',(2.16840434497101E-16,-1.,0.)) ;
#116781=DIRECTION('center_axis',(0.,0.,1.)) ;
#116782=DIRECTION('ref_axis',(1.,0.,0.)) ;
#116783=DIRECTION('center_axis',(-1.25542992828747E-32,1.020425574104E-16,
1.)) ;
#116784=DIRECTION('ref_axis',(-1.28107280532009E-48,-1.,1.020425574104E-16)) ;
#116785=DIRECTION('center_axis',(0.,0.,1.)) ;
#116786=DIRECTION('ref_axis',(1.,0.,0.)) ;
#116787=DIRECTION('center_axis',(0.,0.,-1.)) ;
#116788=DIRECTION('ref_axis',(-1.,0.,0.)) ;
#116789=DIRECTION('center_axis',(1.,1.53063836115601E-16,-2.73691106313441E-48)) ;
#116790=DIRECTION('ref_axis',(-1.53063836115601E-16,1.,4.18922106430579E-64)) ;
#116791=DIRECTION('center_axis',(-1.,0.,0.)) ;
#116792=DIRECTION('ref_axis',(0.,0.,1.)) ;
#116793=DIRECTION('center_axis',(1.,1.53063836115601E-16,0.)) ;
#116794=DIRECTION('ref_axis',(1.53063836115601E-16,-1.,0.)) ;
#116795=DIRECTION('center_axis',(0.,1.,0.)) ;
#116796=DIRECTION('ref_axis',(1.,0.,0.)) ;
#116797=DIRECTION('center_axis',(-1.,-2.16840434497101E-16,0.)) ;
#116798=DIRECTION('ref_axis',(0.,-1.,0.)) ;
#116799=DIRECTION('center_axis',(0.,0.,-1.)) ;
#116800=DIRECTION('ref_axis',(1.,0.,0.)) ;
#116801=DIRECTION('center_axis',(-1.25542992828747E-32,1.020425574104E-16,
1.)) ;
#116802=DIRECTION('ref_axis',(0.,-1.,0.)) ;
#116803=DIRECTION('center_axis',(0.,-1.,0.)) ;
#116804=DIRECTION('ref_axis',(-6.50521303491307E-15,0.,1.)) ;
#116805=DIRECTION('center_axis',(-1.,0.,0.)) ;
#116806=DIRECTION('ref_axis',(0.,0.,-1.)) ;
#116807=DIRECTION('center_axis',(-1.,-1.53063836115601E-16,0.)) ;
#116808=DIRECTION('ref_axis',(0.,-1.,0.)) ;
#116809=DIRECTION('center_axis',(0.,-1.,0.)) ;
#116810=DIRECTION('ref_axis',(0.,0.,1.)) ;
#116811=DIRECTION('center_axis',(0.,0.,-1.)) ;
#116812=DIRECTION('ref_axis',(-1.,0.,0.)) ;
#116813=DIRECTION('center_axis',(0.,0.,-1.)) ;
#116814=DIRECTION('ref_axis',(-1.,0.,0.)) ;
#116815=DIRECTION('center_axis',(1.,1.53063836115601E-16,-3.06472600140763E-33)) ;
#116816=DIRECTION('ref_axis',(-1.53063836115601E-16,1.,4.69098718418678E-49)) ;
#116817=DIRECTION('center_axis',(-1.,0.,0.)) ;
#116818=DIRECTION('ref_axis',(0.,0.,1.)) ;
#116819=DIRECTION('center_axis',(-1.53063836115601E-16,1.,-1.020425574104E-16)) ;
#116820=DIRECTION('ref_axis',(-1.,-1.53063836115601E-16,1.3684555315672E-47)) ;
#116821=DIRECTION('',(1.53063836115601E-16,-1.,1.020425574104E-16)) ;
#116822=DIRECTION('center_axis',(0.,-1.,0.)) ;
#116823=DIRECTION('ref_axis',(0.,0.,-1.)) ;
#116824=DIRECTION('center_axis',(-1.53063836115601E-16,1.,-1.30104260698261E-16)) ;
#116825=DIRECTION('ref_axis',(-1.,-1.53063836115601E-16,1.99142572374599E-32)) ;
#116826=DIRECTION('center_axis',(0.,-1.,0.)) ;
#116827=DIRECTION('ref_axis',(0.,0.,-1.)) ;
#116828=DIRECTION('center_axis',(-1.,-1.53063836115601E-16,2.73691106313441E-48)) ;
#116829=DIRECTION('ref_axis',(1.53063836115601E-16,-1.,-4.18922106430579E-64)) ;
#116830=DIRECTION('center_axis',(1.,2.16840434497101E-16,0.)) ;
#116831=DIRECTION('ref_axis',(2.16840434497101E-16,-1.,0.)) ;
#116832=DIRECTION('center_axis',(-1.,0.,2.16840434497102E-15)) ;
#116833=DIRECTION('ref_axis',(2.16840434497102E-15,0.,1.)) ;
#116834=DIRECTION('center_axis',(-1.,-2.16840434497101E-16,0.)) ;
#116835=DIRECTION('ref_axis',(0.,-1.,0.)) ;
#116836=DIRECTION('center_axis',(0.,0.,1.)) ;
#116837=DIRECTION('ref_axis',(-1.,0.,0.)) ;
#116838=DIRECTION('center_axis',(0.,1.,0.)) ;
#116839=DIRECTION('ref_axis',(1.,0.,0.)) ;
#116840=DIRECTION('center_axis',(0.,1.,0.)) ;
#116841=DIRECTION('ref_axis',(0.,0.,-1.)) ;
#116842=DIRECTION('center_axis',(1.,0.,0.)) ;
#116843=DIRECTION('ref_axis',(0.,-1.,0.)) ;
#116844=DIRECTION('center_axis',(1.,6.50521303491304E-15,0.)) ;
#116845=DIRECTION('ref_axis',(-6.50521303491304E-15,1.,0.)) ;
#116846=DIRECTION('center_axis',(8.67361737988403E-15,1.,0.)) ;
#116847=DIRECTION('ref_axis',(-1.,8.67361737988403E-15,0.)) ;
#116848=DIRECTION('center_axis',(1.2303003375722E-16,-1.,1.020425574104E-16)) ;
#116849=DIRECTION('ref_axis',(1.,1.2303003375722E-16,-1.25542992828747E-32)) ;
#116850=DIRECTION('center_axis',(0.,1.,0.)) ;
#116851=DIRECTION('ref_axis',(0.,0.,1.)) ;
#116852=DIRECTION('center_axis',(0.,1.,0.)) ;
#116853=DIRECTION('ref_axis',(1.,0.,0.)) ;
#116854=DIRECTION('center_axis',(1.,1.2303003375722E-16,0.)) ;
#116855=DIRECTION('ref_axis',(1.2303003375722E-16,-1.,0.)) ;
#116856=DIRECTION('center_axis',(0.,0.,1.)) ;
#116857=DIRECTION('ref_axis',(-1.,0.,0.)) ;
#116858=DIRECTION('center_axis',(0.,1.,0.)) ;
#116859=DIRECTION('ref_axis',(1.,0.,0.)) ;
#116860=DIRECTION('center_axis',(0.,0.,-1.)) ;
#116861=DIRECTION('ref_axis',(1.,0.,0.)) ;
#116862=DIRECTION('center_axis',(0.,0.,-1.)) ;
#116863=DIRECTION('ref_axis',(-1.,0.,0.)) ;
#116864=DIRECTION('center_axis',(0.,0.,1.)) ;
#116865=DIRECTION('ref_axis',(1.,0.,0.)) ;
#116866=DIRECTION('center_axis',(-2.16840434497101E-16,1.,-1.020425574104E-16)) ;
#116867=DIRECTION('ref_axis',(-1.,-2.16840434497101E-16,5.47382212626882E-48)) ;
#116868=DIRECTION('center_axis',(0.,1.,0.)) ;
#116869=DIRECTION('ref_axis',(0.,0.,-1.)) ;
#116870=DIRECTION('center_axis',(1.,0.,1.25542992828747E-32)) ;
#116871=DIRECTION('ref_axis',(1.25542992828747E-32,0.,-1.)) ;
#116872=DIRECTION('center_axis',(1.,0.,0.)) ;
#116873=DIRECTION('ref_axis',(0.,0.,-1.)) ;
#116874=DIRECTION('center_axis',(-1.,-1.2303003375722E-16,0.)) ;
#116875=DIRECTION('ref_axis',(0.,-1.,0.)) ;
#116876=DIRECTION('center_axis',(0.,0.,-1.)) ;
#116877=DIRECTION('ref_axis',(1.,0.,0.)) ;
#116878=DIRECTION('center_axis',(0.,0.,-1.)) ;
#116879=DIRECTION('ref_axis',(-1.,0.,0.)) ;
#116880=DIRECTION('',(0.,0.,1.)) ;
#116881=DIRECTION('center_axis',(0.,0.,1.)) ;
#116882=DIRECTION('ref_axis',(1.,0.,0.)) ;
#116883=DIRECTION('center_axis',(0.,0.,1.)) ;
#116884=DIRECTION('ref_axis',(1.,0.,0.)) ;
#116885=DIRECTION('center_axis',(6.27714964143733E-33,-5.10212787052002E-17,
-1.)) ;
#116886=DIRECTION('ref_axis',(3.20268201330022E-49,1.,-5.10212787052002E-17)) ;
#116887=DIRECTION('center_axis',(1.,1.53063836115601E-16,-1.53236300070382E-33)) ;
#116888=DIRECTION('ref_axis',(-1.53063836115601E-16,1.,2.34549359209339E-49)) ;
#116889=DIRECTION('center_axis',(-1.,0.,0.)) ;
#116890=DIRECTION('ref_axis',(0.,0.,1.)) ;
#116891=DIRECTION('center_axis',(1.,0.,0.)) ;
#116892=DIRECTION('ref_axis',(0.,0.,-1.)) ;
#116893=DIRECTION('center_axis',(0.,1.,0.)) ;
#116894=DIRECTION('ref_axis',(1.,0.,0.)) ;
#116895=DIRECTION('center_axis',(-4.33680868994202E-15,1.,0.)) ;
#116896=DIRECTION('ref_axis',(1.,4.33680868994202E-15,0.)) ;
#116897=DIRECTION('center_axis',(0.,-1.,0.)) ;
#116898=DIRECTION('ref_axis',(0.,0.,-1.)) ;
#116899=DIRECTION('center_axis',(0.,0.,-1.)) ;
#116900=DIRECTION('ref_axis',(1.,0.,0.)) ;
#116901=DIRECTION('center_axis',(0.,0.,1.)) ;
#116902=DIRECTION('ref_axis',(1.,0.,0.)) ;
#116903=DIRECTION('center_axis',(0.,0.,-1.)) ;
#116904=DIRECTION('ref_axis',(-1.,0.,0.)) ;
#116905=DIRECTION('center_axis',(0.,1.,0.)) ;
#116906=DIRECTION('ref_axis',(1.,0.,0.)) ;
#116907=DIRECTION('center_axis',(1.,1.2303003375722E-16,0.)) ;
#116908=DIRECTION('ref_axis',(1.2303003375722E-16,-1.,0.)) ;
#116909=DIRECTION('center_axis',(0.,1.,0.)) ;
#116910=DIRECTION('ref_axis',(-6.50521303491284E-15,0.,-1.)) ;
#116911=DIRECTION('center_axis',(6.27714964143733E-33,-5.10212787052002E-17,
-1.)) ;
#116912=DIRECTION('ref_axis',(0.,1.,0.)) ;
#116913=DIRECTION('center_axis',(0.,-1.,0.)) ;
#116914=DIRECTION('ref_axis',(0.,0.,1.)) ;
#116915=DIRECTION('center_axis',(2.16840434497101E-16,-1.,5.10212787052002E-17)) ;
#116916=DIRECTION('ref_axis',(1.,2.16840434497101E-16,-5.47382212626882E-48)) ;
#116917=DIRECTION('center_axis',(0.,1.,0.)) ;
#116918=DIRECTION('ref_axis',(0.,0.,-1.)) ;
#116919=DIRECTION('center_axis',(0.,0.,1.)) ;
#116920=DIRECTION('ref_axis',(1.,0.,0.)) ;
#116921=DIRECTION('center_axis',(0.,0.,-1.)) ;
#116922=DIRECTION('ref_axis',(-1.,0.,0.)) ;
#116923=DIRECTION('center_axis',(-1.,-1.2303003375722E-16,0.)) ;
#116924=DIRECTION('ref_axis',(0.,-1.,0.)) ;
#116925=DIRECTION('center_axis',(0.,-1.,0.)) ;
#116926=DIRECTION('ref_axis',(0.,0.,1.)) ;
#116927=DIRECTION('center_axis',(1.53063836115601E-16,-1.,5.10212787052002E-17)) ;
#116928=DIRECTION('ref_axis',(1.,1.53063836115601E-16,-6.84227765783602E-48)) ;
#116929=DIRECTION('',(-1.53063836115601E-16,1.,-5.10212787052002E-17)) ;
#116930=DIRECTION('center_axis',(0.,-1.,0.)) ;
#116931=DIRECTION('ref_axis',(0.,0.,-1.)) ;
#116932=DIRECTION('center_axis',(-1.,0.,0.)) ;
#116933=DIRECTION('ref_axis',(0.,0.,-1.)) ;
#116934=DIRECTION('center_axis',(-1.2303003375722E-16,1.,-5.10212787052002E-17)) ;
#116935=DIRECTION('ref_axis',(-1.,-1.2303003375722E-16,6.27714964143733E-33)) ;
#116936=DIRECTION('center_axis',(-8.67361737988403E-15,-1.,0.)) ;
#116937=DIRECTION('ref_axis',(1.,-8.67361737988403E-15,0.)) ;
#116938=DIRECTION('center_axis',(1.,0.,6.27714964143733E-33)) ;
#116939=DIRECTION('ref_axis',(6.27714964143733E-33,0.,-1.)) ;
#116940=DIRECTION('center_axis',(-1.,0.,-6.50521303491284E-15)) ;
#116941=DIRECTION('ref_axis',(-6.50521303491284E-15,0.,1.)) ;
#116942=DIRECTION('center_axis',(1.,0.,0.)) ;
#116943=DIRECTION('ref_axis',(0.,1.,0.)) ;
#116944=DIRECTION('center_axis',(0.,0.,-1.)) ;
#116945=DIRECTION('ref_axis',(-1.,0.,0.)) ;
#116946=DIRECTION('center_axis',(0.,0.,1.)) ;
#116947=DIRECTION('ref_axis',(1.,0.,0.)) ;
#116948=DIRECTION('center_axis',(0.,0.,-1.)) ;
#116949=DIRECTION('ref_axis',(-1.,0.,0.)) ;
#116950=DIRECTION('center_axis',(-1.,0.,0.)) ;
#116951=DIRECTION('ref_axis',(0.,0.,1.)) ;
#116952=DIRECTION('center_axis',(0.,-1.,0.)) ;
#116953=DIRECTION('ref_axis',(0.,0.,-1.)) ;
#116954=DIRECTION('center_axis',(0.,1.,0.)) ;
#116955=DIRECTION('ref_axis',(0.,0.,1.)) ;
#116956=DIRECTION('center_axis',(0.,1.,-6.50521303491284E-15)) ;
#116957=DIRECTION('ref_axis',(0.,6.50521303491284E-15,1.)) ;
#116958=DIRECTION('center_axis',(0.,-1.,0.)) ;
#116959=DIRECTION('ref_axis',(0.,0.,-1.)) ;
#116960=DIRECTION('center_axis',(0.,-1.,0.)) ;
#116961=DIRECTION('ref_axis',(0.,0.,-1.)) ;
#116962=DIRECTION('center_axis',(0.,-1.,-1.07081696047951E-16)) ;
#116963=DIRECTION('ref_axis',(0.,1.07081696047951E-16,-1.)) ;
#116964=DIRECTION('center_axis',(0.,1.,0.)) ;
#116965=DIRECTION('ref_axis',(0.,0.,1.)) ;
#116966=DIRECTION('center_axis',(-1.,0.,0.)) ;
#116967=DIRECTION('ref_axis',(0.,0.,1.)) ;
#116968=DIRECTION('center_axis',(0.,0.,1.)) ;
#116969=DIRECTION('ref_axis',(1.,0.,0.)) ;
#116970=DIRECTION('center_axis',(0.,1.,0.)) ;
#116971=DIRECTION('ref_axis',(0.,0.,1.)) ;
#116972=DIRECTION('center_axis',(0.,0.,-1.)) ;
#116973=DIRECTION('ref_axis',(-1.,0.,0.)) ;
#116974=DIRECTION('center_axis',(0.,0.,1.)) ;
#116975=DIRECTION('ref_axis',(1.,0.,0.)) ;
#116976=DIRECTION('center_axis',(0.,0.,1.)) ;
#116977=DIRECTION('ref_axis',(1.,0.,0.)) ;
#116978=DIRECTION('center_axis',(0.,0.,1.)) ;
#116979=DIRECTION('ref_axis',(1.,0.,0.)) ;
#116980=DIRECTION('center_axis',(0.,0.,-1.)) ;
#116981=DIRECTION('ref_axis',(-1.,0.,0.)) ;
#116982=DIRECTION('center_axis',(0.,1.,0.)) ;
#116983=DIRECTION('ref_axis',(0.,0.,1.)) ;
#116984=DIRECTION('center_axis',(0.,-0.707106781186532,0.707106781186563)) ;
#116985=DIRECTION('ref_axis',(0.,-0.707106781186563,-0.707106781186532)) ;
#116986=DIRECTION('center_axis',(0.,1.,0.)) ;
#116987=DIRECTION('ref_axis',(0.,0.,1.)) ;
#116988=DIRECTION('center_axis',(2.23012492569655E-15,-0.51423179695906,
-0.857651245551627)) ;
#116989=DIRECTION('ref_axis',(2.6714619735869E-30,0.857651245551626,-0.51423179695906)) ;
#116990=DIRECTION('center_axis',(0.,-0.707106781186548,0.707106781186547)) ;
#116991=DIRECTION('ref_axis',(0.,-0.707106781186547,-0.707106781186548)) ;
#116992=DIRECTION('center_axis',(0.,-0.707106781186541,0.707106781186554)) ;
#116993=DIRECTION('ref_axis',(0.,-0.707106781186554,-0.707106781186541)) ;
#116994=DIRECTION('center_axis',(-1.,0.,0.)) ;
#116995=DIRECTION('ref_axis',(0.,0.,1.)) ;
#116996=DIRECTION('center_axis',(0.,0.514231796959095,-0.857651245551606)) ;
#116997=DIRECTION('ref_axis',(0.,0.857651245551606,0.514231796959095)) ;
#116998=DIRECTION('center_axis',(0.,1.,0.)) ;
#116999=DIRECTION('ref_axis',(0.,0.,1.)) ;
#117000=DIRECTION('center_axis',(0.,0.,-1.)) ;
#117001=DIRECTION('ref_axis',(-1.,0.,0.)) ;
#117002=DIRECTION('center_axis',(0.,1.,0.)) ;
#117003=DIRECTION('ref_axis',(0.,0.,1.)) ;
#117004=DIRECTION('center_axis',(0.,0.,-1.)) ;
#117005=DIRECTION('ref_axis',(-1.,0.,0.)) ;
#117006=DIRECTION('center_axis',(0.,0.,-1.)) ;
#117007=DIRECTION('ref_axis',(-1.,0.,0.)) ;
#117008=DIRECTION('center_axis',(0.,0.,1.)) ;
#117009=DIRECTION('ref_axis',(1.,0.,0.)) ;
#117010=DIRECTION('center_axis',(0.,0.,-1.)) ;
#117011=DIRECTION('ref_axis',(-1.,0.,0.)) ;
#117012=DIRECTION('center_axis',(0.,1.,0.)) ;
#117013=DIRECTION('ref_axis',(0.,0.,1.)) ;
#117014=DIRECTION('center_axis',(0.,-1.,8.67361737988409E-15)) ;
#117015=DIRECTION('ref_axis',(0.,-8.67361737988409E-15,-1.)) ;
#117016=DIRECTION('center_axis',(0.,0.707106781186546,0.707106781186549)) ;
#117017=DIRECTION('ref_axis',(0.,-0.707106781186549,0.707106781186546)) ;
#117018=DIRECTION('center_axis',(0.,0.707106781186537,0.707106781186558)) ;
#117019=DIRECTION('ref_axis',(0.,-0.707106781186558,0.707106781186537)) ;
#117020=DIRECTION('center_axis',(0.,1.,1.07081696047951E-16)) ;
#117021=DIRECTION('ref_axis',(0.,-1.07081696047951E-16,1.)) ;
#117022=DIRECTION('center_axis',(0.,-1.,0.)) ;
#117023=DIRECTION('ref_axis',(0.,0.,-1.)) ;
#117024=DIRECTION('center_axis',(0.,1.,0.)) ;
#117025=DIRECTION('ref_axis',(0.,0.,1.)) ;
#117026=DIRECTION('center_axis',(0.,0.,1.)) ;
#117027=DIRECTION('ref_axis',(1.,0.,0.)) ;
#117028=DIRECTION('center_axis',(0.,1.,0.)) ;
#117029=DIRECTION('ref_axis',(0.,0.,1.)) ;
#117030=DIRECTION('center_axis',(0.,0.,1.)) ;
#117031=DIRECTION('ref_axis',(1.,0.,0.)) ;
#117032=DIRECTION('center_axis',(0.,3.99416362155027E-15,1.)) ;
#117033=DIRECTION('ref_axis',(0.,-1.,3.99416362155027E-15)) ;
#117034=DIRECTION('center_axis',(0.,0.,1.)) ;
#117035=DIRECTION('ref_axis',(1.,0.,0.)) ;
#117036=DIRECTION('center_axis',(0.,0.,-1.)) ;
#117037=DIRECTION('ref_axis',(-1.,0.,0.)) ;
#117038=DIRECTION('center_axis',(0.,0.,1.)) ;
#117039=DIRECTION('ref_axis',(1.,0.,0.)) ;
#117040=DIRECTION('center_axis',(-1.,0.,0.)) ;
#117041=DIRECTION('ref_axis',(0.,0.,1.)) ;
#117042=DIRECTION('center_axis',(0.,1.,0.)) ;
#117043=DIRECTION('ref_axis',(0.,0.,1.)) ;
#117044=DIRECTION('center_axis',(-1.,0.,0.)) ;
#117045=DIRECTION('ref_axis',(0.,0.,1.)) ;
#117046=DIRECTION('center_axis',(0.,-1.,0.)) ;
#117047=DIRECTION('ref_axis',(0.,0.,-1.)) ;
#117048=DIRECTION('center_axis',(0.,1.,0.)) ;
#117049=DIRECTION('ref_axis',(0.,0.,1.)) ;
#117050=DIRECTION('center_axis',(1.53063836115601E-16,-1.,-1.30104260698261E-16)) ;
#117051=DIRECTION('ref_axis',(1.,1.53063836115601E-16,1.99142572374599E-32)) ;
#117052=DIRECTION('center_axis',(0.,1.,0.)) ;
#117053=DIRECTION('ref_axis',(0.,0.,1.)) ;
#117054=DIRECTION('center_axis',(0.,-1.,0.)) ;
#117055=DIRECTION('ref_axis',(0.,0.,-1.)) ;
#117056=DIRECTION('center_axis',(1.,1.53063836115601E-16,2.73691106313441E-48)) ;
#117057=DIRECTION('ref_axis',(-1.53063836115601E-16,1.,-4.18922106430579E-64)) ;
#117058=DIRECTION('center_axis',(-1.,0.,0.)) ;
#117059=DIRECTION('ref_axis',(0.,0.,1.)) ;
#117060=DIRECTION('center_axis',(1.,1.53063836115601E-16,0.)) ;
#117061=DIRECTION('ref_axis',(1.53063836115601E-16,-1.,0.)) ;
#117062=DIRECTION('center_axis',(0.,1.,0.)) ;
#117063=DIRECTION('ref_axis',(1.,0.,0.)) ;
#117064=DIRECTION('center_axis',(0.,1.,0.)) ;
#117065=DIRECTION('ref_axis',(0.,0.,-1.)) ;
#117066=DIRECTION('center_axis',(0.,0.,1.)) ;
#117067=DIRECTION('ref_axis',(-1.,0.,0.)) ;
#117068=DIRECTION('center_axis',(0.,1.,0.)) ;
#117069=DIRECTION('ref_axis',(1.,0.,0.)) ;
#117070=DIRECTION('center_axis',(0.,0.,1.)) ;
#117071=DIRECTION('ref_axis',(-1.,0.,0.)) ;
#117072=DIRECTION('center_axis',(1.,1.0842021724855E-15,0.)) ;
#117073=DIRECTION('ref_axis',(1.0842021724855E-15,-1.,0.)) ;
#117074=DIRECTION('center_axis',(-1.,-1.53063836115601E-16,0.)) ;
#117075=DIRECTION('ref_axis',(0.,-1.,0.)) ;
#117076=DIRECTION('center_axis',(0.,0.,-1.)) ;
#117077=DIRECTION('ref_axis',(1.,0.,0.)) ;
#117078=DIRECTION('center_axis',(0.,0.,-1.)) ;
#117079=DIRECTION('ref_axis',(0.804034447892622,0.594582716366703,0.)) ;
#117080=DIRECTION('center_axis',(0.,0.,1.)) ;
#117081=DIRECTION('ref_axis',(1.,0.,0.)) ;
#117082=DIRECTION('',(0.,0.,-1.)) ;
#117083=DIRECTION('center_axis',(-2.16840434497101E-16,1.,1.30104260698261E-16)) ;
#117084=DIRECTION('ref_axis',(1.,2.16840434497101E-16,1.22464679914735E-16)) ;
#117085=DIRECTION('',(-2.16840434497101E-16,1.,1.30104260698261E-16)) ;
#117086=DIRECTION('center_axis',(0.,1.,0.)) ;
#117087=DIRECTION('ref_axis',(0.,0.,1.)) ;
#117088=DIRECTION('center_axis',(-1.,-1.53063836115601E-16,-2.73691106313441E-48)) ;
#117089=DIRECTION('ref_axis',(1.53063836115601E-16,-1.,4.18922106430579E-64)) ;
#117090=DIRECTION('center_axis',(1.,2.16840434497101E-16,0.)) ;
#117091=DIRECTION('ref_axis',(2.16840434497101E-16,-1.,0.)) ;
#117092=DIRECTION('center_axis',(0.,0.,1.)) ;
#117093=DIRECTION('ref_axis',(1.,0.,0.)) ;
#117094=DIRECTION('center_axis',(-1.25542992828747E-32,1.020425574104E-16,
1.)) ;
#117095=DIRECTION('ref_axis',(-1.28107280532009E-48,-1.,1.020425574104E-16)) ;
#117096=DIRECTION('center_axis',(0.,0.,1.)) ;
#117097=DIRECTION('ref_axis',(1.,0.,0.)) ;
#117098=DIRECTION('center_axis',(0.,0.,-1.)) ;
#117099=DIRECTION('ref_axis',(-1.,0.,0.)) ;
#117100=DIRECTION('center_axis',(1.,1.53063836115601E-16,-2.73691106313441E-48)) ;
#117101=DIRECTION('ref_axis',(-1.53063836115601E-16,1.,4.18922106430579E-64)) ;
#117102=DIRECTION('center_axis',(-1.,0.,0.)) ;
#117103=DIRECTION('ref_axis',(0.,0.,1.)) ;
#117104=DIRECTION('center_axis',(1.,1.53063836115601E-16,0.)) ;
#117105=DIRECTION('ref_axis',(1.53063836115601E-16,-1.,0.)) ;
#117106=DIRECTION('center_axis',(0.,1.,0.)) ;
#117107=DIRECTION('ref_axis',(1.,0.,0.)) ;
#117108=DIRECTION('center_axis',(-1.,-2.16840434497101E-16,0.)) ;
#117109=DIRECTION('ref_axis',(0.,-1.,0.)) ;
#117110=DIRECTION('center_axis',(0.,0.,-1.)) ;
#117111=DIRECTION('ref_axis',(1.,0.,0.)) ;
#117112=DIRECTION('center_axis',(-1.25542992828747E-32,1.020425574104E-16,
1.)) ;
#117113=DIRECTION('ref_axis',(0.,-1.,0.)) ;
#117114=DIRECTION('center_axis',(0.,-1.,0.)) ;
#117115=DIRECTION('ref_axis',(-6.50521303491284E-15,0.,1.)) ;
#117116=DIRECTION('center_axis',(-1.,0.,0.)) ;
#117117=DIRECTION('ref_axis',(0.,0.,-1.)) ;
#117118=DIRECTION('center_axis',(-1.,-1.53063836115601E-16,0.)) ;
#117119=DIRECTION('ref_axis',(0.,-1.,0.)) ;
#117120=DIRECTION('center_axis',(0.,-1.,0.)) ;
#117121=DIRECTION('ref_axis',(0.,0.,1.)) ;
#117122=DIRECTION('center_axis',(0.,0.,-1.)) ;
#117123=DIRECTION('ref_axis',(-1.,0.,0.)) ;
#117124=DIRECTION('center_axis',(0.,0.,-1.)) ;
#117125=DIRECTION('ref_axis',(-1.,0.,0.)) ;
#117126=DIRECTION('center_axis',(1.,1.53063836115601E-16,-3.06472600140763E-33)) ;
#117127=DIRECTION('ref_axis',(-1.53063836115601E-16,1.,4.69098718418678E-49)) ;
#117128=DIRECTION('center_axis',(-1.,0.,0.)) ;
#117129=DIRECTION('ref_axis',(0.,0.,1.)) ;
#117130=DIRECTION('center_axis',(-1.53063836115601E-16,1.,-1.020425574104E-16)) ;
#117131=DIRECTION('ref_axis',(-1.,-1.53063836115601E-16,1.3684555315672E-47)) ;
#117132=DIRECTION('',(1.53063836115601E-16,-1.,1.020425574104E-16)) ;
#117133=DIRECTION('center_axis',(0.,-1.,0.)) ;
#117134=DIRECTION('ref_axis',(0.,0.,-1.)) ;
#117135=DIRECTION('center_axis',(-1.53063836115601E-16,1.,-1.30104260698261E-16)) ;
#117136=DIRECTION('ref_axis',(-1.,-1.53063836115601E-16,1.99142572374599E-32)) ;
#117137=DIRECTION('center_axis',(0.,-1.,0.)) ;
#117138=DIRECTION('ref_axis',(0.,0.,-1.)) ;
#117139=DIRECTION('center_axis',(-1.,-1.53063836115601E-16,2.73691106313441E-48)) ;
#117140=DIRECTION('ref_axis',(1.53063836115601E-16,-1.,-4.18922106430579E-64)) ;
#117141=DIRECTION('center_axis',(1.,2.16840434497101E-16,0.)) ;
#117142=DIRECTION('ref_axis',(2.16840434497101E-16,-1.,0.)) ;
#117143=DIRECTION('center_axis',(-1.,0.,2.16840434497095E-15)) ;
#117144=DIRECTION('ref_axis',(2.16840434497095E-15,0.,1.)) ;
#117145=DIRECTION('center_axis',(-1.,-2.16840434497101E-16,0.)) ;
#117146=DIRECTION('ref_axis',(0.,-1.,0.)) ;
#117147=DIRECTION('center_axis',(0.,0.,1.)) ;
#117148=DIRECTION('ref_axis',(-1.,0.,0.)) ;
#117149=DIRECTION('center_axis',(0.,1.,0.)) ;
#117150=DIRECTION('ref_axis',(1.,0.,0.)) ;
#117151=DIRECTION('center_axis',(0.,1.,0.)) ;
#117152=DIRECTION('ref_axis',(0.,0.,-1.)) ;
#117153=DIRECTION('center_axis',(1.,0.,0.)) ;
#117154=DIRECTION('ref_axis',(0.,-1.,0.)) ;
#117155=DIRECTION('center_axis',(1.,6.50521303491304E-15,0.)) ;
#117156=DIRECTION('ref_axis',(-6.50521303491304E-15,1.,0.)) ;
#117157=DIRECTION('center_axis',(8.67361737988403E-15,1.,0.)) ;
#117158=DIRECTION('ref_axis',(-1.,8.67361737988403E-15,0.)) ;
#117159=DIRECTION('center_axis',(1.2303003375722E-16,-1.,1.020425574104E-16)) ;
#117160=DIRECTION('ref_axis',(1.,1.2303003375722E-16,-1.25542992828747E-32)) ;
#117161=DIRECTION('center_axis',(0.,1.,0.)) ;
#117162=DIRECTION('ref_axis',(0.,0.,1.)) ;
#117163=DIRECTION('center_axis',(0.,1.,0.)) ;
#117164=DIRECTION('ref_axis',(1.,0.,0.)) ;
#117165=DIRECTION('center_axis',(1.,1.2303003375722E-16,0.)) ;
#117166=DIRECTION('ref_axis',(1.2303003375722E-16,-1.,0.)) ;
#117167=DIRECTION('center_axis',(0.,0.,1.)) ;
#117168=DIRECTION('ref_axis',(-1.,0.,0.)) ;
#117169=DIRECTION('center_axis',(0.,1.,0.)) ;
#117170=DIRECTION('ref_axis',(1.,0.,0.)) ;
#117171=DIRECTION('center_axis',(0.,0.,-1.)) ;
#117172=DIRECTION('ref_axis',(1.,0.,0.)) ;
#117173=DIRECTION('center_axis',(0.,0.,-1.)) ;
#117174=DIRECTION('ref_axis',(-1.,0.,0.)) ;
#117175=DIRECTION('center_axis',(0.,0.,1.)) ;
#117176=DIRECTION('ref_axis',(1.,0.,0.)) ;
#117177=DIRECTION('center_axis',(-2.16840434497101E-16,1.,-1.020425574104E-16)) ;
#117178=DIRECTION('ref_axis',(-1.,-2.16840434497101E-16,5.47382212626882E-48)) ;
#117179=DIRECTION('center_axis',(0.,1.,0.)) ;
#117180=DIRECTION('ref_axis',(0.,0.,-1.)) ;
#117181=DIRECTION('center_axis',(1.,0.,1.25542992828747E-32)) ;
#117182=DIRECTION('ref_axis',(1.25542992828747E-32,0.,-1.)) ;
#117183=DIRECTION('center_axis',(1.,0.,0.)) ;
#117184=DIRECTION('ref_axis',(0.,0.,-1.)) ;
#117185=DIRECTION('center_axis',(-1.,-1.2303003375722E-16,0.)) ;
#117186=DIRECTION('ref_axis',(0.,-1.,0.)) ;
#117187=DIRECTION('center_axis',(0.,0.,-1.)) ;
#117188=DIRECTION('ref_axis',(1.,0.,0.)) ;
#117189=DIRECTION('center_axis',(0.,0.,-1.)) ;
#117190=DIRECTION('ref_axis',(-1.,0.,0.)) ;
#117191=DIRECTION('',(0.,0.,1.)) ;
#117192=DIRECTION('center_axis',(0.,0.,1.)) ;
#117193=DIRECTION('ref_axis',(1.,0.,0.)) ;
#117194=DIRECTION('center_axis',(0.,0.,1.)) ;
#117195=DIRECTION('ref_axis',(1.,0.,0.)) ;
#117196=DIRECTION('center_axis',(6.27714964143733E-33,-5.10212787052002E-17,
-1.)) ;
#117197=DIRECTION('ref_axis',(3.20268201330022E-49,1.,-5.10212787052002E-17)) ;
#117198=DIRECTION('center_axis',(1.,1.53063836115601E-16,-1.53236300070382E-33)) ;
#117199=DIRECTION('ref_axis',(-1.53063836115601E-16,1.,2.34549359209339E-49)) ;
#117200=DIRECTION('center_axis',(-1.,0.,0.)) ;
#117201=DIRECTION('ref_axis',(0.,0.,1.)) ;
#117202=DIRECTION('center_axis',(1.,0.,0.)) ;
#117203=DIRECTION('ref_axis',(0.,0.,-1.)) ;
#117204=DIRECTION('center_axis',(0.,1.,0.)) ;
#117205=DIRECTION('ref_axis',(1.,0.,0.)) ;
#117206=DIRECTION('center_axis',(-4.33680868994202E-15,1.,0.)) ;
#117207=DIRECTION('ref_axis',(1.,4.33680868994202E-15,0.)) ;
#117208=DIRECTION('center_axis',(0.,-1.,0.)) ;
#117209=DIRECTION('ref_axis',(0.,0.,-1.)) ;
#117210=DIRECTION('center_axis',(0.,0.,-1.)) ;
#117211=DIRECTION('ref_axis',(1.,0.,0.)) ;
#117212=DIRECTION('center_axis',(0.,0.,1.)) ;
#117213=DIRECTION('ref_axis',(1.,0.,0.)) ;
#117214=DIRECTION('center_axis',(0.,0.,-1.)) ;
#117215=DIRECTION('ref_axis',(-1.,0.,0.)) ;
#117216=DIRECTION('center_axis',(0.,1.,0.)) ;
#117217=DIRECTION('ref_axis',(1.,0.,0.)) ;
#117218=DIRECTION('center_axis',(1.,1.2303003375722E-16,0.)) ;
#117219=DIRECTION('ref_axis',(1.2303003375722E-16,-1.,0.)) ;
#117220=DIRECTION('center_axis',(0.,1.,0.)) ;
#117221=DIRECTION('ref_axis',(-6.50521303491284E-15,0.,-1.)) ;
#117222=DIRECTION('center_axis',(6.27714964143733E-33,-5.10212787052002E-17,
-1.)) ;
#117223=DIRECTION('ref_axis',(0.,1.,0.)) ;
#117224=DIRECTION('center_axis',(0.,-1.,0.)) ;
#117225=DIRECTION('ref_axis',(0.,0.,1.)) ;
#117226=DIRECTION('center_axis',(2.16840434497101E-16,-1.,5.10212787052002E-17)) ;
#117227=DIRECTION('ref_axis',(1.,2.16840434497101E-16,-5.47382212626882E-48)) ;
#117228=DIRECTION('center_axis',(0.,1.,0.)) ;
#117229=DIRECTION('ref_axis',(0.,0.,-1.)) ;
#117230=DIRECTION('center_axis',(0.,0.,1.)) ;
#117231=DIRECTION('ref_axis',(1.,0.,0.)) ;
#117232=DIRECTION('center_axis',(0.,0.,-1.)) ;
#117233=DIRECTION('ref_axis',(-1.,0.,0.)) ;
#117234=DIRECTION('center_axis',(-1.,-1.2303003375722E-16,0.)) ;
#117235=DIRECTION('ref_axis',(0.,-1.,0.)) ;
#117236=DIRECTION('center_axis',(0.,-1.,0.)) ;
#117237=DIRECTION('ref_axis',(0.,0.,1.)) ;
#117238=DIRECTION('center_axis',(1.53063836115601E-16,-1.,5.10212787052002E-17)) ;
#117239=DIRECTION('ref_axis',(1.,1.53063836115601E-16,-6.84227765783602E-48)) ;
#117240=DIRECTION('',(-1.53063836115601E-16,1.,-5.10212787052002E-17)) ;
#117241=DIRECTION('center_axis',(0.,-1.,0.)) ;
#117242=DIRECTION('ref_axis',(0.,0.,-1.)) ;
#117243=DIRECTION('center_axis',(-1.,0.,0.)) ;
#117244=DIRECTION('ref_axis',(0.,0.,-1.)) ;
#117245=DIRECTION('center_axis',(-1.2303003375722E-16,1.,-5.10212787052002E-17)) ;
#117246=DIRECTION('ref_axis',(-1.,-1.2303003375722E-16,6.27714964143733E-33)) ;
#117247=DIRECTION('center_axis',(-8.67361737988403E-15,-1.,0.)) ;
#117248=DIRECTION('ref_axis',(1.,-8.67361737988403E-15,0.)) ;
#117249=DIRECTION('center_axis',(1.,0.,6.27714964143733E-33)) ;
#117250=DIRECTION('ref_axis',(6.27714964143733E-33,0.,-1.)) ;
#117251=DIRECTION('center_axis',(-1.,0.,-6.50521303491284E-15)) ;
#117252=DIRECTION('ref_axis',(-6.50521303491284E-15,0.,1.)) ;
#117253=DIRECTION('center_axis',(1.,0.,0.)) ;
#117254=DIRECTION('ref_axis',(0.,1.,0.)) ;
#117255=DIRECTION('center_axis',(0.,0.,-1.)) ;
#117256=DIRECTION('ref_axis',(-1.,0.,0.)) ;
#117257=DIRECTION('center_axis',(0.,0.,1.)) ;
#117258=DIRECTION('ref_axis',(1.,0.,0.)) ;
#117259=DIRECTION('center_axis',(0.,0.,-1.)) ;
#117260=DIRECTION('ref_axis',(-1.,0.,0.)) ;
#117261=DIRECTION('center_axis',(-1.,0.,0.)) ;
#117262=DIRECTION('ref_axis',(0.,0.,1.)) ;
#117263=DIRECTION('center_axis',(0.,-1.,0.)) ;
#117264=DIRECTION('ref_axis',(0.,0.,-1.)) ;
#117265=DIRECTION('center_axis',(0.,1.,0.)) ;
#117266=DIRECTION('ref_axis',(0.,0.,1.)) ;
#117267=DIRECTION('center_axis',(0.,1.,-6.50521303491284E-15)) ;
#117268=DIRECTION('ref_axis',(0.,6.50521303491284E-15,1.)) ;
#117269=DIRECTION('center_axis',(0.,-1.,0.)) ;
#117270=DIRECTION('ref_axis',(0.,0.,-1.)) ;
#117271=DIRECTION('center_axis',(0.,-1.,0.)) ;
#117272=DIRECTION('ref_axis',(0.,0.,-1.)) ;
#117273=DIRECTION('center_axis',(0.,-1.,-1.07081696047951E-16)) ;
#117274=DIRECTION('ref_axis',(0.,1.07081696047951E-16,-1.)) ;
#117275=DIRECTION('center_axis',(0.,1.,0.)) ;
#117276=DIRECTION('ref_axis',(0.,0.,1.)) ;
#117277=DIRECTION('center_axis',(-1.,0.,0.)) ;
#117278=DIRECTION('ref_axis',(0.,0.,1.)) ;
#117279=DIRECTION('center_axis',(0.,0.,1.)) ;
#117280=DIRECTION('ref_axis',(1.,0.,0.)) ;
#117281=DIRECTION('center_axis',(0.,1.,0.)) ;
#117282=DIRECTION('ref_axis',(0.,0.,1.)) ;
#117283=DIRECTION('center_axis',(0.,0.,-1.)) ;
#117284=DIRECTION('ref_axis',(-1.,0.,0.)) ;
#117285=DIRECTION('center_axis',(0.,0.,1.)) ;
#117286=DIRECTION('ref_axis',(1.,0.,0.)) ;
#117287=DIRECTION('center_axis',(0.,0.,1.)) ;
#117288=DIRECTION('ref_axis',(1.,0.,0.)) ;
#117289=DIRECTION('center_axis',(0.,0.,1.)) ;
#117290=DIRECTION('ref_axis',(1.,0.,0.)) ;
#117291=DIRECTION('center_axis',(0.,0.,-1.)) ;
#117292=DIRECTION('ref_axis',(-1.,0.,0.)) ;
#117293=DIRECTION('center_axis',(0.,1.,0.)) ;
#117294=DIRECTION('ref_axis',(0.,0.,1.)) ;
#117295=DIRECTION('center_axis',(0.,-0.707106781186532,0.707106781186563)) ;
#117296=DIRECTION('ref_axis',(0.,-0.707106781186563,-0.707106781186532)) ;
#117297=DIRECTION('center_axis',(0.,1.,0.)) ;
#117298=DIRECTION('ref_axis',(0.,0.,1.)) ;
#117299=DIRECTION('center_axis',(2.23012492569655E-15,-0.51423179695906,
-0.857651245551627)) ;
#117300=DIRECTION('ref_axis',(2.6714619735869E-30,0.857651245551626,-0.51423179695906)) ;
#117301=DIRECTION('center_axis',(0.,-0.707106781186548,0.707106781186547)) ;
#117302=DIRECTION('ref_axis',(0.,-0.707106781186547,-0.707106781186548)) ;
#117303=DIRECTION('center_axis',(0.,-0.707106781186543,0.707106781186552)) ;
#117304=DIRECTION('ref_axis',(0.,-0.707106781186552,-0.707106781186543)) ;
#117305=DIRECTION('center_axis',(-1.,0.,0.)) ;
#117306=DIRECTION('ref_axis',(0.,0.,1.)) ;
#117307=DIRECTION('center_axis',(-6.69037477709043E-15,0.51423179695912,
-0.85765124555159)) ;
#117308=DIRECTION('ref_axis',(-4.44487660401203E-29,0.85765124555159,0.51423179695912)) ;
#117309=DIRECTION('center_axis',(0.,1.,0.)) ;
#117310=DIRECTION('ref_axis',(0.,0.,1.)) ;
#117311=DIRECTION('center_axis',(0.,0.,-1.)) ;
#117312=DIRECTION('ref_axis',(-1.,0.,0.)) ;
#117313=DIRECTION('center_axis',(0.,1.,0.)) ;
#117314=DIRECTION('ref_axis',(0.,0.,1.)) ;
#117315=DIRECTION('center_axis',(0.,0.,-1.)) ;
#117316=DIRECTION('ref_axis',(-1.,0.,0.)) ;
#117317=DIRECTION('center_axis',(0.,0.,-1.)) ;
#117318=DIRECTION('ref_axis',(-1.,0.,0.)) ;
#117319=DIRECTION('center_axis',(0.,0.,1.)) ;
#117320=DIRECTION('ref_axis',(1.,0.,0.)) ;
#117321=DIRECTION('center_axis',(0.,0.,-1.)) ;
#117322=DIRECTION('ref_axis',(-1.,0.,0.)) ;
#117323=DIRECTION('center_axis',(0.,1.,0.)) ;
#117324=DIRECTION('ref_axis',(0.,0.,1.)) ;
#117325=DIRECTION('center_axis',(0.,-1.,8.67361737988379E-15)) ;
#117326=DIRECTION('ref_axis',(0.,-8.67361737988379E-15,-1.)) ;
#117327=DIRECTION('center_axis',(0.,0.707106781186546,0.707106781186549)) ;
#117328=DIRECTION('ref_axis',(0.,-0.707106781186549,0.707106781186546)) ;
#117329=DIRECTION('center_axis',(0.,0.707106781186534,0.707106781186561)) ;
#117330=DIRECTION('ref_axis',(0.,-0.707106781186561,0.707106781186534)) ;
#117331=DIRECTION('center_axis',(0.,1.,1.07081696047951E-16)) ;
#117332=DIRECTION('ref_axis',(0.,-1.07081696047951E-16,1.)) ;
#117333=DIRECTION('center_axis',(0.,-1.,0.)) ;
#117334=DIRECTION('ref_axis',(0.,0.,-1.)) ;
#117335=DIRECTION('center_axis',(0.,1.,0.)) ;
#117336=DIRECTION('ref_axis',(0.,0.,1.)) ;
#117337=DIRECTION('center_axis',(0.,0.,1.)) ;
#117338=DIRECTION('ref_axis',(1.,0.,0.)) ;
#117339=DIRECTION('center_axis',(0.,1.,0.)) ;
#117340=DIRECTION('ref_axis',(0.,0.,1.)) ;
#117341=DIRECTION('center_axis',(0.,6.93889390390723E-14,1.)) ;
#117342=DIRECTION('ref_axis',(0.,-1.,6.93889390390723E-14)) ;
#117343=DIRECTION('center_axis',(0.,3.99416362155027E-15,1.)) ;
#117344=DIRECTION('ref_axis',(0.,-1.,3.99416362155027E-15)) ;
#117345=DIRECTION('center_axis',(0.,0.,1.)) ;
#117346=DIRECTION('ref_axis',(1.,0.,0.)) ;
#117347=DIRECTION('center_axis',(0.,0.,-1.)) ;
#117348=DIRECTION('ref_axis',(-1.,0.,0.)) ;
#117349=DIRECTION('center_axis',(0.,0.,1.)) ;
#117350=DIRECTION('ref_axis',(1.,0.,0.)) ;
#117351=DIRECTION('center_axis',(-1.,0.,0.)) ;
#117352=DIRECTION('ref_axis',(0.,0.,1.)) ;
#117353=DIRECTION('center_axis',(0.,1.,0.)) ;
#117354=DIRECTION('ref_axis',(0.,0.,1.)) ;
#117355=DIRECTION('center_axis',(-1.,0.,0.)) ;
#117356=DIRECTION('ref_axis',(0.,0.,1.)) ;
#117357=DIRECTION('center_axis',(0.,-1.,0.)) ;
#117358=DIRECTION('ref_axis',(0.,0.,-1.)) ;
#117359=DIRECTION('center_axis',(0.,1.,0.)) ;
#117360=DIRECTION('ref_axis',(0.,0.,1.)) ;
#117361=DIRECTION('center_axis',(1.,-9.85638338623186E-18,0.)) ;
#117362=DIRECTION('ref_axis',(9.85638338623186E-18,1.,0.)) ;
#117363=DIRECTION('',(0.,0.,-1.)) ;
#117364=DIRECTION('',(-9.85638338623186E-18,-1.,0.)) ;
#117365=DIRECTION('',(0.,0.,1.)) ;
#117366=DIRECTION('',(9.85638338623186E-18,1.,0.)) ;
#117367=DIRECTION('center_axis',(0.707106781186548,0.707106781186548,0.)) ;
#117368=DIRECTION('ref_axis',(-0.707106781186548,0.707106781186548,0.)) ;
#117369=DIRECTION('',(0.,0.,1.)) ;
#117370=DIRECTION('',(-0.577350269189625,0.577350269189625,0.577350269189627)) ;
#117371=DIRECTION('',(0.,0.,-1.)) ;
#117372=DIRECTION('',(0.577350269189625,-0.577350269189625,0.577350269189627)) ;
#117373=DIRECTION('center_axis',(0.,1.,0.)) ;
#117374=DIRECTION('ref_axis',(0.,0.,1.)) ;
#117375=DIRECTION('',(0.,0.,1.)) ;
#117376=DIRECTION('',(-1.,0.,-9.8563833862319E-18)) ;
#117377=DIRECTION('',(0.,0.,-1.)) ;
#117378=DIRECTION('',(1.,0.,-9.8563833862319E-18)) ;
#117379=DIRECTION('center_axis',(-0.707106781186548,0.707106781186548,0.)) ;
#117380=DIRECTION('ref_axis',(-0.707106781186548,-0.707106781186548,0.)) ;
#117381=DIRECTION('',(0.,0.,1.)) ;
#117382=DIRECTION('',(-0.577350269189625,-0.577350269189625,-0.577350269189627)) ;
#117383=DIRECTION('',(0.,0.,-1.)) ;
#117384=DIRECTION('',(0.577350269189625,0.577350269189625,-0.577350269189627)) ;
#117385=DIRECTION('center_axis',(-1.,9.85638338623186E-18,0.)) ;
#117386=DIRECTION('ref_axis',(-9.85638338623186E-18,-1.,0.)) ;
#117387=DIRECTION('',(0.,0.,-1.)) ;
#117388=DIRECTION('',(9.85638338623186E-18,1.,0.)) ;
#117389=DIRECTION('',(0.,0.,-1.)) ;
#117390=DIRECTION('',(-9.85638338623186E-18,-1.,0.)) ;
#117391=DIRECTION('center_axis',(0.,0.,1.)) ;
#117392=DIRECTION('ref_axis',(1.,0.,0.)) ;
#117393=DIRECTION('',(9.85638338623186E-18,1.,0.)) ;
#117394=DIRECTION('center_axis',(0.,0.,-1.)) ;
#117395=DIRECTION('ref_axis',(1.,0.,0.)) ;
#117396=DIRECTION('center_axis',(0.,0.,1.)) ;
#117397=DIRECTION('ref_axis',(1.,0.,0.)) ;
#117398=DIRECTION('',(-9.85638338623186E-18,-1.,0.)) ;
#117399=DIRECTION('',(1.,-9.85638338623186E-18,0.)) ;
#117400=DIRECTION('center_axis',(0.,0.,1.)) ;
#117401=DIRECTION('ref_axis',(1.,0.,0.)) ;
#117402=DIRECTION('',(9.85638338623186E-18,1.,0.)) ;
#117403=DIRECTION('center_axis',(0.,0.,-1.)) ;
#117404=DIRECTION('ref_axis',(1.,0.,0.)) ;
#117405=DIRECTION('center_axis',(0.,0.,1.)) ;
#117406=DIRECTION('ref_axis',(1.,0.,0.)) ;
#117407=DIRECTION('',(-9.85638338623186E-18,-1.,0.)) ;
#117408=DIRECTION('',(-1.,9.85638338623186E-18,0.)) ;
#117409=DIRECTION('center_axis',(0.,0.,-1.)) ;
#117410=DIRECTION('ref_axis',(-1.,0.,0.)) ;
#117411=DIRECTION('center_axis',(0.,0.,1.)) ;
#117412=DIRECTION('ref_axis',(1.,0.,0.)) ;
#117413=DIRECTION('center_axis',(0.,0.,-1.)) ;
#117414=DIRECTION('ref_axis',(1.,0.,0.)) ;
#117415=DIRECTION('center_axis',(0.,0.,-1.)) ;
#117416=DIRECTION('ref_axis',(-1.,0.,0.)) ;
#117417=DIRECTION('center_axis',(0.,0.,-1.)) ;
#117418=DIRECTION('ref_axis',(1.,0.,0.)) ;
#117419=DIRECTION('center_axis',(0.,0.,1.)) ;
#117420=DIRECTION('ref_axis',(1.,0.,0.)) ;
#117421=DIRECTION('center_axis',(-0.707106781186548,-0.707106781186547,
0.)) ;
#117422=DIRECTION('ref_axis',(0.707106781186547,-0.707106781186548,0.)) ;
#117423=DIRECTION('',(0.,0.,1.)) ;
#117424=DIRECTION('',(0.577350269189625,-0.577350269189626,-0.577350269189626)) ;
#117425=DIRECTION('',(0.,0.,-1.)) ;
#117426=DIRECTION('',(-0.577350269189625,0.577350269189626,-0.577350269189626)) ;
#117427=DIRECTION('center_axis',(1.95511867169517E-16,-1.,0.)) ;
#117428=DIRECTION('ref_axis',(1.,1.95511867169517E-16,0.)) ;
#117429=DIRECTION('',(0.,0.,-1.)) ;
#117430=DIRECTION('',(-1.,-1.95511867169517E-16,0.)) ;
#117431=DIRECTION('',(1.,1.95511867169517E-16,0.)) ;
#117432=DIRECTION('center_axis',(1.06642836637918E-16,1.,0.)) ;
#117433=DIRECTION('ref_axis',(-1.,1.06642836637918E-16,0.)) ;
#117434=DIRECTION('',(1.,-1.06642836637919E-16,0.)) ;
#117435=DIRECTION('',(0.,0.,1.)) ;
#117436=DIRECTION('',(-1.,1.06642836637919E-16,0.)) ;
#117437=DIRECTION('center_axis',(-0.707106781186548,0.707106781186547,0.)) ;
#117438=DIRECTION('ref_axis',(-0.707106781186547,-0.707106781186548,0.)) ;
#117439=DIRECTION('',(0.,0.,1.)) ;
#117440=DIRECTION('',(-0.577350269189625,-0.577350269189626,0.577350269189627)) ;
#117441=DIRECTION('',(0.,0.,-1.)) ;
#117442=DIRECTION('',(0.577350269189625,0.577350269189626,0.577350269189627)) ;
#117443=DIRECTION('center_axis',(-1.,0.,0.)) ;
#117444=DIRECTION('ref_axis',(0.,0.,1.)) ;
#117445=DIRECTION('',(0.,0.,-1.)) ;
#117446=DIRECTION('',(0.,1.,1.95511867169518E-16)) ;
#117447=DIRECTION('',(0.,0.,1.)) ;
#117448=DIRECTION('',(0.,-1.,1.95511867169518E-16)) ;
#117449=DIRECTION('center_axis',(0.,0.,1.)) ;
#117450=DIRECTION('ref_axis',(1.,0.,0.)) ;
#117451=DIRECTION('',(-1.95511867169517E-16,1.,0.)) ;
#117452=DIRECTION('',(-1.,-1.95511867169517E-16,0.)) ;
#117453=DIRECTION('',(1.,-1.06642836637919E-16,0.)) ;
#117454=DIRECTION('center_axis',(0.,0.,1.)) ;
#117455=DIRECTION('ref_axis',(1.,0.,0.)) ;
#117456=DIRECTION('',(1.,1.95511867169517E-16,0.)) ;
#117457=DIRECTION('',(1.95511867169517E-16,-1.,0.)) ;
#117458=DIRECTION('',(-1.,1.06642836637919E-16,0.)) ;
#117459=DIRECTION('center_axis',(1.,-9.85638338623186E-18,0.)) ;
#117460=DIRECTION('ref_axis',(9.85638338623186E-18,1.,0.)) ;
#117461=DIRECTION('',(0.,0.,-1.)) ;
#117462=DIRECTION('',(-9.85638338623186E-18,-1.,0.)) ;
#117463=DIRECTION('',(0.,0.,1.)) ;
#117464=DIRECTION('',(9.85638338623186E-18,1.,0.)) ;
#117465=DIRECTION('center_axis',(0.707106781186548,0.707106781186548,0.)) ;
#117466=DIRECTION('ref_axis',(-0.707106781186548,0.707106781186548,0.)) ;
#117467=DIRECTION('',(0.,0.,1.)) ;
#117468=DIRECTION('',(-0.577350269189625,0.577350269189625,0.577350269189627)) ;
#117469=DIRECTION('',(0.,0.,-1.)) ;
#117470=DIRECTION('',(0.577350269189625,-0.577350269189625,0.577350269189627)) ;
#117471=DIRECTION('center_axis',(0.,1.,0.)) ;
#117472=DIRECTION('ref_axis',(0.,0.,1.)) ;
#117473=DIRECTION('',(0.,0.,1.)) ;
#117474=DIRECTION('',(-1.,0.,-9.8563833862319E-18)) ;
#117475=DIRECTION('',(0.,0.,-1.)) ;
#117476=DIRECTION('',(1.,0.,-9.8563833862319E-18)) ;
#117477=DIRECTION('center_axis',(-0.707106781186548,0.707106781186548,0.)) ;
#117478=DIRECTION('ref_axis',(-0.707106781186548,-0.707106781186548,0.)) ;
#117479=DIRECTION('',(0.,0.,1.)) ;
#117480=DIRECTION('',(-0.577350269189625,-0.577350269189625,-0.577350269189627)) ;
#117481=DIRECTION('',(0.,0.,-1.)) ;
#117482=DIRECTION('',(0.577350269189625,0.577350269189625,-0.577350269189627)) ;
#117483=DIRECTION('center_axis',(-1.,9.85638338623186E-18,0.)) ;
#117484=DIRECTION('ref_axis',(-9.85638338623186E-18,-1.,0.)) ;
#117485=DIRECTION('',(0.,0.,-1.)) ;
#117486=DIRECTION('',(9.85638338623186E-18,1.,0.)) ;
#117487=DIRECTION('',(0.,0.,-1.)) ;
#117488=DIRECTION('',(-9.85638338623186E-18,-1.,0.)) ;
#117489=DIRECTION('center_axis',(0.,0.,1.)) ;
#117490=DIRECTION('ref_axis',(1.,0.,0.)) ;
#117491=DIRECTION('',(9.85638338623186E-18,1.,0.)) ;
#117492=DIRECTION('center_axis',(0.,0.,-1.)) ;
#117493=DIRECTION('ref_axis',(1.,0.,0.)) ;
#117494=DIRECTION('center_axis',(0.,0.,1.)) ;
#117495=DIRECTION('ref_axis',(1.,0.,0.)) ;
#117496=DIRECTION('',(-9.85638338623186E-18,-1.,0.)) ;
#117497=DIRECTION('',(1.,-9.85638338623186E-18,0.)) ;
#117498=DIRECTION('center_axis',(0.,0.,1.)) ;
#117499=DIRECTION('ref_axis',(1.,0.,0.)) ;
#117500=DIRECTION('',(9.85638338623186E-18,1.,0.)) ;
#117501=DIRECTION('center_axis',(0.,0.,-1.)) ;
#117502=DIRECTION('ref_axis',(1.,0.,0.)) ;
#117503=DIRECTION('center_axis',(0.,0.,1.)) ;
#117504=DIRECTION('ref_axis',(1.,0.,0.)) ;
#117505=DIRECTION('',(-9.85638338623186E-18,-1.,0.)) ;
#117506=DIRECTION('',(-1.,9.85638338623186E-18,0.)) ;
#117507=DIRECTION('center_axis',(0.,0.,-1.)) ;
#117508=DIRECTION('ref_axis',(-1.,0.,0.)) ;
#117509=DIRECTION('center_axis',(0.,0.,1.)) ;
#117510=DIRECTION('ref_axis',(1.,0.,0.)) ;
#117511=DIRECTION('center_axis',(0.,0.,-1.)) ;
#117512=DIRECTION('ref_axis',(1.,0.,0.)) ;
#117513=DIRECTION('center_axis',(0.,0.,-1.)) ;
#117514=DIRECTION('ref_axis',(-1.,0.,0.)) ;
#117515=DIRECTION('center_axis',(0.,0.,-1.)) ;
#117516=DIRECTION('ref_axis',(1.,0.,0.)) ;
#117517=DIRECTION('center_axis',(0.,0.,1.)) ;
#117518=DIRECTION('ref_axis',(1.,0.,0.)) ;
#117519=DIRECTION('center_axis',(-0.707106781186548,-0.707106781186547,
0.)) ;
#117520=DIRECTION('ref_axis',(0.707106781186547,-0.707106781186548,0.)) ;
#117521=DIRECTION('',(0.,0.,1.)) ;
#117522=DIRECTION('',(0.577350269189625,-0.577350269189626,-0.577350269189626)) ;
#117523=DIRECTION('',(0.,0.,-1.)) ;
#117524=DIRECTION('',(-0.577350269189625,0.577350269189626,-0.577350269189626)) ;
#117525=DIRECTION('center_axis',(1.95511867169517E-16,-1.,0.)) ;
#117526=DIRECTION('ref_axis',(1.,1.95511867169517E-16,0.)) ;
#117527=DIRECTION('',(0.,0.,-1.)) ;
#117528=DIRECTION('',(-1.,-1.95511867169517E-16,0.)) ;
#117529=DIRECTION('',(1.,1.95511867169517E-16,0.)) ;
#117530=DIRECTION('center_axis',(1.06642836637918E-16,1.,0.)) ;
#117531=DIRECTION('ref_axis',(-1.,1.06642836637918E-16,0.)) ;
#117532=DIRECTION('',(1.,-1.06642836637919E-16,0.)) ;
#117533=DIRECTION('',(0.,0.,1.)) ;
#117534=DIRECTION('',(-1.,1.06642836637919E-16,0.)) ;
#117535=DIRECTION('center_axis',(-0.707106781186548,0.707106781186547,0.)) ;
#117536=DIRECTION('ref_axis',(-0.707106781186547,-0.707106781186548,0.)) ;
#117537=DIRECTION('',(0.,0.,1.)) ;
#117538=DIRECTION('',(-0.577350269189625,-0.577350269189626,0.577350269189627)) ;
#117539=DIRECTION('',(0.,0.,-1.)) ;
#117540=DIRECTION('',(0.577350269189625,0.577350269189626,0.577350269189627)) ;
#117541=DIRECTION('center_axis',(-1.,0.,0.)) ;
#117542=DIRECTION('ref_axis',(0.,0.,1.)) ;
#117543=DIRECTION('',(0.,0.,-1.)) ;
#117544=DIRECTION('',(0.,1.,1.95511867169518E-16)) ;
#117545=DIRECTION('',(0.,0.,1.)) ;
#117546=DIRECTION('',(0.,-1.,1.95511867169518E-16)) ;
#117547=DIRECTION('center_axis',(0.,0.,1.)) ;
#117548=DIRECTION('ref_axis',(1.,0.,0.)) ;
#117549=DIRECTION('',(-1.95511867169517E-16,1.,0.)) ;
#117550=DIRECTION('',(-1.,-1.95511867169517E-16,0.)) ;
#117551=DIRECTION('',(1.,-1.06642836637919E-16,0.)) ;
#117552=DIRECTION('center_axis',(0.,0.,1.)) ;
#117553=DIRECTION('ref_axis',(1.,0.,0.)) ;
#117554=DIRECTION('',(1.,1.95511867169517E-16,0.)) ;
#117555=DIRECTION('',(1.95511867169517E-16,-1.,0.)) ;
#117556=DIRECTION('',(-1.,1.06642836637919E-16,0.)) ;
#117557=DIRECTION('center_axis',(1.,-9.85638338623186E-18,0.)) ;
#117558=DIRECTION('ref_axis',(9.85638338623186E-18,1.,0.)) ;
#117559=DIRECTION('',(0.,0.,-1.)) ;
#117560=DIRECTION('',(-9.85638338623186E-18,-1.,0.)) ;
#117561=DIRECTION('',(0.,0.,1.)) ;
#117562=DIRECTION('',(9.85638338623186E-18,1.,0.)) ;
#117563=DIRECTION('center_axis',(0.707106781186548,0.707106781186548,0.)) ;
#117564=DIRECTION('ref_axis',(-0.707106781186548,0.707106781186548,0.)) ;
#117565=DIRECTION('',(0.,0.,1.)) ;
#117566=DIRECTION('',(-0.577350269189625,0.577350269189625,0.577350269189627)) ;
#117567=DIRECTION('',(0.,0.,-1.)) ;
#117568=DIRECTION('',(0.577350269189625,-0.577350269189625,0.577350269189627)) ;
#117569=DIRECTION('center_axis',(0.,1.,0.)) ;
#117570=DIRECTION('ref_axis',(0.,0.,1.)) ;
#117571=DIRECTION('',(0.,0.,1.)) ;
#117572=DIRECTION('',(-1.,0.,-9.8563833862319E-18)) ;
#117573=DIRECTION('',(0.,0.,-1.)) ;
#117574=DIRECTION('',(1.,0.,-9.8563833862319E-18)) ;
#117575=DIRECTION('center_axis',(-0.707106781186548,0.707106781186548,0.)) ;
#117576=DIRECTION('ref_axis',(-0.707106781186548,-0.707106781186548,0.)) ;
#117577=DIRECTION('',(0.,0.,1.)) ;
#117578=DIRECTION('',(-0.577350269189625,-0.577350269189625,-0.577350269189627)) ;
#117579=DIRECTION('',(0.,0.,-1.)) ;
#117580=DIRECTION('',(0.577350269189625,0.577350269189625,-0.577350269189627)) ;
#117581=DIRECTION('center_axis',(-1.,9.85638338623186E-18,0.)) ;
#117582=DIRECTION('ref_axis',(-9.85638338623186E-18,-1.,0.)) ;
#117583=DIRECTION('',(0.,0.,-1.)) ;
#117584=DIRECTION('',(9.85638338623186E-18,1.,0.)) ;
#117585=DIRECTION('',(0.,0.,-1.)) ;
#117586=DIRECTION('',(-9.85638338623186E-18,-1.,0.)) ;
#117587=DIRECTION('center_axis',(0.,0.,1.)) ;
#117588=DIRECTION('ref_axis',(1.,0.,0.)) ;
#117589=DIRECTION('',(9.85638338623186E-18,1.,0.)) ;
#117590=DIRECTION('center_axis',(0.,0.,-1.)) ;
#117591=DIRECTION('ref_axis',(1.,0.,0.)) ;
#117592=DIRECTION('center_axis',(0.,0.,1.)) ;
#117593=DIRECTION('ref_axis',(1.,0.,0.)) ;
#117594=DIRECTION('',(-9.85638338623186E-18,-1.,0.)) ;
#117595=DIRECTION('',(1.,-9.85638338623186E-18,0.)) ;
#117596=DIRECTION('center_axis',(0.,0.,1.)) ;
#117597=DIRECTION('ref_axis',(1.,0.,0.)) ;
#117598=DIRECTION('',(9.85638338623186E-18,1.,0.)) ;
#117599=DIRECTION('center_axis',(0.,0.,-1.)) ;
#117600=DIRECTION('ref_axis',(1.,0.,0.)) ;
#117601=DIRECTION('center_axis',(0.,0.,1.)) ;
#117602=DIRECTION('ref_axis',(1.,0.,0.)) ;
#117603=DIRECTION('',(-9.85638338623186E-18,-1.,0.)) ;
#117604=DIRECTION('',(-1.,9.85638338623186E-18,0.)) ;
#117605=DIRECTION('center_axis',(0.,0.,-1.)) ;
#117606=DIRECTION('ref_axis',(-1.,0.,0.)) ;
#117607=DIRECTION('center_axis',(0.,0.,1.)) ;
#117608=DIRECTION('ref_axis',(1.,0.,0.)) ;
#117609=DIRECTION('center_axis',(0.,0.,-1.)) ;
#117610=DIRECTION('ref_axis',(1.,0.,0.)) ;
#117611=DIRECTION('center_axis',(0.,0.,-1.)) ;
#117612=DIRECTION('ref_axis',(-1.,0.,0.)) ;
#117613=DIRECTION('center_axis',(0.,0.,-1.)) ;
#117614=DIRECTION('ref_axis',(1.,0.,0.)) ;
#117615=DIRECTION('center_axis',(0.,0.,1.)) ;
#117616=DIRECTION('ref_axis',(1.,0.,0.)) ;
#117617=DIRECTION('center_axis',(-0.707106781186548,-0.707106781186547,
0.)) ;
#117618=DIRECTION('ref_axis',(0.707106781186547,-0.707106781186548,0.)) ;
#117619=DIRECTION('',(0.,0.,1.)) ;
#117620=DIRECTION('',(0.577350269189625,-0.577350269189626,-0.577350269189626)) ;
#117621=DIRECTION('',(0.,0.,-1.)) ;
#117622=DIRECTION('',(-0.577350269189625,0.577350269189626,-0.577350269189626)) ;
#117623=DIRECTION('center_axis',(1.95511867169517E-16,-1.,0.)) ;
#117624=DIRECTION('ref_axis',(1.,1.95511867169517E-16,0.)) ;
#117625=DIRECTION('',(0.,0.,-1.)) ;
#117626=DIRECTION('',(-1.,-1.95511867169517E-16,0.)) ;
#117627=DIRECTION('',(1.,1.95511867169517E-16,0.)) ;
#117628=DIRECTION('center_axis',(1.06642836637918E-16,1.,0.)) ;
#117629=DIRECTION('ref_axis',(-1.,1.06642836637918E-16,0.)) ;
#117630=DIRECTION('',(1.,-1.06642836637919E-16,0.)) ;
#117631=DIRECTION('',(0.,0.,1.)) ;
#117632=DIRECTION('',(-1.,1.06642836637919E-16,0.)) ;
#117633=DIRECTION('center_axis',(-0.707106781186548,0.707106781186547,0.)) ;
#117634=DIRECTION('ref_axis',(-0.707106781186547,-0.707106781186548,0.)) ;
#117635=DIRECTION('',(0.,0.,1.)) ;
#117636=DIRECTION('',(-0.577350269189625,-0.577350269189626,0.577350269189627)) ;
#117637=DIRECTION('',(0.,0.,-1.)) ;
#117638=DIRECTION('',(0.577350269189625,0.577350269189626,0.577350269189627)) ;
#117639=DIRECTION('center_axis',(-1.,0.,0.)) ;
#117640=DIRECTION('ref_axis',(0.,0.,1.)) ;
#117641=DIRECTION('',(0.,0.,-1.)) ;
#117642=DIRECTION('',(0.,1.,1.95511867169518E-16)) ;
#117643=DIRECTION('',(0.,0.,1.)) ;
#117644=DIRECTION('',(0.,-1.,1.95511867169518E-16)) ;
#117645=DIRECTION('center_axis',(0.,0.,1.)) ;
#117646=DIRECTION('ref_axis',(1.,0.,0.)) ;
#117647=DIRECTION('',(-1.95511867169517E-16,1.,0.)) ;
#117648=DIRECTION('',(-1.,-1.95511867169517E-16,0.)) ;
#117649=DIRECTION('',(1.,-1.06642836637919E-16,0.)) ;
#117650=DIRECTION('center_axis',(0.,0.,1.)) ;
#117651=DIRECTION('ref_axis',(1.,0.,0.)) ;
#117652=DIRECTION('',(1.,1.95511867169517E-16,0.)) ;
#117653=DIRECTION('',(1.95511867169517E-16,-1.,0.)) ;
#117654=DIRECTION('',(-1.,1.06642836637919E-16,0.)) ;
#117655=DIRECTION('center_axis',(1.,-9.85638338623186E-18,0.)) ;
#117656=DIRECTION('ref_axis',(9.85638338623186E-18,1.,0.)) ;
#117657=DIRECTION('',(0.,0.,-1.)) ;
#117658=DIRECTION('',(-9.85638338623186E-18,-1.,0.)) ;
#117659=DIRECTION('',(0.,0.,1.)) ;
#117660=DIRECTION('',(9.85638338623186E-18,1.,0.)) ;
#117661=DIRECTION('center_axis',(0.707106781186548,0.707106781186548,0.)) ;
#117662=DIRECTION('ref_axis',(-0.707106781186548,0.707106781186548,0.)) ;
#117663=DIRECTION('',(0.,0.,1.)) ;
#117664=DIRECTION('',(-0.577350269189625,0.577350269189625,0.577350269189627)) ;
#117665=DIRECTION('',(0.,0.,-1.)) ;
#117666=DIRECTION('',(0.577350269189625,-0.577350269189625,0.577350269189627)) ;
#117667=DIRECTION('center_axis',(0.,1.,0.)) ;
#117668=DIRECTION('ref_axis',(0.,0.,1.)) ;
#117669=DIRECTION('',(0.,0.,1.)) ;
#117670=DIRECTION('',(-1.,0.,-9.8563833862319E-18)) ;
#117671=DIRECTION('',(0.,0.,-1.)) ;
#117672=DIRECTION('',(1.,0.,-9.8563833862319E-18)) ;
#117673=DIRECTION('center_axis',(-0.707106781186548,0.707106781186548,0.)) ;
#117674=DIRECTION('ref_axis',(-0.707106781186548,-0.707106781186548,0.)) ;
#117675=DIRECTION('',(0.,0.,1.)) ;
#117676=DIRECTION('',(-0.577350269189625,-0.577350269189625,-0.577350269189627)) ;
#117677=DIRECTION('',(0.,0.,-1.)) ;
#117678=DIRECTION('',(0.577350269189625,0.577350269189625,-0.577350269189627)) ;
#117679=DIRECTION('center_axis',(-1.,9.85638338623186E-18,0.)) ;
#117680=DIRECTION('ref_axis',(-9.85638338623186E-18,-1.,0.)) ;
#117681=DIRECTION('',(0.,0.,-1.)) ;
#117682=DIRECTION('',(9.85638338623186E-18,1.,0.)) ;
#117683=DIRECTION('',(0.,0.,-1.)) ;
#117684=DIRECTION('',(-9.85638338623186E-18,-1.,0.)) ;
#117685=DIRECTION('center_axis',(0.,0.,1.)) ;
#117686=DIRECTION('ref_axis',(1.,0.,0.)) ;
#117687=DIRECTION('',(9.85638338623186E-18,1.,0.)) ;
#117688=DIRECTION('center_axis',(0.,0.,-1.)) ;
#117689=DIRECTION('ref_axis',(1.,0.,0.)) ;
#117690=DIRECTION('center_axis',(0.,0.,1.)) ;
#117691=DIRECTION('ref_axis',(1.,0.,0.)) ;
#117692=DIRECTION('',(-9.85638338623186E-18,-1.,0.)) ;
#117693=DIRECTION('',(1.,-9.85638338623186E-18,0.)) ;
#117694=DIRECTION('center_axis',(0.,0.,1.)) ;
#117695=DIRECTION('ref_axis',(1.,0.,0.)) ;
#117696=DIRECTION('',(9.85638338623186E-18,1.,0.)) ;
#117697=DIRECTION('center_axis',(0.,0.,-1.)) ;
#117698=DIRECTION('ref_axis',(1.,0.,0.)) ;
#117699=DIRECTION('center_axis',(0.,0.,1.)) ;
#117700=DIRECTION('ref_axis',(1.,0.,0.)) ;
#117701=DIRECTION('',(-9.85638338623186E-18,-1.,0.)) ;
#117702=DIRECTION('',(-1.,9.85638338623186E-18,0.)) ;
#117703=DIRECTION('center_axis',(0.,0.,-1.)) ;
#117704=DIRECTION('ref_axis',(-1.,0.,0.)) ;
#117705=DIRECTION('center_axis',(0.,0.,1.)) ;
#117706=DIRECTION('ref_axis',(1.,0.,0.)) ;
#117707=DIRECTION('center_axis',(0.,0.,-1.)) ;
#117708=DIRECTION('ref_axis',(1.,0.,0.)) ;
#117709=DIRECTION('center_axis',(0.,0.,-1.)) ;
#117710=DIRECTION('ref_axis',(-1.,0.,0.)) ;
#117711=DIRECTION('center_axis',(0.,0.,-1.)) ;
#117712=DIRECTION('ref_axis',(1.,0.,0.)) ;
#117713=DIRECTION('center_axis',(0.,0.,1.)) ;
#117714=DIRECTION('ref_axis',(1.,0.,0.)) ;
#117715=DIRECTION('center_axis',(-0.707106781186548,-0.707106781186547,
0.)) ;
#117716=DIRECTION('ref_axis',(0.707106781186547,-0.707106781186548,0.)) ;
#117717=DIRECTION('',(0.,0.,1.)) ;
#117718=DIRECTION('',(0.577350269189625,-0.577350269189626,-0.577350269189626)) ;
#117719=DIRECTION('',(0.,0.,-1.)) ;
#117720=DIRECTION('',(-0.577350269189625,0.577350269189626,-0.577350269189626)) ;
#117721=DIRECTION('center_axis',(1.95511867169517E-16,-1.,0.)) ;
#117722=DIRECTION('ref_axis',(1.,1.95511867169517E-16,0.)) ;
#117723=DIRECTION('',(0.,0.,-1.)) ;
#117724=DIRECTION('',(-1.,-1.95511867169517E-16,0.)) ;
#117725=DIRECTION('',(1.,1.95511867169517E-16,0.)) ;
#117726=DIRECTION('center_axis',(1.06642836637918E-16,1.,0.)) ;
#117727=DIRECTION('ref_axis',(-1.,1.06642836637918E-16,0.)) ;
#117728=DIRECTION('',(1.,-1.06642836637919E-16,0.)) ;
#117729=DIRECTION('',(0.,0.,1.)) ;
#117730=DIRECTION('',(-1.,1.06642836637919E-16,0.)) ;
#117731=DIRECTION('center_axis',(-0.707106781186548,0.707106781186547,0.)) ;
#117732=DIRECTION('ref_axis',(-0.707106781186547,-0.707106781186548,0.)) ;
#117733=DIRECTION('',(0.,0.,1.)) ;
#117734=DIRECTION('',(-0.577350269189625,-0.577350269189626,0.577350269189627)) ;
#117735=DIRECTION('',(0.,0.,-1.)) ;
#117736=DIRECTION('',(0.577350269189625,0.577350269189626,0.577350269189627)) ;
#117737=DIRECTION('center_axis',(-1.,0.,0.)) ;
#117738=DIRECTION('ref_axis',(0.,0.,1.)) ;
#117739=DIRECTION('',(0.,0.,-1.)) ;
#117740=DIRECTION('',(0.,1.,1.95511867169518E-16)) ;
#117741=DIRECTION('',(0.,0.,1.)) ;
#117742=DIRECTION('',(0.,-1.,1.95511867169518E-16)) ;
#117743=DIRECTION('center_axis',(0.,0.,1.)) ;
#117744=DIRECTION('ref_axis',(1.,0.,0.)) ;
#117745=DIRECTION('',(-1.95511867169517E-16,1.,0.)) ;
#117746=DIRECTION('',(-1.,-1.95511867169517E-16,0.)) ;
#117747=DIRECTION('',(1.,-1.06642836637919E-16,0.)) ;
#117748=DIRECTION('center_axis',(0.,0.,1.)) ;
#117749=DIRECTION('ref_axis',(1.,0.,0.)) ;
#117750=DIRECTION('',(1.,1.95511867169517E-16,0.)) ;
#117751=DIRECTION('',(1.95511867169517E-16,-1.,0.)) ;
#117752=DIRECTION('',(-1.,1.06642836637919E-16,0.)) ;
#117753=DIRECTION('center_axis',(1.,-9.85638338623186E-18,0.)) ;
#117754=DIRECTION('ref_axis',(9.85638338623186E-18,1.,0.)) ;
#117755=DIRECTION('',(0.,0.,-1.)) ;
#117756=DIRECTION('',(-9.85638338623186E-18,-1.,0.)) ;
#117757=DIRECTION('',(0.,0.,1.)) ;
#117758=DIRECTION('',(9.85638338623186E-18,1.,0.)) ;
#117759=DIRECTION('center_axis',(0.707106781186548,0.707106781186548,0.)) ;
#117760=DIRECTION('ref_axis',(-0.707106781186548,0.707106781186548,0.)) ;
#117761=DIRECTION('',(0.,0.,1.)) ;
#117762=DIRECTION('',(-0.577350269189625,0.577350269189625,0.577350269189627)) ;
#117763=DIRECTION('',(0.,0.,-1.)) ;
#117764=DIRECTION('',(0.577350269189625,-0.577350269189625,0.577350269189627)) ;
#117765=DIRECTION('center_axis',(0.,1.,0.)) ;
#117766=DIRECTION('ref_axis',(0.,0.,1.)) ;
#117767=DIRECTION('',(0.,0.,1.)) ;
#117768=DIRECTION('',(-1.,0.,-9.8563833862319E-18)) ;
#117769=DIRECTION('',(0.,0.,-1.)) ;
#117770=DIRECTION('',(1.,0.,-9.8563833862319E-18)) ;
#117771=DIRECTION('center_axis',(-0.707106781186548,0.707106781186548,0.)) ;
#117772=DIRECTION('ref_axis',(-0.707106781186548,-0.707106781186548,0.)) ;
#117773=DIRECTION('',(0.,0.,1.)) ;
#117774=DIRECTION('',(-0.577350269189625,-0.577350269189625,-0.577350269189627)) ;
#117775=DIRECTION('',(0.,0.,-1.)) ;
#117776=DIRECTION('',(0.577350269189625,0.577350269189625,-0.577350269189627)) ;
#117777=DIRECTION('center_axis',(-1.,9.85638338623186E-18,0.)) ;
#117778=DIRECTION('ref_axis',(-9.85638338623186E-18,-1.,0.)) ;
#117779=DIRECTION('',(0.,0.,-1.)) ;
#117780=DIRECTION('',(9.85638338623186E-18,1.,0.)) ;
#117781=DIRECTION('',(0.,0.,-1.)) ;
#117782=DIRECTION('',(-9.85638338623186E-18,-1.,0.)) ;
#117783=DIRECTION('center_axis',(0.,0.,1.)) ;
#117784=DIRECTION('ref_axis',(1.,0.,0.)) ;
#117785=DIRECTION('',(9.85638338623186E-18,1.,0.)) ;
#117786=DIRECTION('center_axis',(0.,0.,-1.)) ;
#117787=DIRECTION('ref_axis',(1.,0.,0.)) ;
#117788=DIRECTION('center_axis',(0.,0.,1.)) ;
#117789=DIRECTION('ref_axis',(1.,0.,0.)) ;
#117790=DIRECTION('',(-9.85638338623186E-18,-1.,0.)) ;
#117791=DIRECTION('',(1.,-9.85638338623186E-18,0.)) ;
#117792=DIRECTION('center_axis',(0.,0.,1.)) ;
#117793=DIRECTION('ref_axis',(1.,0.,0.)) ;
#117794=DIRECTION('',(9.85638338623186E-18,1.,0.)) ;
#117795=DIRECTION('center_axis',(0.,0.,-1.)) ;
#117796=DIRECTION('ref_axis',(1.,0.,0.)) ;
#117797=DIRECTION('center_axis',(0.,0.,1.)) ;
#117798=DIRECTION('ref_axis',(1.,0.,0.)) ;
#117799=DIRECTION('',(-9.85638338623186E-18,-1.,0.)) ;
#117800=DIRECTION('',(-1.,9.85638338623186E-18,0.)) ;
#117801=DIRECTION('center_axis',(0.,0.,-1.)) ;
#117802=DIRECTION('ref_axis',(-1.,0.,0.)) ;
#117803=DIRECTION('center_axis',(0.,0.,1.)) ;
#117804=DIRECTION('ref_axis',(1.,0.,0.)) ;
#117805=DIRECTION('center_axis',(0.,0.,-1.)) ;
#117806=DIRECTION('ref_axis',(1.,0.,0.)) ;
#117807=DIRECTION('center_axis',(0.,0.,-1.)) ;
#117808=DIRECTION('ref_axis',(-1.,0.,0.)) ;
#117809=DIRECTION('center_axis',(0.,0.,-1.)) ;
#117810=DIRECTION('ref_axis',(1.,0.,0.)) ;
#117811=DIRECTION('center_axis',(0.,0.,1.)) ;
#117812=DIRECTION('ref_axis',(1.,0.,0.)) ;
#117813=DIRECTION('center_axis',(-0.707106781186548,-0.707106781186547,
0.)) ;
#117814=DIRECTION('ref_axis',(0.707106781186547,-0.707106781186548,0.)) ;
#117815=DIRECTION('',(0.,0.,1.)) ;
#117816=DIRECTION('',(0.577350269189625,-0.577350269189626,-0.577350269189626)) ;
#117817=DIRECTION('',(0.,0.,-1.)) ;
#117818=DIRECTION('',(-0.577350269189625,0.577350269189626,-0.577350269189626)) ;
#117819=DIRECTION('center_axis',(1.95511867169517E-16,-1.,0.)) ;
#117820=DIRECTION('ref_axis',(1.,1.95511867169517E-16,0.)) ;
#117821=DIRECTION('',(0.,0.,-1.)) ;
#117822=DIRECTION('',(-1.,-1.95511867169517E-16,0.)) ;
#117823=DIRECTION('',(1.,1.95511867169517E-16,0.)) ;
#117824=DIRECTION('center_axis',(1.06642836637918E-16,1.,0.)) ;
#117825=DIRECTION('ref_axis',(-1.,1.06642836637918E-16,0.)) ;
#117826=DIRECTION('',(1.,-1.06642836637919E-16,0.)) ;
#117827=DIRECTION('',(0.,0.,1.)) ;
#117828=DIRECTION('',(-1.,1.06642836637919E-16,0.)) ;
#117829=DIRECTION('center_axis',(-0.707106781186548,0.707106781186547,0.)) ;
#117830=DIRECTION('ref_axis',(-0.707106781186547,-0.707106781186548,0.)) ;
#117831=DIRECTION('',(0.,0.,1.)) ;
#117832=DIRECTION('',(-0.577350269189625,-0.577350269189626,0.577350269189627)) ;
#117833=DIRECTION('',(0.,0.,-1.)) ;
#117834=DIRECTION('',(0.577350269189625,0.577350269189626,0.577350269189627)) ;
#117835=DIRECTION('center_axis',(-1.,0.,0.)) ;
#117836=DIRECTION('ref_axis',(0.,0.,1.)) ;
#117837=DIRECTION('',(0.,0.,-1.)) ;
#117838=DIRECTION('',(0.,1.,1.95511867169518E-16)) ;
#117839=DIRECTION('',(0.,0.,1.)) ;
#117840=DIRECTION('',(0.,-1.,1.95511867169518E-16)) ;
#117841=DIRECTION('center_axis',(0.,0.,1.)) ;
#117842=DIRECTION('ref_axis',(1.,0.,0.)) ;
#117843=DIRECTION('',(-1.95511867169517E-16,1.,0.)) ;
#117844=DIRECTION('',(-1.,-1.95511867169517E-16,0.)) ;
#117845=DIRECTION('',(1.,-1.06642836637919E-16,0.)) ;
#117846=DIRECTION('center_axis',(0.,0.,1.)) ;
#117847=DIRECTION('ref_axis',(1.,0.,0.)) ;
#117848=DIRECTION('',(1.,1.95511867169517E-16,0.)) ;
#117849=DIRECTION('',(1.95511867169517E-16,-1.,0.)) ;
#117850=DIRECTION('',(-1.,1.06642836637919E-16,0.)) ;
#117851=DIRECTION('center_axis',(1.,-9.85638338623186E-18,0.)) ;
#117852=DIRECTION('ref_axis',(9.85638338623186E-18,1.,0.)) ;
#117853=DIRECTION('',(0.,0.,-1.)) ;
#117854=DIRECTION('',(-9.85638338623186E-18,-1.,0.)) ;
#117855=DIRECTION('',(0.,0.,1.)) ;
#117856=DIRECTION('',(9.85638338623186E-18,1.,0.)) ;
#117857=DIRECTION('center_axis',(0.707106781186548,0.707106781186548,0.)) ;
#117858=DIRECTION('ref_axis',(-0.707106781186548,0.707106781186548,0.)) ;
#117859=DIRECTION('',(0.,0.,1.)) ;
#117860=DIRECTION('',(-0.577350269189625,0.577350269189625,0.577350269189627)) ;
#117861=DIRECTION('',(0.,0.,-1.)) ;
#117862=DIRECTION('',(0.577350269189625,-0.577350269189625,0.577350269189627)) ;
#117863=DIRECTION('center_axis',(0.,1.,0.)) ;
#117864=DIRECTION('ref_axis',(0.,0.,1.)) ;
#117865=DIRECTION('',(0.,0.,1.)) ;
#117866=DIRECTION('',(-1.,0.,-9.8563833862319E-18)) ;
#117867=DIRECTION('',(0.,0.,-1.)) ;
#117868=DIRECTION('',(1.,0.,-9.8563833862319E-18)) ;
#117869=DIRECTION('center_axis',(-0.707106781186548,0.707106781186548,0.)) ;
#117870=DIRECTION('ref_axis',(-0.707106781186548,-0.707106781186548,0.)) ;
#117871=DIRECTION('',(0.,0.,1.)) ;
#117872=DIRECTION('',(-0.577350269189625,-0.577350269189625,-0.577350269189627)) ;
#117873=DIRECTION('',(0.,0.,-1.)) ;
#117874=DIRECTION('',(0.577350269189625,0.577350269189625,-0.577350269189627)) ;
#117875=DIRECTION('center_axis',(-1.,9.85638338623186E-18,0.)) ;
#117876=DIRECTION('ref_axis',(-9.85638338623186E-18,-1.,0.)) ;
#117877=DIRECTION('',(0.,0.,-1.)) ;
#117878=DIRECTION('',(9.85638338623186E-18,1.,0.)) ;
#117879=DIRECTION('',(0.,0.,-1.)) ;
#117880=DIRECTION('',(-9.85638338623186E-18,-1.,0.)) ;
#117881=DIRECTION('center_axis',(0.,0.,1.)) ;
#117882=DIRECTION('ref_axis',(1.,0.,0.)) ;
#117883=DIRECTION('',(9.85638338623186E-18,1.,0.)) ;
#117884=DIRECTION('center_axis',(0.,0.,-1.)) ;
#117885=DIRECTION('ref_axis',(1.,0.,0.)) ;
#117886=DIRECTION('center_axis',(0.,0.,1.)) ;
#117887=DIRECTION('ref_axis',(1.,0.,0.)) ;
#117888=DIRECTION('',(-9.85638338623186E-18,-1.,0.)) ;
#117889=DIRECTION('',(1.,-9.85638338623186E-18,0.)) ;
#117890=DIRECTION('center_axis',(0.,0.,1.)) ;
#117891=DIRECTION('ref_axis',(1.,0.,0.)) ;
#117892=DIRECTION('',(9.85638338623186E-18,1.,0.)) ;
#117893=DIRECTION('center_axis',(0.,0.,-1.)) ;
#117894=DIRECTION('ref_axis',(1.,0.,0.)) ;
#117895=DIRECTION('center_axis',(0.,0.,1.)) ;
#117896=DIRECTION('ref_axis',(1.,0.,0.)) ;
#117897=DIRECTION('',(-9.85638338623186E-18,-1.,0.)) ;
#117898=DIRECTION('',(-1.,9.85638338623186E-18,0.)) ;
#117899=DIRECTION('center_axis',(0.,0.,-1.)) ;
#117900=DIRECTION('ref_axis',(-1.,0.,0.)) ;
#117901=DIRECTION('center_axis',(0.,0.,1.)) ;
#117902=DIRECTION('ref_axis',(1.,0.,0.)) ;
#117903=DIRECTION('center_axis',(0.,0.,-1.)) ;
#117904=DIRECTION('ref_axis',(1.,0.,0.)) ;
#117905=DIRECTION('center_axis',(0.,0.,-1.)) ;
#117906=DIRECTION('ref_axis',(-1.,0.,0.)) ;
#117907=DIRECTION('center_axis',(0.,0.,-1.)) ;
#117908=DIRECTION('ref_axis',(1.,0.,0.)) ;
#117909=DIRECTION('center_axis',(0.,0.,1.)) ;
#117910=DIRECTION('ref_axis',(1.,0.,0.)) ;
#117911=DIRECTION('center_axis',(-0.707106781186548,-0.707106781186547,
0.)) ;
#117912=DIRECTION('ref_axis',(0.707106781186547,-0.707106781186548,0.)) ;
#117913=DIRECTION('',(0.,0.,1.)) ;
#117914=DIRECTION('',(0.577350269189625,-0.577350269189626,-0.577350269189626)) ;
#117915=DIRECTION('',(0.,0.,-1.)) ;
#117916=DIRECTION('',(-0.577350269189625,0.577350269189626,-0.577350269189626)) ;
#117917=DIRECTION('center_axis',(1.95511867169517E-16,-1.,0.)) ;
#117918=DIRECTION('ref_axis',(1.,1.95511867169517E-16,0.)) ;
#117919=DIRECTION('',(0.,0.,-1.)) ;
#117920=DIRECTION('',(-1.,-1.95511867169517E-16,0.)) ;
#117921=DIRECTION('',(1.,1.95511867169517E-16,0.)) ;
#117922=DIRECTION('center_axis',(1.06642836637918E-16,1.,0.)) ;
#117923=DIRECTION('ref_axis',(-1.,1.06642836637918E-16,0.)) ;
#117924=DIRECTION('',(1.,-1.06642836637919E-16,0.)) ;
#117925=DIRECTION('',(0.,0.,1.)) ;
#117926=DIRECTION('',(-1.,1.06642836637919E-16,0.)) ;
#117927=DIRECTION('center_axis',(-0.707106781186548,0.707106781186547,0.)) ;
#117928=DIRECTION('ref_axis',(-0.707106781186547,-0.707106781186548,0.)) ;
#117929=DIRECTION('',(0.,0.,1.)) ;
#117930=DIRECTION('',(-0.577350269189625,-0.577350269189626,0.577350269189627)) ;
#117931=DIRECTION('',(0.,0.,-1.)) ;
#117932=DIRECTION('',(0.577350269189625,0.577350269189626,0.577350269189627)) ;
#117933=DIRECTION('center_axis',(-1.,0.,0.)) ;
#117934=DIRECTION('ref_axis',(0.,0.,1.)) ;
#117935=DIRECTION('',(0.,0.,-1.)) ;
#117936=DIRECTION('',(0.,1.,1.95511867169518E-16)) ;
#117937=DIRECTION('',(0.,0.,1.)) ;
#117938=DIRECTION('',(0.,-1.,1.95511867169518E-16)) ;
#117939=DIRECTION('center_axis',(0.,0.,1.)) ;
#117940=DIRECTION('ref_axis',(1.,0.,0.)) ;
#117941=DIRECTION('',(-1.95511867169517E-16,1.,0.)) ;
#117942=DIRECTION('',(-1.,-1.95511867169517E-16,0.)) ;
#117943=DIRECTION('',(1.,-1.06642836637919E-16,0.)) ;
#117944=DIRECTION('center_axis',(0.,0.,1.)) ;
#117945=DIRECTION('ref_axis',(1.,0.,0.)) ;
#117946=DIRECTION('',(1.,1.95511867169517E-16,0.)) ;
#117947=DIRECTION('',(1.95511867169517E-16,-1.,0.)) ;
#117948=DIRECTION('',(-1.,1.06642836637919E-16,0.)) ;
#117949=DIRECTION('center_axis',(1.,-9.85638338623186E-18,0.)) ;
#117950=DIRECTION('ref_axis',(9.85638338623186E-18,1.,0.)) ;
#117951=DIRECTION('',(0.,0.,-1.)) ;
#117952=DIRECTION('',(-9.85638338623186E-18,-1.,0.)) ;
#117953=DIRECTION('',(0.,0.,1.)) ;
#117954=DIRECTION('',(9.85638338623186E-18,1.,0.)) ;
#117955=DIRECTION('center_axis',(0.707106781186548,0.707106781186548,0.)) ;
#117956=DIRECTION('ref_axis',(-0.707106781186548,0.707106781186548,0.)) ;
#117957=DIRECTION('',(0.,0.,1.)) ;
#117958=DIRECTION('',(-0.577350269189625,0.577350269189625,0.577350269189627)) ;
#117959=DIRECTION('',(0.,0.,-1.)) ;
#117960=DIRECTION('',(0.577350269189625,-0.577350269189625,0.577350269189627)) ;
#117961=DIRECTION('center_axis',(0.,1.,0.)) ;
#117962=DIRECTION('ref_axis',(0.,0.,1.)) ;
#117963=DIRECTION('',(0.,0.,1.)) ;
#117964=DIRECTION('',(-1.,0.,-9.8563833862319E-18)) ;
#117965=DIRECTION('',(0.,0.,-1.)) ;
#117966=DIRECTION('',(1.,0.,-9.8563833862319E-18)) ;
#117967=DIRECTION('center_axis',(-0.707106781186548,0.707106781186548,0.)) ;
#117968=DIRECTION('ref_axis',(-0.707106781186548,-0.707106781186548,0.)) ;
#117969=DIRECTION('',(0.,0.,1.)) ;
#117970=DIRECTION('',(-0.577350269189625,-0.577350269189625,-0.577350269189627)) ;
#117971=DIRECTION('',(0.,0.,-1.)) ;
#117972=DIRECTION('',(0.577350269189625,0.577350269189625,-0.577350269189627)) ;
#117973=DIRECTION('center_axis',(-1.,9.85638338623186E-18,0.)) ;
#117974=DIRECTION('ref_axis',(-9.85638338623186E-18,-1.,0.)) ;
#117975=DIRECTION('',(0.,0.,-1.)) ;
#117976=DIRECTION('',(9.85638338623186E-18,1.,0.)) ;
#117977=DIRECTION('',(0.,0.,-1.)) ;
#117978=DIRECTION('',(-9.85638338623186E-18,-1.,0.)) ;
#117979=DIRECTION('center_axis',(0.,0.,1.)) ;
#117980=DIRECTION('ref_axis',(1.,0.,0.)) ;
#117981=DIRECTION('',(9.85638338623186E-18,1.,0.)) ;
#117982=DIRECTION('center_axis',(0.,0.,-1.)) ;
#117983=DIRECTION('ref_axis',(1.,0.,0.)) ;
#117984=DIRECTION('center_axis',(0.,0.,1.)) ;
#117985=DIRECTION('ref_axis',(1.,0.,0.)) ;
#117986=DIRECTION('',(-9.85638338623186E-18,-1.,0.)) ;
#117987=DIRECTION('',(1.,-9.85638338623186E-18,0.)) ;
#117988=DIRECTION('center_axis',(0.,0.,1.)) ;
#117989=DIRECTION('ref_axis',(1.,0.,0.)) ;
#117990=DIRECTION('',(9.85638338623186E-18,1.,0.)) ;
#117991=DIRECTION('center_axis',(0.,0.,-1.)) ;
#117992=DIRECTION('ref_axis',(1.,0.,0.)) ;
#117993=DIRECTION('center_axis',(0.,0.,1.)) ;
#117994=DIRECTION('ref_axis',(1.,0.,0.)) ;
#117995=DIRECTION('',(-9.85638338623186E-18,-1.,0.)) ;
#117996=DIRECTION('',(-1.,9.85638338623186E-18,0.)) ;
#117997=DIRECTION('center_axis',(0.,0.,-1.)) ;
#117998=DIRECTION('ref_axis',(-1.,0.,0.)) ;
#117999=DIRECTION('center_axis',(0.,0.,1.)) ;
#118000=DIRECTION('ref_axis',(1.,0.,0.)) ;
#118001=DIRECTION('center_axis',(0.,0.,-1.)) ;
#118002=DIRECTION('ref_axis',(1.,0.,0.)) ;
#118003=DIRECTION('center_axis',(0.,0.,-1.)) ;
#118004=DIRECTION('ref_axis',(-1.,0.,0.)) ;
#118005=DIRECTION('center_axis',(0.,0.,-1.)) ;
#118006=DIRECTION('ref_axis',(1.,0.,0.)) ;
#118007=DIRECTION('center_axis',(0.,0.,1.)) ;
#118008=DIRECTION('ref_axis',(1.,0.,0.)) ;
#118009=DIRECTION('center_axis',(-0.707106781186548,-0.707106781186547,
0.)) ;
#118010=DIRECTION('ref_axis',(0.707106781186547,-0.707106781186548,0.)) ;
#118011=DIRECTION('',(0.,0.,1.)) ;
#118012=DIRECTION('',(0.577350269189625,-0.577350269189626,-0.577350269189626)) ;
#118013=DIRECTION('',(0.,0.,-1.)) ;
#118014=DIRECTION('',(-0.577350269189625,0.577350269189626,-0.577350269189626)) ;
#118015=DIRECTION('center_axis',(1.95511867169517E-16,-1.,0.)) ;
#118016=DIRECTION('ref_axis',(1.,1.95511867169517E-16,0.)) ;
#118017=DIRECTION('',(0.,0.,-1.)) ;
#118018=DIRECTION('',(-1.,-1.95511867169517E-16,0.)) ;
#118019=DIRECTION('',(1.,1.95511867169517E-16,0.)) ;
#118020=DIRECTION('center_axis',(1.06642836637918E-16,1.,0.)) ;
#118021=DIRECTION('ref_axis',(-1.,1.06642836637918E-16,0.)) ;
#118022=DIRECTION('',(1.,-1.06642836637919E-16,0.)) ;
#118023=DIRECTION('',(0.,0.,1.)) ;
#118024=DIRECTION('',(-1.,1.06642836637919E-16,0.)) ;
#118025=DIRECTION('center_axis',(-0.707106781186548,0.707106781186547,0.)) ;
#118026=DIRECTION('ref_axis',(-0.707106781186547,-0.707106781186548,0.)) ;
#118027=DIRECTION('',(0.,0.,1.)) ;
#118028=DIRECTION('',(-0.577350269189625,-0.577350269189626,0.577350269189627)) ;
#118029=DIRECTION('',(0.,0.,-1.)) ;
#118030=DIRECTION('',(0.577350269189625,0.577350269189626,0.577350269189627)) ;
#118031=DIRECTION('center_axis',(-1.,0.,0.)) ;
#118032=DIRECTION('ref_axis',(0.,0.,1.)) ;
#118033=DIRECTION('',(0.,0.,-1.)) ;
#118034=DIRECTION('',(0.,1.,1.95511867169518E-16)) ;
#118035=DIRECTION('',(0.,0.,1.)) ;
#118036=DIRECTION('',(0.,-1.,1.95511867169518E-16)) ;
#118037=DIRECTION('center_axis',(0.,0.,1.)) ;
#118038=DIRECTION('ref_axis',(1.,0.,0.)) ;
#118039=DIRECTION('',(-1.95511867169517E-16,1.,0.)) ;
#118040=DIRECTION('',(-1.,-1.95511867169517E-16,0.)) ;
#118041=DIRECTION('',(1.,-1.06642836637919E-16,0.)) ;
#118042=DIRECTION('center_axis',(0.,0.,1.)) ;
#118043=DIRECTION('ref_axis',(1.,0.,0.)) ;
#118044=DIRECTION('',(1.,1.95511867169517E-16,0.)) ;
#118045=DIRECTION('',(1.95511867169517E-16,-1.,0.)) ;
#118046=DIRECTION('',(-1.,1.06642836637919E-16,0.)) ;
#118047=DIRECTION('center_axis',(1.,-9.85638338623186E-18,0.)) ;
#118048=DIRECTION('ref_axis',(9.85638338623186E-18,1.,0.)) ;
#118049=DIRECTION('',(0.,0.,-1.)) ;
#118050=DIRECTION('',(-9.85638338623186E-18,-1.,0.)) ;
#118051=DIRECTION('',(0.,0.,1.)) ;
#118052=DIRECTION('',(9.85638338623186E-18,1.,0.)) ;
#118053=DIRECTION('center_axis',(0.707106781186548,0.707106781186548,0.)) ;
#118054=DIRECTION('ref_axis',(-0.707106781186548,0.707106781186548,0.)) ;
#118055=DIRECTION('',(0.,0.,1.)) ;
#118056=DIRECTION('',(-0.577350269189625,0.577350269189625,0.577350269189627)) ;
#118057=DIRECTION('',(0.,0.,-1.)) ;
#118058=DIRECTION('',(0.577350269189625,-0.577350269189625,0.577350269189627)) ;
#118059=DIRECTION('center_axis',(0.,1.,0.)) ;
#118060=DIRECTION('ref_axis',(0.,0.,1.)) ;
#118061=DIRECTION('',(0.,0.,1.)) ;
#118062=DIRECTION('',(-1.,0.,-9.8563833862319E-18)) ;
#118063=DIRECTION('',(0.,0.,-1.)) ;
#118064=DIRECTION('',(1.,0.,-9.8563833862319E-18)) ;
#118065=DIRECTION('center_axis',(-0.707106781186548,0.707106781186548,0.)) ;
#118066=DIRECTION('ref_axis',(-0.707106781186548,-0.707106781186548,0.)) ;
#118067=DIRECTION('',(0.,0.,1.)) ;
#118068=DIRECTION('',(-0.577350269189625,-0.577350269189625,-0.577350269189627)) ;
#118069=DIRECTION('',(0.,0.,-1.)) ;
#118070=DIRECTION('',(0.577350269189625,0.577350269189625,-0.577350269189627)) ;
#118071=DIRECTION('center_axis',(-1.,9.85638338623186E-18,0.)) ;
#118072=DIRECTION('ref_axis',(-9.85638338623186E-18,-1.,0.)) ;
#118073=DIRECTION('',(0.,0.,-1.)) ;
#118074=DIRECTION('',(9.85638338623186E-18,1.,0.)) ;
#118075=DIRECTION('',(0.,0.,-1.)) ;
#118076=DIRECTION('',(-9.85638338623186E-18,-1.,0.)) ;
#118077=DIRECTION('center_axis',(0.,0.,1.)) ;
#118078=DIRECTION('ref_axis',(1.,0.,0.)) ;
#118079=DIRECTION('',(9.85638338623186E-18,1.,0.)) ;
#118080=DIRECTION('center_axis',(0.,0.,-1.)) ;
#118081=DIRECTION('ref_axis',(1.,0.,0.)) ;
#118082=DIRECTION('center_axis',(0.,0.,1.)) ;
#118083=DIRECTION('ref_axis',(1.,0.,0.)) ;
#118084=DIRECTION('',(-9.85638338623186E-18,-1.,0.)) ;
#118085=DIRECTION('',(1.,-9.85638338623186E-18,0.)) ;
#118086=DIRECTION('center_axis',(0.,0.,1.)) ;
#118087=DIRECTION('ref_axis',(1.,0.,0.)) ;
#118088=DIRECTION('',(9.85638338623186E-18,1.,0.)) ;
#118089=DIRECTION('center_axis',(0.,0.,-1.)) ;
#118090=DIRECTION('ref_axis',(1.,0.,0.)) ;
#118091=DIRECTION('center_axis',(0.,0.,1.)) ;
#118092=DIRECTION('ref_axis',(1.,0.,0.)) ;
#118093=DIRECTION('',(-9.85638338623186E-18,-1.,0.)) ;
#118094=DIRECTION('',(-1.,9.85638338623186E-18,0.)) ;
#118095=DIRECTION('center_axis',(0.,0.,-1.)) ;
#118096=DIRECTION('ref_axis',(-1.,0.,0.)) ;
#118097=DIRECTION('center_axis',(0.,0.,1.)) ;
#118098=DIRECTION('ref_axis',(1.,0.,0.)) ;
#118099=DIRECTION('center_axis',(0.,0.,-1.)) ;
#118100=DIRECTION('ref_axis',(1.,0.,0.)) ;
#118101=DIRECTION('center_axis',(0.,0.,-1.)) ;
#118102=DIRECTION('ref_axis',(-1.,0.,0.)) ;
#118103=DIRECTION('center_axis',(0.,0.,-1.)) ;
#118104=DIRECTION('ref_axis',(1.,0.,0.)) ;
#118105=DIRECTION('center_axis',(0.,0.,1.)) ;
#118106=DIRECTION('ref_axis',(1.,0.,0.)) ;
#118107=DIRECTION('center_axis',(-0.707106781186548,-0.707106781186547,
0.)) ;
#118108=DIRECTION('ref_axis',(0.707106781186547,-0.707106781186548,0.)) ;
#118109=DIRECTION('',(0.,0.,1.)) ;
#118110=DIRECTION('',(0.577350269189625,-0.577350269189626,-0.577350269189626)) ;
#118111=DIRECTION('',(0.,0.,-1.)) ;
#118112=DIRECTION('',(-0.577350269189625,0.577350269189626,-0.577350269189626)) ;
#118113=DIRECTION('center_axis',(1.95511867169517E-16,-1.,0.)) ;
#118114=DIRECTION('ref_axis',(1.,1.95511867169517E-16,0.)) ;
#118115=DIRECTION('',(0.,0.,-1.)) ;
#118116=DIRECTION('',(-1.,-1.95511867169517E-16,0.)) ;
#118117=DIRECTION('',(1.,1.95511867169517E-16,0.)) ;
#118118=DIRECTION('center_axis',(1.06642836637918E-16,1.,0.)) ;
#118119=DIRECTION('ref_axis',(-1.,1.06642836637918E-16,0.)) ;
#118120=DIRECTION('',(1.,-1.06642836637919E-16,0.)) ;
#118121=DIRECTION('',(0.,0.,1.)) ;
#118122=DIRECTION('',(-1.,1.06642836637919E-16,0.)) ;
#118123=DIRECTION('center_axis',(-0.707106781186548,0.707106781186547,0.)) ;
#118124=DIRECTION('ref_axis',(-0.707106781186547,-0.707106781186548,0.)) ;
#118125=DIRECTION('',(0.,0.,1.)) ;
#118126=DIRECTION('',(-0.577350269189625,-0.577350269189626,0.577350269189627)) ;
#118127=DIRECTION('',(0.,0.,-1.)) ;
#118128=DIRECTION('',(0.577350269189625,0.577350269189626,0.577350269189627)) ;
#118129=DIRECTION('center_axis',(-1.,0.,0.)) ;
#118130=DIRECTION('ref_axis',(0.,0.,1.)) ;
#118131=DIRECTION('',(0.,0.,-1.)) ;
#118132=DIRECTION('',(0.,1.,1.95511867169518E-16)) ;
#118133=DIRECTION('',(0.,0.,1.)) ;
#118134=DIRECTION('',(0.,-1.,1.95511867169518E-16)) ;
#118135=DIRECTION('center_axis',(0.,0.,1.)) ;
#118136=DIRECTION('ref_axis',(1.,0.,0.)) ;
#118137=DIRECTION('',(-1.95511867169517E-16,1.,0.)) ;
#118138=DIRECTION('',(-1.,-1.95511867169517E-16,0.)) ;
#118139=DIRECTION('',(1.,-1.06642836637919E-16,0.)) ;
#118140=DIRECTION('center_axis',(0.,0.,1.)) ;
#118141=DIRECTION('ref_axis',(1.,0.,0.)) ;
#118142=DIRECTION('',(1.,1.95511867169517E-16,0.)) ;
#118143=DIRECTION('',(1.95511867169517E-16,-1.,0.)) ;
#118144=DIRECTION('',(-1.,1.06642836637919E-16,0.)) ;
#118145=DIRECTION('center_axis',(1.,-9.85638338623186E-18,0.)) ;
#118146=DIRECTION('ref_axis',(9.85638338623186E-18,1.,0.)) ;
#118147=DIRECTION('',(0.,0.,-1.)) ;
#118148=DIRECTION('',(-9.85638338623186E-18,-1.,0.)) ;
#118149=DIRECTION('',(0.,0.,1.)) ;
#118150=DIRECTION('',(9.85638338623186E-18,1.,0.)) ;
#118151=DIRECTION('center_axis',(0.707106781186548,0.707106781186548,0.)) ;
#118152=DIRECTION('ref_axis',(-0.707106781186548,0.707106781186548,0.)) ;
#118153=DIRECTION('',(0.,0.,1.)) ;
#118154=DIRECTION('',(-0.577350269189625,0.577350269189625,0.577350269189627)) ;
#118155=DIRECTION('',(0.,0.,-1.)) ;
#118156=DIRECTION('',(0.577350269189625,-0.577350269189625,0.577350269189627)) ;
#118157=DIRECTION('center_axis',(0.,1.,0.)) ;
#118158=DIRECTION('ref_axis',(0.,0.,1.)) ;
#118159=DIRECTION('',(0.,0.,1.)) ;
#118160=DIRECTION('',(-1.,0.,-9.8563833862319E-18)) ;
#118161=DIRECTION('',(0.,0.,-1.)) ;
#118162=DIRECTION('',(1.,0.,-9.8563833862319E-18)) ;
#118163=DIRECTION('center_axis',(-0.707106781186548,0.707106781186548,0.)) ;
#118164=DIRECTION('ref_axis',(-0.707106781186548,-0.707106781186548,0.)) ;
#118165=DIRECTION('',(0.,0.,1.)) ;
#118166=DIRECTION('',(-0.577350269189625,-0.577350269189625,-0.577350269189627)) ;
#118167=DIRECTION('',(0.,0.,-1.)) ;
#118168=DIRECTION('',(0.577350269189625,0.577350269189625,-0.577350269189627)) ;
#118169=DIRECTION('center_axis',(-1.,9.85638338623186E-18,0.)) ;
#118170=DIRECTION('ref_axis',(-9.85638338623186E-18,-1.,0.)) ;
#118171=DIRECTION('',(0.,0.,-1.)) ;
#118172=DIRECTION('',(9.85638338623186E-18,1.,0.)) ;
#118173=DIRECTION('',(0.,0.,-1.)) ;
#118174=DIRECTION('',(-9.85638338623186E-18,-1.,0.)) ;
#118175=DIRECTION('center_axis',(0.,0.,1.)) ;
#118176=DIRECTION('ref_axis',(1.,0.,0.)) ;
#118177=DIRECTION('',(9.85638338623186E-18,1.,0.)) ;
#118178=DIRECTION('center_axis',(0.,0.,-1.)) ;
#118179=DIRECTION('ref_axis',(1.,0.,0.)) ;
#118180=DIRECTION('center_axis',(0.,0.,1.)) ;
#118181=DIRECTION('ref_axis',(1.,0.,0.)) ;
#118182=DIRECTION('',(-9.85638338623186E-18,-1.,0.)) ;
#118183=DIRECTION('',(1.,-9.85638338623186E-18,0.)) ;
#118184=DIRECTION('center_axis',(0.,0.,1.)) ;
#118185=DIRECTION('ref_axis',(1.,0.,0.)) ;
#118186=DIRECTION('',(9.85638338623186E-18,1.,0.)) ;
#118187=DIRECTION('center_axis',(0.,0.,-1.)) ;
#118188=DIRECTION('ref_axis',(1.,0.,0.)) ;
#118189=DIRECTION('center_axis',(0.,0.,1.)) ;
#118190=DIRECTION('ref_axis',(1.,0.,0.)) ;
#118191=DIRECTION('',(-9.85638338623186E-18,-1.,0.)) ;
#118192=DIRECTION('',(-1.,9.85638338623186E-18,0.)) ;
#118193=DIRECTION('center_axis',(0.,0.,-1.)) ;
#118194=DIRECTION('ref_axis',(-1.,0.,0.)) ;
#118195=DIRECTION('center_axis',(0.,0.,1.)) ;
#118196=DIRECTION('ref_axis',(1.,0.,0.)) ;
#118197=DIRECTION('center_axis',(0.,0.,-1.)) ;
#118198=DIRECTION('ref_axis',(1.,0.,0.)) ;
#118199=DIRECTION('center_axis',(0.,0.,-1.)) ;
#118200=DIRECTION('ref_axis',(-1.,0.,0.)) ;
#118201=DIRECTION('center_axis',(0.,0.,-1.)) ;
#118202=DIRECTION('ref_axis',(1.,0.,0.)) ;
#118203=DIRECTION('center_axis',(0.,0.,1.)) ;
#118204=DIRECTION('ref_axis',(1.,0.,0.)) ;
#118205=DIRECTION('center_axis',(-0.707106781186548,-0.707106781186547,
0.)) ;
#118206=DIRECTION('ref_axis',(0.707106781186547,-0.707106781186548,0.)) ;
#118207=DIRECTION('',(0.,0.,1.)) ;
#118208=DIRECTION('',(0.577350269189625,-0.577350269189626,-0.577350269189626)) ;
#118209=DIRECTION('',(0.,0.,-1.)) ;
#118210=DIRECTION('',(-0.577350269189625,0.577350269189626,-0.577350269189626)) ;
#118211=DIRECTION('center_axis',(1.95511867169517E-16,-1.,0.)) ;
#118212=DIRECTION('ref_axis',(1.,1.95511867169517E-16,0.)) ;
#118213=DIRECTION('',(0.,0.,-1.)) ;
#118214=DIRECTION('',(-1.,-1.95511867169517E-16,0.)) ;
#118215=DIRECTION('',(1.,1.95511867169517E-16,0.)) ;
#118216=DIRECTION('center_axis',(1.06642836637918E-16,1.,0.)) ;
#118217=DIRECTION('ref_axis',(-1.,1.06642836637918E-16,0.)) ;
#118218=DIRECTION('',(1.,-1.06642836637919E-16,0.)) ;
#118219=DIRECTION('',(0.,0.,1.)) ;
#118220=DIRECTION('',(-1.,1.06642836637919E-16,0.)) ;
#118221=DIRECTION('center_axis',(-0.707106781186548,0.707106781186547,0.)) ;
#118222=DIRECTION('ref_axis',(-0.707106781186547,-0.707106781186548,0.)) ;
#118223=DIRECTION('',(0.,0.,1.)) ;
#118224=DIRECTION('',(-0.577350269189625,-0.577350269189626,0.577350269189627)) ;
#118225=DIRECTION('',(0.,0.,-1.)) ;
#118226=DIRECTION('',(0.577350269189625,0.577350269189626,0.577350269189627)) ;
#118227=DIRECTION('center_axis',(-1.,0.,0.)) ;
#118228=DIRECTION('ref_axis',(0.,0.,1.)) ;
#118229=DIRECTION('',(0.,0.,-1.)) ;
#118230=DIRECTION('',(0.,1.,1.95511867169518E-16)) ;
#118231=DIRECTION('',(0.,0.,1.)) ;
#118232=DIRECTION('',(0.,-1.,1.95511867169518E-16)) ;
#118233=DIRECTION('center_axis',(0.,0.,1.)) ;
#118234=DIRECTION('ref_axis',(1.,0.,0.)) ;
#118235=DIRECTION('',(-1.95511867169517E-16,1.,0.)) ;
#118236=DIRECTION('',(-1.,-1.95511867169517E-16,0.)) ;
#118237=DIRECTION('',(1.,-1.06642836637919E-16,0.)) ;
#118238=DIRECTION('center_axis',(0.,0.,1.)) ;
#118239=DIRECTION('ref_axis',(1.,0.,0.)) ;
#118240=DIRECTION('',(1.,1.95511867169517E-16,0.)) ;
#118241=DIRECTION('',(1.95511867169517E-16,-1.,0.)) ;
#118242=DIRECTION('',(-1.,1.06642836637919E-16,0.)) ;
#118243=DIRECTION('center_axis',(6.96951553037899E-18,0.707106781186549,
0.707106781186546)) ;
#118244=DIRECTION('ref_axis',(-8.6424177776148E-34,-0.707106781186546,0.707106781186549)) ;
#118245=DIRECTION('',(-0.577350269189625,0.577350269189625,-0.577350269189627)) ;
#118246=DIRECTION('',(1.,-9.85638338623186E-18,0.)) ;
#118247=DIRECTION('',(-0.577350269189625,-0.577350269189625,0.577350269189627)) ;
#118248=DIRECTION('',(-1.,7.70371977754894E-34,9.8563833862319E-18)) ;
#118249=DIRECTION('center_axis',(6.96951553037899E-18,0.707106781186549,
-0.707106781186546)) ;
#118250=DIRECTION('ref_axis',(8.6424177776148E-34,0.707106781186546,0.707106781186549)) ;
#118251=DIRECTION('',(0.577350269189625,0.577350269189625,0.577350269189627)) ;
#118252=DIRECTION('',(-1.,9.85638338623186E-18,0.)) ;
#118253=DIRECTION('',(0.577350269189625,-0.577350269189625,-0.577350269189627)) ;
#118254=DIRECTION('',(1.,-7.70371977754894E-34,9.8563833862319E-18)) ;
#118255=DIRECTION('center_axis',(6.96951553037899E-18,0.707106781186549,
0.707106781186546)) ;
#118256=DIRECTION('ref_axis',(-8.6424177776148E-34,-0.707106781186546,0.707106781186549)) ;
#118257=DIRECTION('',(-0.577350269189625,0.577350269189625,-0.577350269189627)) ;
#118258=DIRECTION('',(1.,-9.85638338623186E-18,0.)) ;
#118259=DIRECTION('',(-0.577350269189625,-0.577350269189625,0.577350269189627)) ;
#118260=DIRECTION('',(-1.,7.70371977754894E-34,9.8563833862319E-18)) ;
#118261=DIRECTION('center_axis',(6.96951553037899E-18,0.707106781186549,
-0.707106781186546)) ;
#118262=DIRECTION('ref_axis',(8.6424177776148E-34,0.707106781186546,0.707106781186549)) ;
#118263=DIRECTION('',(0.577350269189625,0.577350269189625,0.577350269189627)) ;
#118264=DIRECTION('',(-1.,9.85638338623186E-18,0.)) ;
#118265=DIRECTION('',(0.577350269189625,-0.577350269189625,-0.577350269189627)) ;
#118266=DIRECTION('',(1.,-7.70371977754894E-34,9.8563833862319E-18)) ;
#118267=DIRECTION('center_axis',(6.96951553037899E-18,0.707106781186549,
0.707106781186546)) ;
#118268=DIRECTION('ref_axis',(-8.6424177776148E-34,-0.707106781186546,0.707106781186549)) ;
#118269=DIRECTION('',(-0.577350269189625,0.577350269189625,-0.577350269189627)) ;
#118270=DIRECTION('',(1.,-9.85638338623186E-18,0.)) ;
#118271=DIRECTION('',(-0.577350269189625,-0.577350269189625,0.577350269189627)) ;
#118272=DIRECTION('',(-1.,7.70371977754894E-34,9.8563833862319E-18)) ;
#118273=DIRECTION('center_axis',(6.96951553037899E-18,0.707106781186549,
-0.707106781186546)) ;
#118274=DIRECTION('ref_axis',(8.6424177776148E-34,0.707106781186546,0.707106781186549)) ;
#118275=DIRECTION('',(0.577350269189625,0.577350269189625,0.577350269189627)) ;
#118276=DIRECTION('',(-1.,9.85638338623186E-18,0.)) ;
#118277=DIRECTION('',(0.577350269189625,-0.577350269189625,-0.577350269189627)) ;
#118278=DIRECTION('',(1.,-7.70371977754894E-34,9.8563833862319E-18)) ;
#118279=DIRECTION('center_axis',(6.96951553037899E-18,0.707106781186549,
0.707106781186546)) ;
#118280=DIRECTION('ref_axis',(-8.6424177776148E-34,-0.707106781186546,0.707106781186549)) ;
#118281=DIRECTION('',(-0.577350269189625,0.577350269189625,-0.577350269189627)) ;
#118282=DIRECTION('',(1.,-9.85638338623186E-18,0.)) ;
#118283=DIRECTION('',(-0.577350269189625,-0.577350269189625,0.577350269189627)) ;
#118284=DIRECTION('',(-1.,7.70371977754894E-34,9.8563833862319E-18)) ;
#118285=DIRECTION('center_axis',(6.96951553037899E-18,0.707106781186549,
-0.707106781186546)) ;
#118286=DIRECTION('ref_axis',(8.6424177776148E-34,0.707106781186546,0.707106781186549)) ;
#118287=DIRECTION('',(0.577350269189625,0.577350269189625,0.577350269189627)) ;
#118288=DIRECTION('',(-1.,9.85638338623186E-18,0.)) ;
#118289=DIRECTION('',(0.577350269189625,-0.577350269189625,-0.577350269189627)) ;
#118290=DIRECTION('',(1.,-7.70371977754894E-34,9.8563833862319E-18)) ;
#118291=DIRECTION('center_axis',(6.96951553037899E-18,0.707106781186549,
0.707106781186546)) ;
#118292=DIRECTION('ref_axis',(-8.6424177776148E-34,-0.707106781186546,0.707106781186549)) ;
#118293=DIRECTION('',(-0.577350269189625,0.577350269189625,-0.577350269189627)) ;
#118294=DIRECTION('',(1.,-9.85638338623186E-18,0.)) ;
#118295=DIRECTION('',(-0.577350269189625,-0.577350269189625,0.577350269189627)) ;
#118296=DIRECTION('',(-1.,7.70371977754894E-34,9.8563833862319E-18)) ;
#118297=DIRECTION('center_axis',(6.96951553037899E-18,0.707106781186549,
-0.707106781186546)) ;
#118298=DIRECTION('ref_axis',(8.6424177776148E-34,0.707106781186546,0.707106781186549)) ;
#118299=DIRECTION('',(0.577350269189625,0.577350269189625,0.577350269189627)) ;
#118300=DIRECTION('',(-1.,9.85638338623186E-18,0.)) ;
#118301=DIRECTION('',(0.577350269189625,-0.577350269189625,-0.577350269189627)) ;
#118302=DIRECTION('',(1.,-7.70371977754894E-34,9.8563833862319E-18)) ;
#118303=DIRECTION('center_axis',(6.96951553037899E-18,0.707106781186549,
0.707106781186546)) ;
#118304=DIRECTION('ref_axis',(-8.6424177776148E-34,-0.707106781186546,0.707106781186549)) ;
#118305=DIRECTION('',(-0.577350269189625,0.577350269189625,-0.577350269189627)) ;
#118306=DIRECTION('',(1.,-9.85638338623186E-18,0.)) ;
#118307=DIRECTION('',(-0.577350269189625,-0.577350269189625,0.577350269189627)) ;
#118308=DIRECTION('',(-1.,7.70371977754894E-34,9.8563833862319E-18)) ;
#118309=DIRECTION('center_axis',(6.96951553037899E-18,0.707106781186549,
-0.707106781186546)) ;
#118310=DIRECTION('ref_axis',(8.6424177776148E-34,0.707106781186546,0.707106781186549)) ;
#118311=DIRECTION('',(0.577350269189625,0.577350269189625,0.577350269189627)) ;
#118312=DIRECTION('',(-1.,9.85638338623186E-18,0.)) ;
#118313=DIRECTION('',(0.577350269189625,-0.577350269189625,-0.577350269189627)) ;
#118314=DIRECTION('',(1.,-7.70371977754894E-34,9.8563833862319E-18)) ;
#118315=DIRECTION('center_axis',(6.96951553037899E-18,0.707106781186549,
0.707106781186546)) ;
#118316=DIRECTION('ref_axis',(-8.6424177776148E-34,-0.707106781186546,0.707106781186549)) ;
#118317=DIRECTION('',(-0.577350269189625,0.577350269189625,-0.577350269189627)) ;
#118318=DIRECTION('',(1.,-9.85638338623186E-18,0.)) ;
#118319=DIRECTION('',(-0.577350269189625,-0.577350269189625,0.577350269189627)) ;
#118320=DIRECTION('',(-1.,7.70371977754894E-34,9.8563833862319E-18)) ;
#118321=DIRECTION('center_axis',(6.96951553037899E-18,0.707106781186549,
-0.707106781186546)) ;
#118322=DIRECTION('ref_axis',(8.6424177776148E-34,0.707106781186546,0.707106781186549)) ;
#118323=DIRECTION('',(0.577350269189625,0.577350269189625,0.577350269189627)) ;
#118324=DIRECTION('',(-1.,9.85638338623186E-18,0.)) ;
#118325=DIRECTION('',(0.577350269189625,-0.577350269189625,-0.577350269189627)) ;
#118326=DIRECTION('',(1.,-7.70371977754894E-34,9.8563833862319E-18)) ;
#118327=DIRECTION('center_axis',(6.96951553037899E-18,0.707106781186549,
0.707106781186546)) ;
#118328=DIRECTION('ref_axis',(-8.6424177776148E-34,-0.707106781186546,0.707106781186549)) ;
#118329=DIRECTION('',(-0.577350269189625,0.577350269189625,-0.577350269189627)) ;
#118330=DIRECTION('',(1.,-9.85638338623186E-18,0.)) ;
#118331=DIRECTION('',(-0.577350269189625,-0.577350269189625,0.577350269189627)) ;
#118332=DIRECTION('',(-1.,7.70371977754894E-34,9.8563833862319E-18)) ;
#118333=DIRECTION('center_axis',(6.96951553037899E-18,0.707106781186549,
-0.707106781186546)) ;
#118334=DIRECTION('ref_axis',(8.6424177776148E-34,0.707106781186546,0.707106781186549)) ;
#118335=DIRECTION('',(0.577350269189625,0.577350269189625,0.577350269189627)) ;
#118336=DIRECTION('',(-1.,9.85638338623186E-18,0.)) ;
#118337=DIRECTION('',(0.577350269189625,-0.577350269189625,-0.577350269189627)) ;
#118338=DIRECTION('',(1.,-7.70371977754894E-34,9.8563833862319E-18)) ;
#118339=DIRECTION('center_axis',(6.96951553037899E-18,0.707106781186549,
0.707106781186546)) ;
#118340=DIRECTION('ref_axis',(-8.6424177776148E-34,-0.707106781186546,0.707106781186549)) ;
#118341=DIRECTION('',(-0.577350269189625,0.577350269189625,-0.577350269189627)) ;
#118342=DIRECTION('',(1.,-9.85638338623186E-18,0.)) ;
#118343=DIRECTION('',(-0.577350269189625,-0.577350269189625,0.577350269189627)) ;
#118344=DIRECTION('',(-1.,7.70371977754894E-34,9.8563833862319E-18)) ;
#118345=DIRECTION('center_axis',(6.96951553037899E-18,0.707106781186549,
-0.707106781186546)) ;
#118346=DIRECTION('ref_axis',(8.6424177776148E-34,0.707106781186546,0.707106781186549)) ;
#118347=DIRECTION('',(0.577350269189625,0.577350269189625,0.577350269189627)) ;
#118348=DIRECTION('',(-1.,9.85638338623186E-18,0.)) ;
#118349=DIRECTION('',(0.577350269189625,-0.577350269189625,-0.577350269189627)) ;
#118350=DIRECTION('',(1.,-7.70371977754894E-34,9.8563833862319E-18)) ;
#118351=DIRECTION('center_axis',(-0.707106781186548,-1.38247767078009E-16,
0.707106781186547)) ;
#118352=DIRECTION('ref_axis',(0.707106781186547,8.815972061965E-34,0.707106781186548)) ;
#118353=DIRECTION('',(-0.577350269189625,-0.577350269189626,-0.577350269189626)) ;
#118354=DIRECTION('',(-1.95511867169517E-16,1.,0.)) ;
#118355=DIRECTION('',(0.577350269189625,-0.577350269189626,0.577350269189626)) ;
#118356=DIRECTION('',(0.,-1.,-1.95511867169518E-16)) ;
#118357=DIRECTION('center_axis',(-0.707106781186548,-1.38247767078009E-16,
-0.707106781186547)) ;
#118358=DIRECTION('ref_axis',(-0.707106781186547,-8.815972061965E-34,0.707106781186548)) ;
#118359=DIRECTION('',(-0.577350269189625,0.577350269189626,0.577350269189626)) ;
#118360=DIRECTION('',(1.95511867169517E-16,-1.,0.)) ;
#118361=DIRECTION('',(0.577350269189625,0.577350269189626,-0.577350269189626)) ;
#118362=DIRECTION('',(0.,1.,-1.95511867169518E-16)) ;
#118363=DIRECTION('center_axis',(-0.707106781186548,-1.38247767078009E-16,
0.707106781186547)) ;
#118364=DIRECTION('ref_axis',(0.707106781186547,8.815972061965E-34,0.707106781186548)) ;
#118365=DIRECTION('',(-0.577350269189625,-0.577350269189626,-0.577350269189626)) ;
#118366=DIRECTION('',(-1.95511867169517E-16,1.,0.)) ;
#118367=DIRECTION('',(0.577350269189625,-0.577350269189626,0.577350269189626)) ;
#118368=DIRECTION('',(0.,-1.,-1.95511867169518E-16)) ;
#118369=DIRECTION('center_axis',(-0.707106781186548,-1.38247767078009E-16,
-0.707106781186547)) ;
#118370=DIRECTION('ref_axis',(-0.707106781186547,-8.815972061965E-34,0.707106781186548)) ;
#118371=DIRECTION('',(-0.577350269189625,0.577350269189626,0.577350269189626)) ;
#118372=DIRECTION('',(1.95511867169517E-16,-1.,0.)) ;
#118373=DIRECTION('',(0.577350269189625,0.577350269189626,-0.577350269189626)) ;
#118374=DIRECTION('',(0.,1.,-1.95511867169518E-16)) ;
#118375=DIRECTION('center_axis',(-0.707106781186548,-1.38247767078009E-16,
0.707106781186547)) ;
#118376=DIRECTION('ref_axis',(0.707106781186547,8.815972061965E-34,0.707106781186548)) ;
#118377=DIRECTION('',(-0.577350269189625,-0.577350269189626,-0.577350269189626)) ;
#118378=DIRECTION('',(-1.95511867169517E-16,1.,0.)) ;
#118379=DIRECTION('',(0.577350269189625,-0.577350269189626,0.577350269189626)) ;
#118380=DIRECTION('',(0.,-1.,-1.95511867169518E-16)) ;
#118381=DIRECTION('center_axis',(-0.707106781186548,-1.38247767078009E-16,
-0.707106781186547)) ;
#118382=DIRECTION('ref_axis',(-0.707106781186547,-8.815972061965E-34,0.707106781186548)) ;
#118383=DIRECTION('',(-0.577350269189625,0.577350269189626,0.577350269189626)) ;
#118384=DIRECTION('',(1.95511867169517E-16,-1.,0.)) ;
#118385=DIRECTION('',(0.577350269189625,0.577350269189626,-0.577350269189626)) ;
#118386=DIRECTION('',(0.,1.,-1.95511867169518E-16)) ;
#118387=DIRECTION('center_axis',(-0.707106781186548,-1.38247767078009E-16,
0.707106781186547)) ;
#118388=DIRECTION('ref_axis',(0.707106781186547,8.815972061965E-34,0.707106781186548)) ;
#118389=DIRECTION('',(-0.577350269189625,-0.577350269189626,-0.577350269189626)) ;
#118390=DIRECTION('',(-1.95511867169517E-16,1.,0.)) ;
#118391=DIRECTION('',(0.577350269189625,-0.577350269189626,0.577350269189626)) ;
#118392=DIRECTION('',(0.,-1.,-1.95511867169518E-16)) ;
#118393=DIRECTION('center_axis',(-0.707106781186548,-1.38247767078009E-16,
-0.707106781186547)) ;
#118394=DIRECTION('ref_axis',(-0.707106781186547,-8.815972061965E-34,0.707106781186548)) ;
#118395=DIRECTION('',(-0.577350269189625,0.577350269189626,0.577350269189626)) ;
#118396=DIRECTION('',(1.95511867169517E-16,-1.,0.)) ;
#118397=DIRECTION('',(0.577350269189625,0.577350269189626,-0.577350269189626)) ;
#118398=DIRECTION('',(0.,1.,-1.95511867169518E-16)) ;
#118399=DIRECTION('center_axis',(-0.707106781186548,-1.38247767078009E-16,
0.707106781186547)) ;
#118400=DIRECTION('ref_axis',(0.707106781186547,8.815972061965E-34,0.707106781186548)) ;
#118401=DIRECTION('',(-0.577350269189625,-0.577350269189626,-0.577350269189626)) ;
#118402=DIRECTION('',(-1.95511867169517E-16,1.,0.)) ;
#118403=DIRECTION('',(0.577350269189625,-0.577350269189626,0.577350269189626)) ;
#118404=DIRECTION('',(0.,-1.,-1.95511867169518E-16)) ;
#118405=DIRECTION('center_axis',(-0.707106781186548,-1.38247767078009E-16,
-0.707106781186547)) ;
#118406=DIRECTION('ref_axis',(-0.707106781186547,-8.815972061965E-34,0.707106781186548)) ;
#118407=DIRECTION('',(-0.577350269189625,0.577350269189626,0.577350269189626)) ;
#118408=DIRECTION('',(1.95511867169517E-16,-1.,0.)) ;
#118409=DIRECTION('',(0.577350269189625,0.577350269189626,-0.577350269189626)) ;
#118410=DIRECTION('',(0.,1.,-1.95511867169518E-16)) ;
#118411=DIRECTION('center_axis',(-0.707106781186548,-1.38247767078009E-16,
0.707106781186547)) ;
#118412=DIRECTION('ref_axis',(0.707106781186547,8.815972061965E-34,0.707106781186548)) ;
#118413=DIRECTION('',(-0.577350269189625,-0.577350269189626,-0.577350269189626)) ;
#118414=DIRECTION('',(-1.95511867169517E-16,1.,0.)) ;
#118415=DIRECTION('',(0.577350269189625,-0.577350269189626,0.577350269189626)) ;
#118416=DIRECTION('',(0.,-1.,-1.95511867169518E-16)) ;
#118417=DIRECTION('center_axis',(-0.707106781186548,-1.38247767078009E-16,
-0.707106781186547)) ;
#118418=DIRECTION('ref_axis',(-0.707106781186547,-8.815972061965E-34,0.707106781186548)) ;
#118419=DIRECTION('',(-0.577350269189625,0.577350269189626,0.577350269189626)) ;
#118420=DIRECTION('',(1.95511867169517E-16,-1.,0.)) ;
#118421=DIRECTION('',(0.577350269189625,0.577350269189626,-0.577350269189626)) ;
#118422=DIRECTION('',(0.,1.,-1.95511867169518E-16)) ;
#118423=DIRECTION('center_axis',(-0.707106781186548,-1.38247767078009E-16,
0.707106781186547)) ;
#118424=DIRECTION('ref_axis',(0.707106781186547,8.815972061965E-34,0.707106781186548)) ;
#118425=DIRECTION('',(-0.577350269189625,-0.577350269189626,-0.577350269189626)) ;
#118426=DIRECTION('',(-1.95511867169517E-16,1.,0.)) ;
#118427=DIRECTION('',(0.577350269189625,-0.577350269189626,0.577350269189626)) ;
#118428=DIRECTION('',(0.,-1.,-1.95511867169518E-16)) ;
#118429=DIRECTION('center_axis',(-0.707106781186548,-1.38247767078009E-16,
-0.707106781186547)) ;
#118430=DIRECTION('ref_axis',(-0.707106781186547,-8.815972061965E-34,0.707106781186548)) ;
#118431=DIRECTION('',(-0.577350269189625,0.577350269189626,0.577350269189626)) ;
#118432=DIRECTION('',(1.95511867169517E-16,-1.,0.)) ;
#118433=DIRECTION('',(0.577350269189625,0.577350269189626,-0.577350269189626)) ;
#118434=DIRECTION('',(0.,1.,-1.95511867169518E-16)) ;
#118435=DIRECTION('center_axis',(-0.707106781186548,-1.38247767078009E-16,
0.707106781186547)) ;
#118436=DIRECTION('ref_axis',(0.707106781186547,8.815972061965E-34,0.707106781186548)) ;
#118437=DIRECTION('',(-0.577350269189625,-0.577350269189626,-0.577350269189626)) ;
#118438=DIRECTION('',(-1.95511867169517E-16,1.,0.)) ;
#118439=DIRECTION('',(0.577350269189625,-0.577350269189626,0.577350269189626)) ;
#118440=DIRECTION('',(0.,-1.,-1.95511867169518E-16)) ;
#118441=DIRECTION('center_axis',(-0.707106781186548,-1.38247767078009E-16,
-0.707106781186547)) ;
#118442=DIRECTION('ref_axis',(-0.707106781186547,-8.815972061965E-34,0.707106781186548)) ;
#118443=DIRECTION('',(-0.577350269189625,0.577350269189626,0.577350269189626)) ;
#118444=DIRECTION('',(1.95511867169517E-16,-1.,0.)) ;
#118445=DIRECTION('',(0.577350269189625,0.577350269189626,-0.577350269189626)) ;
#118446=DIRECTION('',(0.,1.,-1.95511867169518E-16)) ;
#118447=DIRECTION('center_axis',(-0.707106781186548,-1.38247767078009E-16,
0.707106781186547)) ;
#118448=DIRECTION('ref_axis',(0.707106781186547,8.815972061965E-34,0.707106781186548)) ;
#118449=DIRECTION('',(-0.577350269189625,-0.577350269189626,-0.577350269189626)) ;
#118450=DIRECTION('',(-1.95511867169517E-16,1.,0.)) ;
#118451=DIRECTION('',(0.577350269189625,-0.577350269189626,0.577350269189626)) ;
#118452=DIRECTION('',(0.,-1.,-1.95511867169518E-16)) ;
#118453=DIRECTION('center_axis',(-0.707106781186548,-1.38247767078009E-16,
-0.707106781186547)) ;
#118454=DIRECTION('ref_axis',(-0.707106781186547,-8.815972061965E-34,0.707106781186548)) ;
#118455=DIRECTION('',(-0.577350269189625,0.577350269189626,0.577350269189626)) ;
#118456=DIRECTION('',(1.95511867169517E-16,-1.,0.)) ;
#118457=DIRECTION('',(0.577350269189625,0.577350269189626,-0.577350269189626)) ;
#118458=DIRECTION('',(0.,1.,-1.95511867169518E-16)) ;
#118459=DIRECTION('center_axis',(0.577350269189625,0.577350269189625,-0.577350269189628)) ;
#118460=DIRECTION('ref_axis',(-0.70710678118655,2.50449302218608E-16,-0.707106781186546)) ;
#118461=DIRECTION('center_axis',(-0.577350269189625,-0.577350269189625,
0.577350269189628)) ;
#118462=DIRECTION('ref_axis',(-0.707106781186548,-2.12258087602815E-15,
-0.707106781186547)) ;
#118463=DIRECTION('center_axis',(-0.577350269189622,-0.577350269189626,
0.57735026918963)) ;
#118464=DIRECTION('ref_axis',(4.78608867599257E-17,-0.70710678118655,-0.707106781186545)) ;
#118465=DIRECTION('center_axis',(0.,0.,-1.)) ;
#118466=DIRECTION('ref_axis',(-1.,0.,0.)) ;
#118467=DIRECTION('center_axis',(0.,0.,1.)) ;
#118468=DIRECTION('ref_axis',(-1.,-8.67361737988404E-15,0.)) ;
#118469=DIRECTION('center_axis',(0.,0.,-1.)) ;
#118470=DIRECTION('ref_axis',(-1.,0.,0.)) ;
#118471=DIRECTION('center_axis',(2.08166817117218E-16,1.,0.)) ;
#118472=DIRECTION('ref_axis',(1.,0.,0.)) ;
#118473=DIRECTION('center_axis',(-1.,0.,-4.40821857296472E-15)) ;
#118474=DIRECTION('ref_axis',(4.40821857296472E-15,0.,-1.)) ;
#118475=DIRECTION('center_axis',(8.67361737988402E-15,8.67361737988401E-15,
1.)) ;
#118476=DIRECTION('ref_axis',(-1.,-9.79595207717063E-44,8.67361737988402E-15)) ;
#118477=DIRECTION('center_axis',(-0.577350269189625,-0.577350269189625,
-0.577350269189628)) ;
#118478=DIRECTION('ref_axis',(-0.70710678118655,2.50449302218608E-16,0.707106781186546)) ;
#118479=DIRECTION('center_axis',(-0.577350269189625,-0.577350269189625,
-0.577350269189628)) ;
#118480=DIRECTION('ref_axis',(-0.70710678118655,2.22693726602979E-16,0.707106781186546)) ;
#118481=DIRECTION('center_axis',(-0.577350269189624,-0.577350269189623,
-0.577350269189631)) ;
#118482=DIRECTION('ref_axis',(-0.707106781186552,5.79770761800025E-17,0.707106781186543)) ;
#118483=DIRECTION('center_axis',(0.,0.,-1.)) ;
#118484=DIRECTION('ref_axis',(-1.,0.,0.)) ;
#118485=DIRECTION('center_axis',(-6.1331736667335E-15,0.,1.)) ;
#118486=DIRECTION('ref_axis',(1.,0.,6.1331736667335E-15)) ;
#118487=DIRECTION('center_axis',(-1.,0.,9.8563833862319E-18)) ;
#118488=DIRECTION('ref_axis',(9.8563833862319E-18,0.,1.)) ;
#118489=DIRECTION('center_axis',(-1.,3.93023287525994E-15,-3.93023287525997E-15)) ;
#118490=DIRECTION('ref_axis',(-3.93023287525997E-15,2.80259692864963E-44,
1.)) ;
#118491=DIRECTION('center_axis',(2.08166817117218E-16,1.,0.)) ;
#118492=DIRECTION('ref_axis',(1.,0.,0.)) ;
#118493=DIRECTION('center_axis',(-1.,-8.13151629364126E-16,-8.13151629364131E-16)) ;
#118494=DIRECTION('ref_axis',(8.13151629364131E-16,1.13855500226391E-45,
-1.)) ;
#118495=DIRECTION('center_axis',(2.08166817117218E-16,1.,0.)) ;
#118496=DIRECTION('ref_axis',(1.,0.,0.)) ;
#118497=DIRECTION('center_axis',(-0.577350269189623,0.577350269189622,-0.577350269189633)) ;
#118498=DIRECTION('ref_axis',(0.707106781186554,7.82055407754491E-16,-0.707106781186541)) ;
#118499=DIRECTION('center_axis',(-6.1331736667335E-15,0.,1.)) ;
#118500=DIRECTION('ref_axis',(-1.,0.,-6.1331736667335E-15)) ;
#118501=DIRECTION('center_axis',(-1.,0.,-9.8563833862319E-18)) ;
#118502=DIRECTION('ref_axis',(-9.8563833862319E-18,0.,1.)) ;
#118503=DIRECTION('center_axis',(-1.,0.,-2.10827844793965E-15)) ;
#118504=DIRECTION('ref_axis',(-2.10827844793965E-15,0.,1.)) ;
#118505=DIRECTION('center_axis',(0.,0.,-1.)) ;
#118506=DIRECTION('ref_axis',(-1.,0.,0.)) ;
#118507=DIRECTION('center_axis',(0.,0.,1.)) ;
#118508=DIRECTION('ref_axis',(1.,0.,0.)) ;
#118509=DIRECTION('center_axis',(0.577350269189625,-0.577350269189625,0.577350269189628)) ;
#118510=DIRECTION('ref_axis',(0.707106781186549,-7.23605167296792E-16,-0.707106781186546)) ;
#118511=DIRECTION('center_axis',(0.577350269189625,-0.577350269189625,0.577350269189628)) ;
#118512=DIRECTION('ref_axis',(0.707106781186549,-7.51360742912421E-16,-0.707106781186546)) ;
#118513=DIRECTION('center_axis',(2.08166817117218E-16,1.,0.)) ;
#118514=DIRECTION('ref_axis',(1.,0.,0.)) ;
#118515=DIRECTION('center_axis',(-0.577350269189626,0.577350269189624,0.577350269189628)) ;
#118516=DIRECTION('ref_axis',(-0.707106781186549,-7.24154524606924E-16,
-0.707106781186546)) ;
#118517=DIRECTION('center_axis',(0.,0.,-1.)) ;
#118518=DIRECTION('ref_axis',(-1.,0.,0.)) ;
#118519=DIRECTION('center_axis',(0.,0.,1.)) ;
#118520=DIRECTION('ref_axis',(-1.,0.,0.)) ;
#118521=DIRECTION('center_axis',(0.,0.,-1.)) ;
#118522=DIRECTION('ref_axis',(-1.,0.,0.)) ;
#118523=DIRECTION('center_axis',(-0.577350269189625,0.577350269189625,0.577350269189628)) ;
#118524=DIRECTION('ref_axis',(0.70710678118655,2.22693726602979E-16,0.707106781186546)) ;
#118525=DIRECTION('center_axis',(0.577350269189625,-0.577350269189625,-0.577350269189628)) ;
#118526=DIRECTION('ref_axis',(0.707106781186549,-8.43215074740835E-16,0.707106781186546)) ;
#118527=DIRECTION('center_axis',(-0.577350269189625,0.577350269189626,-0.577350269189626)) ;
#118528=DIRECTION('ref_axis',(6.27941990732594E-17,0.707106781186548,0.707106781186548)) ;
#118529=DIRECTION('center_axis',(0.577350269189625,-0.577350269189626,0.577350269189626)) ;
#118530=DIRECTION('ref_axis',(5.0289788758123E-16,0.707106781186548,0.707106781186547)) ;
#118531=DIRECTION('center_axis',(0.577350269189624,-0.57735026918963,0.577350269189624)) ;
#118532=DIRECTION('ref_axis',(0.707106781186551,0.707106781186544,6.33763658455854E-16)) ;
#118533=DIRECTION('center_axis',(0.,0.,-1.)) ;
#118534=DIRECTION('ref_axis',(-1.,0.,0.)) ;
#118535=DIRECTION('center_axis',(0.,0.,1.)) ;
#118536=DIRECTION('ref_axis',(-1.,2.71050543121375E-15,0.)) ;
#118537=DIRECTION('center_axis',(0.,0.,-1.)) ;
#118538=DIRECTION('ref_axis',(-1.,0.,0.)) ;
#118539=DIRECTION('center_axis',(0.,1.,0.)) ;
#118540=DIRECTION('ref_axis',(1.,0.,0.)) ;
#118541=DIRECTION('center_axis',(0.,-1.,-3.25824851045217E-15)) ;
#118542=DIRECTION('ref_axis',(0.,-3.25824851045217E-15,1.)) ;
#118543=DIRECTION('center_axis',(4.33680868994201E-15,-4.33680868994202E-15,
1.)) ;
#118544=DIRECTION('ref_axis',(3.0828566215146E-44,1.,4.33680868994202E-15)) ;
#118545=DIRECTION('center_axis',(0.577350269189625,-0.577350269189626,-0.577350269189626)) ;
#118546=DIRECTION('ref_axis',(6.27941990732594E-17,0.707106781186548,-0.707106781186548)) ;
#118547=DIRECTION('center_axis',(0.577350269189625,-0.577350269189626,-0.577350269189626)) ;
#118548=DIRECTION('ref_axis',(-7.7646791370609E-16,0.707106781186547,-0.707106781186548)) ;
#118549=DIRECTION('center_axis',(0.577350269189625,-0.577350269189626,-0.577350269189627)) ;
#118550=DIRECTION('ref_axis',(-3.31150339748933E-16,0.707106781186548,-0.707106781186547)) ;
#118551=DIRECTION('center_axis',(0.,0.,-1.)) ;
#118552=DIRECTION('ref_axis',(-1.,0.,0.)) ;
#118553=DIRECTION('center_axis',(0.,-6.1331736667335E-15,1.)) ;
#118554=DIRECTION('ref_axis',(0.,-1.,-6.1331736667335E-15)) ;
#118555=DIRECTION('center_axis',(0.,1.,1.95511867169518E-16)) ;
#118556=DIRECTION('ref_axis',(0.,-1.95511867169518E-16,1.)) ;
#118557=DIRECTION('center_axis',(2.71050543121375E-16,-1.,7.93888660359539E-17)) ;
#118558=DIRECTION('ref_axis',(1.,2.71050543121375E-16,0.)) ;
#118559=DIRECTION('center_axis',(0.,1.,0.)) ;
#118560=DIRECTION('ref_axis',(1.,0.,0.)) ;
#118561=DIRECTION('center_axis',(-1.28749007982653E-15,-1.,1.47915175691195E-15)) ;
#118562=DIRECTION('ref_axis',(-1.49686561198851E-32,1.47915175691195E-15,
1.)) ;
#118563=DIRECTION('center_axis',(0.,1.,0.)) ;
#118564=DIRECTION('ref_axis',(1.,0.,0.)) ;
#118565=DIRECTION('center_axis',(-0.577350269189624,-0.577350269189626,
-0.577350269189628)) ;
#118566=DIRECTION('ref_axis',(-1.24495925064522E-15,-0.707106781186548,
0.707106781186547)) ;
#118567=DIRECTION('center_axis',(0.,-6.1331736667335E-15,1.)) ;
#118568=DIRECTION('ref_axis',(0.,1.,6.1331736667335E-15)) ;
#118569=DIRECTION('center_axis',(0.,1.,-1.95511867169518E-16)) ;
#118570=DIRECTION('ref_axis',(0.,1.95511867169518E-16,1.)) ;
#118571=DIRECTION('center_axis',(0.,-1.,-4.59988025005012E-15)) ;
#118572=DIRECTION('ref_axis',(0.,4.59988025005012E-15,-1.)) ;
#118573=DIRECTION('center_axis',(0.,0.,-1.)) ;
#118574=DIRECTION('ref_axis',(-1.,0.,0.)) ;
#118575=DIRECTION('center_axis',(0.,0.,1.)) ;
#118576=DIRECTION('ref_axis',(1.,0.,0.)) ;
#118577=DIRECTION('center_axis',(0.577350269189625,0.577350269189626,0.577350269189627)) ;
#118578=DIRECTION('ref_axis',(-2.71345386026911E-16,-0.707106781186548,
0.707106781186547)) ;
#118579=DIRECTION('center_axis',(0.577350269189625,0.577350269189626,0.577350269189627)) ;
#118580=DIRECTION('ref_axis',(-2.71345386026911E-16,-0.707106781186548,
0.707106781186547)) ;
#118581=DIRECTION('center_axis',(0.,1.,0.)) ;
#118582=DIRECTION('ref_axis',(1.,0.,0.)) ;
#118583=DIRECTION('center_axis',(-0.577350269189624,-0.577350269189628,
0.577350269189625)) ;
#118584=DIRECTION('ref_axis',(-6.89490688817364E-15,0.707106781186549,0.707106781186546)) ;
#118585=DIRECTION('center_axis',(0.,0.,-1.)) ;
#118586=DIRECTION('ref_axis',(-1.,0.,0.)) ;
#118587=DIRECTION('center_axis',(0.,0.,1.)) ;
#118588=DIRECTION('ref_axis',(-1.,1.0842021724855E-15,0.)) ;
#118589=DIRECTION('center_axis',(0.,0.,-1.)) ;
#118590=DIRECTION('ref_axis',(-1.,0.,0.)) ;
#118591=DIRECTION('center_axis',(-0.577350269189625,-0.577350269189626,
0.577350269189627)) ;
#118592=DIRECTION('ref_axis',(-2.71345386026911E-16,-0.707106781186548,
-0.707106781186547)) ;
#118593=DIRECTION('center_axis',(0.577350269189625,0.577350269189626,-0.577350269189627)) ;
#118594=DIRECTION('ref_axis',(-9.76085677604559E-15,-0.707106781186543,
-0.707106781186552)) ;
#118595=DIRECTION('center_axis',(0.577350269189625,0.577350269189625,-0.577350269189628)) ;
#118596=DIRECTION('ref_axis',(-0.707106781186549,-7.23605167296792E-16,
-0.707106781186546)) ;
#118597=DIRECTION('center_axis',(-0.577350269189625,-0.577350269189625,
0.577350269189628)) ;
#118598=DIRECTION('ref_axis',(-0.707106781186542,-1.47047746496289E-14,
-0.707106781186553)) ;
#118599=DIRECTION('center_axis',(-0.577350269189629,-0.577350269189624,
0.577350269189624)) ;
#118600=DIRECTION('ref_axis',(0.707106781186545,-9.59471324968973E-16,0.70710678118655)) ;
#118601=DIRECTION('center_axis',(0.,0.,-1.)) ;
#118602=DIRECTION('ref_axis',(-1.,0.,0.)) ;
#118603=DIRECTION('center_axis',(0.,0.,1.)) ;
#118604=DIRECTION('ref_axis',(-1.,0.,0.)) ;
#118605=DIRECTION('center_axis',(0.,0.,-1.)) ;
#118606=DIRECTION('ref_axis',(-1.,0.,0.)) ;
#118607=DIRECTION('center_axis',(2.08166817117218E-16,1.,0.)) ;
#118608=DIRECTION('ref_axis',(1.,0.,0.)) ;
#118609=DIRECTION('center_axis',(-1.,0.,-5.94151198964807E-15)) ;
#118610=DIRECTION('ref_axis',(5.94151198964807E-15,0.,-1.)) ;
#118611=DIRECTION('center_axis',(0.,0.,1.)) ;
#118612=DIRECTION('ref_axis',(-1.,0.,0.)) ;
#118613=DIRECTION('center_axis',(-0.577350269189625,-0.577350269189625,
-0.577350269189628)) ;
#118614=DIRECTION('ref_axis',(-0.707106781186549,-7.23605167296792E-16,
0.707106781186546)) ;
#118615=DIRECTION('center_axis',(-0.577350269189625,-0.577350269189625,
-0.577350269189628)) ;
#118616=DIRECTION('ref_axis',(-0.707106781186549,-7.51360742912421E-16,
0.707106781186546)) ;
#118617=DIRECTION('center_axis',(-0.577350269189629,-0.577350269189628,
-0.577350269189621)) ;
#118618=DIRECTION('ref_axis',(0.707106781186547,-0.707106781186548,-9.25270248417546E-17)) ;
#118619=DIRECTION('center_axis',(0.,0.,-1.)) ;
#118620=DIRECTION('ref_axis',(-1.,0.,0.)) ;
#118621=DIRECTION('center_axis',(1.2266347333467E-14,0.,1.)) ;
#118622=DIRECTION('ref_axis',(1.,0.,-1.2266347333467E-14)) ;
#118623=DIRECTION('center_axis',(-1.,0.,9.8563833862319E-18)) ;
#118624=DIRECTION('ref_axis',(9.8563833862319E-18,0.,1.)) ;
#118625=DIRECTION('center_axis',(-1.,1.62630325872825E-15,-1.62630325872825E-15)) ;
#118626=DIRECTION('ref_axis',(-1.62630325872825E-15,0.,1.)) ;
#118627=DIRECTION('center_axis',(2.08166817117218E-16,1.,0.)) ;
#118628=DIRECTION('ref_axis',(1.,0.,0.)) ;
#118629=DIRECTION('center_axis',(-1.,1.35525271560688E-16,1.35525271560688E-16)) ;
#118630=DIRECTION('ref_axis',(-1.35525271560688E-16,0.,-1.)) ;
#118631=DIRECTION('center_axis',(2.08166817117218E-16,1.,0.)) ;
#118632=DIRECTION('ref_axis',(1.,0.,0.)) ;
#118633=DIRECTION('center_axis',(-0.577350269189628,0.577350269189628,-0.577350269189621)) ;
#118634=DIRECTION('ref_axis',(0.707106781186547,0.707106781186548,5.83290435273539E-16)) ;
#118635=DIRECTION('center_axis',(1.2266347333467E-14,0.,1.)) ;
#118636=DIRECTION('ref_axis',(-1.,0.,1.2266347333467E-14)) ;
#118637=DIRECTION('center_axis',(-1.,0.,-9.8563833862319E-18)) ;
#118638=DIRECTION('ref_axis',(-9.8563833862319E-18,0.,1.)) ;
#118639=DIRECTION('center_axis',(-1.,0.,9.58308385427108E-16)) ;
#118640=DIRECTION('ref_axis',(9.58308385427108E-16,0.,1.)) ;
#118641=DIRECTION('center_axis',(0.,0.,-1.)) ;
#118642=DIRECTION('ref_axis',(-1.,0.,0.)) ;
#118643=DIRECTION('center_axis',(-8.67361737988402E-15,8.67361737988401E-15,
1.)) ;
#118644=DIRECTION('ref_axis',(1.,-9.79595207717063E-44,8.67361737988402E-15)) ;
#118645=DIRECTION('center_axis',(0.577350269189625,-0.577350269189625,0.577350269189628)) ;
#118646=DIRECTION('ref_axis',(0.707106781186549,-7.23605167296792E-16,-0.707106781186546)) ;
#118647=DIRECTION('center_axis',(0.577350269189625,-0.577350269189625,0.577350269189628)) ;
#118648=DIRECTION('ref_axis',(0.707106781186549,-7.51360742912421E-16,-0.707106781186546)) ;
#118649=DIRECTION('center_axis',(2.08166817117218E-16,1.,0.)) ;
#118650=DIRECTION('ref_axis',(1.,0.,0.)) ;
#118651=DIRECTION('center_axis',(-0.577350269189631,0.577350269189623,0.577350269189623)) ;
#118652=DIRECTION('ref_axis',(-0.707106781186542,1.43689139429453E-15,-0.707106781186553)) ;
#118653=DIRECTION('center_axis',(0.,0.,-1.)) ;
#118654=DIRECTION('ref_axis',(-1.,0.,0.)) ;
#118655=DIRECTION('center_axis',(0.,0.,1.)) ;
#118656=DIRECTION('ref_axis',(-1.,0.,0.)) ;
#118657=DIRECTION('center_axis',(0.,0.,-1.)) ;
#118658=DIRECTION('ref_axis',(-1.,0.,0.)) ;
#118659=DIRECTION('center_axis',(-0.577350269189625,0.577350269189625,0.577350269189628)) ;
#118660=DIRECTION('ref_axis',(0.707106781186549,-7.51360742912421E-16,0.707106781186546)) ;
#118661=DIRECTION('center_axis',(0.577350269189625,-0.577350269189625,-0.577350269189628)) ;
#118662=DIRECTION('ref_axis',(0.707106781186549,-8.43215074740835E-16,0.707106781186546)) ;
#118663=DIRECTION('center_axis',(-0.577350269189625,0.577350269189626,-0.577350269189626)) ;
#118664=DIRECTION('ref_axis',(6.27941990732594E-17,0.707106781186548,0.707106781186548)) ;
#118665=DIRECTION('center_axis',(0.577350269189625,-0.577350269189626,0.577350269189626)) ;
#118666=DIRECTION('ref_axis',(-4.12932450763554E-14,0.707106781186527,0.707106781186568)) ;
#118667=DIRECTION('center_axis',(0.577350269189626,-0.577350269189626,0.577350269189626)) ;
#118668=DIRECTION('ref_axis',(0.707106781186548,0.707106781186547,-6.70219100485003E-16)) ;
#118669=DIRECTION('center_axis',(0.,0.,-1.)) ;
#118670=DIRECTION('ref_axis',(-1.,0.,0.)) ;
#118671=DIRECTION('center_axis',(0.,0.,1.)) ;
#118672=DIRECTION('ref_axis',(-1.,0.,0.)) ;
#118673=DIRECTION('center_axis',(0.,0.,-1.)) ;
#118674=DIRECTION('ref_axis',(-1.,0.,0.)) ;
#118675=DIRECTION('center_axis',(0.,1.,0.)) ;
#118676=DIRECTION('ref_axis',(1.,0.,0.)) ;
#118677=DIRECTION('center_axis',(0.,-1.,-1.05413922396982E-14)) ;
#118678=DIRECTION('ref_axis',(0.,-1.05413922396982E-14,1.)) ;
#118679=DIRECTION('center_axis',(-8.67361737988401E-15,8.67361737988403E-15,
1.)) ;
#118680=DIRECTION('ref_axis',(-4.48415508583941E-44,1.,-8.67361737988403E-15)) ;
#118681=DIRECTION('center_axis',(0.577350269189625,-0.577350269189626,-0.577350269189626)) ;
#118682=DIRECTION('ref_axis',(6.27941990732594E-17,0.707106781186548,-0.707106781186548)) ;
#118683=DIRECTION('center_axis',(0.577350269189625,-0.577350269189626,-0.577350269189626)) ;
#118684=DIRECTION('ref_axis',(-7.7646791370609E-16,0.707106781186547,-0.707106781186548)) ;
#118685=DIRECTION('center_axis',(0.577350269189627,-0.577350269189628,-0.577350269189622)) ;
#118686=DIRECTION('ref_axis',(0.707106781186548,0.707106781186547,-7.93962717014541E-17)) ;
#118687=DIRECTION('center_axis',(0.,0.,-1.)) ;
#118688=DIRECTION('ref_axis',(-1.,0.,0.)) ;
#118689=DIRECTION('center_axis',(0.,1.2266347333467E-14,1.)) ;
#118690=DIRECTION('ref_axis',(0.,-1.,1.2266347333467E-14)) ;
#118691=DIRECTION('center_axis',(0.,1.,1.95511867169518E-16)) ;
#118692=DIRECTION('ref_axis',(0.,-1.95511867169518E-16,1.)) ;
#118693=DIRECTION('center_axis',(-1.42301535138722E-15,-1.,-1.61467702847264E-15)) ;
#118694=DIRECTION('ref_axis',(-1.65443041324959E-32,1.61467702847264E-15,
-1.)) ;
#118695=DIRECTION('center_axis',(0.,1.,0.)) ;
#118696=DIRECTION('ref_axis',(1.,0.,0.)) ;
#118697=DIRECTION('center_axis',(3.72694496791891E-15,-1.,-3.53528329083349E-15)) ;
#118698=DIRECTION('ref_axis',(-1.,-3.72694496791891E-15,0.)) ;
#118699=DIRECTION('center_axis',(0.,1.,0.)) ;
#118700=DIRECTION('ref_axis',(1.,0.,0.)) ;
#118701=DIRECTION('center_axis',(-0.577350269189623,-0.577350269189624,
-0.577350269189631)) ;
#118702=DIRECTION('ref_axis',(1.89964573407132E-15,-0.707106781186553,0.707106781186542)) ;
#118703=DIRECTION('center_axis',(0.,-1.2266347333467E-14,1.)) ;
#118704=DIRECTION('ref_axis',(0.,1.,1.2266347333467E-14)) ;
#118705=DIRECTION('center_axis',(0.,1.,-1.95511867169518E-16)) ;
#118706=DIRECTION('ref_axis',(0.,1.95511867169518E-16,1.)) ;
#118707=DIRECTION('center_axis',(0.,-1.,-7.66646708341686E-16)) ;
#118708=DIRECTION('ref_axis',(0.,7.66646708341686E-16,-1.)) ;
#118709=DIRECTION('center_axis',(0.,0.,-1.)) ;
#118710=DIRECTION('ref_axis',(-1.,0.,0.)) ;
#118711=DIRECTION('center_axis',(0.,0.,1.)) ;
#118712=DIRECTION('ref_axis',(1.,0.,0.)) ;
#118713=DIRECTION('center_axis',(0.577350269189625,0.577350269189626,0.577350269189627)) ;
#118714=DIRECTION('ref_axis',(-2.71345386026911E-16,-0.707106781186548,
0.707106781186547)) ;
#118715=DIRECTION('center_axis',(0.577350269189625,0.577350269189626,0.577350269189627)) ;
#118716=DIRECTION('ref_axis',(-2.71345386026911E-16,-0.707106781186548,
0.707106781186547)) ;
#118717=DIRECTION('center_axis',(0.,1.,0.)) ;
#118718=DIRECTION('ref_axis',(1.,0.,0.)) ;
#118719=DIRECTION('center_axis',(-0.577350269189625,-0.577350269189627,
0.577350269189625)) ;
#118720=DIRECTION('ref_axis',(4.24759239037863E-16,0.707106781186546,0.707106781186549)) ;
#118721=DIRECTION('center_axis',(0.,0.,-1.)) ;
#118722=DIRECTION('ref_axis',(-1.,0.,0.)) ;
#118723=DIRECTION('center_axis',(0.,0.,1.)) ;
#118724=DIRECTION('ref_axis',(-1.,1.0842021724855E-15,0.)) ;
#118725=DIRECTION('center_axis',(0.,0.,-1.)) ;
#118726=DIRECTION('ref_axis',(-1.,0.,0.)) ;
#118727=DIRECTION('center_axis',(-0.577350269189625,-0.577350269189626,
0.577350269189627)) ;
#118728=DIRECTION('ref_axis',(-2.71345386026911E-16,-0.707106781186548,
-0.707106781186547)) ;
#118729=DIRECTION('center_axis',(0.577350269189625,0.577350269189626,-0.577350269189627)) ;
#118730=DIRECTION('ref_axis',(-8.1269550549169E-15,-0.707106781186544,-0.707106781186551)) ;
#118731=DIRECTION('center_axis',(0.577350269189625,0.577350269189625,-0.577350269189628)) ;
#118732=DIRECTION('ref_axis',(-0.707106781186549,-7.23605167296792E-16,
-0.707106781186546)) ;
#118733=DIRECTION('center_axis',(-0.577350269189625,-0.577350269189625,
0.577350269189628)) ;
#118734=DIRECTION('ref_axis',(-0.707106781186545,-8.33999502129868E-15,
-0.70710678118655)) ;
#118735=DIRECTION('center_axis',(-0.577350269189627,-0.577350269189625,
0.577350269189625)) ;
#118736=DIRECTION('ref_axis',(0.707106781186546,1.26631399429469E-16,0.707106781186549)) ;
#118737=DIRECTION('center_axis',(0.,0.,-1.)) ;
#118738=DIRECTION('ref_axis',(-1.,0.,0.)) ;
#118739=DIRECTION('center_axis',(0.,0.,1.)) ;
#118740=DIRECTION('ref_axis',(-1.,0.,0.)) ;
#118741=DIRECTION('center_axis',(0.,0.,-1.)) ;
#118742=DIRECTION('ref_axis',(-1.,0.,0.)) ;
#118743=DIRECTION('center_axis',(2.08166817117218E-16,1.,0.)) ;
#118744=DIRECTION('ref_axis',(1.,0.,0.)) ;
#118745=DIRECTION('center_axis',(-1.,0.,9.58308385427108E-16)) ;
#118746=DIRECTION('ref_axis',(-9.58308385427108E-16,0.,-1.)) ;
#118747=DIRECTION('center_axis',(0.,0.,1.)) ;
#118748=DIRECTION('ref_axis',(-1.,0.,0.)) ;
#118749=DIRECTION('center_axis',(-0.577350269189625,-0.577350269189625,
-0.577350269189628)) ;
#118750=DIRECTION('ref_axis',(-0.707106781186549,-7.23605167296792E-16,
0.707106781186546)) ;
#118751=DIRECTION('center_axis',(-0.577350269189625,-0.577350269189625,
-0.577350269189628)) ;
#118752=DIRECTION('ref_axis',(-0.707106781186549,-7.51360742912421E-16,
0.707106781186546)) ;
#118753=DIRECTION('center_axis',(-0.577350269189633,-0.577350269189632,
-0.577350269189612)) ;
#118754=DIRECTION('ref_axis',(0.707106781186547,-0.707106781186548,-7.39398349810839E-17)) ;
#118755=DIRECTION('center_axis',(0.,0.,-1.)) ;
#118756=DIRECTION('ref_axis',(-1.,0.,0.)) ;
#118757=DIRECTION('center_axis',(2.4532694666934E-14,0.,1.)) ;
#118758=DIRECTION('ref_axis',(1.,0.,-2.4532694666934E-14)) ;
#118759=DIRECTION('center_axis',(-1.,0.,9.8563833862319E-18)) ;
#118760=DIRECTION('ref_axis',(9.8563833862319E-18,0.,1.)) ;
#118761=DIRECTION('center_axis',(-1.,-8.40256683676264E-15,8.40256683676264E-15)) ;
#118762=DIRECTION('ref_axis',(8.40256683676264E-15,-6.05360936588321E-43,
1.)) ;
#118763=DIRECTION('center_axis',(2.08166817117218E-16,1.,0.)) ;
#118764=DIRECTION('ref_axis',(1.,0.,0.)) ;
#118765=DIRECTION('center_axis',(-1.,4.9466724119651E-15,4.9466724119651E-15)) ;
#118766=DIRECTION('ref_axis',(-4.9466724119651E-15,-2.12997366577372E-43,
-1.)) ;
#118767=DIRECTION('center_axis',(2.08166817117218E-16,1.,0.)) ;
#118768=DIRECTION('ref_axis',(1.,0.,0.)) ;
#118769=DIRECTION('center_axis',(-0.577350269189629,0.577350269189628,-0.577350269189621)) ;
#118770=DIRECTION('ref_axis',(0.707106781186547,0.707106781186548,-3.27220711197328E-17)) ;
#118771=DIRECTION('center_axis',(0.,0.,1.)) ;
#118772=DIRECTION('ref_axis',(-1.,0.,0.)) ;
#118773=DIRECTION('center_axis',(-1.,0.,-9.8563833862319E-18)) ;
#118774=DIRECTION('ref_axis',(-9.8563833862319E-18,0.,1.)) ;
#118775=DIRECTION('center_axis',(-1.,0.,-1.05413922396982E-14)) ;
#118776=DIRECTION('ref_axis',(-1.05413922396982E-14,0.,1.)) ;
#118777=DIRECTION('center_axis',(0.,0.,-1.)) ;
#118778=DIRECTION('ref_axis',(-1.,0.,0.)) ;
#118779=DIRECTION('center_axis',(0.,0.,1.)) ;
#118780=DIRECTION('ref_axis',(1.,0.,0.)) ;
#118781=DIRECTION('center_axis',(0.577350269189625,-0.577350269189625,0.577350269189628)) ;
#118782=DIRECTION('ref_axis',(0.707106781186549,-7.23605167296792E-16,-0.707106781186546)) ;
#118783=DIRECTION('center_axis',(0.577350269189625,-0.577350269189625,0.577350269189628)) ;
#118784=DIRECTION('ref_axis',(0.707106781186549,-7.51360742912421E-16,-0.707106781186546)) ;
#118785=DIRECTION('center_axis',(2.08166817117218E-16,1.,0.)) ;
#118786=DIRECTION('ref_axis',(1.,0.,0.)) ;
#118787=DIRECTION('center_axis',(-0.577350269189631,0.577350269189623,0.577350269189623)) ;
#118788=DIRECTION('ref_axis',(-0.707106781186544,-2.28159610212341E-15,
-0.707106781186551)) ;
#118789=DIRECTION('center_axis',(0.,0.,-1.)) ;
#118790=DIRECTION('ref_axis',(-1.,0.,0.)) ;
#118791=DIRECTION('center_axis',(0.,0.,1.)) ;
#118792=DIRECTION('ref_axis',(-1.,0.,0.)) ;
#118793=DIRECTION('center_axis',(0.,0.,-1.)) ;
#118794=DIRECTION('ref_axis',(-1.,0.,0.)) ;
#118795=DIRECTION('center_axis',(-0.577350269189625,0.577350269189625,0.577350269189628)) ;
#118796=DIRECTION('ref_axis',(0.707106781186549,-7.51360742912421E-16,0.707106781186546)) ;
#118797=DIRECTION('center_axis',(0.577350269189625,-0.577350269189625,-0.577350269189628)) ;
#118798=DIRECTION('ref_axis',(0.707106781186548,-2.12258087602815E-15,0.707106781186547)) ;
#118799=DIRECTION('center_axis',(-0.577350269189625,0.577350269189626,-0.577350269189626)) ;
#118800=DIRECTION('ref_axis',(6.27941990732594E-17,0.707106781186548,0.707106781186548)) ;
#118801=DIRECTION('center_axis',(0.577350269189625,-0.577350269189626,0.577350269189626)) ;
#118802=DIRECTION('ref_axis',(-2.74316855014674E-14,0.707106781186534,0.707106781186561)) ;
#118803=DIRECTION('center_axis',(0.577350269189617,-0.577350269189643,0.577350269189617)) ;
#118804=DIRECTION('ref_axis',(0.707106781186564,0.707106781186531,-7.69284786604672E-16)) ;
#118805=DIRECTION('center_axis',(0.,0.,-1.)) ;
#118806=DIRECTION('ref_axis',(-1.,0.,0.)) ;
#118807=DIRECTION('center_axis',(0.,0.,1.)) ;
#118808=DIRECTION('ref_axis',(-1.,0.,0.)) ;
#118809=DIRECTION('center_axis',(0.,0.,-1.)) ;
#118810=DIRECTION('ref_axis',(-1.,0.,0.)) ;
#118811=DIRECTION('center_axis',(0.,1.,0.)) ;
#118812=DIRECTION('ref_axis',(1.,0.,0.)) ;
#118813=DIRECTION('center_axis',(0.,-1.,-1.39913024272358E-14)) ;
#118814=DIRECTION('ref_axis',(0.,-1.39913024272358E-14,1.)) ;
#118815=DIRECTION('center_axis',(1.7347234759768E-14,-1.73472347597681E-14,
1.)) ;
#118816=DIRECTION('ref_axis',(-1.79366203433577E-43,1.,1.73472347597681E-14)) ;
#118817=DIRECTION('center_axis',(0.577350269189625,-0.577350269189626,-0.577350269189626)) ;
#118818=DIRECTION('ref_axis',(6.27941990732594E-17,0.707106781186548,-0.707106781186548)) ;
#118819=DIRECTION('center_axis',(0.577350269189625,-0.577350269189626,-0.577350269189626)) ;
#118820=DIRECTION('ref_axis',(-7.7646791370609E-16,0.707106781186547,-0.707106781186548)) ;
#118821=DIRECTION('center_axis',(0.577350269189636,-0.577350269189637,-0.577350269189605)) ;
#118822=DIRECTION('ref_axis',(0.707106781186548,0.707106781186547,-1.89650892222054E-16)) ;
#118823=DIRECTION('center_axis',(0.,0.,-1.)) ;
#118824=DIRECTION('ref_axis',(-1.,0.,0.)) ;
#118825=DIRECTION('center_axis',(0.,2.4532694666934E-14,1.)) ;
#118826=DIRECTION('ref_axis',(0.,-1.,2.4532694666934E-14)) ;
#118827=DIRECTION('center_axis',(0.,1.,1.95511867169518E-16)) ;
#118828=DIRECTION('ref_axis',(0.,-1.95511867169518E-16,1.)) ;
#118829=DIRECTION('center_axis',(1.21972744404619E-15,-1.,1.02806576696077E-15)) ;
#118830=DIRECTION('ref_axis',(1.,1.21972744404619E-15,0.)) ;
#118831=DIRECTION('center_axis',(0.,1.,0.)) ;
#118832=DIRECTION('ref_axis',(1.,0.,0.)) ;
#118833=DIRECTION('center_axis',(-1.41623908780917E-14,-1.,1.43540525551772E-14)) ;
#118834=DIRECTION('ref_axis',(-1.64655217322172E-31,1.43540525551772E-14,
1.)) ;
#118835=DIRECTION('center_axis',(0.,1.,0.)) ;
#118836=DIRECTION('ref_axis',(1.,0.,0.)) ;
#118837=DIRECTION('center_axis',(-0.577350269189625,-0.577350269189626,
-0.577350269189626)) ;
#118838=DIRECTION('ref_axis',(4.43092933859209E-16,-0.707106781186548,0.707106781186547)) ;
#118839=DIRECTION('center_axis',(0.,0.,1.)) ;
#118840=DIRECTION('ref_axis',(-1.,8.87690528722505E-15,0.)) ;
#118841=DIRECTION('center_axis',(0.,1.,-1.95511867169518E-16)) ;
#118842=DIRECTION('ref_axis',(0.,1.95511867169518E-16,1.)) ;
#118843=DIRECTION('center_axis',(0.,-1.,-2.17536003491953E-14)) ;
#118844=DIRECTION('ref_axis',(0.,2.17536003491953E-14,-1.)) ;
#118845=DIRECTION('center_axis',(0.,0.,-1.)) ;
#118846=DIRECTION('ref_axis',(-1.,0.,0.)) ;
#118847=DIRECTION('center_axis',(-1.7347234759768E-14,-1.73472347597681E-14,
1.)) ;
#118848=DIRECTION('ref_axis',(-8.96831017167883E-44,-1.,-1.73472347597681E-14)) ;
#118849=DIRECTION('center_axis',(0.577350269189625,0.577350269189626,0.577350269189627)) ;
#118850=DIRECTION('ref_axis',(-2.71345386026911E-16,-0.707106781186548,
0.707106781186547)) ;
#118851=DIRECTION('center_axis',(0.577350269189625,0.577350269189626,0.577350269189627)) ;
#118852=DIRECTION('ref_axis',(-2.71345386026911E-16,-0.707106781186548,
0.707106781186547)) ;
#118853=DIRECTION('center_axis',(0.,1.,0.)) ;
#118854=DIRECTION('ref_axis',(1.,0.,0.)) ;
#118855=DIRECTION('center_axis',(-0.577350269189615,-0.577350269189648,
0.577350269189615)) ;
#118856=DIRECTION('ref_axis',(-7.65039491896549E-15,0.707106781186531,0.707106781186564)) ;
#118857=DIRECTION('center_axis',(0.,0.,-1.)) ;
#118858=DIRECTION('ref_axis',(-1.,0.,0.)) ;
#118859=DIRECTION('center_axis',(0.,0.,1.)) ;
#118860=DIRECTION('ref_axis',(-1.,1.0842021724855E-15,0.)) ;
#118861=DIRECTION('center_axis',(0.,0.,-1.)) ;
#118862=DIRECTION('ref_axis',(-1.,0.,0.)) ;
#118863=DIRECTION('center_axis',(-0.577350269189625,-0.577350269189626,
0.577350269189627)) ;
#118864=DIRECTION('ref_axis',(-2.71345386026911E-16,-0.707106781186548,
-0.707106781186547)) ;
#118865=DIRECTION('center_axis',(0.577350269189625,0.577350269189626,-0.577350269189627)) ;
#118866=DIRECTION('ref_axis',(1.27552458785726E-14,-0.707106781186554,-0.707106781186541)) ;
#118867=DIRECTION('center_axis',(0.577350269189625,0.577350269189625,-0.577350269189628)) ;
#118868=DIRECTION('ref_axis',(-0.707106781186549,-7.23605167296792E-16,
-0.707106781186546)) ;
#118869=DIRECTION('center_axis',(-0.577350269189625,-0.577350269189625,
0.577350269189628)) ;
#118870=DIRECTION('ref_axis',(-0.707106781186545,-8.28019006757666E-15,
-0.70710678118655)) ;
#118871=DIRECTION('center_axis',(-0.577350269189628,-0.577350269189625,
0.577350269189625)) ;
#118872=DIRECTION('ref_axis',(0.707106781186546,1.58001979428239E-16,0.707106781186549)) ;
#118873=DIRECTION('center_axis',(0.,0.,-1.)) ;
#118874=DIRECTION('ref_axis',(-1.,0.,0.)) ;
#118875=DIRECTION('center_axis',(0.,0.,1.)) ;
#118876=DIRECTION('ref_axis',(-1.,-8.67361737988404E-15,0.)) ;
#118877=DIRECTION('center_axis',(0.,0.,-1.)) ;
#118878=DIRECTION('ref_axis',(-1.,0.,0.)) ;
#118879=DIRECTION('center_axis',(2.08166817117218E-16,1.,0.)) ;
#118880=DIRECTION('ref_axis',(1.,0.,0.)) ;
#118881=DIRECTION('center_axis',(-1.,0.,-4.40821857296469E-15)) ;
#118882=DIRECTION('ref_axis',(4.40821857296469E-15,0.,-1.)) ;
#118883=DIRECTION('center_axis',(0.,0.,1.)) ;
#118884=DIRECTION('ref_axis',(-1.,0.,0.)) ;
#118885=DIRECTION('center_axis',(-0.577350269189625,-0.577350269189625,
-0.577350269189628)) ;
#118886=DIRECTION('ref_axis',(-0.707106781186549,-7.23605167296792E-16,
0.707106781186546)) ;
#118887=DIRECTION('center_axis',(-0.577350269189625,-0.577350269189625,
-0.577350269189628)) ;
#118888=DIRECTION('ref_axis',(-0.707106781186549,-7.51360742912421E-16,
0.707106781186546)) ;
#118889=DIRECTION('center_axis',(-0.577350269189624,-0.577350269189624,
-0.57735026918963)) ;
#118890=DIRECTION('ref_axis',(-0.70710678118655,-1.90469774984546E-15,0.707106781186545)) ;
#118891=DIRECTION('center_axis',(0.,0.,-1.)) ;
#118892=DIRECTION('ref_axis',(-1.,0.,0.)) ;
#118893=DIRECTION('center_axis',(0.,0.,1.)) ;
#118894=DIRECTION('ref_axis',(1.,0.,0.)) ;
#118895=DIRECTION('center_axis',(-1.,0.,9.8563833862319E-18)) ;
#118896=DIRECTION('ref_axis',(9.8563833862319E-18,0.,1.)) ;
#118897=DIRECTION('center_axis',(-1.,3.93023287525994E-15,-3.93023287525994E-15)) ;
#118898=DIRECTION('ref_axis',(-3.93023287525994E-15,-1.34524652575182E-43,
1.)) ;
#118899=DIRECTION('center_axis',(2.08166817117218E-16,1.,0.)) ;
#118900=DIRECTION('ref_axis',(1.,0.,0.)) ;
#118901=DIRECTION('center_axis',(-1.,-4.33680868994201E-15,-4.33680868994201E-15)) ;
#118902=DIRECTION('ref_axis',(4.33680868994201E-15,-1.59748024933029E-43,
-1.)) ;
#118903=DIRECTION('center_axis',(2.08166817117218E-16,1.,0.)) ;
#118904=DIRECTION('ref_axis',(1.,0.,0.)) ;
#118905=DIRECTION('center_axis',(-0.577350269189625,0.577350269189624,-0.577350269189628)) ;
#118906=DIRECTION('ref_axis',(0.707106781186549,-6.77492742903108E-16,-0.707106781186546)) ;
#118907=DIRECTION('center_axis',(0.,0.,1.)) ;
#118908=DIRECTION('ref_axis',(-1.,0.,0.)) ;
#118909=DIRECTION('center_axis',(-1.,0.,-9.8563833862319E-18)) ;
#118910=DIRECTION('ref_axis',(-9.8563833862319E-18,0.,1.)) ;
#118911=DIRECTION('center_axis',(-1.,0.,-9.00809882301481E-15)) ;
#118912=DIRECTION('ref_axis',(-9.00809882301481E-15,0.,1.)) ;
#118913=DIRECTION('center_axis',(0.,0.,-1.)) ;
#118914=DIRECTION('ref_axis',(-1.,0.,0.)) ;
#118915=DIRECTION('center_axis',(0.,0.,1.)) ;
#118916=DIRECTION('ref_axis',(1.,0.,0.)) ;
#118917=DIRECTION('center_axis',(0.577350269189625,-0.577350269189625,0.577350269189628)) ;
#118918=DIRECTION('ref_axis',(0.707106781186549,-7.23605167296792E-16,-0.707106781186546)) ;
#118919=DIRECTION('center_axis',(0.577350269189625,-0.577350269189625,0.577350269189628)) ;
#118920=DIRECTION('ref_axis',(0.707106781186549,-7.51360742912421E-16,-0.707106781186546)) ;
#118921=DIRECTION('center_axis',(2.08166817117218E-16,1.,0.)) ;
#118922=DIRECTION('ref_axis',(1.,0.,0.)) ;
#118923=DIRECTION('center_axis',(-0.57735026918963,0.577350269189624,0.577350269189624)) ;
#118924=DIRECTION('ref_axis',(-0.707106781186544,-8.1317851962192E-16,-0.707106781186551)) ;
#118925=DIRECTION('center_axis',(0.,0.,-1.)) ;
#118926=DIRECTION('ref_axis',(-1.,0.,0.)) ;
#118927=DIRECTION('center_axis',(0.,0.,1.)) ;
#118928=DIRECTION('ref_axis',(-1.,0.,0.)) ;
#118929=DIRECTION('center_axis',(0.,0.,-1.)) ;
#118930=DIRECTION('ref_axis',(-1.,0.,0.)) ;
#118931=DIRECTION('center_axis',(-0.577350269189625,0.577350269189625,0.577350269189628)) ;
#118932=DIRECTION('ref_axis',(0.707106781186549,-7.51360742912421E-16,0.707106781186546)) ;
#118933=DIRECTION('center_axis',(0.577350269189625,-0.577350269189625,-0.577350269189628)) ;
#118934=DIRECTION('ref_axis',(0.707106781186545,-8.51940988246475E-15,0.70710678118655)) ;
#118935=DIRECTION('center_axis',(-0.577350269189625,0.577350269189626,-0.577350269189626)) ;
#118936=DIRECTION('ref_axis',(6.27941990732594E-17,0.707106781186548,0.707106781186548)) ;
#118937=DIRECTION('center_axis',(0.577350269189625,-0.577350269189626,0.577350269189626)) ;
#118938=DIRECTION('ref_axis',(-6.96183268087023E-15,0.707106781186544,0.707106781186551)) ;
#118939=DIRECTION('center_axis',(0.577350269189619,-0.57735026918964,0.577350269189619)) ;
#118940=DIRECTION('ref_axis',(0.70710678118656,0.707106781186535,9.56388759536482E-16)) ;
#118941=DIRECTION('center_axis',(0.,0.,-1.)) ;
#118942=DIRECTION('ref_axis',(-1.,0.,0.)) ;
#118943=DIRECTION('center_axis',(0.,0.,1.)) ;
#118944=DIRECTION('ref_axis',(-1.,0.,0.)) ;
#118945=DIRECTION('center_axis',(0.,0.,-1.)) ;
#118946=DIRECTION('ref_axis',(-1.,0.,0.)) ;
#118947=DIRECTION('center_axis',(0.,1.,0.)) ;
#118948=DIRECTION('ref_axis',(1.,0.,0.)) ;
#118949=DIRECTION('center_axis',(0.,-1.,-5.94151198964807E-15)) ;
#118950=DIRECTION('ref_axis',(0.,-5.94151198964807E-15,1.)) ;
#118951=DIRECTION('center_axis',(1.7347234759768E-14,-1.73472347597681E-14,
1.)) ;
#118952=DIRECTION('ref_axis',(-1.79366203433577E-43,1.,1.73472347597681E-14)) ;
#118953=DIRECTION('center_axis',(0.577350269189625,-0.577350269189626,-0.577350269189626)) ;
#118954=DIRECTION('ref_axis',(6.27941990732594E-17,0.707106781186548,-0.707106781186548)) ;
#118955=DIRECTION('center_axis',(0.577350269189625,-0.577350269189626,-0.577350269189626)) ;
#118956=DIRECTION('ref_axis',(3.83287980137187E-16,0.707106781186548,-0.707106781186547)) ;
#118957=DIRECTION('center_axis',(0.57735026918963,-0.577350269189631,-0.577350269189617)) ;
#118958=DIRECTION('ref_axis',(0.707106781186548,0.707106781186547,-9.21608659434825E-17)) ;
#118959=DIRECTION('center_axis',(0.,0.,-1.)) ;
#118960=DIRECTION('ref_axis',(-1.,0.,0.)) ;
#118961=DIRECTION('center_axis',(0.,0.,1.)) ;
#118962=DIRECTION('ref_axis',(1.,0.,0.)) ;
#118963=DIRECTION('center_axis',(0.,1.,1.95511867169518E-16)) ;
#118964=DIRECTION('ref_axis',(0.,-1.95511867169518E-16,1.)) ;
#118965=DIRECTION('center_axis',(1.15196480826585E-15,-1.,9.60303131180424E-16)) ;
#118966=DIRECTION('ref_axis',(1.,1.15196480826585E-15,0.)) ;
#118967=DIRECTION('center_axis',(0.,1.,0.)) ;
#118968=DIRECTION('ref_axis',(1.,0.,0.)) ;
#118969=DIRECTION('center_axis',(-7.5216525716181E-15,-1.,7.71331424870352E-15)) ;
#118970=DIRECTION('ref_axis',(-8.74484647013228E-32,7.71331424870352E-15,
1.)) ;
#118971=DIRECTION('center_axis',(0.,1.,0.)) ;
#118972=DIRECTION('ref_axis',(1.,0.,0.)) ;
#118973=DIRECTION('center_axis',(-0.577350269189626,-0.577350269189627,
-0.577350269189625)) ;
#118974=DIRECTION('ref_axis',(-0.707106781186548,0.707106781186547,-9.19305248608458E-17)) ;
#118975=DIRECTION('center_axis',(0.,0.,1.)) ;
#118976=DIRECTION('ref_axis',(-1.,1.76182853028894E-15,0.)) ;
#118977=DIRECTION('center_axis',(0.,1.,-1.95511867169518E-16)) ;
#118978=DIRECTION('ref_axis',(0.,1.95511867169518E-16,1.)) ;
#118979=DIRECTION('center_axis',(0.,-1.,-7.95395959904499E-15)) ;
#118980=DIRECTION('ref_axis',(0.,7.95395959904499E-15,-1.)) ;
#118981=DIRECTION('center_axis',(0.,0.,-1.)) ;
#118982=DIRECTION('ref_axis',(-1.,0.,0.)) ;
#118983=DIRECTION('center_axis',(0.,0.,1.)) ;
#118984=DIRECTION('ref_axis',(1.,0.,0.)) ;
#118985=DIRECTION('center_axis',(0.577350269189625,0.577350269189626,0.577350269189627)) ;
#118986=DIRECTION('ref_axis',(-2.71345386026911E-16,-0.707106781186548,
0.707106781186547)) ;
#118987=DIRECTION('center_axis',(0.577350269189625,0.577350269189626,0.577350269189627)) ;
#118988=DIRECTION('ref_axis',(-2.71345386026911E-16,-0.707106781186548,
0.707106781186547)) ;
#118989=DIRECTION('center_axis',(0.,1.,0.)) ;
#118990=DIRECTION('ref_axis',(1.,0.,0.)) ;
#118991=DIRECTION('center_axis',(-0.577350269189622,-0.577350269189633,
0.577350269189622)) ;
#118992=DIRECTION('ref_axis',(-1.42949951585321E-15,0.707106781186542,0.707106781186553)) ;
#118993=DIRECTION('center_axis',(0.,0.,-1.)) ;
#118994=DIRECTION('ref_axis',(-1.,0.,0.)) ;
#118995=DIRECTION('center_axis',(0.,0.,1.)) ;
#118996=DIRECTION('ref_axis',(-1.,1.0842021724855E-15,0.)) ;
#118997=DIRECTION('center_axis',(0.,0.,-1.)) ;
#118998=DIRECTION('ref_axis',(-1.,0.,0.)) ;
#118999=DIRECTION('center_axis',(-0.577350269189625,-0.577350269189626,
0.577350269189627)) ;
#119000=DIRECTION('ref_axis',(-2.71345386026911E-16,-0.707106781186548,
-0.707106781186547)) ;
#119001=DIRECTION('center_axis',(0.577350269189625,0.577350269189626,-0.577350269189627)) ;
#119002=DIRECTION('ref_axis',(-2.71345386026911E-16,-0.707106781186548,
-0.707106781186547)) ;
#119003=DIRECTION('center_axis',(0.577350269189625,0.577350269189625,-0.577350269189628)) ;
#119004=DIRECTION('ref_axis',(-0.707106781186552,5.19478420936363E-15,-0.707106781186543)) ;
#119005=DIRECTION('center_axis',(-0.577350269189625,-0.577350269189625,
0.577350269189628)) ;
#119006=DIRECTION('ref_axis',(-0.707106781186566,3.31891725521342E-14,-0.707106781186529)) ;
#119007=DIRECTION('center_axis',(-0.577350269189652,-0.577350269189606,
0.57735026918962)) ;
#119008=DIRECTION('ref_axis',(0.707106781186528,-3.96520952299298E-16,0.707106781186567)) ;
#119009=DIRECTION('center_axis',(0.,0.,-1.)) ;
#119010=DIRECTION('ref_axis',(-1.,0.,0.)) ;
#119011=DIRECTION('center_axis',(0.,0.,1.)) ;
#119012=DIRECTION('ref_axis',(-1.,-8.67361737988404E-15,0.)) ;
#119013=DIRECTION('center_axis',(0.,0.,-1.)) ;
#119014=DIRECTION('ref_axis',(-1.,0.,0.)) ;
#119015=DIRECTION('center_axis',(2.08166817117218E-16,1.,0.)) ;
#119016=DIRECTION('ref_axis',(1.,0.,0.)) ;
#119017=DIRECTION('center_axis',(-1.,0.,-1.66745659064321E-14)) ;
#119018=DIRECTION('ref_axis',(1.66745659064321E-14,2.60208521396523E-14,
-1.)) ;
#119019=DIRECTION('center_axis',(-3.46944695195361E-14,-3.4694469519536E-14,
1.)) ;
#119020=DIRECTION('ref_axis',(-1.,-1.68611237719883E-42,-3.46944695195361E-14)) ;
#119021=DIRECTION('center_axis',(-0.577350269189625,-0.577350269189625,
-0.577350269189628)) ;
#119022=DIRECTION('ref_axis',(-0.707106781186552,5.19478420936363E-15,0.707106781186543)) ;
#119023=DIRECTION('center_axis',(-0.577350269189625,-0.577350269189625,
-0.577350269189628)) ;
#119024=DIRECTION('ref_axis',(-0.707106781186552,5.1349792556416E-15,0.707106781186543)) ;
#119025=DIRECTION('center_axis',(-0.577350269189626,-0.577350269189626,
-0.577350269189626)) ;
#119026=DIRECTION('ref_axis',(0.707106781186547,-0.707106781186548,6.36902276417946E-16)) ;
#119027=DIRECTION('center_axis',(0.,0.,-1.)) ;
#119028=DIRECTION('ref_axis',(-1.,0.,0.)) ;
#119029=DIRECTION('center_axis',(0.,0.,1.)) ;
#119030=DIRECTION('ref_axis',(1.,0.,0.)) ;
#119031=DIRECTION('center_axis',(-1.,0.,9.8563833862319E-18)) ;
#119032=DIRECTION('ref_axis',(9.8563833862319E-18,0.,1.)) ;
#119033=DIRECTION('center_axis',(-1.,8.87690528722497E-15,-8.87690528722518E-15)) ;
#119034=DIRECTION('ref_axis',(-8.87690528722518E-15,4.48415508583942E-43,
1.)) ;
#119035=DIRECTION('center_axis',(2.08166817117218E-16,1.,0.)) ;
#119036=DIRECTION('ref_axis',(1.,0.,0.)) ;
#119037=DIRECTION('center_axis',(-1.,8.53809210832325E-15,8.53809210832346E-15)) ;
#119038=DIRECTION('ref_axis',(-8.53809210832339E-15,8.67361737988409E-15,
-1.)) ;
#119039=DIRECTION('center_axis',(2.08166817117218E-16,1.,0.)) ;
#119040=DIRECTION('ref_axis',(1.,0.,0.)) ;
#119041=DIRECTION('center_axis',(-0.577350269189622,0.577350269189621,-0.577350269189634)) ;
#119042=DIRECTION('ref_axis',(0.707106781186563,1.66970714627838E-14,-0.707106781186532)) ;
#119043=DIRECTION('center_axis',(0.,0.,1.)) ;
#119044=DIRECTION('ref_axis',(-1.,0.,0.)) ;
#119045=DIRECTION('center_axis',(-1.,0.,-9.8563833862319E-18)) ;
#119046=DIRECTION('ref_axis',(-9.8563833862319E-18,0.,1.)) ;
#119047=DIRECTION('center_axis',(-1.,0.,-1.34163173959798E-15)) ;
#119048=DIRECTION('ref_axis',(-1.34163173959798E-15,0.,1.)) ;
#119049=DIRECTION('center_axis',(0.,0.,-1.)) ;
#119050=DIRECTION('ref_axis',(-1.,0.,0.)) ;
#119051=DIRECTION('center_axis',(-3.46944695195361E-14,3.4694469519536E-14,
1.)) ;
#119052=DIRECTION('ref_axis',(1.,-1.68611237719883E-42,3.46944695195361E-14)) ;
#119053=DIRECTION('center_axis',(0.577350269189625,-0.577350269189625,0.577350269189628)) ;
#119054=DIRECTION('ref_axis',(0.707106781186552,5.19478420936363E-15,-0.707106781186543)) ;
#119055=DIRECTION('center_axis',(0.577350269189625,-0.577350269189625,0.577350269189628)) ;
#119056=DIRECTION('ref_axis',(0.707106781186552,5.1349792556416E-15,-0.707106781186543)) ;
#119057=DIRECTION('center_axis',(2.08166817117218E-16,1.,0.)) ;
#119058=DIRECTION('ref_axis',(1.,0.,0.)) ;
#119059=DIRECTION('center_axis',(-0.577350269189646,0.577350269189609,0.577350269189623)) ;
#119060=DIRECTION('ref_axis',(-0.707106781186529,8.66006384940495E-15,-0.707106781186566)) ;
#119061=DIRECTION('center_axis',(0.,0.,-1.)) ;
#119062=DIRECTION('ref_axis',(-1.,0.,0.)) ;
#119063=DIRECTION('center_axis',(0.,0.,1.)) ;
#119064=DIRECTION('ref_axis',(-1.,0.,0.)) ;
#119065=DIRECTION('center_axis',(0.,0.,-1.)) ;
#119066=DIRECTION('ref_axis',(-1.,0.,0.)) ;
#119067=DIRECTION('center_axis',(-0.577350269189625,0.577350269189625,0.577350269189628)) ;
#119068=DIRECTION('ref_axis',(0.707106781186552,5.1349792556416E-15,0.707106781186543)) ;
#119069=DIRECTION('center_axis',(0.577350269189625,-0.577350269189625,-0.577350269189628)) ;
#119070=DIRECTION('ref_axis',(0.707106781186559,1.92955635991398E-14,0.707106781186536)) ;
#119071=DIRECTION('center_axis',(-0.577350269189625,0.577350269189626,-0.577350269189626)) ;
#119072=DIRECTION('ref_axis',(5.20172641667636E-15,0.70710678118655,0.707106781186545)) ;
#119073=DIRECTION('center_axis',(0.577350269189625,-0.577350269189626,0.577350269189626)) ;
#119074=DIRECTION('ref_axis',(1.27903606950626E-14,0.707106781186554,0.707106781186541)) ;
#119075=DIRECTION('center_axis',(0.577350269189636,-0.577350269189592,0.57735026918965)) ;
#119076=DIRECTION('ref_axis',(0.707106781186558,3.40611850366138E-15,-0.707106781186537)) ;
#119077=DIRECTION('center_axis',(0.,0.,-1.)) ;
#119078=DIRECTION('ref_axis',(-1.,0.,0.)) ;
#119079=DIRECTION('center_axis',(0.,0.,1.)) ;
#119080=DIRECTION('ref_axis',(-1.,1.57209315010398E-14,0.)) ;
#119081=DIRECTION('center_axis',(0.,0.,-1.)) ;
#119082=DIRECTION('ref_axis',(-1.,0.,0.)) ;
#119083=DIRECTION('center_axis',(0.,1.,0.)) ;
#119084=DIRECTION('ref_axis',(1.,0.,0.)) ;
#119085=DIRECTION('center_axis',(0.,-1.,7.76229792195976E-15)) ;
#119086=DIRECTION('ref_axis',(3.46944695195364E-14,7.76229792195976E-15,
1.)) ;
#119087=DIRECTION('center_axis',(-3.46944695195361E-14,3.46944695195361E-14,
1.)) ;
#119088=DIRECTION('ref_axis',(-7.17464813734306E-43,1.,-3.46944695195361E-14)) ;
#119089=DIRECTION('center_axis',(0.577350269189625,-0.577350269189626,-0.577350269189626)) ;
#119090=DIRECTION('ref_axis',(5.20172641667636E-15,0.70710678118655,-0.707106781186545)) ;
#119091=DIRECTION('center_axis',(0.577350269189625,-0.577350269189626,-0.577350269189626)) ;
#119092=DIRECTION('ref_axis',(5.11416588733871E-15,0.70710678118655,-0.707106781186545)) ;
#119093=DIRECTION('center_axis',(0.577350269189624,-0.577350269189625,-0.577350269189629)) ;
#119094=DIRECTION('ref_axis',(4.29556475679742E-15,0.707106781186552,-0.707106781186543)) ;
#119095=DIRECTION('center_axis',(0.,0.,-1.)) ;
#119096=DIRECTION('ref_axis',(-1.,0.,0.)) ;
#119097=DIRECTION('center_axis',(0.,0.,1.)) ;
#119098=DIRECTION('ref_axis',(1.,0.,0.)) ;
#119099=DIRECTION('center_axis',(0.,1.,1.95511867169518E-16)) ;
#119100=DIRECTION('ref_axis',(0.,-1.95511867169518E-16,1.)) ;
#119101=DIRECTION('center_axis',(-7.65717784317885E-15,-1.,-7.84883952026447E-15)) ;
#119102=DIRECTION('ref_axis',(-8.90241127119925E-32,7.84883952026447E-15,
-1.)) ;
#119103=DIRECTION('center_axis',(0.,1.,0.)) ;
#119104=DIRECTION('ref_axis',(1.,0.,0.)) ;
#119105=DIRECTION('center_axis',(-1.28749007982652E-15,-1.,1.47915175691198E-15)) ;
#119106=DIRECTION('ref_axis',(3.46944695195364E-14,1.47915175691194E-15,
1.)) ;
#119107=DIRECTION('center_axis',(0.,1.,0.)) ;
#119108=DIRECTION('ref_axis',(1.,0.,0.)) ;
#119109=DIRECTION('center_axis',(-0.577350269189619,-0.577350269189621,
-0.577350269189638)) ;
#119110=DIRECTION('ref_axis',(1.66660234080318E-14,-0.707106781186566,0.707106781186529)) ;
#119111=DIRECTION('center_axis',(0.,0.,1.)) ;
#119112=DIRECTION('ref_axis',(-1.,-3.52365706057788E-15,0.)) ;
#119113=DIRECTION('center_axis',(0.,1.,-1.95511867169518E-16)) ;
#119114=DIRECTION('ref_axis',(0.,1.95511867169518E-16,1.)) ;
#119115=DIRECTION('center_axis',(0.,-1.,3.06658683336682E-15)) ;
#119116=DIRECTION('ref_axis',(0.,-3.06658683336682E-15,-1.)) ;
#119117=DIRECTION('center_axis',(0.,0.,-1.)) ;
#119118=DIRECTION('ref_axis',(-1.,0.,0.)) ;
#119119=DIRECTION('center_axis',(-3.4694469519536E-14,-3.46944695195361E-14,
1.)) ;
#119120=DIRECTION('ref_axis',(-8.96831017167883E-43,-1.,-3.46944695195361E-14)) ;
#119121=DIRECTION('center_axis',(0.577350269189625,0.577350269189626,0.577350269189627)) ;
#119122=DIRECTION('ref_axis',(5.35231302451417E-15,-0.707106781186551,0.707106781186544)) ;
#119123=DIRECTION('center_axis',(0.577350269189625,0.577350269189626,0.577350269189627)) ;
#119124=DIRECTION('ref_axis',(5.35231302451417E-15,-0.707106781186551,0.707106781186544)) ;
#119125=DIRECTION('center_axis',(0.,1.,0.)) ;
#119126=DIRECTION('ref_axis',(1.,0.,0.)) ;
#119127=DIRECTION('center_axis',(-0.577350269189609,-0.577350269189646,
0.577350269189623)) ;
#119128=DIRECTION('ref_axis',(8.91337114590872E-15,0.707106781186529,0.707106781186566)) ;
#119129=DIRECTION('center_axis',(0.,0.,-1.)) ;
#119130=DIRECTION('ref_axis',(-1.,0.,0.)) ;
#119131=DIRECTION('center_axis',(0.,0.,1.)) ;
#119132=DIRECTION('ref_axis',(-1.,1.0842021724855E-15,0.)) ;
#119133=DIRECTION('center_axis',(0.,0.,-1.)) ;
#119134=DIRECTION('ref_axis',(-1.,0.,0.)) ;
#119135=DIRECTION('center_axis',(-0.577350269189625,-0.577350269189626,
0.577350269189627)) ;
#119136=DIRECTION('ref_axis',(5.35231302451417E-15,-0.707106781186551,-0.707106781186544)) ;
#119137=DIRECTION('center_axis',(0.577350269189625,0.577350269189626,-0.577350269189627)) ;
#119138=DIRECTION('ref_axis',(-6.40836823623517E-14,-0.707106781186516,
-0.707106781186579)) ;
#119139=DIRECTION('center_axis',(0.577350269189625,0.577350269189625,-0.577350269189628)) ;
#119140=DIRECTION('ref_axis',(-0.707106781186552,5.19478420936363E-15,-0.707106781186543)) ;
#119141=DIRECTION('center_axis',(-0.577350269189625,-0.577350269189625,
0.577350269189628)) ;
#119142=DIRECTION('ref_axis',(-0.707106781186566,3.31891725521342E-14,-0.707106781186529)) ;
#119143=DIRECTION('center_axis',(-0.577350269189652,-0.577350269189606,
0.57735026918962)) ;
#119144=DIRECTION('ref_axis',(0.707106781186528,-3.96520952299298E-16,0.707106781186567)) ;
#119145=DIRECTION('center_axis',(0.,0.,-1.)) ;
#119146=DIRECTION('ref_axis',(-1.,0.,0.)) ;
#119147=DIRECTION('center_axis',(0.,0.,1.)) ;
#119148=DIRECTION('ref_axis',(-1.,-8.67361737988404E-15,0.)) ;
#119149=DIRECTION('center_axis',(0.,0.,-1.)) ;
#119150=DIRECTION('ref_axis',(-1.,0.,0.)) ;
#119151=DIRECTION('center_axis',(2.08166817117218E-16,1.,0.)) ;
#119152=DIRECTION('ref_axis',(1.,0.,0.)) ;
#119153=DIRECTION('center_axis',(-1.,0.,-1.66745659064321E-14)) ;
#119154=DIRECTION('ref_axis',(1.66745659064321E-14,2.60208521396523E-14,
-1.)) ;
#119155=DIRECTION('center_axis',(-3.46944695195361E-14,-3.4694469519536E-14,
1.)) ;
#119156=DIRECTION('ref_axis',(-1.,-1.68611237719883E-42,-3.46944695195361E-14)) ;
#119157=DIRECTION('center_axis',(-0.577350269189625,-0.577350269189625,
-0.577350269189628)) ;
#119158=DIRECTION('ref_axis',(-0.707106781186552,5.19478420936363E-15,0.707106781186543)) ;
#119159=DIRECTION('center_axis',(-0.577350269189625,-0.577350269189625,
-0.577350269189628)) ;
#119160=DIRECTION('ref_axis',(-0.707106781186552,5.1349792556416E-15,0.707106781186543)) ;
#119161=DIRECTION('center_axis',(-0.577350269189626,-0.577350269189626,
-0.577350269189626)) ;
#119162=DIRECTION('ref_axis',(0.707106781186547,-0.707106781186548,6.36902276417946E-16)) ;
#119163=DIRECTION('center_axis',(0.,0.,-1.)) ;
#119164=DIRECTION('ref_axis',(-1.,0.,0.)) ;
#119165=DIRECTION('center_axis',(0.,0.,1.)) ;
#119166=DIRECTION('ref_axis',(1.,0.,0.)) ;
#119167=DIRECTION('center_axis',(-1.,0.,9.8563833862319E-18)) ;
#119168=DIRECTION('ref_axis',(9.8563833862319E-18,0.,1.)) ;
#119169=DIRECTION('center_axis',(-1.,8.87690528722497E-15,-8.87690528722518E-15)) ;
#119170=DIRECTION('ref_axis',(-8.87690528722518E-15,4.48415508583942E-43,
1.)) ;
#119171=DIRECTION('center_axis',(2.08166817117218E-16,1.,0.)) ;
#119172=DIRECTION('ref_axis',(1.,0.,0.)) ;
#119173=DIRECTION('center_axis',(-1.,8.53809210832325E-15,8.53809210832346E-15)) ;
#119174=DIRECTION('ref_axis',(-8.53809210832339E-15,8.67361737988409E-15,
-1.)) ;
#119175=DIRECTION('center_axis',(2.08166817117218E-16,1.,0.)) ;
#119176=DIRECTION('ref_axis',(1.,0.,0.)) ;
#119177=DIRECTION('center_axis',(-0.577350269189622,0.577350269189621,-0.577350269189634)) ;
#119178=DIRECTION('ref_axis',(0.707106781186563,1.66970714627838E-14,-0.707106781186532)) ;
#119179=DIRECTION('center_axis',(0.,0.,1.)) ;
#119180=DIRECTION('ref_axis',(-1.,0.,0.)) ;
#119181=DIRECTION('center_axis',(-1.,0.,-9.8563833862319E-18)) ;
#119182=DIRECTION('ref_axis',(-9.8563833862319E-18,0.,1.)) ;
#119183=DIRECTION('center_axis',(-1.,0.,-1.34163173959798E-15)) ;
#119184=DIRECTION('ref_axis',(-1.34163173959798E-15,0.,1.)) ;
#119185=DIRECTION('center_axis',(0.,0.,-1.)) ;
#119186=DIRECTION('ref_axis',(-1.,0.,0.)) ;
#119187=DIRECTION('center_axis',(-3.46944695195361E-14,3.4694469519536E-14,
1.)) ;
#119188=DIRECTION('ref_axis',(1.,-1.68611237719883E-42,3.46944695195361E-14)) ;
#119189=DIRECTION('center_axis',(0.577350269189625,-0.577350269189625,0.577350269189628)) ;
#119190=DIRECTION('ref_axis',(0.707106781186552,5.19478420936363E-15,-0.707106781186543)) ;
#119191=DIRECTION('center_axis',(0.577350269189625,-0.577350269189625,0.577350269189628)) ;
#119192=DIRECTION('ref_axis',(0.707106781186552,5.1349792556416E-15,-0.707106781186543)) ;
#119193=DIRECTION('center_axis',(2.08166817117218E-16,1.,0.)) ;
#119194=DIRECTION('ref_axis',(1.,0.,0.)) ;
#119195=DIRECTION('center_axis',(-0.577350269189646,0.577350269189609,0.577350269189623)) ;
#119196=DIRECTION('ref_axis',(-0.707106781186529,8.66006384940495E-15,-0.707106781186566)) ;
#119197=DIRECTION('center_axis',(0.,0.,-1.)) ;
#119198=DIRECTION('ref_axis',(-1.,0.,0.)) ;
#119199=DIRECTION('center_axis',(0.,0.,1.)) ;
#119200=DIRECTION('ref_axis',(-1.,0.,0.)) ;
#119201=DIRECTION('center_axis',(0.,0.,-1.)) ;
#119202=DIRECTION('ref_axis',(-1.,0.,0.)) ;
#119203=DIRECTION('center_axis',(-0.577350269189625,0.577350269189625,0.577350269189628)) ;
#119204=DIRECTION('ref_axis',(0.707106781186552,5.1349792556416E-15,0.707106781186543)) ;
#119205=DIRECTION('center_axis',(0.577350269189625,-0.577350269189625,-0.577350269189628)) ;
#119206=DIRECTION('ref_axis',(0.707106781186559,1.92955635991398E-14,0.707106781186536)) ;
#119207=DIRECTION('center_axis',(-0.577350269189625,0.577350269189626,-0.577350269189626)) ;
#119208=DIRECTION('ref_axis',(5.20172641667636E-15,0.70710678118655,0.707106781186545)) ;
#119209=DIRECTION('center_axis',(0.577350269189625,-0.577350269189626,0.577350269189626)) ;
#119210=DIRECTION('ref_axis',(1.27903606950626E-14,0.707106781186554,0.707106781186541)) ;
#119211=DIRECTION('center_axis',(0.577350269189636,-0.577350269189592,0.57735026918965)) ;
#119212=DIRECTION('ref_axis',(0.707106781186558,3.40611850366138E-15,-0.707106781186537)) ;
#119213=DIRECTION('center_axis',(0.,0.,-1.)) ;
#119214=DIRECTION('ref_axis',(-1.,0.,0.)) ;
#119215=DIRECTION('center_axis',(0.,0.,1.)) ;
#119216=DIRECTION('ref_axis',(-1.,1.57209315010398E-14,0.)) ;
#119217=DIRECTION('center_axis',(0.,0.,-1.)) ;
#119218=DIRECTION('ref_axis',(-1.,0.,0.)) ;
#119219=DIRECTION('center_axis',(0.,1.,0.)) ;
#119220=DIRECTION('ref_axis',(1.,0.,0.)) ;
#119221=DIRECTION('center_axis',(0.,-1.,7.76229792195976E-15)) ;
#119222=DIRECTION('ref_axis',(3.46944695195364E-14,7.76229792195976E-15,
1.)) ;
#119223=DIRECTION('center_axis',(-3.46944695195361E-14,3.46944695195361E-14,
1.)) ;
#119224=DIRECTION('ref_axis',(-7.17464813734306E-43,1.,-3.46944695195361E-14)) ;
#119225=DIRECTION('center_axis',(0.577350269189625,-0.577350269189626,-0.577350269189626)) ;
#119226=DIRECTION('ref_axis',(5.20172641667636E-15,0.70710678118655,-0.707106781186545)) ;
#119227=DIRECTION('center_axis',(0.577350269189625,-0.577350269189626,-0.577350269189626)) ;
#119228=DIRECTION('ref_axis',(5.11416588733871E-15,0.70710678118655,-0.707106781186545)) ;
#119229=DIRECTION('center_axis',(0.577350269189624,-0.577350269189625,-0.577350269189629)) ;
#119230=DIRECTION('ref_axis',(4.29556475679742E-15,0.707106781186552,-0.707106781186543)) ;
#119231=DIRECTION('center_axis',(0.,0.,-1.)) ;
#119232=DIRECTION('ref_axis',(-1.,0.,0.)) ;
#119233=DIRECTION('center_axis',(0.,0.,1.)) ;
#119234=DIRECTION('ref_axis',(1.,0.,0.)) ;
#119235=DIRECTION('center_axis',(0.,1.,1.95511867169518E-16)) ;
#119236=DIRECTION('ref_axis',(0.,-1.95511867169518E-16,1.)) ;
#119237=DIRECTION('center_axis',(-7.65717784317885E-15,-1.,-7.84883952026447E-15)) ;
#119238=DIRECTION('ref_axis',(-8.90241127119925E-32,7.84883952026447E-15,
-1.)) ;
#119239=DIRECTION('center_axis',(0.,1.,0.)) ;
#119240=DIRECTION('ref_axis',(1.,0.,0.)) ;
#119241=DIRECTION('center_axis',(-1.28749007982652E-15,-1.,1.47915175691198E-15)) ;
#119242=DIRECTION('ref_axis',(3.46944695195364E-14,1.47915175691194E-15,
1.)) ;
#119243=DIRECTION('center_axis',(0.,1.,0.)) ;
#119244=DIRECTION('ref_axis',(1.,0.,0.)) ;
#119245=DIRECTION('center_axis',(-0.577350269189619,-0.577350269189621,
-0.577350269189638)) ;
#119246=DIRECTION('ref_axis',(1.66660234080318E-14,-0.707106781186566,0.707106781186529)) ;
#119247=DIRECTION('center_axis',(0.,0.,1.)) ;
#119248=DIRECTION('ref_axis',(-1.,-3.52365706057788E-15,0.)) ;
#119249=DIRECTION('center_axis',(0.,1.,-1.95511867169518E-16)) ;
#119250=DIRECTION('ref_axis',(0.,1.95511867169518E-16,1.)) ;
#119251=DIRECTION('center_axis',(0.,-1.,3.06658683336682E-15)) ;
#119252=DIRECTION('ref_axis',(0.,-3.06658683336682E-15,-1.)) ;
#119253=DIRECTION('center_axis',(0.,0.,-1.)) ;
#119254=DIRECTION('ref_axis',(-1.,0.,0.)) ;
#119255=DIRECTION('center_axis',(-3.4694469519536E-14,-3.46944695195361E-14,
1.)) ;
#119256=DIRECTION('ref_axis',(-8.96831017167883E-43,-1.,-3.46944695195361E-14)) ;
#119257=DIRECTION('center_axis',(0.577350269189625,0.577350269189626,0.577350269189627)) ;
#119258=DIRECTION('ref_axis',(5.35231302451417E-15,-0.707106781186551,0.707106781186544)) ;
#119259=DIRECTION('center_axis',(0.577350269189625,0.577350269189626,0.577350269189627)) ;
#119260=DIRECTION('ref_axis',(5.35231302451417E-15,-0.707106781186551,0.707106781186544)) ;
#119261=DIRECTION('center_axis',(0.,1.,0.)) ;
#119262=DIRECTION('ref_axis',(1.,0.,0.)) ;
#119263=DIRECTION('center_axis',(-0.577350269189609,-0.577350269189646,
0.577350269189623)) ;
#119264=DIRECTION('ref_axis',(8.91337114590872E-15,0.707106781186529,0.707106781186566)) ;
#119265=DIRECTION('center_axis',(0.,0.,-1.)) ;
#119266=DIRECTION('ref_axis',(-1.,0.,0.)) ;
#119267=DIRECTION('center_axis',(0.,0.,1.)) ;
#119268=DIRECTION('ref_axis',(-1.,1.0842021724855E-15,0.)) ;
#119269=DIRECTION('center_axis',(0.,0.,-1.)) ;
#119270=DIRECTION('ref_axis',(-1.,0.,0.)) ;
#119271=DIRECTION('center_axis',(-0.577350269189625,-0.577350269189626,
0.577350269189627)) ;
#119272=DIRECTION('ref_axis',(5.35231302451417E-15,-0.707106781186551,-0.707106781186544)) ;
#119273=DIRECTION('center_axis',(0.577350269189625,0.577350269189626,-0.577350269189627)) ;
#119274=DIRECTION('ref_axis',(-6.40836823623517E-14,-0.707106781186516,
-0.707106781186579)) ;
#119275=DIRECTION('center_axis',(0.577350269189625,0.577350269189625,-0.577350269189628)) ;
#119276=DIRECTION('ref_axis',(-0.707106781186552,5.19478420936363E-15,-0.707106781186543)) ;
#119277=DIRECTION('center_axis',(-0.577350269189625,-0.577350269189625,
0.577350269189628)) ;
#119278=DIRECTION('ref_axis',(-0.707106781186566,3.31891725521342E-14,-0.707106781186529)) ;
#119279=DIRECTION('center_axis',(-0.577350269189652,-0.577350269189606,
0.57735026918962)) ;
#119280=DIRECTION('ref_axis',(0.707106781186528,-3.96520952299298E-16,0.707106781186567)) ;
#119281=DIRECTION('center_axis',(0.,0.,-1.)) ;
#119282=DIRECTION('ref_axis',(-1.,0.,0.)) ;
#119283=DIRECTION('center_axis',(0.,0.,1.)) ;
#119284=DIRECTION('ref_axis',(-1.,-8.67361737988404E-15,0.)) ;
#119285=DIRECTION('center_axis',(0.,0.,-1.)) ;
#119286=DIRECTION('ref_axis',(-1.,0.,0.)) ;
#119287=DIRECTION('center_axis',(2.08166817117218E-16,1.,0.)) ;
#119288=DIRECTION('ref_axis',(1.,0.,0.)) ;
#119289=DIRECTION('center_axis',(-1.,0.,-1.66745659064321E-14)) ;
#119290=DIRECTION('ref_axis',(1.66745659064321E-14,2.60208521396523E-14,
-1.)) ;
#119291=DIRECTION('center_axis',(-3.46944695195361E-14,-3.4694469519536E-14,
1.)) ;
#119292=DIRECTION('ref_axis',(-1.,-1.68611237719883E-42,-3.46944695195361E-14)) ;
#119293=DIRECTION('center_axis',(-0.577350269189625,-0.577350269189625,
-0.577350269189628)) ;
#119294=DIRECTION('ref_axis',(-0.707106781186552,5.19478420936363E-15,0.707106781186543)) ;
#119295=DIRECTION('center_axis',(-0.577350269189625,-0.577350269189625,
-0.577350269189628)) ;
#119296=DIRECTION('ref_axis',(-0.707106781186552,5.1349792556416E-15,0.707106781186543)) ;
#119297=DIRECTION('center_axis',(-0.577350269189626,-0.577350269189626,
-0.577350269189626)) ;
#119298=DIRECTION('ref_axis',(0.707106781186547,-0.707106781186548,6.36902276417946E-16)) ;
#119299=DIRECTION('center_axis',(0.,0.,-1.)) ;
#119300=DIRECTION('ref_axis',(-1.,0.,0.)) ;
#119301=DIRECTION('center_axis',(0.,0.,1.)) ;
#119302=DIRECTION('ref_axis',(1.,0.,0.)) ;
#119303=DIRECTION('center_axis',(-1.,0.,9.8563833862319E-18)) ;
#119304=DIRECTION('ref_axis',(9.8563833862319E-18,0.,1.)) ;
#119305=DIRECTION('center_axis',(-1.,8.87690528722497E-15,-8.87690528722518E-15)) ;
#119306=DIRECTION('ref_axis',(-8.87690528722518E-15,4.48415508583942E-43,
1.)) ;
#119307=DIRECTION('center_axis',(2.08166817117218E-16,1.,0.)) ;
#119308=DIRECTION('ref_axis',(1.,0.,0.)) ;
#119309=DIRECTION('center_axis',(-1.,8.53809210832325E-15,8.53809210832346E-15)) ;
#119310=DIRECTION('ref_axis',(-8.53809210832339E-15,8.67361737988409E-15,
-1.)) ;
#119311=DIRECTION('center_axis',(2.08166817117218E-16,1.,0.)) ;
#119312=DIRECTION('ref_axis',(1.,0.,0.)) ;
#119313=DIRECTION('center_axis',(-0.577350269189622,0.577350269189621,-0.577350269189634)) ;
#119314=DIRECTION('ref_axis',(0.707106781186563,1.66970714627838E-14,-0.707106781186532)) ;
#119315=DIRECTION('center_axis',(0.,0.,1.)) ;
#119316=DIRECTION('ref_axis',(-1.,0.,0.)) ;
#119317=DIRECTION('center_axis',(-1.,0.,-9.8563833862319E-18)) ;
#119318=DIRECTION('ref_axis',(-9.8563833862319E-18,0.,1.)) ;
#119319=DIRECTION('center_axis',(-1.,0.,-1.34163173959798E-15)) ;
#119320=DIRECTION('ref_axis',(-1.34163173959798E-15,0.,1.)) ;
#119321=DIRECTION('center_axis',(0.,0.,-1.)) ;
#119322=DIRECTION('ref_axis',(-1.,0.,0.)) ;
#119323=DIRECTION('center_axis',(-3.46944695195361E-14,3.4694469519536E-14,
1.)) ;
#119324=DIRECTION('ref_axis',(1.,-1.68611237719883E-42,3.46944695195361E-14)) ;
#119325=DIRECTION('center_axis',(0.577350269189625,-0.577350269189625,0.577350269189628)) ;
#119326=DIRECTION('ref_axis',(0.707106781186552,5.19478420936363E-15,-0.707106781186543)) ;
#119327=DIRECTION('center_axis',(0.577350269189625,-0.577350269189625,0.577350269189628)) ;
#119328=DIRECTION('ref_axis',(0.707106781186552,5.1349792556416E-15,-0.707106781186543)) ;
#119329=DIRECTION('center_axis',(2.08166817117218E-16,1.,0.)) ;
#119330=DIRECTION('ref_axis',(1.,0.,0.)) ;
#119331=DIRECTION('center_axis',(-0.577350269189646,0.577350269189609,0.577350269189623)) ;
#119332=DIRECTION('ref_axis',(-0.707106781186529,8.66006384940495E-15,-0.707106781186566)) ;
#119333=DIRECTION('center_axis',(0.,0.,-1.)) ;
#119334=DIRECTION('ref_axis',(-1.,0.,0.)) ;
#119335=DIRECTION('center_axis',(0.,0.,1.)) ;
#119336=DIRECTION('ref_axis',(-1.,0.,0.)) ;
#119337=DIRECTION('center_axis',(0.,0.,-1.)) ;
#119338=DIRECTION('ref_axis',(-1.,0.,0.)) ;
#119339=DIRECTION('center_axis',(-0.577350269189625,0.577350269189625,0.577350269189628)) ;
#119340=DIRECTION('ref_axis',(0.707106781186552,5.1349792556416E-15,0.707106781186543)) ;
#119341=DIRECTION('center_axis',(0.577350269189625,-0.577350269189625,-0.577350269189628)) ;
#119342=DIRECTION('ref_axis',(0.707106781186559,1.92955635991398E-14,0.707106781186536)) ;
#119343=DIRECTION('center_axis',(-0.577350269189625,0.577350269189626,-0.577350269189626)) ;
#119344=DIRECTION('ref_axis',(5.20172641667636E-15,0.70710678118655,0.707106781186545)) ;
#119345=DIRECTION('center_axis',(0.577350269189625,-0.577350269189626,0.577350269189626)) ;
#119346=DIRECTION('ref_axis',(1.27903606950626E-14,0.707106781186554,0.707106781186541)) ;
#119347=DIRECTION('center_axis',(0.577350269189636,-0.577350269189592,0.57735026918965)) ;
#119348=DIRECTION('ref_axis',(0.707106781186558,3.40611850366138E-15,-0.707106781186537)) ;
#119349=DIRECTION('center_axis',(0.,0.,-1.)) ;
#119350=DIRECTION('ref_axis',(-1.,0.,0.)) ;
#119351=DIRECTION('center_axis',(0.,0.,1.)) ;
#119352=DIRECTION('ref_axis',(-1.,1.57209315010398E-14,0.)) ;
#119353=DIRECTION('center_axis',(0.,0.,-1.)) ;
#119354=DIRECTION('ref_axis',(-1.,0.,0.)) ;
#119355=DIRECTION('center_axis',(0.,1.,0.)) ;
#119356=DIRECTION('ref_axis',(1.,0.,0.)) ;
#119357=DIRECTION('center_axis',(0.,-1.,7.76229792195976E-15)) ;
#119358=DIRECTION('ref_axis',(3.46944695195364E-14,7.76229792195976E-15,
1.)) ;
#119359=DIRECTION('center_axis',(-3.46944695195361E-14,3.46944695195361E-14,
1.)) ;
#119360=DIRECTION('ref_axis',(-7.17464813734306E-43,1.,-3.46944695195361E-14)) ;
#119361=DIRECTION('center_axis',(0.577350269189625,-0.577350269189626,-0.577350269189626)) ;
#119362=DIRECTION('ref_axis',(5.20172641667636E-15,0.70710678118655,-0.707106781186545)) ;
#119363=DIRECTION('center_axis',(0.577350269189625,-0.577350269189626,-0.577350269189626)) ;
#119364=DIRECTION('ref_axis',(5.11416588733871E-15,0.70710678118655,-0.707106781186545)) ;
#119365=DIRECTION('center_axis',(0.577350269189624,-0.577350269189625,-0.577350269189629)) ;
#119366=DIRECTION('ref_axis',(4.29556475679742E-15,0.707106781186552,-0.707106781186543)) ;
#119367=DIRECTION('center_axis',(0.,0.,-1.)) ;
#119368=DIRECTION('ref_axis',(-1.,0.,0.)) ;
#119369=DIRECTION('center_axis',(0.,0.,1.)) ;
#119370=DIRECTION('ref_axis',(1.,0.,0.)) ;
#119371=DIRECTION('center_axis',(0.,1.,1.95511867169518E-16)) ;
#119372=DIRECTION('ref_axis',(0.,-1.95511867169518E-16,1.)) ;
#119373=DIRECTION('center_axis',(-7.65717784317885E-15,-1.,-7.84883952026447E-15)) ;
#119374=DIRECTION('ref_axis',(-8.90241127119925E-32,7.84883952026447E-15,
-1.)) ;
#119375=DIRECTION('center_axis',(0.,1.,0.)) ;
#119376=DIRECTION('ref_axis',(1.,0.,0.)) ;
#119377=DIRECTION('center_axis',(-1.28749007982652E-15,-1.,1.47915175691198E-15)) ;
#119378=DIRECTION('ref_axis',(3.46944695195364E-14,1.47915175691194E-15,
1.)) ;
#119379=DIRECTION('center_axis',(0.,1.,0.)) ;
#119380=DIRECTION('ref_axis',(1.,0.,0.)) ;
#119381=DIRECTION('center_axis',(-0.577350269189619,-0.577350269189621,
-0.577350269189638)) ;
#119382=DIRECTION('ref_axis',(1.66660234080318E-14,-0.707106781186566,0.707106781186529)) ;
#119383=DIRECTION('center_axis',(0.,0.,1.)) ;
#119384=DIRECTION('ref_axis',(-1.,-3.52365706057788E-15,0.)) ;
#119385=DIRECTION('center_axis',(0.,1.,-1.95511867169518E-16)) ;
#119386=DIRECTION('ref_axis',(0.,1.95511867169518E-16,1.)) ;
#119387=DIRECTION('center_axis',(0.,-1.,3.06658683336682E-15)) ;
#119388=DIRECTION('ref_axis',(0.,-3.06658683336682E-15,-1.)) ;
#119389=DIRECTION('center_axis',(0.,0.,-1.)) ;
#119390=DIRECTION('ref_axis',(-1.,0.,0.)) ;
#119391=DIRECTION('center_axis',(-3.4694469519536E-14,-3.46944695195361E-14,
1.)) ;
#119392=DIRECTION('ref_axis',(-8.96831017167883E-43,-1.,-3.46944695195361E-14)) ;
#119393=DIRECTION('center_axis',(0.577350269189625,0.577350269189626,0.577350269189627)) ;
#119394=DIRECTION('ref_axis',(5.35231302451417E-15,-0.707106781186551,0.707106781186544)) ;
#119395=DIRECTION('center_axis',(0.577350269189625,0.577350269189626,0.577350269189627)) ;
#119396=DIRECTION('ref_axis',(5.35231302451417E-15,-0.707106781186551,0.707106781186544)) ;
#119397=DIRECTION('center_axis',(0.,1.,0.)) ;
#119398=DIRECTION('ref_axis',(1.,0.,0.)) ;
#119399=DIRECTION('center_axis',(-0.577350269189609,-0.577350269189646,
0.577350269189623)) ;
#119400=DIRECTION('ref_axis',(8.91337114590872E-15,0.707106781186529,0.707106781186566)) ;
#119401=DIRECTION('center_axis',(0.,0.,-1.)) ;
#119402=DIRECTION('ref_axis',(-1.,0.,0.)) ;
#119403=DIRECTION('center_axis',(0.,0.,1.)) ;
#119404=DIRECTION('ref_axis',(-1.,1.0842021724855E-15,0.)) ;
#119405=DIRECTION('center_axis',(0.,0.,-1.)) ;
#119406=DIRECTION('ref_axis',(-1.,0.,0.)) ;
#119407=DIRECTION('center_axis',(-0.577350269189625,-0.577350269189626,
0.577350269189627)) ;
#119408=DIRECTION('ref_axis',(5.35231302451417E-15,-0.707106781186551,-0.707106781186544)) ;
#119409=DIRECTION('center_axis',(0.577350269189625,0.577350269189626,-0.577350269189627)) ;
#119410=DIRECTION('ref_axis',(-6.40836823623517E-14,-0.707106781186516,
-0.707106781186579)) ;
#119411=DIRECTION('center_axis',(0.577350269189625,0.577350269189625,-0.577350269189628)) ;
#119412=DIRECTION('ref_axis',(-0.707106781186552,5.19478420936363E-15,-0.707106781186543)) ;
#119413=DIRECTION('center_axis',(-0.577350269189625,-0.577350269189625,
0.577350269189628)) ;
#119414=DIRECTION('ref_axis',(-0.707106781186566,3.31891725521342E-14,-0.707106781186529)) ;
#119415=DIRECTION('center_axis',(-0.577350269189652,-0.577350269189606,
0.57735026918962)) ;
#119416=DIRECTION('ref_axis',(0.707106781186528,-3.96520952299298E-16,0.707106781186567)) ;
#119417=DIRECTION('center_axis',(0.,0.,-1.)) ;
#119418=DIRECTION('ref_axis',(-1.,0.,0.)) ;
#119419=DIRECTION('center_axis',(0.,0.,1.)) ;
#119420=DIRECTION('ref_axis',(-1.,-8.67361737988404E-15,0.)) ;
#119421=DIRECTION('center_axis',(0.,0.,-1.)) ;
#119422=DIRECTION('ref_axis',(-1.,0.,0.)) ;
#119423=DIRECTION('center_axis',(2.08166817117218E-16,1.,0.)) ;
#119424=DIRECTION('ref_axis',(1.,0.,0.)) ;
#119425=DIRECTION('center_axis',(-1.,0.,-1.66745659064321E-14)) ;
#119426=DIRECTION('ref_axis',(1.66745659064321E-14,2.60208521396523E-14,
-1.)) ;
#119427=DIRECTION('center_axis',(-3.46944695195361E-14,-3.4694469519536E-14,
1.)) ;
#119428=DIRECTION('ref_axis',(-1.,-1.68611237719883E-42,-3.46944695195361E-14)) ;
#119429=DIRECTION('center_axis',(-0.577350269189625,-0.577350269189625,
-0.577350269189628)) ;
#119430=DIRECTION('ref_axis',(-0.707106781186552,5.19478420936363E-15,0.707106781186543)) ;
#119431=DIRECTION('center_axis',(-0.577350269189625,-0.577350269189625,
-0.577350269189628)) ;
#119432=DIRECTION('ref_axis',(-0.707106781186552,5.1349792556416E-15,0.707106781186543)) ;
#119433=DIRECTION('center_axis',(-0.577350269189626,-0.577350269189626,
-0.577350269189626)) ;
#119434=DIRECTION('ref_axis',(0.707106781186547,-0.707106781186548,6.36902276417946E-16)) ;
#119435=DIRECTION('center_axis',(0.,0.,-1.)) ;
#119436=DIRECTION('ref_axis',(-1.,0.,0.)) ;
#119437=DIRECTION('center_axis',(0.,0.,1.)) ;
#119438=DIRECTION('ref_axis',(1.,0.,0.)) ;
#119439=DIRECTION('center_axis',(-1.,0.,9.8563833862319E-18)) ;
#119440=DIRECTION('ref_axis',(9.8563833862319E-18,0.,1.)) ;
#119441=DIRECTION('center_axis',(-1.,8.87690528722497E-15,-8.87690528722518E-15)) ;
#119442=DIRECTION('ref_axis',(-8.87690528722518E-15,4.48415508583942E-43,
1.)) ;
#119443=DIRECTION('center_axis',(2.08166817117218E-16,1.,0.)) ;
#119444=DIRECTION('ref_axis',(1.,0.,0.)) ;
#119445=DIRECTION('center_axis',(-1.,8.53809210832325E-15,8.53809210832346E-15)) ;
#119446=DIRECTION('ref_axis',(-8.53809210832339E-15,8.67361737988409E-15,
-1.)) ;
#119447=DIRECTION('center_axis',(2.08166817117218E-16,1.,0.)) ;
#119448=DIRECTION('ref_axis',(1.,0.,0.)) ;
#119449=DIRECTION('center_axis',(-0.577350269189622,0.577350269189621,-0.577350269189634)) ;
#119450=DIRECTION('ref_axis',(0.707106781186563,1.66970714627838E-14,-0.707106781186532)) ;
#119451=DIRECTION('center_axis',(0.,0.,1.)) ;
#119452=DIRECTION('ref_axis',(-1.,0.,0.)) ;
#119453=DIRECTION('center_axis',(-1.,0.,-9.8563833862319E-18)) ;
#119454=DIRECTION('ref_axis',(-9.8563833862319E-18,0.,1.)) ;
#119455=DIRECTION('center_axis',(-1.,0.,-1.34163173959798E-15)) ;
#119456=DIRECTION('ref_axis',(-1.34163173959798E-15,0.,1.)) ;
#119457=DIRECTION('center_axis',(0.,0.,-1.)) ;
#119458=DIRECTION('ref_axis',(-1.,0.,0.)) ;
#119459=DIRECTION('center_axis',(-3.46944695195361E-14,3.4694469519536E-14,
1.)) ;
#119460=DIRECTION('ref_axis',(1.,-1.68611237719883E-42,3.46944695195361E-14)) ;
#119461=DIRECTION('center_axis',(0.577350269189625,-0.577350269189625,0.577350269189628)) ;
#119462=DIRECTION('ref_axis',(0.707106781186552,5.19478420936363E-15,-0.707106781186543)) ;
#119463=DIRECTION('center_axis',(0.577350269189625,-0.577350269189625,0.577350269189628)) ;
#119464=DIRECTION('ref_axis',(0.707106781186552,5.1349792556416E-15,-0.707106781186543)) ;
#119465=DIRECTION('center_axis',(2.08166817117218E-16,1.,0.)) ;
#119466=DIRECTION('ref_axis',(1.,0.,0.)) ;
#119467=DIRECTION('center_axis',(-0.577350269189646,0.577350269189609,0.577350269189623)) ;
#119468=DIRECTION('ref_axis',(-0.707106781186529,8.66006384940495E-15,-0.707106781186566)) ;
#119469=DIRECTION('center_axis',(0.,0.,-1.)) ;
#119470=DIRECTION('ref_axis',(-1.,0.,0.)) ;
#119471=DIRECTION('center_axis',(0.,0.,1.)) ;
#119472=DIRECTION('ref_axis',(-1.,0.,0.)) ;
#119473=DIRECTION('center_axis',(0.,0.,-1.)) ;
#119474=DIRECTION('ref_axis',(-1.,0.,0.)) ;
#119475=DIRECTION('center_axis',(-0.577350269189625,0.577350269189625,0.577350269189628)) ;
#119476=DIRECTION('ref_axis',(0.707106781186552,5.1349792556416E-15,0.707106781186543)) ;
#119477=DIRECTION('center_axis',(0.577350269189625,-0.577350269189625,-0.577350269189628)) ;
#119478=DIRECTION('ref_axis',(0.707106781186559,1.92955635991398E-14,0.707106781186536)) ;
#119479=DIRECTION('center_axis',(-0.577350269189625,0.577350269189626,-0.577350269189626)) ;
#119480=DIRECTION('ref_axis',(5.20172641667636E-15,0.70710678118655,0.707106781186545)) ;
#119481=DIRECTION('center_axis',(0.577350269189625,-0.577350269189626,0.577350269189626)) ;
#119482=DIRECTION('ref_axis',(1.27903606950626E-14,0.707106781186554,0.707106781186541)) ;
#119483=DIRECTION('center_axis',(0.577350269189636,-0.577350269189592,0.57735026918965)) ;
#119484=DIRECTION('ref_axis',(0.707106781186558,3.40611850366138E-15,-0.707106781186537)) ;
#119485=DIRECTION('center_axis',(0.,0.,-1.)) ;
#119486=DIRECTION('ref_axis',(-1.,0.,0.)) ;
#119487=DIRECTION('center_axis',(0.,0.,1.)) ;
#119488=DIRECTION('ref_axis',(-1.,1.57209315010398E-14,0.)) ;
#119489=DIRECTION('center_axis',(0.,0.,-1.)) ;
#119490=DIRECTION('ref_axis',(-1.,0.,0.)) ;
#119491=DIRECTION('center_axis',(0.,1.,0.)) ;
#119492=DIRECTION('ref_axis',(1.,0.,0.)) ;
#119493=DIRECTION('center_axis',(0.,-1.,7.76229792195976E-15)) ;
#119494=DIRECTION('ref_axis',(3.46944695195364E-14,7.76229792195976E-15,
1.)) ;
#119495=DIRECTION('center_axis',(-3.46944695195361E-14,3.46944695195361E-14,
1.)) ;
#119496=DIRECTION('ref_axis',(-7.17464813734306E-43,1.,-3.46944695195361E-14)) ;
#119497=DIRECTION('center_axis',(0.577350269189625,-0.577350269189626,-0.577350269189626)) ;
#119498=DIRECTION('ref_axis',(5.20172641667636E-15,0.70710678118655,-0.707106781186545)) ;
#119499=DIRECTION('center_axis',(0.577350269189625,-0.577350269189626,-0.577350269189626)) ;
#119500=DIRECTION('ref_axis',(5.11416588733871E-15,0.70710678118655,-0.707106781186545)) ;
#119501=DIRECTION('center_axis',(0.577350269189624,-0.577350269189625,-0.577350269189629)) ;
#119502=DIRECTION('ref_axis',(4.29556475679742E-15,0.707106781186552,-0.707106781186543)) ;
#119503=DIRECTION('center_axis',(0.,0.,-1.)) ;
#119504=DIRECTION('ref_axis',(-1.,0.,0.)) ;
#119505=DIRECTION('center_axis',(0.,0.,1.)) ;
#119506=DIRECTION('ref_axis',(1.,0.,0.)) ;
#119507=DIRECTION('center_axis',(0.,1.,1.95511867169518E-16)) ;
#119508=DIRECTION('ref_axis',(0.,-1.95511867169518E-16,1.)) ;
#119509=DIRECTION('center_axis',(-7.65717784317885E-15,-1.,-7.84883952026447E-15)) ;
#119510=DIRECTION('ref_axis',(-8.90241127119925E-32,7.84883952026447E-15,
-1.)) ;
#119511=DIRECTION('center_axis',(0.,1.,0.)) ;
#119512=DIRECTION('ref_axis',(1.,0.,0.)) ;
#119513=DIRECTION('center_axis',(-1.28749007982652E-15,-1.,1.47915175691198E-15)) ;
#119514=DIRECTION('ref_axis',(3.46944695195364E-14,1.47915175691194E-15,
1.)) ;
#119515=DIRECTION('center_axis',(0.,1.,0.)) ;
#119516=DIRECTION('ref_axis',(1.,0.,0.)) ;
#119517=DIRECTION('center_axis',(-0.577350269189619,-0.577350269189621,
-0.577350269189638)) ;
#119518=DIRECTION('ref_axis',(1.66660234080318E-14,-0.707106781186566,0.707106781186529)) ;
#119519=DIRECTION('center_axis',(0.,0.,1.)) ;
#119520=DIRECTION('ref_axis',(-1.,-3.52365706057788E-15,0.)) ;
#119521=DIRECTION('center_axis',(0.,1.,-1.95511867169518E-16)) ;
#119522=DIRECTION('ref_axis',(0.,1.95511867169518E-16,1.)) ;
#119523=DIRECTION('center_axis',(0.,-1.,3.06658683336682E-15)) ;
#119524=DIRECTION('ref_axis',(0.,-3.06658683336682E-15,-1.)) ;
#119525=DIRECTION('center_axis',(0.,0.,-1.)) ;
#119526=DIRECTION('ref_axis',(-1.,0.,0.)) ;
#119527=DIRECTION('center_axis',(-3.4694469519536E-14,-3.46944695195361E-14,
1.)) ;
#119528=DIRECTION('ref_axis',(-8.96831017167883E-43,-1.,-3.46944695195361E-14)) ;
#119529=DIRECTION('center_axis',(0.577350269189625,0.577350269189626,0.577350269189627)) ;
#119530=DIRECTION('ref_axis',(5.35231302451417E-15,-0.707106781186551,0.707106781186544)) ;
#119531=DIRECTION('center_axis',(0.577350269189625,0.577350269189626,0.577350269189627)) ;
#119532=DIRECTION('ref_axis',(5.35231302451417E-15,-0.707106781186551,0.707106781186544)) ;
#119533=DIRECTION('center_axis',(0.,1.,0.)) ;
#119534=DIRECTION('ref_axis',(1.,0.,0.)) ;
#119535=DIRECTION('center_axis',(-0.577350269189609,-0.577350269189646,
0.577350269189623)) ;
#119536=DIRECTION('ref_axis',(8.91337114590872E-15,0.707106781186529,0.707106781186566)) ;
#119537=DIRECTION('center_axis',(0.,0.,-1.)) ;
#119538=DIRECTION('ref_axis',(-1.,0.,0.)) ;
#119539=DIRECTION('center_axis',(0.,0.,1.)) ;
#119540=DIRECTION('ref_axis',(-1.,1.0842021724855E-15,0.)) ;
#119541=DIRECTION('center_axis',(0.,0.,-1.)) ;
#119542=DIRECTION('ref_axis',(-1.,0.,0.)) ;
#119543=DIRECTION('center_axis',(-0.577350269189625,-0.577350269189626,
0.577350269189627)) ;
#119544=DIRECTION('ref_axis',(5.35231302451417E-15,-0.707106781186551,-0.707106781186544)) ;
#119545=DIRECTION('center_axis',(0.577350269189625,0.577350269189626,-0.577350269189627)) ;
#119546=DIRECTION('ref_axis',(-6.40836823623517E-14,-0.707106781186516,
-0.707106781186579)) ;
#119547=DIRECTION('center_axis',(0.577350269189625,0.577350269189625,-0.577350269189628)) ;
#119548=DIRECTION('ref_axis',(-0.707106781186552,5.19478420936363E-15,-0.707106781186543)) ;
#119549=DIRECTION('center_axis',(-0.577350269189625,-0.577350269189625,
0.577350269189628)) ;
#119550=DIRECTION('ref_axis',(-0.707106781186562,2.56048320762387E-14,-0.707106781186533)) ;
#119551=DIRECTION('center_axis',(-0.577350269189542,-0.577350269189661,
0.577350269189675)) ;
#119552=DIRECTION('ref_axis',(3.44881489367205E-15,-0.707106781186558,-0.707106781186537)) ;
#119553=DIRECTION('center_axis',(0.,0.,-1.)) ;
#119554=DIRECTION('ref_axis',(-1.,0.,0.)) ;
#119555=DIRECTION('center_axis',(0.,0.,1.)) ;
#119556=DIRECTION('ref_axis',(-1.,-8.67361737988404E-15,0.)) ;
#119557=DIRECTION('center_axis',(0.,0.,-1.)) ;
#119558=DIRECTION('ref_axis',(-1.,0.,0.)) ;
#119559=DIRECTION('center_axis',(2.08166817117218E-16,1.,0.)) ;
#119560=DIRECTION('ref_axis',(1.,0.,0.)) ;
#119561=DIRECTION('center_axis',(-1.,0.,9.05601424228639E-14)) ;
#119562=DIRECTION('ref_axis',(-9.05601424228639E-14,0.,-1.)) ;
#119563=DIRECTION('center_axis',(6.93889390390722E-14,6.93889390390721E-14,
1.)) ;
#119564=DIRECTION('ref_axis',(-1.,-6.3534872372487E-42,6.93889390390722E-14)) ;
#119565=DIRECTION('center_axis',(-0.577350269189625,-0.577350269189625,
-0.577350269189628)) ;
#119566=DIRECTION('ref_axis',(-0.707106781186552,5.19478420936363E-15,0.707106781186543)) ;
#119567=DIRECTION('center_axis',(-0.577350269189625,-0.577350269189625,
-0.577350269189628)) ;
#119568=DIRECTION('ref_axis',(-0.707106781186552,5.1349792556416E-15,0.707106781186543)) ;
#119569=DIRECTION('center_axis',(-0.577350269189609,-0.577350269189608,
-0.57735026918966)) ;
#119570=DIRECTION('ref_axis',(-0.707106781186576,-5.08171669240118E-15,
0.707106781186519)) ;
#119571=DIRECTION('center_axis',(0.,0.,-1.)) ;
#119572=DIRECTION('ref_axis',(-1.,0.,0.)) ;
#119573=DIRECTION('center_axis',(0.,0.,1.)) ;
#119574=DIRECTION('ref_axis',(1.,0.,0.)) ;
#119575=DIRECTION('center_axis',(-1.,0.,9.8563833862319E-18)) ;
#119576=DIRECTION('ref_axis',(9.8563833862319E-18,0.,1.)) ;
#119577=DIRECTION('center_axis',(-1.,1.31459513413869E-14,-1.31459513413873E-14)) ;
#119578=DIRECTION('ref_axis',(-1.31459513413873E-14,1.17484863248993E-41,
1.)) ;
#119579=DIRECTION('center_axis',(2.08166817117218E-16,1.,0.)) ;
#119580=DIRECTION('ref_axis',(1.,0.,0.)) ;
#119581=DIRECTION('center_axis',(-1.,-1.77538105744504E-14,-1.77538105744508E-14)) ;
#119582=DIRECTION('ref_axis',(1.77538105744506E-14,8.67361737988379E-15,
-1.)) ;
#119583=DIRECTION('center_axis',(2.08166817117218E-16,1.,0.)) ;
#119584=DIRECTION('ref_axis',(1.,0.,0.)) ;
#119585=DIRECTION('center_axis',(-0.577350269189595,0.577350269189594,-0.577350269189688)) ;
#119586=DIRECTION('ref_axis',(0.707106781186627,4.55186387217293E-14,-0.707106781186468)) ;
#119587=DIRECTION('center_axis',(-9.81307786677359E-14,0.,1.)) ;
#119588=DIRECTION('ref_axis',(-1.,0.,-9.81307786677359E-14)) ;
#119589=DIRECTION('center_axis',(-1.,0.,-9.8563833862319E-18)) ;
#119590=DIRECTION('ref_axis',(-9.8563833862319E-18,0.,1.)) ;
#119591=DIRECTION('center_axis',(-1.,0.,8.71102322353262E-14)) ;
#119592=DIRECTION('ref_axis',(8.71102322353262E-14,0.,1.)) ;
#119593=DIRECTION('center_axis',(0.,0.,-1.)) ;
#119594=DIRECTION('ref_axis',(-1.,0.,0.)) ;
#119595=DIRECTION('center_axis',(6.93889390390722E-14,-6.93889390390721E-14,
1.)) ;
#119596=DIRECTION('ref_axis',(1.,-6.3534872372487E-42,-6.93889390390722E-14)) ;
#119597=DIRECTION('center_axis',(0.577350269189625,-0.577350269189625,0.577350269189628)) ;
#119598=DIRECTION('ref_axis',(0.707106781186552,5.19478420936363E-15,-0.707106781186543)) ;
#119599=DIRECTION('center_axis',(0.577350269189625,-0.577350269189625,0.577350269189628)) ;
#119600=DIRECTION('ref_axis',(0.707106781186552,5.1349792556416E-15,-0.707106781186543)) ;
#119601=DIRECTION('center_axis',(2.08166817117218E-16,1.,0.)) ;
#119602=DIRECTION('ref_axis',(1.,0.,0.)) ;
#119603=DIRECTION('center_axis',(-0.577350269189538,0.577350269189662,0.577350269189676)) ;
#119604=DIRECTION('ref_axis',(1.74300544639431E-14,0.707106781186565,-0.70710678118653)) ;
#119605=DIRECTION('center_axis',(0.,0.,-1.)) ;
#119606=DIRECTION('ref_axis',(-1.,0.,0.)) ;
#119607=DIRECTION('center_axis',(0.,0.,1.)) ;
#119608=DIRECTION('ref_axis',(-1.,0.,0.)) ;
#119609=DIRECTION('center_axis',(0.,0.,-1.)) ;
#119610=DIRECTION('ref_axis',(-1.,0.,0.)) ;
#119611=DIRECTION('center_axis',(-0.577350269189625,0.577350269189625,0.577350269189628)) ;
#119612=DIRECTION('ref_axis',(0.707106781186552,5.1349792556416E-15,0.707106781186543)) ;
#119613=DIRECTION('center_axis',(0.577350269189625,-0.577350269189625,-0.577350269189628)) ;
#119614=DIRECTION('ref_axis',(0.707106781186562,2.5899563042358E-14,0.707106781186533)) ;
#119615=DIRECTION('center_axis',(-0.577350269189625,0.577350269189626,-0.577350269189626)) ;
#119616=DIRECTION('ref_axis',(5.20172641667636E-15,0.70710678118655,0.707106781186545)) ;
#119617=DIRECTION('center_axis',(0.577350269189625,-0.577350269189626,0.577350269189626)) ;
#119618=DIRECTION('ref_axis',(4.10196750502305E-14,0.707106781186568,0.707106781186527)) ;
#119619=DIRECTION('center_axis',(0.577350269189612,-0.57735026918964,0.577350269189626)) ;
#119620=DIRECTION('ref_axis',(-8.27428663398926E-15,-0.707106781186543,
-0.707106781186552)) ;
#119621=DIRECTION('center_axis',(0.,0.,-1.)) ;
#119622=DIRECTION('ref_axis',(-1.,0.,0.)) ;
#119623=DIRECTION('center_axis',(0.,0.,1.)) ;
#119624=DIRECTION('ref_axis',(-1.,1.35525271560688E-14,0.)) ;
#119625=DIRECTION('center_axis',(0.,0.,-1.)) ;
#119626=DIRECTION('ref_axis',(-1.,0.,0.)) ;
#119627=DIRECTION('center_axis',(0.,1.,0.)) ;
#119628=DIRECTION('ref_axis',(1.,0.,0.)) ;
#119629=DIRECTION('center_axis',(0.,-1.,1.13080389480401E-14)) ;
#119630=DIRECTION('ref_axis',(1.12757025938489E-13,1.13080389480401E-14,
1.)) ;
#119631=DIRECTION('center_axis',(0.,0.,1.)) ;
#119632=DIRECTION('ref_axis',(-1.,0.,0.)) ;
#119633=DIRECTION('center_axis',(0.577350269189625,-0.577350269189626,-0.577350269189626)) ;
#119634=DIRECTION('ref_axis',(5.20172641667636E-15,0.70710678118655,-0.707106781186545)) ;
#119635=DIRECTION('center_axis',(0.577350269189625,-0.577350269189626,-0.577350269189626)) ;
#119636=DIRECTION('ref_axis',(5.11416588733871E-15,0.70710678118655,-0.707106781186545)) ;
#119637=DIRECTION('center_axis',(0.577350269189618,-0.577350269189619,-0.57735026918964)) ;
#119638=DIRECTION('ref_axis',(1.15945863464918E-15,0.707106781186561,-0.707106781186534)) ;
#119639=DIRECTION('center_axis',(0.,0.,-1.)) ;
#119640=DIRECTION('ref_axis',(-1.,0.,0.)) ;
#119641=DIRECTION('center_axis',(0.,0.,1.)) ;
#119642=DIRECTION('ref_axis',(1.,0.,0.)) ;
#119643=DIRECTION('center_axis',(0.,1.,1.95511867169518E-16)) ;
#119644=DIRECTION('ref_axis',(0.,-1.95511867169518E-16,1.)) ;
#119645=DIRECTION('center_axis',(4.26226979058352E-14,-1.,4.24310362287508E-14)) ;
#119646=DIRECTION('ref_axis',(1.,4.26226979058352E-14,4.69939452995971E-41)) ;
#119647=DIRECTION('center_axis',(0.,1.,0.)) ;
#119648=DIRECTION('ref_axis',(1.,0.,0.)) ;
#119649=DIRECTION('center_axis',(-1.00288700954911E-14,-1.,1.02205317725767E-14)) ;
#119650=DIRECTION('ref_axis',(3.46944695195352E-14,1.02205317725764E-14,
1.)) ;
#119651=DIRECTION('center_axis',(0.,1.,0.)) ;
#119652=DIRECTION('ref_axis',(1.,0.,0.)) ;
#119653=DIRECTION('center_axis',(-0.577350269189659,-0.57735026918966,-0.577350269189558)) ;
#119654=DIRECTION('ref_axis',(-0.707106781186543,0.707106781186552,-1.03102727271032E-14)) ;
#119655=DIRECTION('center_axis',(0.,9.8130778667736E-14,1.)) ;
#119656=DIRECTION('ref_axis',(-8.67361737988403E-15,1.,-9.8130778667736E-14)) ;
#119657=DIRECTION('center_axis',(0.,1.,-1.95511867169518E-16)) ;
#119658=DIRECTION('ref_axis',(0.,1.95511867169518E-16,1.)) ;
#119659=DIRECTION('center_axis',(0.,-1.,9.83224403448236E-14)) ;
#119660=DIRECTION('ref_axis',(0.,-9.83224403448236E-14,-1.)) ;
#119661=DIRECTION('center_axis',(0.,0.,-1.)) ;
#119662=DIRECTION('ref_axis',(-1.,0.,0.)) ;
#119663=DIRECTION('center_axis',(0.,0.,1.)) ;
#119664=DIRECTION('ref_axis',(1.,0.,0.)) ;
#119665=DIRECTION('center_axis',(0.577350269189625,0.577350269189626,0.577350269189627)) ;
#119666=DIRECTION('ref_axis',(5.35231302451417E-15,-0.707106781186551,0.707106781186544)) ;
#119667=DIRECTION('center_axis',(0.577350269189625,0.577350269189626,0.577350269189627)) ;
#119668=DIRECTION('ref_axis',(5.35231302451417E-15,-0.707106781186551,0.707106781186544)) ;
#119669=DIRECTION('center_axis',(0.,1.,0.)) ;
#119670=DIRECTION('ref_axis',(1.,0.,0.)) ;
#119671=DIRECTION('center_axis',(-0.57735026918964,-0.577350269189583,0.577350269189654)) ;
#119672=DIRECTION('ref_axis',(-0.707106781186567,2.1970613508967E-14,-0.707106781186528)) ;
#119673=DIRECTION('center_axis',(0.,0.,-1.)) ;
#119674=DIRECTION('ref_axis',(-1.,0.,0.)) ;
#119675=DIRECTION('center_axis',(0.,0.,1.)) ;
#119676=DIRECTION('ref_axis',(-1.,1.0842021724855E-15,0.)) ;
#119677=DIRECTION('center_axis',(0.,0.,-1.)) ;
#119678=DIRECTION('ref_axis',(-1.,0.,0.)) ;
#119679=DIRECTION('center_axis',(-0.577350269189625,-0.577350269189626,
0.577350269189627)) ;
#119680=DIRECTION('ref_axis',(5.35231302451417E-15,-0.707106781186551,-0.707106781186544)) ;
#119681=DIRECTION('center_axis',(0.577350269189625,0.577350269189626,-0.577350269189627)) ;
#119682=DIRECTION('ref_axis',(4.8009187113684E-14,-0.707106781186572,-0.707106781186523)) ;
#119683=DIRECTION('center_axis',(0.,0.,1.)) ;
#119684=DIRECTION('ref_axis',(1.,0.,0.)) ;
#119685=DIRECTION('center_axis',(0.,-1.,0.)) ;
#119686=DIRECTION('ref_axis',(0.,0.,-1.)) ;
#119687=DIRECTION('center_axis',(9.85638338623186E-18,1.,0.)) ;
#119688=DIRECTION('ref_axis',(-1.,9.85638338623186E-18,0.)) ;
#119689=DIRECTION('center_axis',(0.,-1.,0.)) ;
#119690=DIRECTION('ref_axis',(0.,0.,-1.)) ;
#119691=DIRECTION('center_axis',(0.,1.,0.)) ;
#119692=DIRECTION('ref_axis',(1.,0.,0.)) ;
#119693=DIRECTION('center_axis',(-1.,-7.66646708341686E-16,0.)) ;
#119694=DIRECTION('ref_axis',(7.66646708341686E-16,-1.,0.)) ;
#119695=DIRECTION('center_axis',(1.,-9.85638338623186E-18,0.)) ;
#119696=DIRECTION('ref_axis',(9.85638338623186E-18,1.,0.)) ;
#119697=DIRECTION('center_axis',(-1.,0.,0.)) ;
#119698=DIRECTION('ref_axis',(0.,0.,1.)) ;
#119699=DIRECTION('center_axis',(0.,1.,0.)) ;
#119700=DIRECTION('ref_axis',(1.,0.,0.)) ;
#119701=DIRECTION('center_axis',(0.,1.,0.)) ;
#119702=DIRECTION('ref_axis',(0.,0.,1.)) ;
#119703=DIRECTION('center_axis',(-9.85638338623186E-18,-1.,0.)) ;
#119704=DIRECTION('ref_axis',(1.,-9.85638338623186E-18,0.)) ;
#119705=DIRECTION('center_axis',(0.,1.,0.)) ;
#119706=DIRECTION('ref_axis',(0.,0.,1.)) ;
#119707=DIRECTION('center_axis',(0.,0.,1.)) ;
#119708=DIRECTION('ref_axis',(1.,0.,0.)) ;
#119709=DIRECTION('center_axis',(0.,0.,1.)) ;
#119710=DIRECTION('ref_axis',(1.,0.,0.)) ;
#119711=DIRECTION('center_axis',(0.,-1.,0.)) ;
#119712=DIRECTION('ref_axis',(0.,0.,-1.)) ;
#119713=DIRECTION('center_axis',(-9.85638338623186E-18,-1.,0.)) ;
#119714=DIRECTION('ref_axis',(1.,-9.85638338623186E-18,0.)) ;
#119715=DIRECTION('center_axis',(0.,-1.,0.)) ;
#119716=DIRECTION('ref_axis',(0.,0.,-1.)) ;
#119717=DIRECTION('center_axis',(0.,1.,0.)) ;
#119718=DIRECTION('ref_axis',(1.,0.,0.)) ;
#119719=DIRECTION('center_axis',(1.,-3.06658683336674E-15,0.)) ;
#119720=DIRECTION('ref_axis',(3.06658683336674E-15,1.,0.)) ;
#119721=DIRECTION('center_axis',(1.,-9.85638338623186E-18,0.)) ;
#119722=DIRECTION('ref_axis',(9.85638338623186E-18,1.,0.)) ;
#119723=DIRECTION('center_axis',(1.,0.,0.)) ;
#119724=DIRECTION('ref_axis',(0.,0.,-1.)) ;
#119725=DIRECTION('center_axis',(0.,1.,0.)) ;
#119726=DIRECTION('ref_axis',(1.,0.,0.)) ;
#119727=DIRECTION('center_axis',(0.,1.,0.)) ;
#119728=DIRECTION('ref_axis',(0.,0.,1.)) ;
#119729=DIRECTION('center_axis',(-9.85638338623186E-18,-1.,0.)) ;
#119730=DIRECTION('ref_axis',(1.,-9.85638338623186E-18,0.)) ;
#119731=DIRECTION('center_axis',(0.,1.,0.)) ;
#119732=DIRECTION('ref_axis',(0.,0.,1.)) ;
#119733=DIRECTION('center_axis',(0.,0.,1.)) ;
#119734=DIRECTION('ref_axis',(1.,0.,0.)) ;
#119735=DIRECTION('center_axis',(-1.,-1.95511867169517E-16,0.)) ;
#119736=DIRECTION('ref_axis',(1.95511867169517E-16,-1.,0.)) ;
#119737=DIRECTION('center_axis',(1.,0.,0.)) ;
#119738=DIRECTION('ref_axis',(0.,0.,-1.)) ;
#119739=DIRECTION('center_axis',(0.,1.,0.)) ;
#119740=DIRECTION('ref_axis',(1.,0.,0.)) ;
#119741=DIRECTION('center_axis',(7.66646708341686E-16,-1.,0.)) ;
#119742=DIRECTION('ref_axis',(1.,7.66646708341686E-16,0.)) ;
#119743=DIRECTION('center_axis',(-1.95511867169517E-16,1.,0.)) ;
#119744=DIRECTION('ref_axis',(-1.,-1.95511867169517E-16,0.)) ;
#119745=DIRECTION('center_axis',(0.,-1.,0.)) ;
#119746=DIRECTION('ref_axis',(0.,0.,-1.)) ;
#119747=DIRECTION('center_axis',(0.,1.,0.)) ;
#119748=DIRECTION('ref_axis',(1.,0.,0.)) ;
#119749=DIRECTION('center_axis',(-1.,0.,0.)) ;
#119750=DIRECTION('ref_axis',(0.,0.,1.)) ;
#119751=DIRECTION('center_axis',(1.,-1.06642836637918E-16,0.)) ;
#119752=DIRECTION('ref_axis',(1.06642836637918E-16,1.,0.)) ;
#119753=DIRECTION('center_axis',(1.,1.95511867169517E-16,0.)) ;
#119754=DIRECTION('ref_axis',(-1.95511867169517E-16,1.,0.)) ;
#119755=DIRECTION('center_axis',(1.,0.,0.)) ;
#119756=DIRECTION('ref_axis',(0.,0.,-1.)) ;
#119757=DIRECTION('center_axis',(0.,1.,0.)) ;
#119758=DIRECTION('ref_axis',(1.,0.,0.)) ;
#119759=DIRECTION('center_axis',(2.29994012502506E-15,-1.,0.)) ;
#119760=DIRECTION('ref_axis',(1.,2.29994012502506E-15,0.)) ;
#119761=DIRECTION('center_axis',(-1.95511867169517E-16,1.,0.)) ;
#119762=DIRECTION('ref_axis',(-1.,-1.95511867169517E-16,0.)) ;
#119763=DIRECTION('center_axis',(0.,-1.,0.)) ;
#119764=DIRECTION('ref_axis',(0.,0.,-1.)) ;
#119765=DIRECTION('center_axis',(-1.,1.06642836637918E-16,0.)) ;
#119766=DIRECTION('ref_axis',(-1.06642836637918E-16,-1.,0.)) ;
#119767=DIRECTION('center_axis',(1.,0.,0.)) ;
#119768=DIRECTION('ref_axis',(0.,0.,-1.)) ;
#119769=DIRECTION('center_axis',(0.,1.,0.)) ;
#119770=DIRECTION('ref_axis',(1.,0.,0.)) ;
#119771=DIRECTION('center_axis',(0.,0.,1.)) ;
#119772=DIRECTION('ref_axis',(1.,0.,0.)) ;
#119773=DIRECTION('center_axis',(0.,-1.,0.)) ;
#119774=DIRECTION('ref_axis',(0.,0.,-1.)) ;
#119775=DIRECTION('center_axis',(9.85638338623186E-18,1.,0.)) ;
#119776=DIRECTION('ref_axis',(-1.,9.85638338623186E-18,0.)) ;
#119777=DIRECTION('center_axis',(0.,-1.,0.)) ;
#119778=DIRECTION('ref_axis',(0.,0.,-1.)) ;
#119779=DIRECTION('center_axis',(0.,1.,0.)) ;
#119780=DIRECTION('ref_axis',(1.,0.,0.)) ;
#119781=DIRECTION('center_axis',(-1.,-1.14997006251252E-14,0.)) ;
#119782=DIRECTION('ref_axis',(1.14997006251252E-14,-1.,0.)) ;
#119783=DIRECTION('center_axis',(1.,-9.85638338623186E-18,0.)) ;
#119784=DIRECTION('ref_axis',(9.85638338623186E-18,1.,0.)) ;
#119785=DIRECTION('center_axis',(-1.,0.,0.)) ;
#119786=DIRECTION('ref_axis',(0.,0.,1.)) ;
#119787=DIRECTION('center_axis',(0.,1.,0.)) ;
#119788=DIRECTION('ref_axis',(1.,0.,0.)) ;
#119789=DIRECTION('center_axis',(0.,1.,0.)) ;
#119790=DIRECTION('ref_axis',(0.,0.,1.)) ;
#119791=DIRECTION('center_axis',(-9.85638338623186E-18,-1.,0.)) ;
#119792=DIRECTION('ref_axis',(1.,-9.85638338623186E-18,0.)) ;
#119793=DIRECTION('center_axis',(0.,1.,0.)) ;
#119794=DIRECTION('ref_axis',(0.,0.,1.)) ;
#119795=DIRECTION('center_axis',(0.,0.,1.)) ;
#119796=DIRECTION('ref_axis',(1.,0.,0.)) ;
#119797=DIRECTION('center_axis',(0.,0.,1.)) ;
#119798=DIRECTION('ref_axis',(1.,0.,0.)) ;
#119799=DIRECTION('center_axis',(0.,-1.,0.)) ;
#119800=DIRECTION('ref_axis',(0.,0.,-1.)) ;
#119801=DIRECTION('center_axis',(-9.85638338623186E-18,-1.,0.)) ;
#119802=DIRECTION('ref_axis',(1.,-9.85638338623186E-18,0.)) ;
#119803=DIRECTION('center_axis',(0.,-1.,0.)) ;
#119804=DIRECTION('ref_axis',(0.,0.,-1.)) ;
#119805=DIRECTION('center_axis',(0.,1.,0.)) ;
#119806=DIRECTION('ref_axis',(1.,0.,0.)) ;
#119807=DIRECTION('center_axis',(1.,3.83323354170843E-15,0.)) ;
#119808=DIRECTION('ref_axis',(-3.83323354170843E-15,1.,0.)) ;
#119809=DIRECTION('center_axis',(1.,-9.85638338623186E-18,0.)) ;
#119810=DIRECTION('ref_axis',(9.85638338623186E-18,1.,0.)) ;
#119811=DIRECTION('center_axis',(1.,0.,0.)) ;
#119812=DIRECTION('ref_axis',(0.,0.,-1.)) ;
#119813=DIRECTION('center_axis',(0.,1.,0.)) ;
#119814=DIRECTION('ref_axis',(1.,0.,0.)) ;
#119815=DIRECTION('center_axis',(0.,1.,0.)) ;
#119816=DIRECTION('ref_axis',(0.,0.,1.)) ;
#119817=DIRECTION('center_axis',(-9.85638338623186E-18,-1.,0.)) ;
#119818=DIRECTION('ref_axis',(1.,-9.85638338623186E-18,0.)) ;
#119819=DIRECTION('center_axis',(0.,1.,0.)) ;
#119820=DIRECTION('ref_axis',(0.,0.,1.)) ;
#119821=DIRECTION('center_axis',(0.,0.,1.)) ;
#119822=DIRECTION('ref_axis',(1.,0.,0.)) ;
#119823=DIRECTION('center_axis',(-1.,-1.95511867169517E-16,0.)) ;
#119824=DIRECTION('ref_axis',(1.95511867169517E-16,-1.,0.)) ;
#119825=DIRECTION('center_axis',(1.,0.,0.)) ;
#119826=DIRECTION('ref_axis',(0.,0.,-1.)) ;
#119827=DIRECTION('center_axis',(0.,1.,0.)) ;
#119828=DIRECTION('ref_axis',(1.,0.,0.)) ;
#119829=DIRECTION('center_axis',(4.59988025005012E-15,-1.,0.)) ;
#119830=DIRECTION('ref_axis',(1.,4.59988025005012E-15,0.)) ;
#119831=DIRECTION('center_axis',(-1.95511867169517E-16,1.,0.)) ;
#119832=DIRECTION('ref_axis',(-1.,-1.95511867169517E-16,0.)) ;
#119833=DIRECTION('center_axis',(0.,-1.,0.)) ;
#119834=DIRECTION('ref_axis',(0.,0.,-1.)) ;
#119835=DIRECTION('center_axis',(0.,1.,0.)) ;
#119836=DIRECTION('ref_axis',(1.,0.,0.)) ;
#119837=DIRECTION('center_axis',(-1.,0.,0.)) ;
#119838=DIRECTION('ref_axis',(0.,0.,1.)) ;
#119839=DIRECTION('center_axis',(1.,-1.06642836637918E-16,0.)) ;
#119840=DIRECTION('ref_axis',(1.06642836637918E-16,1.,0.)) ;
#119841=DIRECTION('center_axis',(1.,1.95511867169517E-16,0.)) ;
#119842=DIRECTION('ref_axis',(-1.95511867169517E-16,1.,0.)) ;
#119843=DIRECTION('center_axis',(1.,0.,0.)) ;
#119844=DIRECTION('ref_axis',(0.,0.,-1.)) ;
#119845=DIRECTION('center_axis',(0.,1.,0.)) ;
#119846=DIRECTION('ref_axis',(1.,0.,0.)) ;
#119847=DIRECTION('center_axis',(-1.53329341668337E-15,-1.,0.)) ;
#119848=DIRECTION('ref_axis',(1.,-1.53329341668337E-15,0.)) ;
#119849=DIRECTION('center_axis',(-1.95511867169517E-16,1.,0.)) ;
#119850=DIRECTION('ref_axis',(-1.,-1.95511867169517E-16,0.)) ;
#119851=DIRECTION('center_axis',(0.,-1.,0.)) ;
#119852=DIRECTION('ref_axis',(0.,0.,-1.)) ;
#119853=DIRECTION('center_axis',(-1.,1.06642836637918E-16,0.)) ;
#119854=DIRECTION('ref_axis',(-1.06642836637918E-16,-1.,0.)) ;
#119855=DIRECTION('center_axis',(1.,0.,0.)) ;
#119856=DIRECTION('ref_axis',(0.,0.,-1.)) ;
#119857=DIRECTION('center_axis',(0.,1.,0.)) ;
#119858=DIRECTION('ref_axis',(1.,0.,0.)) ;
#119859=DIRECTION('center_axis',(0.,0.,1.)) ;
#119860=DIRECTION('ref_axis',(1.,0.,0.)) ;
#119861=DIRECTION('center_axis',(0.,-1.,0.)) ;
#119862=DIRECTION('ref_axis',(0.,0.,-1.)) ;
#119863=DIRECTION('center_axis',(9.85638338623186E-18,1.,0.)) ;
#119864=DIRECTION('ref_axis',(-1.,9.85638338623186E-18,0.)) ;
#119865=DIRECTION('center_axis',(0.,-1.,0.)) ;
#119866=DIRECTION('ref_axis',(0.,0.,-1.)) ;
#119867=DIRECTION('center_axis',(0.,1.,0.)) ;
#119868=DIRECTION('ref_axis',(1.,0.,0.)) ;
#119869=DIRECTION('center_axis',(-1.,-2.29994012502506E-15,0.)) ;
#119870=DIRECTION('ref_axis',(2.29994012502506E-15,-1.,0.)) ;
#119871=DIRECTION('center_axis',(1.,-9.85638338623186E-18,0.)) ;
#119872=DIRECTION('ref_axis',(9.85638338623186E-18,1.,0.)) ;
#119873=DIRECTION('center_axis',(-1.,0.,0.)) ;
#119874=DIRECTION('ref_axis',(0.,0.,1.)) ;
#119875=DIRECTION('center_axis',(0.,1.,0.)) ;
#119876=DIRECTION('ref_axis',(1.,0.,0.)) ;
#119877=DIRECTION('center_axis',(0.,1.,0.)) ;
#119878=DIRECTION('ref_axis',(0.,0.,1.)) ;
#119879=DIRECTION('center_axis',(-9.85638338623186E-18,-1.,0.)) ;
#119880=DIRECTION('ref_axis',(1.,-9.85638338623186E-18,0.)) ;
#119881=DIRECTION('center_axis',(0.,1.,0.)) ;
#119882=DIRECTION('ref_axis',(0.,0.,1.)) ;
#119883=DIRECTION('center_axis',(0.,0.,1.)) ;
#119884=DIRECTION('ref_axis',(1.,0.,0.)) ;
#119885=DIRECTION('center_axis',(0.,0.,1.)) ;
#119886=DIRECTION('ref_axis',(1.,0.,0.)) ;
#119887=DIRECTION('center_axis',(0.,-1.,0.)) ;
#119888=DIRECTION('ref_axis',(0.,0.,-1.)) ;
#119889=DIRECTION('center_axis',(-9.85638338623186E-18,-1.,0.)) ;
#119890=DIRECTION('ref_axis',(1.,-9.85638338623186E-18,0.)) ;
#119891=DIRECTION('center_axis',(0.,-1.,0.)) ;
#119892=DIRECTION('ref_axis',(0.,0.,-1.)) ;
#119893=DIRECTION('center_axis',(0.,1.,0.)) ;
#119894=DIRECTION('ref_axis',(1.,0.,0.)) ;
#119895=DIRECTION('center_axis',(1.,-7.66646708341686E-15,0.)) ;
#119896=DIRECTION('ref_axis',(7.66646708341686E-15,1.,0.)) ;
#119897=DIRECTION('center_axis',(1.,-9.85638338623186E-18,0.)) ;
#119898=DIRECTION('ref_axis',(9.85638338623186E-18,1.,0.)) ;
#119899=DIRECTION('center_axis',(1.,0.,0.)) ;
#119900=DIRECTION('ref_axis',(0.,0.,-1.)) ;
#119901=DIRECTION('center_axis',(0.,1.,0.)) ;
#119902=DIRECTION('ref_axis',(1.,0.,0.)) ;
#119903=DIRECTION('center_axis',(0.,1.,0.)) ;
#119904=DIRECTION('ref_axis',(0.,0.,1.)) ;
#119905=DIRECTION('center_axis',(-9.85638338623186E-18,-1.,0.)) ;
#119906=DIRECTION('ref_axis',(1.,-9.85638338623186E-18,0.)) ;
#119907=DIRECTION('center_axis',(0.,1.,0.)) ;
#119908=DIRECTION('ref_axis',(0.,0.,1.)) ;
#119909=DIRECTION('center_axis',(0.,0.,1.)) ;
#119910=DIRECTION('ref_axis',(1.,0.,0.)) ;
#119911=DIRECTION('center_axis',(-1.,-1.95511867169517E-16,0.)) ;
#119912=DIRECTION('ref_axis',(1.95511867169517E-16,-1.,0.)) ;
#119913=DIRECTION('center_axis',(1.,0.,0.)) ;
#119914=DIRECTION('ref_axis',(0.,0.,-1.)) ;
#119915=DIRECTION('center_axis',(0.,1.,0.)) ;
#119916=DIRECTION('ref_axis',(1.,0.,0.)) ;
#119917=DIRECTION('center_axis',(9.9664072084418E-15,-1.,0.)) ;
#119918=DIRECTION('ref_axis',(1.,9.9664072084418E-15,0.)) ;
#119919=DIRECTION('center_axis',(-1.95511867169517E-16,1.,0.)) ;
#119920=DIRECTION('ref_axis',(-1.,-1.95511867169517E-16,0.)) ;
#119921=DIRECTION('center_axis',(0.,-1.,0.)) ;
#119922=DIRECTION('ref_axis',(0.,0.,-1.)) ;
#119923=DIRECTION('center_axis',(0.,1.,0.)) ;
#119924=DIRECTION('ref_axis',(1.,0.,0.)) ;
#119925=DIRECTION('center_axis',(-1.,0.,0.)) ;
#119926=DIRECTION('ref_axis',(0.,0.,1.)) ;
#119927=DIRECTION('center_axis',(1.,-1.06642836637918E-16,0.)) ;
#119928=DIRECTION('ref_axis',(1.06642836637918E-16,1.,0.)) ;
#119929=DIRECTION('center_axis',(1.,1.95511867169517E-16,0.)) ;
#119930=DIRECTION('ref_axis',(-1.95511867169517E-16,1.,0.)) ;
#119931=DIRECTION('center_axis',(1.,0.,0.)) ;
#119932=DIRECTION('ref_axis',(0.,0.,-1.)) ;
#119933=DIRECTION('center_axis',(0.,1.,0.)) ;
#119934=DIRECTION('ref_axis',(1.,0.,0.)) ;
#119935=DIRECTION('center_axis',(6.89982037507517E-15,-1.,0.)) ;
#119936=DIRECTION('ref_axis',(1.,6.89982037507517E-15,0.)) ;
#119937=DIRECTION('center_axis',(-1.95511867169517E-16,1.,0.)) ;
#119938=DIRECTION('ref_axis',(-1.,-1.95511867169517E-16,0.)) ;
#119939=DIRECTION('center_axis',(0.,-1.,0.)) ;
#119940=DIRECTION('ref_axis',(0.,0.,-1.)) ;
#119941=DIRECTION('center_axis',(-1.,1.06642836637918E-16,0.)) ;
#119942=DIRECTION('ref_axis',(-1.06642836637918E-16,-1.,0.)) ;
#119943=DIRECTION('center_axis',(1.,0.,0.)) ;
#119944=DIRECTION('ref_axis',(0.,0.,-1.)) ;
#119945=DIRECTION('center_axis',(0.,1.,0.)) ;
#119946=DIRECTION('ref_axis',(1.,0.,0.)) ;
#119947=DIRECTION('center_axis',(0.,0.,1.)) ;
#119948=DIRECTION('ref_axis',(1.,0.,0.)) ;
#119949=DIRECTION('center_axis',(0.,-1.,0.)) ;
#119950=DIRECTION('ref_axis',(0.,0.,-1.)) ;
#119951=DIRECTION('center_axis',(9.85638338623186E-18,1.,0.)) ;
#119952=DIRECTION('ref_axis',(-1.,9.85638338623186E-18,0.)) ;
#119953=DIRECTION('center_axis',(0.,-1.,0.)) ;
#119954=DIRECTION('ref_axis',(0.,0.,-1.)) ;
#119955=DIRECTION('center_axis',(0.,1.,0.)) ;
#119956=DIRECTION('ref_axis',(1.,0.,0.)) ;
#119957=DIRECTION('center_axis',(-1.,0.,0.)) ;
#119958=DIRECTION('ref_axis',(0.,0.,1.)) ;
#119959=DIRECTION('center_axis',(1.,-9.85638338623186E-18,0.)) ;
#119960=DIRECTION('ref_axis',(9.85638338623186E-18,1.,0.)) ;
#119961=DIRECTION('center_axis',(-1.,0.,0.)) ;
#119962=DIRECTION('ref_axis',(0.,0.,1.)) ;
#119963=DIRECTION('center_axis',(0.,1.,0.)) ;
#119964=DIRECTION('ref_axis',(1.,0.,0.)) ;
#119965=DIRECTION('center_axis',(0.,1.,0.)) ;
#119966=DIRECTION('ref_axis',(0.,0.,1.)) ;
#119967=DIRECTION('center_axis',(-9.85638338623186E-18,-1.,0.)) ;
#119968=DIRECTION('ref_axis',(1.,-9.85638338623186E-18,0.)) ;
#119969=DIRECTION('center_axis',(0.,1.,0.)) ;
#119970=DIRECTION('ref_axis',(0.,0.,1.)) ;
#119971=DIRECTION('center_axis',(0.,0.,1.)) ;
#119972=DIRECTION('ref_axis',(1.,0.,0.)) ;
#119973=DIRECTION('center_axis',(0.,0.,1.)) ;
#119974=DIRECTION('ref_axis',(1.,0.,0.)) ;
#119975=DIRECTION('center_axis',(0.,-1.,0.)) ;
#119976=DIRECTION('ref_axis',(0.,0.,-1.)) ;
#119977=DIRECTION('center_axis',(-9.85638338623186E-18,-1.,0.)) ;
#119978=DIRECTION('ref_axis',(1.,-9.85638338623186E-18,0.)) ;
#119979=DIRECTION('center_axis',(0.,-1.,0.)) ;
#119980=DIRECTION('ref_axis',(0.,0.,-1.)) ;
#119981=DIRECTION('center_axis',(0.,1.,0.)) ;
#119982=DIRECTION('ref_axis',(1.,0.,0.)) ;
#119983=DIRECTION('center_axis',(1.,-9.19976050010023E-15,0.)) ;
#119984=DIRECTION('ref_axis',(9.19976050010023E-15,1.,0.)) ;
#119985=DIRECTION('center_axis',(1.,-9.85638338623186E-18,0.)) ;
#119986=DIRECTION('ref_axis',(9.85638338623186E-18,1.,0.)) ;
#119987=DIRECTION('center_axis',(1.,0.,0.)) ;
#119988=DIRECTION('ref_axis',(0.,0.,-1.)) ;
#119989=DIRECTION('center_axis',(0.,1.,0.)) ;
#119990=DIRECTION('ref_axis',(1.,0.,0.)) ;
#119991=DIRECTION('center_axis',(0.,1.,0.)) ;
#119992=DIRECTION('ref_axis',(0.,0.,1.)) ;
#119993=DIRECTION('center_axis',(-9.85638338623186E-18,-1.,0.)) ;
#119994=DIRECTION('ref_axis',(1.,-9.85638338623186E-18,0.)) ;
#119995=DIRECTION('center_axis',(0.,1.,0.)) ;
#119996=DIRECTION('ref_axis',(0.,0.,1.)) ;
#119997=DIRECTION('center_axis',(0.,0.,1.)) ;
#119998=DIRECTION('ref_axis',(1.,0.,0.)) ;
#119999=DIRECTION('center_axis',(-1.,-1.95511867169517E-16,0.)) ;
#120000=DIRECTION('ref_axis',(1.95511867169517E-16,-1.,0.)) ;
#120001=DIRECTION('center_axis',(1.,0.,0.)) ;
#120002=DIRECTION('ref_axis',(0.,0.,-1.)) ;
#120003=DIRECTION('center_axis',(0.,1.,0.)) ;
#120004=DIRECTION('ref_axis',(1.,0.,0.)) ;
#120005=DIRECTION('center_axis',(-1.53329341668337E-15,-1.,0.)) ;
#120006=DIRECTION('ref_axis',(1.,-1.53329341668337E-15,0.)) ;
#120007=DIRECTION('center_axis',(-1.95511867169517E-16,1.,0.)) ;
#120008=DIRECTION('ref_axis',(-1.,-1.95511867169517E-16,0.)) ;
#120009=DIRECTION('center_axis',(0.,-1.,0.)) ;
#120010=DIRECTION('ref_axis',(0.,0.,-1.)) ;
#120011=DIRECTION('center_axis',(0.,1.,0.)) ;
#120012=DIRECTION('ref_axis',(1.,0.,0.)) ;
#120013=DIRECTION('center_axis',(-1.,0.,0.)) ;
#120014=DIRECTION('ref_axis',(0.,0.,1.)) ;
#120015=DIRECTION('center_axis',(1.,-1.06642836637918E-16,0.)) ;
#120016=DIRECTION('ref_axis',(1.06642836637918E-16,1.,0.)) ;
#120017=DIRECTION('center_axis',(1.,1.95511867169517E-16,0.)) ;
#120018=DIRECTION('ref_axis',(-1.95511867169517E-16,1.,0.)) ;
#120019=DIRECTION('center_axis',(1.,0.,0.)) ;
#120020=DIRECTION('ref_axis',(0.,0.,-1.)) ;
#120021=DIRECTION('center_axis',(0.,1.,0.)) ;
#120022=DIRECTION('ref_axis',(1.,0.,0.)) ;
#120023=DIRECTION('center_axis',(-3.06658683336674E-15,-1.,0.)) ;
#120024=DIRECTION('ref_axis',(1.,-3.06658683336674E-15,0.)) ;
#120025=DIRECTION('center_axis',(-1.95511867169517E-16,1.,0.)) ;
#120026=DIRECTION('ref_axis',(-1.,-1.95511867169517E-16,0.)) ;
#120027=DIRECTION('center_axis',(0.,-1.,0.)) ;
#120028=DIRECTION('ref_axis',(0.,0.,-1.)) ;
#120029=DIRECTION('center_axis',(-1.,1.06642836637918E-16,0.)) ;
#120030=DIRECTION('ref_axis',(-1.06642836637918E-16,-1.,0.)) ;
#120031=DIRECTION('center_axis',(1.,0.,0.)) ;
#120032=DIRECTION('ref_axis',(0.,0.,-1.)) ;
#120033=DIRECTION('center_axis',(0.,1.,0.)) ;
#120034=DIRECTION('ref_axis',(1.,0.,0.)) ;
#120035=DIRECTION('center_axis',(0.,0.,1.)) ;
#120036=DIRECTION('ref_axis',(1.,0.,0.)) ;
#120037=DIRECTION('center_axis',(0.,-1.,0.)) ;
#120038=DIRECTION('ref_axis',(0.,0.,-1.)) ;
#120039=DIRECTION('center_axis',(9.85638338623186E-18,1.,0.)) ;
#120040=DIRECTION('ref_axis',(-1.,9.85638338623186E-18,0.)) ;
#120041=DIRECTION('center_axis',(0.,-1.,0.)) ;
#120042=DIRECTION('ref_axis',(0.,0.,-1.)) ;
#120043=DIRECTION('center_axis',(0.,1.,0.)) ;
#120044=DIRECTION('ref_axis',(1.,0.,0.)) ;
#120045=DIRECTION('center_axis',(-1.,4.59988025005012E-15,0.)) ;
#120046=DIRECTION('ref_axis',(-4.59988025005012E-15,-1.,0.)) ;
#120047=DIRECTION('center_axis',(1.,-9.85638338623186E-18,0.)) ;
#120048=DIRECTION('ref_axis',(9.85638338623186E-18,1.,0.)) ;
#120049=DIRECTION('center_axis',(-1.,0.,0.)) ;
#120050=DIRECTION('ref_axis',(0.,0.,1.)) ;
#120051=DIRECTION('center_axis',(0.,1.,0.)) ;
#120052=DIRECTION('ref_axis',(1.,0.,0.)) ;
#120053=DIRECTION('center_axis',(0.,1.,0.)) ;
#120054=DIRECTION('ref_axis',(0.,0.,1.)) ;
#120055=DIRECTION('center_axis',(-9.85638338623186E-18,-1.,0.)) ;
#120056=DIRECTION('ref_axis',(1.,-9.85638338623186E-18,0.)) ;
#120057=DIRECTION('center_axis',(0.,1.,0.)) ;
#120058=DIRECTION('ref_axis',(0.,0.,1.)) ;
#120059=DIRECTION('center_axis',(0.,0.,1.)) ;
#120060=DIRECTION('ref_axis',(1.,0.,0.)) ;
#120061=DIRECTION('center_axis',(0.,0.,1.)) ;
#120062=DIRECTION('ref_axis',(1.,0.,0.)) ;
#120063=DIRECTION('center_axis',(0.,-1.,0.)) ;
#120064=DIRECTION('ref_axis',(0.,0.,-1.)) ;
#120065=DIRECTION('center_axis',(-9.85638338623186E-18,-1.,0.)) ;
#120066=DIRECTION('ref_axis',(1.,-9.85638338623186E-18,0.)) ;
#120067=DIRECTION('center_axis',(0.,-1.,0.)) ;
#120068=DIRECTION('ref_axis',(0.,0.,-1.)) ;
#120069=DIRECTION('center_axis',(0.,1.,0.)) ;
#120070=DIRECTION('ref_axis',(1.,0.,0.)) ;
#120071=DIRECTION('center_axis',(1.,-6.13317366673349E-15,0.)) ;
#120072=DIRECTION('ref_axis',(6.13317366673349E-15,1.,0.)) ;
#120073=DIRECTION('center_axis',(1.,-9.85638338623186E-18,0.)) ;
#120074=DIRECTION('ref_axis',(9.85638338623186E-18,1.,0.)) ;
#120075=DIRECTION('center_axis',(1.,0.,0.)) ;
#120076=DIRECTION('ref_axis',(0.,0.,-1.)) ;
#120077=DIRECTION('center_axis',(0.,1.,0.)) ;
#120078=DIRECTION('ref_axis',(1.,0.,0.)) ;
#120079=DIRECTION('center_axis',(0.,1.,0.)) ;
#120080=DIRECTION('ref_axis',(0.,0.,1.)) ;
#120081=DIRECTION('center_axis',(-9.85638338623186E-18,-1.,0.)) ;
#120082=DIRECTION('ref_axis',(1.,-9.85638338623186E-18,0.)) ;
#120083=DIRECTION('center_axis',(0.,1.,0.)) ;
#120084=DIRECTION('ref_axis',(0.,0.,1.)) ;
#120085=DIRECTION('center_axis',(0.,0.,1.)) ;
#120086=DIRECTION('ref_axis',(1.,0.,0.)) ;
#120087=DIRECTION('center_axis',(-1.,-1.95511867169517E-16,0.)) ;
#120088=DIRECTION('ref_axis',(1.95511867169517E-16,-1.,0.)) ;
#120089=DIRECTION('center_axis',(1.,0.,0.)) ;
#120090=DIRECTION('ref_axis',(0.,0.,-1.)) ;
#120091=DIRECTION('center_axis',(0.,1.,0.)) ;
#120092=DIRECTION('ref_axis',(1.,0.,0.)) ;
#120093=DIRECTION('center_axis',(1.22663473334668E-14,-1.,0.)) ;
#120094=DIRECTION('ref_axis',(1.,1.22663473334668E-14,0.)) ;
#120095=DIRECTION('center_axis',(-1.95511867169517E-16,1.,0.)) ;
#120096=DIRECTION('ref_axis',(-1.,-1.95511867169517E-16,0.)) ;
#120097=DIRECTION('center_axis',(0.,-1.,0.)) ;
#120098=DIRECTION('ref_axis',(0.,0.,-1.)) ;
#120099=DIRECTION('center_axis',(0.,1.,0.)) ;
#120100=DIRECTION('ref_axis',(1.,0.,0.)) ;
#120101=DIRECTION('center_axis',(-1.,0.,0.)) ;
#120102=DIRECTION('ref_axis',(0.,0.,1.)) ;
#120103=DIRECTION('center_axis',(1.,-1.06642836637918E-16,0.)) ;
#120104=DIRECTION('ref_axis',(1.06642836637918E-16,1.,0.)) ;
#120105=DIRECTION('center_axis',(1.,1.95511867169517E-16,0.)) ;
#120106=DIRECTION('ref_axis',(-1.95511867169517E-16,1.,0.)) ;
#120107=DIRECTION('center_axis',(1.,0.,0.)) ;
#120108=DIRECTION('ref_axis',(0.,0.,-1.)) ;
#120109=DIRECTION('center_axis',(0.,1.,0.)) ;
#120110=DIRECTION('ref_axis',(1.,0.,0.)) ;
#120111=DIRECTION('center_axis',(-8.43311379175855E-15,-1.,0.)) ;
#120112=DIRECTION('ref_axis',(1.,-8.43311379175855E-15,0.)) ;
#120113=DIRECTION('center_axis',(-1.95511867169517E-16,1.,0.)) ;
#120114=DIRECTION('ref_axis',(-1.,-1.95511867169517E-16,0.)) ;
#120115=DIRECTION('center_axis',(0.,-1.,0.)) ;
#120116=DIRECTION('ref_axis',(0.,0.,-1.)) ;
#120117=DIRECTION('center_axis',(-1.,1.06642836637918E-16,0.)) ;
#120118=DIRECTION('ref_axis',(-1.06642836637918E-16,-1.,0.)) ;
#120119=DIRECTION('center_axis',(1.,0.,0.)) ;
#120120=DIRECTION('ref_axis',(0.,0.,-1.)) ;
#120121=DIRECTION('center_axis',(0.,1.,0.)) ;
#120122=DIRECTION('ref_axis',(1.,0.,0.)) ;
#120123=DIRECTION('center_axis',(0.,0.,1.)) ;
#120124=DIRECTION('ref_axis',(1.,0.,0.)) ;
#120125=DIRECTION('center_axis',(0.,-1.,0.)) ;
#120126=DIRECTION('ref_axis',(0.,0.,-1.)) ;
#120127=DIRECTION('center_axis',(9.85638338623186E-18,1.,0.)) ;
#120128=DIRECTION('ref_axis',(-1.,9.85638338623186E-18,0.)) ;
#120129=DIRECTION('center_axis',(0.,-1.,0.)) ;
#120130=DIRECTION('ref_axis',(0.,0.,-1.)) ;
#120131=DIRECTION('center_axis',(0.,1.,0.)) ;
#120132=DIRECTION('ref_axis',(1.,0.,0.)) ;
#120133=DIRECTION('center_axis',(-1.,4.59988025005012E-15,0.)) ;
#120134=DIRECTION('ref_axis',(-4.59988025005012E-15,-1.,0.)) ;
#120135=DIRECTION('center_axis',(1.,-9.85638338623186E-18,0.)) ;
#120136=DIRECTION('ref_axis',(9.85638338623186E-18,1.,0.)) ;
#120137=DIRECTION('center_axis',(-1.,0.,0.)) ;
#120138=DIRECTION('ref_axis',(0.,0.,1.)) ;
#120139=DIRECTION('center_axis',(0.,1.,0.)) ;
#120140=DIRECTION('ref_axis',(1.,0.,0.)) ;
#120141=DIRECTION('center_axis',(0.,1.,0.)) ;
#120142=DIRECTION('ref_axis',(0.,0.,1.)) ;
#120143=DIRECTION('center_axis',(-9.85638338623186E-18,-1.,0.)) ;
#120144=DIRECTION('ref_axis',(1.,-9.85638338623186E-18,0.)) ;
#120145=DIRECTION('center_axis',(0.,1.,0.)) ;
#120146=DIRECTION('ref_axis',(0.,0.,1.)) ;
#120147=DIRECTION('center_axis',(0.,0.,1.)) ;
#120148=DIRECTION('ref_axis',(1.,0.,0.)) ;
#120149=DIRECTION('center_axis',(0.,0.,1.)) ;
#120150=DIRECTION('ref_axis',(1.,0.,0.)) ;
#120151=DIRECTION('center_axis',(0.,-1.,0.)) ;
#120152=DIRECTION('ref_axis',(0.,0.,-1.)) ;
#120153=DIRECTION('center_axis',(-9.85638338623186E-18,-1.,0.)) ;
#120154=DIRECTION('ref_axis',(1.,-9.85638338623186E-18,0.)) ;
#120155=DIRECTION('center_axis',(0.,-1.,0.)) ;
#120156=DIRECTION('ref_axis',(0.,0.,-1.)) ;
#120157=DIRECTION('center_axis',(0.,1.,0.)) ;
#120158=DIRECTION('ref_axis',(1.,0.,0.)) ;
#120159=DIRECTION('center_axis',(1.,-6.13317366673349E-15,0.)) ;
#120160=DIRECTION('ref_axis',(6.13317366673349E-15,1.,0.)) ;
#120161=DIRECTION('center_axis',(1.,-9.85638338623186E-18,0.)) ;
#120162=DIRECTION('ref_axis',(9.85638338623186E-18,1.,0.)) ;
#120163=DIRECTION('center_axis',(1.,0.,0.)) ;
#120164=DIRECTION('ref_axis',(0.,0.,-1.)) ;
#120165=DIRECTION('center_axis',(0.,1.,0.)) ;
#120166=DIRECTION('ref_axis',(1.,0.,0.)) ;
#120167=DIRECTION('center_axis',(0.,1.,0.)) ;
#120168=DIRECTION('ref_axis',(0.,0.,1.)) ;
#120169=DIRECTION('center_axis',(-9.85638338623186E-18,-1.,0.)) ;
#120170=DIRECTION('ref_axis',(1.,-9.85638338623186E-18,0.)) ;
#120171=DIRECTION('center_axis',(0.,1.,0.)) ;
#120172=DIRECTION('ref_axis',(0.,0.,1.)) ;
#120173=DIRECTION('center_axis',(0.,0.,1.)) ;
#120174=DIRECTION('ref_axis',(1.,0.,0.)) ;
#120175=DIRECTION('center_axis',(-1.,-1.95511867169517E-16,0.)) ;
#120176=DIRECTION('ref_axis',(1.95511867169517E-16,-1.,0.)) ;
#120177=DIRECTION('center_axis',(1.,0.,0.)) ;
#120178=DIRECTION('ref_axis',(0.,0.,-1.)) ;
#120179=DIRECTION('center_axis',(0.,1.,0.)) ;
#120180=DIRECTION('ref_axis',(1.,0.,0.)) ;
#120181=DIRECTION('center_axis',(1.22663473334668E-14,-1.,0.)) ;
#120182=DIRECTION('ref_axis',(1.,1.22663473334668E-14,0.)) ;
#120183=DIRECTION('center_axis',(-1.95511867169517E-16,1.,0.)) ;
#120184=DIRECTION('ref_axis',(-1.,-1.95511867169517E-16,0.)) ;
#120185=DIRECTION('center_axis',(0.,-1.,0.)) ;
#120186=DIRECTION('ref_axis',(0.,0.,-1.)) ;
#120187=DIRECTION('center_axis',(0.,1.,0.)) ;
#120188=DIRECTION('ref_axis',(1.,0.,0.)) ;
#120189=DIRECTION('center_axis',(-1.,0.,0.)) ;
#120190=DIRECTION('ref_axis',(0.,0.,1.)) ;
#120191=DIRECTION('center_axis',(1.,-1.06642836637918E-16,0.)) ;
#120192=DIRECTION('ref_axis',(1.06642836637918E-16,1.,0.)) ;
#120193=DIRECTION('center_axis',(1.,1.95511867169517E-16,0.)) ;
#120194=DIRECTION('ref_axis',(-1.95511867169517E-16,1.,0.)) ;
#120195=DIRECTION('center_axis',(1.,0.,0.)) ;
#120196=DIRECTION('ref_axis',(0.,0.,-1.)) ;
#120197=DIRECTION('center_axis',(0.,1.,0.)) ;
#120198=DIRECTION('ref_axis',(1.,0.,0.)) ;
#120199=DIRECTION('center_axis',(-8.43311379175855E-15,-1.,0.)) ;
#120200=DIRECTION('ref_axis',(1.,-8.43311379175855E-15,0.)) ;
#120201=DIRECTION('center_axis',(-1.95511867169517E-16,1.,0.)) ;
#120202=DIRECTION('ref_axis',(-1.,-1.95511867169517E-16,0.)) ;
#120203=DIRECTION('center_axis',(0.,-1.,0.)) ;
#120204=DIRECTION('ref_axis',(0.,0.,-1.)) ;
#120205=DIRECTION('center_axis',(-1.,1.06642836637918E-16,0.)) ;
#120206=DIRECTION('ref_axis',(-1.06642836637918E-16,-1.,0.)) ;
#120207=DIRECTION('center_axis',(1.,0.,0.)) ;
#120208=DIRECTION('ref_axis',(0.,0.,-1.)) ;
#120209=DIRECTION('center_axis',(0.,1.,0.)) ;
#120210=DIRECTION('ref_axis',(1.,0.,0.)) ;
#120211=DIRECTION('center_axis',(0.,0.,1.)) ;
#120212=DIRECTION('ref_axis',(1.,0.,0.)) ;
#120213=DIRECTION('center_axis',(0.,-1.,0.)) ;
#120214=DIRECTION('ref_axis',(0.,0.,-1.)) ;
#120215=DIRECTION('center_axis',(9.85638338623186E-18,1.,0.)) ;
#120216=DIRECTION('ref_axis',(-1.,9.85638338623186E-18,0.)) ;
#120217=DIRECTION('center_axis',(0.,-1.,0.)) ;
#120218=DIRECTION('ref_axis',(0.,0.,-1.)) ;
#120219=DIRECTION('center_axis',(0.,1.,0.)) ;
#120220=DIRECTION('ref_axis',(1.,0.,0.)) ;
#120221=DIRECTION('center_axis',(-1.,4.59988025005012E-15,0.)) ;
#120222=DIRECTION('ref_axis',(-4.59988025005012E-15,-1.,0.)) ;
#120223=DIRECTION('center_axis',(1.,-9.85638338623186E-18,0.)) ;
#120224=DIRECTION('ref_axis',(9.85638338623186E-18,1.,0.)) ;
#120225=DIRECTION('center_axis',(-1.,0.,0.)) ;
#120226=DIRECTION('ref_axis',(0.,0.,1.)) ;
#120227=DIRECTION('center_axis',(0.,1.,0.)) ;
#120228=DIRECTION('ref_axis',(1.,0.,0.)) ;
#120229=DIRECTION('center_axis',(0.,1.,0.)) ;
#120230=DIRECTION('ref_axis',(0.,0.,1.)) ;
#120231=DIRECTION('center_axis',(-9.85638338623186E-18,-1.,0.)) ;
#120232=DIRECTION('ref_axis',(1.,-9.85638338623186E-18,0.)) ;
#120233=DIRECTION('center_axis',(0.,1.,0.)) ;
#120234=DIRECTION('ref_axis',(0.,0.,1.)) ;
#120235=DIRECTION('center_axis',(0.,0.,1.)) ;
#120236=DIRECTION('ref_axis',(1.,0.,0.)) ;
#120237=DIRECTION('center_axis',(0.,0.,1.)) ;
#120238=DIRECTION('ref_axis',(1.,0.,0.)) ;
#120239=DIRECTION('center_axis',(0.,-1.,0.)) ;
#120240=DIRECTION('ref_axis',(0.,0.,-1.)) ;
#120241=DIRECTION('center_axis',(-9.85638338623186E-18,-1.,0.)) ;
#120242=DIRECTION('ref_axis',(1.,-9.85638338623186E-18,0.)) ;
#120243=DIRECTION('center_axis',(0.,-1.,0.)) ;
#120244=DIRECTION('ref_axis',(0.,0.,-1.)) ;
#120245=DIRECTION('center_axis',(0.,1.,0.)) ;
#120246=DIRECTION('ref_axis',(1.,0.,0.)) ;
#120247=DIRECTION('center_axis',(1.,-6.13317366673349E-15,0.)) ;
#120248=DIRECTION('ref_axis',(6.13317366673349E-15,1.,0.)) ;
#120249=DIRECTION('center_axis',(1.,-9.85638338623186E-18,0.)) ;
#120250=DIRECTION('ref_axis',(9.85638338623186E-18,1.,0.)) ;
#120251=DIRECTION('center_axis',(1.,0.,0.)) ;
#120252=DIRECTION('ref_axis',(0.,0.,-1.)) ;
#120253=DIRECTION('center_axis',(0.,1.,0.)) ;
#120254=DIRECTION('ref_axis',(1.,0.,0.)) ;
#120255=DIRECTION('center_axis',(0.,1.,0.)) ;
#120256=DIRECTION('ref_axis',(0.,0.,1.)) ;
#120257=DIRECTION('center_axis',(-9.85638338623186E-18,-1.,0.)) ;
#120258=DIRECTION('ref_axis',(1.,-9.85638338623186E-18,0.)) ;
#120259=DIRECTION('center_axis',(0.,1.,0.)) ;
#120260=DIRECTION('ref_axis',(0.,0.,1.)) ;
#120261=DIRECTION('center_axis',(0.,0.,1.)) ;
#120262=DIRECTION('ref_axis',(1.,0.,0.)) ;
#120263=DIRECTION('center_axis',(-1.,-1.95511867169517E-16,0.)) ;
#120264=DIRECTION('ref_axis',(1.95511867169517E-16,-1.,0.)) ;
#120265=DIRECTION('center_axis',(1.,0.,0.)) ;
#120266=DIRECTION('ref_axis',(0.,0.,-1.)) ;
#120267=DIRECTION('center_axis',(0.,1.,0.)) ;
#120268=DIRECTION('ref_axis',(1.,0.,0.)) ;
#120269=DIRECTION('center_axis',(1.22663473334668E-14,-1.,0.)) ;
#120270=DIRECTION('ref_axis',(1.,1.22663473334668E-14,0.)) ;
#120271=DIRECTION('center_axis',(-1.95511867169517E-16,1.,0.)) ;
#120272=DIRECTION('ref_axis',(-1.,-1.95511867169517E-16,0.)) ;
#120273=DIRECTION('center_axis',(0.,-1.,0.)) ;
#120274=DIRECTION('ref_axis',(0.,0.,-1.)) ;
#120275=DIRECTION('center_axis',(0.,1.,0.)) ;
#120276=DIRECTION('ref_axis',(1.,0.,0.)) ;
#120277=DIRECTION('center_axis',(-1.,0.,0.)) ;
#120278=DIRECTION('ref_axis',(0.,0.,1.)) ;
#120279=DIRECTION('center_axis',(1.,-1.06642836637918E-16,0.)) ;
#120280=DIRECTION('ref_axis',(1.06642836637918E-16,1.,0.)) ;
#120281=DIRECTION('center_axis',(1.,1.95511867169517E-16,0.)) ;
#120282=DIRECTION('ref_axis',(-1.95511867169517E-16,1.,0.)) ;
#120283=DIRECTION('center_axis',(1.,0.,0.)) ;
#120284=DIRECTION('ref_axis',(0.,0.,-1.)) ;
#120285=DIRECTION('center_axis',(0.,1.,0.)) ;
#120286=DIRECTION('ref_axis',(1.,0.,0.)) ;
#120287=DIRECTION('center_axis',(-8.43311379175855E-15,-1.,0.)) ;
#120288=DIRECTION('ref_axis',(1.,-8.43311379175855E-15,0.)) ;
#120289=DIRECTION('center_axis',(-1.95511867169517E-16,1.,0.)) ;
#120290=DIRECTION('ref_axis',(-1.,-1.95511867169517E-16,0.)) ;
#120291=DIRECTION('center_axis',(0.,-1.,0.)) ;
#120292=DIRECTION('ref_axis',(0.,0.,-1.)) ;
#120293=DIRECTION('center_axis',(-1.,1.06642836637918E-16,0.)) ;
#120294=DIRECTION('ref_axis',(-1.06642836637918E-16,-1.,0.)) ;
#120295=DIRECTION('center_axis',(1.,0.,0.)) ;
#120296=DIRECTION('ref_axis',(0.,0.,-1.)) ;
#120297=DIRECTION('center_axis',(0.,1.,0.)) ;
#120298=DIRECTION('ref_axis',(1.,0.,0.)) ;
#120299=DIRECTION('center_axis',(0.,0.,1.)) ;
#120300=DIRECTION('ref_axis',(1.,0.,0.)) ;
#120301=DIRECTION('center_axis',(0.,-1.,0.)) ;
#120302=DIRECTION('ref_axis',(0.,0.,-1.)) ;
#120303=DIRECTION('center_axis',(9.85638338623186E-18,1.,0.)) ;
#120304=DIRECTION('ref_axis',(-1.,9.85638338623186E-18,0.)) ;
#120305=DIRECTION('center_axis',(0.,-1.,0.)) ;
#120306=DIRECTION('ref_axis',(0.,0.,-1.)) ;
#120307=DIRECTION('center_axis',(0.,1.,0.)) ;
#120308=DIRECTION('ref_axis',(1.,0.,0.)) ;
#120309=DIRECTION('center_axis',(-1.,4.59988025005012E-15,0.)) ;
#120310=DIRECTION('ref_axis',(-4.59988025005012E-15,-1.,0.)) ;
#120311=DIRECTION('center_axis',(1.,-9.85638338623186E-18,0.)) ;
#120312=DIRECTION('ref_axis',(9.85638338623186E-18,1.,0.)) ;
#120313=DIRECTION('center_axis',(-1.,0.,0.)) ;
#120314=DIRECTION('ref_axis',(0.,0.,1.)) ;
#120315=DIRECTION('center_axis',(0.,1.,0.)) ;
#120316=DIRECTION('ref_axis',(1.,0.,0.)) ;
#120317=DIRECTION('center_axis',(0.,1.,0.)) ;
#120318=DIRECTION('ref_axis',(0.,0.,1.)) ;
#120319=DIRECTION('center_axis',(-9.85638338623186E-18,-1.,0.)) ;
#120320=DIRECTION('ref_axis',(1.,-9.85638338623186E-18,0.)) ;
#120321=DIRECTION('center_axis',(0.,1.,0.)) ;
#120322=DIRECTION('ref_axis',(0.,0.,1.)) ;
#120323=DIRECTION('center_axis',(0.,0.,1.)) ;
#120324=DIRECTION('ref_axis',(1.,0.,0.)) ;
#120325=DIRECTION('center_axis',(0.,0.,1.)) ;
#120326=DIRECTION('ref_axis',(1.,0.,0.)) ;
#120327=DIRECTION('center_axis',(0.,-1.,0.)) ;
#120328=DIRECTION('ref_axis',(0.,0.,-1.)) ;
#120329=DIRECTION('center_axis',(-9.85638338623186E-18,-1.,0.)) ;
#120330=DIRECTION('ref_axis',(1.,-9.85638338623186E-18,0.)) ;
#120331=DIRECTION('center_axis',(0.,-1.,0.)) ;
#120332=DIRECTION('ref_axis',(0.,0.,-1.)) ;
#120333=DIRECTION('center_axis',(0.,1.,0.)) ;
#120334=DIRECTION('ref_axis',(1.,0.,0.)) ;
#120335=DIRECTION('center_axis',(1.,-6.13317366673349E-15,0.)) ;
#120336=DIRECTION('ref_axis',(6.13317366673349E-15,1.,0.)) ;
#120337=DIRECTION('center_axis',(1.,-9.85638338623186E-18,0.)) ;
#120338=DIRECTION('ref_axis',(9.85638338623186E-18,1.,0.)) ;
#120339=DIRECTION('center_axis',(1.,0.,0.)) ;
#120340=DIRECTION('ref_axis',(0.,0.,-1.)) ;
#120341=DIRECTION('center_axis',(0.,1.,0.)) ;
#120342=DIRECTION('ref_axis',(1.,0.,0.)) ;
#120343=DIRECTION('center_axis',(0.,1.,0.)) ;
#120344=DIRECTION('ref_axis',(0.,0.,1.)) ;
#120345=DIRECTION('center_axis',(-9.85638338623186E-18,-1.,0.)) ;
#120346=DIRECTION('ref_axis',(1.,-9.85638338623186E-18,0.)) ;
#120347=DIRECTION('center_axis',(0.,1.,0.)) ;
#120348=DIRECTION('ref_axis',(0.,0.,1.)) ;
#120349=DIRECTION('center_axis',(0.,0.,1.)) ;
#120350=DIRECTION('ref_axis',(1.,0.,0.)) ;
#120351=DIRECTION('center_axis',(-1.,-1.95511867169517E-16,0.)) ;
#120352=DIRECTION('ref_axis',(1.95511867169517E-16,-1.,0.)) ;
#120353=DIRECTION('center_axis',(1.,0.,0.)) ;
#120354=DIRECTION('ref_axis',(0.,0.,-1.)) ;
#120355=DIRECTION('center_axis',(0.,1.,0.)) ;
#120356=DIRECTION('ref_axis',(1.,0.,0.)) ;
#120357=DIRECTION('center_axis',(1.22663473334668E-14,-1.,0.)) ;
#120358=DIRECTION('ref_axis',(1.,1.22663473334668E-14,0.)) ;
#120359=DIRECTION('center_axis',(-1.95511867169517E-16,1.,0.)) ;
#120360=DIRECTION('ref_axis',(-1.,-1.95511867169517E-16,0.)) ;
#120361=DIRECTION('center_axis',(0.,-1.,0.)) ;
#120362=DIRECTION('ref_axis',(0.,0.,-1.)) ;
#120363=DIRECTION('center_axis',(0.,1.,0.)) ;
#120364=DIRECTION('ref_axis',(1.,0.,0.)) ;
#120365=DIRECTION('center_axis',(-1.,0.,0.)) ;
#120366=DIRECTION('ref_axis',(0.,0.,1.)) ;
#120367=DIRECTION('center_axis',(1.,-1.06642836637918E-16,0.)) ;
#120368=DIRECTION('ref_axis',(1.06642836637918E-16,1.,0.)) ;
#120369=DIRECTION('center_axis',(1.,1.95511867169517E-16,0.)) ;
#120370=DIRECTION('ref_axis',(-1.95511867169517E-16,1.,0.)) ;
#120371=DIRECTION('center_axis',(1.,0.,0.)) ;
#120372=DIRECTION('ref_axis',(0.,0.,-1.)) ;
#120373=DIRECTION('center_axis',(0.,1.,0.)) ;
#120374=DIRECTION('ref_axis',(1.,0.,0.)) ;
#120375=DIRECTION('center_axis',(-8.43311379175855E-15,-1.,0.)) ;
#120376=DIRECTION('ref_axis',(1.,-8.43311379175855E-15,0.)) ;
#120377=DIRECTION('center_axis',(-1.95511867169517E-16,1.,0.)) ;
#120378=DIRECTION('ref_axis',(-1.,-1.95511867169517E-16,0.)) ;
#120379=DIRECTION('center_axis',(0.,-1.,0.)) ;
#120380=DIRECTION('ref_axis',(0.,0.,-1.)) ;
#120381=DIRECTION('center_axis',(-1.,1.06642836637918E-16,0.)) ;
#120382=DIRECTION('ref_axis',(-1.06642836637918E-16,-1.,0.)) ;
#120383=DIRECTION('center_axis',(1.,0.,0.)) ;
#120384=DIRECTION('ref_axis',(0.,0.,-1.)) ;
#120385=DIRECTION('center_axis',(0.,1.,0.)) ;
#120386=DIRECTION('ref_axis',(1.,0.,0.)) ;
#120387=DIRECTION('center_axis',(0.,0.,1.)) ;
#120388=DIRECTION('ref_axis',(1.,0.,0.)) ;
#120389=DIRECTION('center_axis',(0.,-1.,0.)) ;
#120390=DIRECTION('ref_axis',(0.,0.,-1.)) ;
#120391=DIRECTION('center_axis',(9.85638338623186E-18,1.,0.)) ;
#120392=DIRECTION('ref_axis',(-1.,9.85638338623186E-18,0.)) ;
#120393=DIRECTION('center_axis',(0.,-1.,0.)) ;
#120394=DIRECTION('ref_axis',(0.,0.,-1.)) ;
#120395=DIRECTION('center_axis',(0.,1.,0.)) ;
#120396=DIRECTION('ref_axis',(1.,0.,0.)) ;
#120397=DIRECTION('center_axis',(-1.,1.83995210002007E-14,0.)) ;
#120398=DIRECTION('ref_axis',(-1.83995210002007E-14,-1.,0.)) ;
#120399=DIRECTION('center_axis',(1.,-9.85638338623186E-18,0.)) ;
#120400=DIRECTION('ref_axis',(9.85638338623186E-18,1.,0.)) ;
#120401=DIRECTION('center_axis',(-1.,0.,0.)) ;
#120402=DIRECTION('ref_axis',(0.,0.,1.)) ;
#120403=DIRECTION('center_axis',(0.,1.,0.)) ;
#120404=DIRECTION('ref_axis',(1.,0.,0.)) ;
#120405=DIRECTION('center_axis',(0.,1.,0.)) ;
#120406=DIRECTION('ref_axis',(0.,0.,1.)) ;
#120407=DIRECTION('center_axis',(-9.85638338623186E-18,-1.,0.)) ;
#120408=DIRECTION('ref_axis',(1.,-9.85638338623186E-18,0.)) ;
#120409=DIRECTION('center_axis',(0.,1.,0.)) ;
#120410=DIRECTION('ref_axis',(0.,0.,1.)) ;
#120411=DIRECTION('center_axis',(0.,0.,1.)) ;
#120412=DIRECTION('ref_axis',(1.,0.,0.)) ;
#120413=DIRECTION('center_axis',(0.,0.,1.)) ;
#120414=DIRECTION('ref_axis',(1.,0.,0.)) ;
#120415=DIRECTION('center_axis',(0.,-1.,0.)) ;
#120416=DIRECTION('ref_axis',(0.,0.,-1.)) ;
#120417=DIRECTION('center_axis',(-9.85638338623186E-18,-1.,0.)) ;
#120418=DIRECTION('ref_axis',(1.,-9.85638338623186E-18,0.)) ;
#120419=DIRECTION('center_axis',(0.,-1.,0.)) ;
#120420=DIRECTION('ref_axis',(0.,0.,-1.)) ;
#120421=DIRECTION('center_axis',(0.,1.,0.)) ;
#120422=DIRECTION('ref_axis',(1.,0.,0.)) ;
#120423=DIRECTION('center_axis',(1.,2.22327545419092E-14,0.)) ;
#120424=DIRECTION('ref_axis',(-2.22327545419092E-14,1.,0.)) ;
#120425=DIRECTION('center_axis',(1.,-9.85638338623186E-18,0.)) ;
#120426=DIRECTION('ref_axis',(9.85638338623186E-18,1.,0.)) ;
#120427=DIRECTION('center_axis',(1.,0.,0.)) ;
#120428=DIRECTION('ref_axis',(0.,0.,-1.)) ;
#120429=DIRECTION('center_axis',(0.,1.,0.)) ;
#120430=DIRECTION('ref_axis',(1.,0.,0.)) ;
#120431=DIRECTION('center_axis',(0.,1.,0.)) ;
#120432=DIRECTION('ref_axis',(0.,0.,1.)) ;
#120433=DIRECTION('center_axis',(-9.85638338623186E-18,-1.,0.)) ;
#120434=DIRECTION('ref_axis',(1.,-9.85638338623186E-18,0.)) ;
#120435=DIRECTION('center_axis',(0.,1.,0.)) ;
#120436=DIRECTION('ref_axis',(0.,0.,1.)) ;
#120437=DIRECTION('center_axis',(0.,0.,1.)) ;
#120438=DIRECTION('ref_axis',(1.,0.,0.)) ;
#120439=DIRECTION('center_axis',(-1.,-1.95511867169517E-16,0.)) ;
#120440=DIRECTION('ref_axis',(1.95511867169517E-16,-1.,0.)) ;
#120441=DIRECTION('center_axis',(1.,0.,0.)) ;
#120442=DIRECTION('ref_axis',(0.,0.,-1.)) ;
#120443=DIRECTION('center_axis',(0.,1.,0.)) ;
#120444=DIRECTION('ref_axis',(1.,0.,0.)) ;
#120445=DIRECTION('center_axis',(-1.83995210002007E-14,-1.,0.)) ;
#120446=DIRECTION('ref_axis',(1.,-1.83995210002007E-14,0.)) ;
#120447=DIRECTION('center_axis',(-1.95511867169517E-16,1.,0.)) ;
#120448=DIRECTION('ref_axis',(-1.,-1.95511867169517E-16,0.)) ;
#120449=DIRECTION('center_axis',(0.,-1.,0.)) ;
#120450=DIRECTION('ref_axis',(0.,0.,-1.)) ;
#120451=DIRECTION('center_axis',(0.,1.,0.)) ;
#120452=DIRECTION('ref_axis',(1.,0.,0.)) ;
#120453=DIRECTION('center_axis',(-1.,0.,0.)) ;
#120454=DIRECTION('ref_axis',(0.,0.,1.)) ;
#120455=DIRECTION('center_axis',(1.,-1.06642836637918E-16,0.)) ;
#120456=DIRECTION('ref_axis',(1.06642836637918E-16,1.,0.)) ;
#120457=DIRECTION('center_axis',(1.,1.95511867169517E-16,0.)) ;
#120458=DIRECTION('ref_axis',(-1.95511867169517E-16,1.,0.)) ;
#120459=DIRECTION('center_axis',(1.,0.,0.)) ;
#120460=DIRECTION('ref_axis',(0.,0.,-1.)) ;
#120461=DIRECTION('center_axis',(0.,1.,0.)) ;
#120462=DIRECTION('ref_axis',(1.,0.,0.)) ;
#120463=DIRECTION('center_axis',(2.68326347919587E-14,-1.,0.)) ;
#120464=DIRECTION('ref_axis',(1.,2.68326347919587E-14,0.)) ;
#120465=DIRECTION('center_axis',(-1.95511867169517E-16,1.,0.)) ;
#120466=DIRECTION('ref_axis',(-1.,-1.95511867169517E-16,0.)) ;
#120467=DIRECTION('center_axis',(0.,-1.,0.)) ;
#120468=DIRECTION('ref_axis',(0.,0.,-1.)) ;
#120469=DIRECTION('center_axis',(-1.,1.06642836637918E-16,0.)) ;
#120470=DIRECTION('ref_axis',(-1.06642836637918E-16,-1.,0.)) ;
#120471=DIRECTION('center_axis',(1.,0.,0.)) ;
#120472=DIRECTION('ref_axis',(0.,0.,-1.)) ;
#120473=DIRECTION('center_axis',(0.,1.,0.)) ;
#120474=DIRECTION('ref_axis',(1.,0.,0.)) ;
#141826=CARTESIAN_POINT('',(0.,0.,0.)) ;
#141827=CARTESIAN_POINT('Origin',(2.3,0.,-34.29)) ;
#141828=CARTESIAN_POINT('',(2.4,-1.10218211923262E-16,-33.39)) ;
#141829=CARTESIAN_POINT('Origin',(2.4,0.,-34.29)) ;
#141830=CARTESIAN_POINT('',(2.3,-1.22464679914735E-16,-33.29)) ;
#141831=CARTESIAN_POINT('Origin',(2.3,-1.10218211923262E-16,-33.39)) ;
#141832=CARTESIAN_POINT('',(2.3,1.22464679914735E-16,-35.29)) ;
#141833=CARTESIAN_POINT('Origin',(2.3,0.,-34.29)) ;
#141834=CARTESIAN_POINT('Origin',(2.3,0.,-34.29)) ;
#141835=CARTESIAN_POINT('Origin',(1.5,0.,-34.29)) ;
#141836=CARTESIAN_POINT('',(1.4,-1.34711147906208E-16,-35.39)) ;
#141837=CARTESIAN_POINT('Origin',(1.4,0.,-34.29)) ;
#141838=CARTESIAN_POINT('',(1.5,-1.22464679914735E-16,-35.29)) ;
#141839=CARTESIAN_POINT('Origin',(1.5,-1.34711147906209E-16,-35.39)) ;
#141840=CARTESIAN_POINT('Origin',(1.5,0.,-34.29)) ;
#141841=CARTESIAN_POINT('Origin',(1.5,3.15,-33.0314213562373)) ;
#141842=CARTESIAN_POINT('',(1.5,3.07928932188135,-32.9607106781187)) ;
#141843=CARTESIAN_POINT('',(1.5,3.25,-33.0314213562373)) ;
#141844=CARTESIAN_POINT('Origin',(1.5,3.15,-33.0314213562373)) ;
#141845=CARTESIAN_POINT('',(1.4,3.15,-33.0314213562373)) ;
#141846=CARTESIAN_POINT('Origin',(1.5,3.15,-33.0314213562373)) ;
#141847=CARTESIAN_POINT('Origin',(1.5,3.15,-33.0314213562373)) ;
#141848=CARTESIAN_POINT('Origin',(0.500000000000001,-4.56640444411537E-17,
-34.69)) ;
#141849=CARTESIAN_POINT('',(0.600000000000001,0.4,-34.69)) ;
#141850=CARTESIAN_POINT('',(0.59561299721608,0.370705721320401,-34.6607057213204)) ;
#141851=CARTESIAN_POINT('Origin',(0.500000000014529,0.399999999998192,-34.6899999999979)) ;
#141852=CARTESIAN_POINT('',(0.500000000000001,0.4,-34.79)) ;
#141853=CARTESIAN_POINT('Origin',(0.500000000000001,0.4,-34.69)) ;
#141854=CARTESIAN_POINT('',(0.500000000000001,-1.9,-34.79)) ;
#141855=CARTESIAN_POINT('',(0.500000000000001,0.5,-34.79)) ;
#141856=CARTESIAN_POINT('',(0.600000000000001,-1.9,-34.69)) ;
#141857=CARTESIAN_POINT('Origin',(0.500000000000001,-1.9,-34.69)) ;
#141858=CARTESIAN_POINT('',(0.600000000000001,-0.3,-34.69)) ;
#141859=CARTESIAN_POINT('',(0.600000000000001,-2.39800009914437E-17,-34.69)) ;
#141860=CARTESIAN_POINT('',(0.600000000000001,0.299999999999999,-34.69)) ;
#141861=CARTESIAN_POINT('',(0.600000000000001,-2.39800009914437E-17,-34.69)) ;
#141862=CARTESIAN_POINT('Ctrl Pts',(0.600000000000001,0.300000000000003,
-34.69)) ;
#141863=CARTESIAN_POINT('Ctrl Pts',(0.600000000000001,0.312243016306297,
-34.69)) ;
#141864=CARTESIAN_POINT('Ctrl Pts',(0.60006974742297,0.324350425899703,
-34.6877515285214)) ;
#141865=CARTESIAN_POINT('Ctrl Pts',(0.599517124288205,0.34619696929781,
-34.6793954490601)) ;
#141866=CARTESIAN_POINT('Ctrl Pts',(0.598927484301131,0.355857825373572,
-34.6736750447227)) ;
#141867=CARTESIAN_POINT('Ctrl Pts',(0.596766673872563,0.366539012308038,
-34.6647023851096)) ;
#141868=CARTESIAN_POINT('Ctrl Pts',(0.59623562910414,0.368676603883175,
-34.6627379168092)) ;
#141869=CARTESIAN_POINT('Ctrl Pts',(0.59561299721608,0.370705721320409,
-34.6607057213204)) ;
#141870=CARTESIAN_POINT('Origin',(2.3,0.,-30.48)) ;
#141871=CARTESIAN_POINT('',(2.4,-1.10218211923262E-16,-29.58)) ;
#141872=CARTESIAN_POINT('Origin',(2.4,0.,-30.48)) ;
#141873=CARTESIAN_POINT('',(2.3,-1.22464679914735E-16,-29.48)) ;
#141874=CARTESIAN_POINT('Origin',(2.3,-1.10218211923262E-16,-29.58)) ;
#141875=CARTESIAN_POINT('',(2.3,1.22464679914735E-16,-31.48)) ;
#141876=CARTESIAN_POINT('Origin',(2.3,0.,-30.48)) ;
#141877=CARTESIAN_POINT('Origin',(2.3,0.,-30.48)) ;
#141878=CARTESIAN_POINT('Origin',(1.5,0.,-30.48)) ;
#141879=CARTESIAN_POINT('',(1.4,-1.34711147906209E-16,-31.58)) ;
#141880=CARTESIAN_POINT('Origin',(1.4,0.,-30.48)) ;
#141881=CARTESIAN_POINT('',(1.5,-1.22464679914735E-16,-31.48)) ;
#141882=CARTESIAN_POINT('Origin',(1.5,-1.34711147906209E-16,-31.58)) ;
#141883=CARTESIAN_POINT('Origin',(1.5,0.,-30.48)) ;
#141884=CARTESIAN_POINT('Origin',(1.5,3.15,-29.2214213562373)) ;
#141885=CARTESIAN_POINT('',(1.5,3.07928932188135,-29.1507106781187)) ;
#141886=CARTESIAN_POINT('',(1.5,3.25,-29.2214213562373)) ;
#141887=CARTESIAN_POINT('Origin',(1.5,3.15,-29.2214213562373)) ;
#141888=CARTESIAN_POINT('',(1.4,3.15,-29.2214213562373)) ;
#141889=CARTESIAN_POINT('Origin',(1.5,3.15,-29.2214213562373)) ;
#141890=CARTESIAN_POINT('Origin',(1.5,3.15,-29.2214213562373)) ;
#141891=CARTESIAN_POINT('Origin',(0.500000000000001,-4.56640444411542E-17,
-30.88)) ;
#141892=CARTESIAN_POINT('',(0.600000000000001,0.4,-30.88)) ;
#141893=CARTESIAN_POINT('',(0.595612997216081,0.370705721320403,-30.8507057213204)) ;
#141894=CARTESIAN_POINT('Origin',(0.500000000043895,0.399999999994469,-30.8799999999944)) ;
#141895=CARTESIAN_POINT('',(0.500000000000001,0.4,-30.98)) ;
#141896=CARTESIAN_POINT('Origin',(0.500000000000001,0.4,-30.88)) ;
#141897=CARTESIAN_POINT('',(0.500000000000001,-1.9,-30.98)) ;
#141898=CARTESIAN_POINT('',(0.500000000000001,0.5,-30.98)) ;
#141899=CARTESIAN_POINT('',(0.600000000000001,-1.9,-30.88)) ;
#141900=CARTESIAN_POINT('Origin',(0.500000000000001,-1.9,-30.88)) ;
#141901=CARTESIAN_POINT('',(0.600000000000001,-0.3,-30.88)) ;
#141902=CARTESIAN_POINT('',(0.600000000000001,-2.39800009914441E-17,-30.88)) ;
#141903=CARTESIAN_POINT('',(0.600000000000001,0.299999999999999,-30.88)) ;
#141904=CARTESIAN_POINT('',(0.600000000000001,-2.39800009914441E-17,-30.88)) ;
#141905=CARTESIAN_POINT('Ctrl Pts',(0.600000000000001,0.300000000000003,
-30.88)) ;
#141906=CARTESIAN_POINT('Ctrl Pts',(0.600000000000001,0.312243016306059,
-30.88)) ;
#141907=CARTESIAN_POINT('Ctrl Pts',(0.600069747422976,0.324350425899479,
-30.8777515285215)) ;
#141908=CARTESIAN_POINT('Ctrl Pts',(0.59951712428821,0.346196969297596,
-30.8693954490601)) ;
#141909=CARTESIAN_POINT('Ctrl Pts',(0.598927484301166,0.355857825373397,
-30.8636750447228)) ;
#141910=CARTESIAN_POINT('Ctrl Pts',(0.596766673872565,0.36653901230802,
-30.8547023851096)) ;
#141911=CARTESIAN_POINT('Ctrl Pts',(0.596235629104145,0.368676603883157,
-30.8527379168092)) ;
#141912=CARTESIAN_POINT('Ctrl Pts',(0.595612997216081,0.370705721320405,
-30.8507057213204)) ;
#141913=CARTESIAN_POINT('Origin',(2.3,0.,-26.67)) ;
#141914=CARTESIAN_POINT('',(2.4,-1.10218211923262E-16,-25.77)) ;
#141915=CARTESIAN_POINT('Origin',(2.4,0.,-26.67)) ;
#141916=CARTESIAN_POINT('',(2.3,-1.22464679914735E-16,-25.67)) ;
#141917=CARTESIAN_POINT('Origin',(2.3,-1.10218211923262E-16,-25.77)) ;
#141918=CARTESIAN_POINT('',(2.3,1.22464679914735E-16,-27.67)) ;
#141919=CARTESIAN_POINT('Origin',(2.3,0.,-26.67)) ;
#141920=CARTESIAN_POINT('Origin',(2.3,0.,-26.67)) ;
#141921=CARTESIAN_POINT('Origin',(1.5,0.,-26.67)) ;
#141922=CARTESIAN_POINT('',(1.4,-1.34711147906209E-16,-27.77)) ;
#141923=CARTESIAN_POINT('Origin',(1.4,0.,-26.67)) ;
#141924=CARTESIAN_POINT('',(1.5,-1.22464679914735E-16,-27.67)) ;
#141925=CARTESIAN_POINT('Origin',(1.5,-1.34711147906209E-16,-27.77)) ;
#141926=CARTESIAN_POINT('Origin',(1.5,0.,-26.67)) ;
#141927=CARTESIAN_POINT('Origin',(1.5,3.15,-25.4114213562373)) ;
#141928=CARTESIAN_POINT('',(1.5,3.07928932188135,-25.3407106781187)) ;
#141929=CARTESIAN_POINT('',(1.5,3.25,-25.4114213562373)) ;
#141930=CARTESIAN_POINT('Origin',(1.5,3.15,-25.4114213562373)) ;
#141931=CARTESIAN_POINT('',(1.4,3.15,-25.4114213562373)) ;
#141932=CARTESIAN_POINT('Origin',(1.5,3.15,-25.4114213562373)) ;
#141933=CARTESIAN_POINT('Origin',(1.5,3.15,-25.4114213562373)) ;
#141934=CARTESIAN_POINT('Origin',(0.500000000000001,-4.56640444411542E-17,
-27.07)) ;
#141935=CARTESIAN_POINT('',(0.600000000000001,0.4,-27.07)) ;
#141936=CARTESIAN_POINT('',(0.595612997216081,0.370705721320403,-27.0407057213204)) ;
#141937=CARTESIAN_POINT('Origin',(0.500000000043127,0.39999999999434,-27.0699999999943)) ;
#141938=CARTESIAN_POINT('',(0.500000000000001,0.4,-27.17)) ;
#141939=CARTESIAN_POINT('Origin',(0.500000000000001,0.4,-27.07)) ;
#141940=CARTESIAN_POINT('',(0.500000000000001,-1.9,-27.17)) ;
#141941=CARTESIAN_POINT('',(0.500000000000001,0.5,-27.17)) ;
#141942=CARTESIAN_POINT('',(0.600000000000001,-1.9,-27.07)) ;
#141943=CARTESIAN_POINT('Origin',(0.500000000000001,-1.9,-27.07)) ;
#141944=CARTESIAN_POINT('',(0.600000000000001,-0.3,-27.07)) ;
#141945=CARTESIAN_POINT('',(0.600000000000001,-2.39800009914441E-17,-27.07)) ;
#141946=CARTESIAN_POINT('',(0.600000000000001,0.299999999999999,-27.07)) ;
#141947=CARTESIAN_POINT('',(0.600000000000001,-2.39800009914441E-17,-27.07)) ;
#141948=CARTESIAN_POINT('Ctrl Pts',(0.600000000000001,0.300000000000003,
-27.07)) ;
#141949=CARTESIAN_POINT('Ctrl Pts',(0.600000000000001,0.312243016306037,
-27.07)) ;
#141950=CARTESIAN_POINT('Ctrl Pts',(0.600069747422976,0.324350425899459,
-27.0677515285215)) ;
#141951=CARTESIAN_POINT('Ctrl Pts',(0.59951712428821,0.346196969297585,
-27.0593954490602)) ;
#141952=CARTESIAN_POINT('Ctrl Pts',(0.598927484301167,0.355857825373385,
-27.0536750447229)) ;
#141953=CARTESIAN_POINT('Ctrl Pts',(0.596766673872565,0.366539012308015,
-27.0447023851096)) ;
#141954=CARTESIAN_POINT('Ctrl Pts',(0.596235629104144,0.368676603883154,
-27.0427379168092)) ;
#141955=CARTESIAN_POINT('Ctrl Pts',(0.59561299721608,0.370705721320403,
-27.0407057213204)) ;
#141956=CARTESIAN_POINT('Origin',(2.3,0.,-22.86)) ;
#141957=CARTESIAN_POINT('',(2.4,-1.10218211923262E-16,-21.96)) ;
#141958=CARTESIAN_POINT('Origin',(2.4,0.,-22.86)) ;
#141959=CARTESIAN_POINT('',(2.3,-1.22464679914735E-16,-21.86)) ;
#141960=CARTESIAN_POINT('Origin',(2.3,-1.10218211923262E-16,-21.96)) ;
#141961=CARTESIAN_POINT('',(2.3,1.22464679914735E-16,-23.86)) ;
#141962=CARTESIAN_POINT('Origin',(2.3,0.,-22.86)) ;
#141963=CARTESIAN_POINT('Origin',(2.3,0.,-22.86)) ;
#141964=CARTESIAN_POINT('Origin',(1.5,0.,-22.86)) ;
#141965=CARTESIAN_POINT('',(1.4,-1.34711147906209E-16,-23.96)) ;
#141966=CARTESIAN_POINT('Origin',(1.4,0.,-22.86)) ;
#141967=CARTESIAN_POINT('',(1.5,-1.22464679914735E-16,-23.86)) ;
#141968=CARTESIAN_POINT('Origin',(1.5,-1.34711147906209E-16,-23.96)) ;
#141969=CARTESIAN_POINT('Origin',(1.5,0.,-22.86)) ;
#141970=CARTESIAN_POINT('Origin',(1.5,3.15,-21.6014213562373)) ;
#141971=CARTESIAN_POINT('',(1.5,3.07928932188135,-21.5307106781187)) ;
#141972=CARTESIAN_POINT('',(1.5,3.25,-21.6014213562373)) ;
#141973=CARTESIAN_POINT('Origin',(1.5,3.15,-21.6014213562373)) ;
#141974=CARTESIAN_POINT('',(1.4,3.15,-21.6014213562373)) ;
#141975=CARTESIAN_POINT('Origin',(1.5,3.15,-21.6014213562373)) ;
#141976=CARTESIAN_POINT('Origin',(1.5,3.15,-21.6014213562373)) ;
#141977=CARTESIAN_POINT('Origin',(0.500000000000001,-4.56640444411542E-17,
-23.26)) ;
#141978=CARTESIAN_POINT('',(0.600000000000001,0.4,-23.26)) ;
#141979=CARTESIAN_POINT('',(0.595612997216081,0.370705721320403,-23.2307057213204)) ;
#141980=CARTESIAN_POINT('Origin',(0.50000000005309,0.399999999992667,-23.2599999999926)) ;
#141981=CARTESIAN_POINT('',(0.500000000000001,0.4,-23.36)) ;
#141982=CARTESIAN_POINT('Origin',(0.500000000000001,0.4,-23.26)) ;
#141983=CARTESIAN_POINT('',(0.500000000000001,-1.9,-23.36)) ;
#141984=CARTESIAN_POINT('',(0.500000000000001,0.5,-23.36)) ;
#141985=CARTESIAN_POINT('',(0.600000000000001,-1.9,-23.26)) ;
#141986=CARTESIAN_POINT('Origin',(0.500000000000001,-1.9,-23.26)) ;
#141987=CARTESIAN_POINT('',(0.600000000000001,-0.3,-23.26)) ;
#141988=CARTESIAN_POINT('',(0.600000000000001,-2.39800009914441E-17,-23.26)) ;
#141989=CARTESIAN_POINT('',(0.600000000000001,0.299999999999999,-23.26)) ;
#141990=CARTESIAN_POINT('',(0.600000000000001,-2.39800009914441E-17,-23.26)) ;
#141991=CARTESIAN_POINT('Ctrl Pts',(0.600000000000001,0.300000000000003,
-23.26)) ;
#141992=CARTESIAN_POINT('Ctrl Pts',(0.600000000000001,0.312243016306061,
-23.26)) ;
#141993=CARTESIAN_POINT('Ctrl Pts',(0.600069747422976,0.324350425899477,
-23.2577515285215)) ;
#141994=CARTESIAN_POINT('Ctrl Pts',(0.599517124288211,0.346196969297576,
-23.2493954490602)) ;
#141995=CARTESIAN_POINT('Ctrl Pts',(0.598927484301166,0.35585782537339,
-23.2436750447229)) ;
#141996=CARTESIAN_POINT('Ctrl Pts',(0.596766673872565,0.36653901230802,
-23.2347023851096)) ;
#141997=CARTESIAN_POINT('Ctrl Pts',(0.596235629104145,0.368676603883157,
-23.2327379168092)) ;
#141998=CARTESIAN_POINT('Ctrl Pts',(0.595612997216081,0.370705721320404,
-23.2307057213204)) ;
#141999=CARTESIAN_POINT('Origin',(2.3,0.,-19.05)) ;
#142000=CARTESIAN_POINT('',(2.4,-1.10218211923262E-16,-18.15)) ;
#142001=CARTESIAN_POINT('Origin',(2.4,0.,-19.05)) ;
#142002=CARTESIAN_POINT('',(2.3,-1.22464679914735E-16,-18.05)) ;
#142003=CARTESIAN_POINT('Origin',(2.3,-1.10218211923262E-16,-18.15)) ;
#142004=CARTESIAN_POINT('',(2.3,1.22464679914735E-16,-20.05)) ;
#142005=CARTESIAN_POINT('Origin',(2.3,0.,-19.05)) ;
#142006=CARTESIAN_POINT('Origin',(2.3,0.,-19.05)) ;
#142007=CARTESIAN_POINT('Origin',(1.5,0.,-19.05)) ;
#142008=CARTESIAN_POINT('',(1.4,-1.34711147906209E-16,-20.15)) ;
#142009=CARTESIAN_POINT('Origin',(1.4,0.,-19.05)) ;
#142010=CARTESIAN_POINT('',(1.5,-1.22464679914735E-16,-20.05)) ;
#142011=CARTESIAN_POINT('Origin',(1.5,-1.34711147906209E-16,-20.15)) ;
#142012=CARTESIAN_POINT('Origin',(1.5,0.,-19.05)) ;
#142013=CARTESIAN_POINT('Origin',(1.5,3.15,-17.7914213562373)) ;
#142014=CARTESIAN_POINT('',(1.5,3.07928932188135,-17.7207106781187)) ;
#142015=CARTESIAN_POINT('',(1.5,3.25,-17.7914213562373)) ;
#142016=CARTESIAN_POINT('Origin',(1.5,3.15,-17.7914213562373)) ;
#142017=CARTESIAN_POINT('',(1.4,3.15,-17.7914213562373)) ;
#142018=CARTESIAN_POINT('Origin',(1.5,3.15,-17.7914213562373)) ;
#142019=CARTESIAN_POINT('Origin',(1.5,3.15,-17.7914213562373)) ;
#142020=CARTESIAN_POINT('Origin',(0.500000000000001,-4.56640444411542E-17,
-19.45)) ;
#142021=CARTESIAN_POINT('',(0.600000000000001,0.4,-19.45)) ;
#142022=CARTESIAN_POINT('',(0.595612997216081,0.370705721320403,-19.4207057213204)) ;
#142023=CARTESIAN_POINT('Origin',(0.500000000041676,0.399999999994165,-19.4499999999941)) ;
#142024=CARTESIAN_POINT('',(0.500000000000001,0.4,-19.55)) ;
#142025=CARTESIAN_POINT('Origin',(0.500000000000001,0.4,-19.45)) ;
#142026=CARTESIAN_POINT('',(0.500000000000001,-1.9,-19.55)) ;
#142027=CARTESIAN_POINT('',(0.500000000000001,0.5,-19.55)) ;
#142028=CARTESIAN_POINT('',(0.600000000000001,-1.9,-19.45)) ;
#142029=CARTESIAN_POINT('Origin',(0.500000000000001,-1.9,-19.45)) ;
#142030=CARTESIAN_POINT('',(0.600000000000001,-0.3,-19.45)) ;
#142031=CARTESIAN_POINT('',(0.600000000000001,-2.39800009914441E-17,-19.45)) ;
#142032=CARTESIAN_POINT('',(0.600000000000001,0.299999999999999,-19.45)) ;
#142033=CARTESIAN_POINT('',(0.600000000000001,-2.39800009914441E-17,-19.45)) ;
#142034=CARTESIAN_POINT('Ctrl Pts',(0.600000000000001,0.300000000000003,
-19.45)) ;
#142035=CARTESIAN_POINT('Ctrl Pts',(0.600000000000001,0.312243016306433,
-19.45)) ;
#142036=CARTESIAN_POINT('Ctrl Pts',(0.600069747422966,0.324350425899823,
-19.4477515285214)) ;
#142037=CARTESIAN_POINT('Ctrl Pts',(0.599517124288202,0.346196969297921,
-19.43939544906)) ;
#142038=CARTESIAN_POINT('Ctrl Pts',(0.598927484301112,0.355857825373661,
-19.4336750447226)) ;
#142039=CARTESIAN_POINT('Ctrl Pts',(0.596766673872561,0.366539012308041,
-19.4247023851096)) ;
#142040=CARTESIAN_POINT('Ctrl Pts',(0.596235629104139,0.368676603883175,
-19.4227379168092)) ;
#142041=CARTESIAN_POINT('Ctrl Pts',(0.595612997216081,0.370705721320404,
-19.4207057213204)) ;
#142042=CARTESIAN_POINT('Origin',(2.3,0.,-15.24)) ;
#142043=CARTESIAN_POINT('',(2.4,-1.10218211923262E-16,-14.34)) ;
#142044=CARTESIAN_POINT('Origin',(2.4,0.,-15.24)) ;
#142045=CARTESIAN_POINT('',(2.3,-1.22464679914735E-16,-14.24)) ;
#142046=CARTESIAN_POINT('Origin',(2.3,-1.10218211923262E-16,-14.34)) ;
#142047=CARTESIAN_POINT('',(2.3,1.22464679914735E-16,-16.24)) ;
#142048=CARTESIAN_POINT('Origin',(2.3,0.,-15.24)) ;
#142049=CARTESIAN_POINT('Origin',(2.3,0.,-15.24)) ;
#142050=CARTESIAN_POINT('Origin',(1.5,0.,-15.24)) ;
#142051=CARTESIAN_POINT('',(1.4,-1.34711147906209E-16,-16.34)) ;
#142052=CARTESIAN_POINT('Origin',(1.4,0.,-15.24)) ;
#142053=CARTESIAN_POINT('',(1.5,-1.22464679914735E-16,-16.24)) ;
#142054=CARTESIAN_POINT('Origin',(1.5,-1.34711147906209E-16,-16.34)) ;
#142055=CARTESIAN_POINT('Origin',(1.5,0.,-15.24)) ;
#142056=CARTESIAN_POINT('Origin',(1.5,3.15,-13.9814213562373)) ;
#142057=CARTESIAN_POINT('',(1.5,3.07928932188135,-13.9107106781187)) ;
#142058=CARTESIAN_POINT('',(1.5,3.25,-13.9814213562373)) ;
#142059=CARTESIAN_POINT('Origin',(1.5,3.15,-13.9814213562373)) ;
#142060=CARTESIAN_POINT('',(1.4,3.15,-13.9814213562373)) ;
#142061=CARTESIAN_POINT('Origin',(1.5,3.15,-13.9814213562373)) ;
#142062=CARTESIAN_POINT('Origin',(1.5,3.15,-13.9814213562373)) ;
#142063=CARTESIAN_POINT('Origin',(0.500000000000001,-4.56640444411542E-17,
-15.64)) ;
#142064=CARTESIAN_POINT('',(0.600000000000001,0.4,-15.64)) ;
#142065=CARTESIAN_POINT('',(0.595612997216081,0.370705721320403,-15.6107057213204)) ;
#142066=CARTESIAN_POINT('Origin',(0.499999999962138,0.400000000005185,-15.6400000000051)) ;
#142067=CARTESIAN_POINT('',(0.500000000000001,0.4,-15.74)) ;
#142068=CARTESIAN_POINT('Origin',(0.500000000000001,0.4,-15.64)) ;
#142069=CARTESIAN_POINT('',(0.500000000000001,-1.9,-15.74)) ;
#142070=CARTESIAN_POINT('',(0.500000000000001,0.5,-15.74)) ;
#142071=CARTESIAN_POINT('',(0.600000000000001,-1.9,-15.64)) ;
#142072=CARTESIAN_POINT('Origin',(0.500000000000001,-1.9,-15.64)) ;
#142073=CARTESIAN_POINT('',(0.600000000000001,-0.3,-15.64)) ;
#142074=CARTESIAN_POINT('',(0.600000000000001,-2.39800009914441E-17,-15.64)) ;
#142075=CARTESIAN_POINT('',(0.600000000000001,0.299999999999999,-15.64)) ;
#142076=CARTESIAN_POINT('',(0.600000000000001,-2.39800009914441E-17,-15.64)) ;
#142077=CARTESIAN_POINT('Ctrl Pts',(0.600000000000001,0.300000000000003,
-15.64)) ;
#142078=CARTESIAN_POINT('Ctrl Pts',(0.600000000000001,0.312243016306305,
-15.64)) ;
#142079=CARTESIAN_POINT('Ctrl Pts',(0.60006974742297,0.324350425899701,
-15.6377515285214)) ;
#142080=CARTESIAN_POINT('Ctrl Pts',(0.599517124288205,0.346196969297796,
-15.6293954490601)) ;
#142081=CARTESIAN_POINT('Ctrl Pts',(0.59892748430113,0.355857825373563,
-15.6236750447227)) ;
#142082=CARTESIAN_POINT('Ctrl Pts',(0.596766673872562,0.366539012308031,
-15.6147023851096)) ;
#142083=CARTESIAN_POINT('Ctrl Pts',(0.596235629104141,0.368676603883168,
-15.6127379168092)) ;
#142084=CARTESIAN_POINT('Ctrl Pts',(0.59561299721608,0.370705721320404,
-15.6107057213204)) ;
#142085=CARTESIAN_POINT('Origin',(2.3,0.,-11.43)) ;
#142086=CARTESIAN_POINT('',(2.4,-1.10218211923262E-16,-10.53)) ;
#142087=CARTESIAN_POINT('Origin',(2.4,0.,-11.43)) ;
#142088=CARTESIAN_POINT('',(2.3,-1.22464679914735E-16,-10.43)) ;
#142089=CARTESIAN_POINT('Origin',(2.3,-1.10218211923262E-16,-10.53)) ;
#142090=CARTESIAN_POINT('',(2.3,1.22464679914735E-16,-12.43)) ;
#142091=CARTESIAN_POINT('Origin',(2.3,0.,-11.43)) ;
#142092=CARTESIAN_POINT('Origin',(2.3,0.,-11.43)) ;
#142093=CARTESIAN_POINT('Origin',(1.5,0.,-11.43)) ;
#142094=CARTESIAN_POINT('',(1.4,-1.34711147906209E-16,-12.53)) ;
#142095=CARTESIAN_POINT('Origin',(1.4,0.,-11.43)) ;
#142096=CARTESIAN_POINT('',(1.5,-1.22464679914735E-16,-12.43)) ;
#142097=CARTESIAN_POINT('Origin',(1.5,-1.34711147906209E-16,-12.53)) ;
#142098=CARTESIAN_POINT('Origin',(1.5,0.,-11.43)) ;
#142099=CARTESIAN_POINT('Origin',(1.5,3.15,-10.1714213562373)) ;
#142100=CARTESIAN_POINT('',(1.5,3.07928932188135,-10.1007106781187)) ;
#142101=CARTESIAN_POINT('',(1.5,3.25,-10.1714213562373)) ;
#142102=CARTESIAN_POINT('Origin',(1.5,3.15,-10.1714213562373)) ;
#142103=CARTESIAN_POINT('',(1.4,3.15,-10.1714213562373)) ;
#142104=CARTESIAN_POINT('Origin',(1.5,3.15,-10.1714213562373)) ;
#142105=CARTESIAN_POINT('Origin',(1.5,3.15,-10.1714213562373)) ;
#142106=CARTESIAN_POINT('Origin',(0.500000000000001,-4.56640444411542E-17,
-11.83)) ;
#142107=CARTESIAN_POINT('',(0.600000000000001,0.4,-11.83)) ;
#142108=CARTESIAN_POINT('',(0.59561299721608,0.370705721320402,-11.8007057213204)) ;
#142109=CARTESIAN_POINT('Origin',(0.500000000002749,0.399999999999878,-11.8299999999996)) ;
#142110=CARTESIAN_POINT('',(0.500000000000001,0.4,-11.93)) ;
#142111=CARTESIAN_POINT('Origin',(0.500000000000001,0.4,-11.83)) ;
#142112=CARTESIAN_POINT('',(0.500000000000001,-1.9,-11.93)) ;
#142113=CARTESIAN_POINT('',(0.500000000000001,0.5,-11.93)) ;
#142114=CARTESIAN_POINT('',(0.600000000000001,-1.9,-11.83)) ;
#142115=CARTESIAN_POINT('Origin',(0.500000000000001,-1.9,-11.83)) ;
#142116=CARTESIAN_POINT('',(0.600000000000001,-0.3,-11.83)) ;
#142117=CARTESIAN_POINT('',(0.600000000000001,-2.39800009914441E-17,-11.83)) ;
#142118=CARTESIAN_POINT('',(0.600000000000001,0.299999999999999,-11.83)) ;
#142119=CARTESIAN_POINT('',(0.600000000000001,-2.39800009914441E-17,-11.83)) ;
#142120=CARTESIAN_POINT('Ctrl Pts',(0.600000000000001,0.300000000000003,
-11.83)) ;
#142121=CARTESIAN_POINT('Ctrl Pts',(0.600000000000001,0.312243016306181,
-11.83)) ;
#142122=CARTESIAN_POINT('Ctrl Pts',(0.600069747422973,0.324350425899585,
-11.8277515285214)) ;
#142123=CARTESIAN_POINT('Ctrl Pts',(0.599517124288208,0.346196969297684,
-11.8193954490601)) ;
#142124=CARTESIAN_POINT('Ctrl Pts',(0.598927484301148,0.355857825373472,
-11.8136750447228)) ;
#142125=CARTESIAN_POINT('Ctrl Pts',(0.596766673872564,0.366539012308024,
-11.8047023851096)) ;
#142126=CARTESIAN_POINT('Ctrl Pts',(0.596235629104143,0.368676603883159,
-11.8027379168092)) ;
#142127=CARTESIAN_POINT('Ctrl Pts',(0.595612997216081,0.370705721320402,
-11.8007057213204)) ;
#142128=CARTESIAN_POINT('Origin',(2.3,0.,-7.62)) ;
#142129=CARTESIAN_POINT('',(2.4,-1.10218211923262E-16,-6.72)) ;
#142130=CARTESIAN_POINT('Origin',(2.4,0.,-7.62)) ;
#142131=CARTESIAN_POINT('',(2.3,-1.22464679914735E-16,-6.62)) ;
#142132=CARTESIAN_POINT('Origin',(2.3,-1.10218211923262E-16,-6.72)) ;
#142133=CARTESIAN_POINT('',(2.3,1.22464679914735E-16,-8.62)) ;
#142134=CARTESIAN_POINT('Origin',(2.3,0.,-7.62)) ;
#142135=CARTESIAN_POINT('Origin',(2.3,0.,-7.62)) ;
#142136=CARTESIAN_POINT('Origin',(1.5,0.,-7.62)) ;
#142137=CARTESIAN_POINT('',(1.4,-1.34711147906209E-16,-8.72)) ;
#142138=CARTESIAN_POINT('Origin',(1.4,0.,-7.62)) ;
#142139=CARTESIAN_POINT('',(1.5,-1.22464679914735E-16,-8.62)) ;
#142140=CARTESIAN_POINT('Origin',(1.5,-1.34711147906209E-16,-8.72)) ;
#142141=CARTESIAN_POINT('Origin',(1.5,0.,-7.62)) ;
#142142=CARTESIAN_POINT('Origin',(1.5,3.15,-6.36142135623731)) ;
#142143=CARTESIAN_POINT('',(1.5,3.07928932188135,-6.29071067811866)) ;
#142144=CARTESIAN_POINT('',(1.5,3.25,-6.36142135623731)) ;
#142145=CARTESIAN_POINT('Origin',(1.5,3.15,-6.36142135623731)) ;
#142146=CARTESIAN_POINT('',(1.4,3.15,-6.36142135623731)) ;
#142147=CARTESIAN_POINT('Origin',(1.5,3.15,-6.36142135623731)) ;
#142148=CARTESIAN_POINT('Origin',(1.5,3.15,-6.36142135623731)) ;
#142149=CARTESIAN_POINT('Origin',(0.500000000000001,-4.56640444411542E-17,
-8.02)) ;
#142150=CARTESIAN_POINT('',(0.600000000000001,0.4,-8.02)) ;
#142151=CARTESIAN_POINT('',(0.59561299721608,0.370705721320402,-7.9907057213204)) ;
#142152=CARTESIAN_POINT('Origin',(0.499999999996157,0.400000000000788,-8.02000000000056)) ;
#142153=CARTESIAN_POINT('',(0.500000000000001,0.4,-8.12)) ;
#142154=CARTESIAN_POINT('Origin',(0.500000000000001,0.4,-8.02)) ;
#142155=CARTESIAN_POINT('',(0.500000000000001,-1.9,-8.12)) ;
#142156=CARTESIAN_POINT('',(0.500000000000001,0.5,-8.12)) ;
#142157=CARTESIAN_POINT('',(0.600000000000001,-1.9,-8.02)) ;
#142158=CARTESIAN_POINT('Origin',(0.500000000000001,-1.9,-8.02)) ;
#142159=CARTESIAN_POINT('',(0.600000000000001,-0.3,-8.02)) ;
#142160=CARTESIAN_POINT('',(0.600000000000001,-2.39800009914441E-17,-8.02)) ;
#142161=CARTESIAN_POINT('',(0.600000000000001,0.299999999999999,-8.02)) ;
#142162=CARTESIAN_POINT('',(0.600000000000001,-2.39800009914441E-17,-8.02)) ;
#142163=CARTESIAN_POINT('Ctrl Pts',(0.600000000000001,0.300000000000003,
-8.02)) ;
#142164=CARTESIAN_POINT('Ctrl Pts',(0.600000000000001,0.312243016306057,
-8.02)) ;
#142165=CARTESIAN_POINT('Ctrl Pts',(0.600069747422976,0.32435042589947,
-8.01775152852148)) ;
#142166=CARTESIAN_POINT('Ctrl Pts',(0.599517124288211,0.346196969297575,
-8.00939544906016)) ;
#142167=CARTESIAN_POINT('Ctrl Pts',(0.598927484301167,0.355857825373384,
-8.00367504472285)) ;
#142168=CARTESIAN_POINT('Ctrl Pts',(0.596766673872565,0.366539012308017,
-7.99470238510958)) ;
#142169=CARTESIAN_POINT('Ctrl Pts',(0.596235629104145,0.368676603883154,
-7.9927379168092)) ;
#142170=CARTESIAN_POINT('Ctrl Pts',(0.59561299721608,0.370705721320404,
-7.9907057213204)) ;
#142171=CARTESIAN_POINT('Origin',(2.3,0.,-3.81)) ;
#142172=CARTESIAN_POINT('',(2.4,-1.10218211923262E-16,-2.91)) ;
#142173=CARTESIAN_POINT('Origin',(2.4,0.,-3.81)) ;
#142174=CARTESIAN_POINT('',(2.3,-1.22464679914735E-16,-2.81)) ;
#142175=CARTESIAN_POINT('Origin',(2.3,-1.10218211923262E-16,-2.91)) ;
#142176=CARTESIAN_POINT('',(2.3,1.22464679914735E-16,-4.81)) ;
#142177=CARTESIAN_POINT('Origin',(2.3,0.,-3.81)) ;
#142178=CARTESIAN_POINT('Origin',(2.3,0.,-3.81)) ;
#142179=CARTESIAN_POINT('Origin',(7.9,3.15,-5.06857864376269)) ;
#142180=CARTESIAN_POINT('',(8.,3.35,-5.06857864376269)) ;
#142181=CARTESIAN_POINT('',(8.,3.00857864376269,-5.21)) ;
#142182=CARTESIAN_POINT('Origin',(8.,3.15,-5.06857864376269)) ;
#142183=CARTESIAN_POINT('',(7.9,3.25,-5.06857864376269)) ;
#142184=CARTESIAN_POINT('Origin',(7.9,3.35,-5.06857864376269)) ;
#142185=CARTESIAN_POINT('',(7.9,3.07928932188135,-5.13928932188135)) ;
#142186=CARTESIAN_POINT('Origin',(7.9,3.15,-5.06857864376269)) ;
#142187=CARTESIAN_POINT('Origin',(7.9,3.00857864376269,-5.21)) ;
#142188=CARTESIAN_POINT('Origin',(7.9,3.15,-8.87857864376269)) ;
#142189=CARTESIAN_POINT('',(8.,3.35,-8.87857864376269)) ;
#142190=CARTESIAN_POINT('',(8.,3.00857864376269,-9.02)) ;
#142191=CARTESIAN_POINT('Origin',(8.,3.15,-8.87857864376269)) ;
#142192=CARTESIAN_POINT('',(7.9,3.25,-8.87857864376269)) ;
#142193=CARTESIAN_POINT('Origin',(7.9,3.35,-8.87857864376269)) ;
#142194=CARTESIAN_POINT('',(7.9,3.07928932188135,-8.94928932188134)) ;
#142195=CARTESIAN_POINT('Origin',(7.9,3.15,-8.87857864376269)) ;
#142196=CARTESIAN_POINT('Origin',(7.9,3.00857864376269,-9.02)) ;
#142197=CARTESIAN_POINT('Origin',(7.9,3.15,-12.6885786437627)) ;
#142198=CARTESIAN_POINT('',(8.,3.35,-12.6885786437627)) ;
#142199=CARTESIAN_POINT('',(8.,3.00857864376269,-12.83)) ;
#142200=CARTESIAN_POINT('Origin',(8.,3.15,-12.6885786437627)) ;
#142201=CARTESIAN_POINT('',(7.9,3.25,-12.6885786437627)) ;
#142202=CARTESIAN_POINT('Origin',(7.9,3.35,-12.6885786437627)) ;
#142203=CARTESIAN_POINT('',(7.9,3.07928932188135,-12.7592893218813)) ;
#142204=CARTESIAN_POINT('Origin',(7.9,3.15,-12.6885786437627)) ;
#142205=CARTESIAN_POINT('Origin',(7.9,3.00857864376269,-12.83)) ;
#142206=CARTESIAN_POINT('Origin',(7.9,3.15,-16.4985786437627)) ;
#142207=CARTESIAN_POINT('',(8.,3.35,-16.4985786437627)) ;
#142208=CARTESIAN_POINT('',(8.,3.00857864376269,-16.64)) ;
#142209=CARTESIAN_POINT('Origin',(8.,3.15,-16.4985786437627)) ;
#142210=CARTESIAN_POINT('',(7.9,3.25,-16.4985786437627)) ;
#142211=CARTESIAN_POINT('Origin',(7.9,3.35,-16.4985786437627)) ;
#142212=CARTESIAN_POINT('',(7.9,3.07928932188135,-16.5692893218813)) ;
#142213=CARTESIAN_POINT('Origin',(7.9,3.15,-16.4985786437627)) ;
#142214=CARTESIAN_POINT('Origin',(7.9,3.00857864376269,-16.64)) ;
#142215=CARTESIAN_POINT('Origin',(7.9,3.15,-20.3085786437627)) ;
#142216=CARTESIAN_POINT('',(8.,3.35,-20.3085786437627)) ;
#142217=CARTESIAN_POINT('',(8.,3.00857864376269,-20.45)) ;
#142218=CARTESIAN_POINT('Origin',(8.,3.15,-20.3085786437627)) ;
#142219=CARTESIAN_POINT('',(7.9,3.25,-20.3085786437627)) ;
#142220=CARTESIAN_POINT('Origin',(7.9,3.35,-20.3085786437627)) ;
#142221=CARTESIAN_POINT('',(7.9,3.07928932188135,-20.3792893218813)) ;
#142222=CARTESIAN_POINT('Origin',(7.9,3.15,-20.3085786437627)) ;
#142223=CARTESIAN_POINT('Origin',(7.9,3.00857864376269,-20.45)) ;
#142224=CARTESIAN_POINT('Origin',(7.9,3.15,-24.1185786437627)) ;
#142225=CARTESIAN_POINT('',(8.,3.35,-24.1185786437627)) ;
#142226=CARTESIAN_POINT('',(8.,3.00857864376269,-24.26)) ;
#142227=CARTESIAN_POINT('Origin',(8.,3.15,-24.1185786437627)) ;
#142228=CARTESIAN_POINT('',(7.9,3.25,-24.1185786437627)) ;
#142229=CARTESIAN_POINT('Origin',(7.9,3.35,-24.1185786437627)) ;
#142230=CARTESIAN_POINT('',(7.9,3.07928932188135,-24.1892893218813)) ;
#142231=CARTESIAN_POINT('Origin',(7.9,3.15,-24.1185786437627)) ;
#142232=CARTESIAN_POINT('Origin',(7.9,3.00857864376269,-24.26)) ;
#142233=CARTESIAN_POINT('Origin',(7.9,3.15,-27.9285786437627)) ;
#142234=CARTESIAN_POINT('',(8.,3.35,-27.9285786437627)) ;
#142235=CARTESIAN_POINT('',(8.,3.00857864376269,-28.07)) ;
#142236=CARTESIAN_POINT('Origin',(8.,3.15,-27.9285786437627)) ;
#142237=CARTESIAN_POINT('',(7.9,3.25,-27.9285786437627)) ;
#142238=CARTESIAN_POINT('Origin',(7.9,3.35,-27.9285786437627)) ;
#142239=CARTESIAN_POINT('',(7.9,3.07928932188135,-27.9992893218813)) ;
#142240=CARTESIAN_POINT('Origin',(7.9,3.15,-27.9285786437627)) ;
#142241=CARTESIAN_POINT('Origin',(7.9,3.00857864376269,-28.07)) ;
#142242=CARTESIAN_POINT('Origin',(7.9,3.15,-31.7385786437627)) ;
#142243=CARTESIAN_POINT('',(8.,3.35,-31.7385786437627)) ;
#142244=CARTESIAN_POINT('',(8.,3.00857864376269,-31.88)) ;
#142245=CARTESIAN_POINT('Origin',(8.,3.15,-31.7385786437627)) ;
#142246=CARTESIAN_POINT('',(7.9,3.25,-31.7385786437627)) ;
#142247=CARTESIAN_POINT('Origin',(7.9,3.35,-31.7385786437627)) ;
#142248=CARTESIAN_POINT('',(7.9,3.07928932188135,-31.8092893218813)) ;
#142249=CARTESIAN_POINT('Origin',(7.9,3.15,-31.7385786437627)) ;
#142250=CARTESIAN_POINT('Origin',(7.9,3.00857864376269,-31.88)) ;
#142251=CARTESIAN_POINT('Origin',(7.9,3.15,-35.5485786437627)) ;
#142252=CARTESIAN_POINT('',(8.,3.35,-35.5485786437627)) ;
#142253=CARTESIAN_POINT('',(8.,3.00857864376269,-35.69)) ;
#142254=CARTESIAN_POINT('Origin',(8.,3.15,-35.5485786437627)) ;
#142255=CARTESIAN_POINT('',(7.9,3.25,-35.5485786437627)) ;
#142256=CARTESIAN_POINT('Origin',(7.9,3.35,-35.5485786437627)) ;
#142257=CARTESIAN_POINT('',(7.9,3.07928932188135,-35.6192893218813)) ;
#142258=CARTESIAN_POINT('Origin',(7.9,3.15,-35.5485786437627)) ;
#142259=CARTESIAN_POINT('Origin',(7.9,3.00857864376269,-35.69)) ;
#142260=CARTESIAN_POINT('Origin',(1.5,0.,-3.81)) ;
#142261=CARTESIAN_POINT('',(1.4,-1.34711147906209E-16,-4.91)) ;
#142262=CARTESIAN_POINT('Origin',(1.4,0.,-3.81)) ;
#142263=CARTESIAN_POINT('',(1.5,-1.22464679914735E-16,-4.81)) ;
#142264=CARTESIAN_POINT('Origin',(1.5,-1.34711147906209E-16,-4.91)) ;
#142265=CARTESIAN_POINT('Origin',(1.5,0.,-3.81)) ;
#142266=CARTESIAN_POINT('Origin',(1.5,3.15,-2.55142135623731)) ;
#142267=CARTESIAN_POINT('',(1.5,3.07928932188135,-2.48071067811865)) ;
#142268=CARTESIAN_POINT('',(1.5,3.25,-2.55142135623731)) ;
#142269=CARTESIAN_POINT('Origin',(1.5,3.15,-2.55142135623731)) ;
#142270=CARTESIAN_POINT('',(1.4,3.15,-2.55142135623731)) ;
#142271=CARTESIAN_POINT('Origin',(1.5,3.15,-2.55142135623731)) ;
#142272=CARTESIAN_POINT('Origin',(1.5,3.15,-2.55142135623731)) ;
#142273=CARTESIAN_POINT('Origin',(0.500000000000001,-4.56640444411539E-17,
-4.21)) ;
#142274=CARTESIAN_POINT('',(0.600000000000001,0.4,-4.21)) ;
#142275=CARTESIAN_POINT('',(0.595612997216081,0.370705721320403,-4.1807057213204)) ;
#142276=CARTESIAN_POINT('Origin',(0.499999999992608,0.400000000001211,-4.21000000000122)) ;
#142277=CARTESIAN_POINT('',(0.500000000000001,0.4,-4.31)) ;
#142278=CARTESIAN_POINT('Origin',(0.500000000000001,0.4,-4.21)) ;
#142279=CARTESIAN_POINT('',(0.500000000000001,-1.9,-4.31)) ;
#142280=CARTESIAN_POINT('',(0.500000000000001,0.5,-4.31)) ;
#142281=CARTESIAN_POINT('',(0.600000000000001,-1.9,-4.21)) ;
#142282=CARTESIAN_POINT('Origin',(0.500000000000001,-1.9,-4.21)) ;
#142283=CARTESIAN_POINT('',(0.600000000000001,-0.3,-4.21)) ;
#142284=CARTESIAN_POINT('',(0.600000000000001,-2.39800009914439E-17,-4.21)) ;
#142285=CARTESIAN_POINT('',(0.600000000000001,0.299999999999999,-4.21)) ;
#142286=CARTESIAN_POINT('',(0.600000000000001,-2.39800009914439E-17,-4.21)) ;
#142287=CARTESIAN_POINT('Ctrl Pts',(0.600000000000001,0.300000000000003,
-4.21)) ;
#142288=CARTESIAN_POINT('Ctrl Pts',(0.600000000000001,0.312243016306119,
-4.21)) ;
#142289=CARTESIAN_POINT('Ctrl Pts',(0.600069747422974,0.324350425899533,
-4.20775152852146)) ;
#142290=CARTESIAN_POINT('Ctrl Pts',(0.599517124288209,0.346196969297642,
-4.19939544906013)) ;
#142291=CARTESIAN_POINT('Ctrl Pts',(0.598927484301157,0.355857825373437,
-4.19367504472281)) ;
#142292=CARTESIAN_POINT('Ctrl Pts',(0.596766673872564,0.366539012308024,
-4.18470238510957)) ;
#142293=CARTESIAN_POINT('Ctrl Pts',(0.596235629104143,0.36867660388316,
-4.18273791680919)) ;
#142294=CARTESIAN_POINT('Ctrl Pts',(0.595612997216081,0.370705721320404,
-4.1807057213204)) ;
#142295=CARTESIAN_POINT('Origin',(2.4,0.,-34.29)) ;
#142296=CARTESIAN_POINT('',(2.4,-1.22464679914735E-16,-35.29)) ;
#142297=CARTESIAN_POINT('Origin',(2.4,0.,-30.48)) ;
#142298=CARTESIAN_POINT('',(2.4,-1.22464679914735E-16,-31.48)) ;
#142299=CARTESIAN_POINT('Origin',(2.4,0.,-26.67)) ;
#142300=CARTESIAN_POINT('',(2.4,-1.22464679914735E-16,-27.67)) ;
#142301=CARTESIAN_POINT('Origin',(2.4,0.,-22.86)) ;
#142302=CARTESIAN_POINT('',(2.4,-1.22464679914735E-16,-23.86)) ;
#142303=CARTESIAN_POINT('Origin',(2.4,0.,-19.05)) ;
#142304=CARTESIAN_POINT('',(2.4,-1.22464679914735E-16,-20.05)) ;
#142305=CARTESIAN_POINT('Origin',(2.4,0.,-15.24)) ;
#142306=CARTESIAN_POINT('',(2.4,-1.22464679914735E-16,-16.24)) ;
#142307=CARTESIAN_POINT('Origin',(2.4,0.,-11.43)) ;
#142308=CARTESIAN_POINT('',(2.4,-1.22464679914735E-16,-12.43)) ;
#142309=CARTESIAN_POINT('Origin',(2.4,0.,-7.62)) ;
#142310=CARTESIAN_POINT('',(2.4,-1.22464679914735E-16,-8.62)) ;
#142311=CARTESIAN_POINT('Origin',(2.4,0.,-3.81)) ;
#142312=CARTESIAN_POINT('',(2.4,-1.22464679914735E-16,-4.81)) ;
#142313=CARTESIAN_POINT('Origin',(1.4,3.15,-5.06857864376269)) ;
#142314=CARTESIAN_POINT('',(1.5,3.25,-5.06857864376269)) ;
#142315=CARTESIAN_POINT('',(1.5,3.07928932188135,-5.13928932188135)) ;
#142316=CARTESIAN_POINT('Origin',(1.5,3.15,-5.06857864376269)) ;
#142317=CARTESIAN_POINT('',(1.4,3.07928932188135,-5.13928932188135)) ;
#142318=CARTESIAN_POINT('',(1.4,3.25,-5.06857864376269)) ;
#142319=CARTESIAN_POINT('Origin',(1.4,3.15,-8.87857864376269)) ;
#142320=CARTESIAN_POINT('',(1.5,3.25,-8.87857864376269)) ;
#142321=CARTESIAN_POINT('',(1.5,3.07928932188135,-8.94928932188134)) ;
#142322=CARTESIAN_POINT('Origin',(1.5,3.15,-8.87857864376269)) ;
#142323=CARTESIAN_POINT('',(1.4,3.07928932188135,-8.94928932188134)) ;
#142324=CARTESIAN_POINT('',(1.4,3.25,-8.87857864376269)) ;
#142325=CARTESIAN_POINT('Origin',(1.4,3.15,-12.6885786437627)) ;
#142326=CARTESIAN_POINT('',(1.5,3.25,-12.6885786437627)) ;
#142327=CARTESIAN_POINT('',(1.5,3.07928932188135,-12.7592893218813)) ;
#142328=CARTESIAN_POINT('Origin',(1.5,3.15,-12.6885786437627)) ;
#142329=CARTESIAN_POINT('',(1.4,3.07928932188135,-12.7592893218813)) ;
#142330=CARTESIAN_POINT('',(1.4,3.25,-12.6885786437627)) ;
#142331=CARTESIAN_POINT('Origin',(1.4,3.15,-16.4985786437627)) ;
#142332=CARTESIAN_POINT('',(1.5,3.25,-16.4985786437627)) ;
#142333=CARTESIAN_POINT('',(1.5,3.07928932188135,-16.5692893218813)) ;
#142334=CARTESIAN_POINT('Origin',(1.5,3.15,-16.4985786437627)) ;
#142335=CARTESIAN_POINT('',(1.4,3.07928932188135,-16.5692893218813)) ;
#142336=CARTESIAN_POINT('',(1.4,3.25,-16.4985786437627)) ;
#142337=CARTESIAN_POINT('Origin',(1.4,3.15,-20.3085786437627)) ;
#142338=CARTESIAN_POINT('',(1.5,3.25,-20.3085786437627)) ;
#142339=CARTESIAN_POINT('',(1.5,3.07928932188135,-20.3792893218813)) ;
#142340=CARTESIAN_POINT('Origin',(1.5,3.15,-20.3085786437627)) ;
#142341=CARTESIAN_POINT('',(1.4,3.07928932188135,-20.3792893218813)) ;
#142342=CARTESIAN_POINT('',(1.4,3.25,-20.3085786437627)) ;
#142343=CARTESIAN_POINT('Origin',(1.4,3.15,-24.1185786437627)) ;
#142344=CARTESIAN_POINT('',(1.5,3.25,-24.1185786437627)) ;
#142345=CARTESIAN_POINT('',(1.5,3.07928932188135,-24.1892893218813)) ;
#142346=CARTESIAN_POINT('Origin',(1.5,3.15,-24.1185786437627)) ;
#142347=CARTESIAN_POINT('',(1.4,3.07928932188135,-24.1892893218813)) ;
#142348=CARTESIAN_POINT('',(1.4,3.25,-24.1185786437627)) ;
#142349=CARTESIAN_POINT('Origin',(1.4,3.15,-27.9285786437627)) ;
#142350=CARTESIAN_POINT('',(1.5,3.25,-27.9285786437627)) ;
#142351=CARTESIAN_POINT('',(1.5,3.07928932188135,-27.9992893218813)) ;
#142352=CARTESIAN_POINT('Origin',(1.5,3.15,-27.9285786437627)) ;
#142353=CARTESIAN_POINT('',(1.4,3.07928932188135,-27.9992893218813)) ;
#142354=CARTESIAN_POINT('',(1.4,3.25,-27.9285786437627)) ;
#142355=CARTESIAN_POINT('Origin',(1.4,3.15,-31.7385786437627)) ;
#142356=CARTESIAN_POINT('',(1.5,3.25,-31.7385786437627)) ;
#142357=CARTESIAN_POINT('',(1.5,3.07928932188135,-31.8092893218813)) ;
#142358=CARTESIAN_POINT('Origin',(1.5,3.15,-31.7385786437627)) ;
#142359=CARTESIAN_POINT('',(1.4,3.07928932188135,-31.8092893218813)) ;
#142360=CARTESIAN_POINT('',(1.4,3.25,-31.7385786437627)) ;
#142361=CARTESIAN_POINT('Origin',(1.4,3.15,-35.5485786437627)) ;
#142362=CARTESIAN_POINT('',(1.5,3.25,-35.5485786437627)) ;
#142363=CARTESIAN_POINT('',(1.5,3.07928932188135,-35.6192893218813)) ;
#142364=CARTESIAN_POINT('Origin',(1.5,3.15,-35.5485786437627)) ;
#142365=CARTESIAN_POINT('',(1.4,3.07928932188135,-35.6192893218813)) ;
#142366=CARTESIAN_POINT('',(1.4,3.25,-35.5485786437627)) ;
#142367=CARTESIAN_POINT('Origin',(2.3,0.,0.)) ;
#142368=CARTESIAN_POINT('',(2.4,-1.10218211923262E-16,0.9)) ;
#142369=CARTESIAN_POINT('Origin',(2.4,0.,0.)) ;
#142370=CARTESIAN_POINT('',(2.3,-1.22464679914735E-16,1.)) ;
#142371=CARTESIAN_POINT('Origin',(2.3,-1.10218211923262E-16,0.9)) ;
#142372=CARTESIAN_POINT('',(2.3,1.22464679914735E-16,-1.)) ;
#142373=CARTESIAN_POINT('Origin',(2.3,0.,0.)) ;
#142374=CARTESIAN_POINT('Origin',(2.3,0.,0.)) ;
#142375=CARTESIAN_POINT('Origin',(7.9,3.15,-1.25857864376269)) ;
#142376=CARTESIAN_POINT('',(8.,3.35,-1.25857864376269)) ;
#142377=CARTESIAN_POINT('',(8.,3.00857864376269,-1.4)) ;
#142378=CARTESIAN_POINT('Origin',(8.,3.15,-1.25857864376269)) ;
#142379=CARTESIAN_POINT('',(7.9,3.25,-1.25857864376269)) ;
#142380=CARTESIAN_POINT('Origin',(7.9,3.35,-1.25857864376269)) ;
#142381=CARTESIAN_POINT('',(7.9,3.07928932188135,-1.32928932188135)) ;
#142382=CARTESIAN_POINT('Origin',(7.9,3.15,-1.25857864376269)) ;
#142383=CARTESIAN_POINT('Origin',(7.9,3.00857864376269,-1.4)) ;
#142384=CARTESIAN_POINT('Origin',(1.5,0.,0.)) ;
#142385=CARTESIAN_POINT('',(1.4,-1.34711147906209E-16,-1.1)) ;
#142386=CARTESIAN_POINT('Origin',(1.4,0.,0.)) ;
#142387=CARTESIAN_POINT('',(1.5,-1.22464679914735E-16,-1.)) ;
#142388=CARTESIAN_POINT('Origin',(1.5,-1.34711147906209E-16,-1.1)) ;
#142389=CARTESIAN_POINT('Origin',(1.5,0.,0.)) ;
#142390=CARTESIAN_POINT('Origin',(1.5,3.15,1.25857864376269)) ;
#142391=CARTESIAN_POINT('',(1.5,3.07928932188135,1.32928932188135)) ;
#142392=CARTESIAN_POINT('',(1.5,3.25,1.25857864376269)) ;
#142393=CARTESIAN_POINT('Origin',(1.5,3.15,1.25857864376269)) ;
#142394=CARTESIAN_POINT('',(1.4,3.15,1.25857864376269)) ;
#142395=CARTESIAN_POINT('Origin',(1.5,3.15,1.25857864376269)) ;
#142396=CARTESIAN_POINT('Origin',(1.5,3.15,1.25857864376269)) ;
#142397=CARTESIAN_POINT('Origin',(0.500000000000001,-4.5664044441154E-17,
-0.4)) ;
#142398=CARTESIAN_POINT('',(0.600000000000001,0.4,-0.4)) ;
#142399=CARTESIAN_POINT('',(0.595612997216081,0.370705721320403,-0.370705721320403)) ;
#142400=CARTESIAN_POINT('Origin',(0.499999999989667,0.400000000001553,-0.400000000001553)) ;
#142401=CARTESIAN_POINT('',(0.500000000000001,0.4,-0.5)) ;
#142402=CARTESIAN_POINT('Origin',(0.500000000000001,0.4,-0.4)) ;
#142403=CARTESIAN_POINT('',(0.500000000000001,-1.9,-0.5)) ;
#142404=CARTESIAN_POINT('',(0.500000000000001,0.5,-0.5)) ;
#142405=CARTESIAN_POINT('',(0.600000000000001,-1.9,-0.4)) ;
#142406=CARTESIAN_POINT('Origin',(0.500000000000001,-1.9,-0.4)) ;
#142407=CARTESIAN_POINT('',(0.600000000000001,-0.3,-0.4)) ;
#142408=CARTESIAN_POINT('',(0.600000000000001,-2.3980000991444E-17,-0.4)) ;
#142409=CARTESIAN_POINT('',(0.600000000000001,0.299999999999999,-0.4)) ;
#142410=CARTESIAN_POINT('',(0.600000000000001,-2.3980000991444E-17,-0.4)) ;
#142411=CARTESIAN_POINT('Ctrl Pts',(0.600000000000001,0.300000000000003,
-0.4)) ;
#142412=CARTESIAN_POINT('Ctrl Pts',(0.600000000000001,0.312243016306053,
-0.4)) ;
#142413=CARTESIAN_POINT('Ctrl Pts',(0.600069747422976,0.324350425899471,
-0.397751528521482)) ;
#142414=CARTESIAN_POINT('Ctrl Pts',(0.599517124288211,0.34619696929758,
-0.389395449060154)) ;
#142415=CARTESIAN_POINT('Ctrl Pts',(0.598927484301167,0.355857825373388,
-0.383675044722851)) ;
#142416=CARTESIAN_POINT('Ctrl Pts',(0.596766673872565,0.36653901230802,
-0.374702385109574)) ;
#142417=CARTESIAN_POINT('Ctrl Pts',(0.596235629104145,0.368676603883155,
-0.372737916809195)) ;
#142418=CARTESIAN_POINT('Ctrl Pts',(0.595612997216081,0.370705721320403,
-0.370705721320403)) ;
#142419=CARTESIAN_POINT('Origin',(2.4,0.,0.)) ;
#142420=CARTESIAN_POINT('',(2.4,-1.22464679914735E-16,-1.)) ;
#142421=CARTESIAN_POINT('Origin',(1.4,3.15,-1.25857864376269)) ;
#142422=CARTESIAN_POINT('',(1.5,3.25,-1.25857864376269)) ;
#142423=CARTESIAN_POINT('',(1.5,3.07928932188135,-1.32928932188135)) ;
#142424=CARTESIAN_POINT('Origin',(1.5,3.15,-1.25857864376269)) ;
#142425=CARTESIAN_POINT('',(1.4,3.07928932188135,-1.32928932188135)) ;
#142426=CARTESIAN_POINT('',(1.4,3.25,-1.25857864376269)) ;
#142427=CARTESIAN_POINT('Origin',(0.600000000000001,2.80617032878603E-17,
-34.29)) ;
#142428=CARTESIAN_POINT('',(0.600000000000001,-1.9,-33.89)) ;
#142429=CARTESIAN_POINT('',(0.600000000000001,-0.3,-33.89)) ;
#142430=CARTESIAN_POINT('',(0.600000000000001,-2.39800009914436E-17,-33.89)) ;
#142431=CARTESIAN_POINT('',(0.6,-0.4,-33.99)) ;
#142432=CARTESIAN_POINT('Origin',(0.6,-0.3,-33.99)) ;
#142433=CARTESIAN_POINT('',(0.6,-0.4,-34.59)) ;
#142434=CARTESIAN_POINT('',(0.6,-0.4,-33.89)) ;
#142435=CARTESIAN_POINT('Origin',(0.6,-0.3,-34.59)) ;
#142436=CARTESIAN_POINT('',(0.600000000000001,-2.1,-34.89)) ;
#142437=CARTESIAN_POINT('Origin',(0.600000000000001,-1.9,-34.89)) ;
#142438=CARTESIAN_POINT('',(0.600000000000001,-2.1,-35.565)) ;
#142439=CARTESIAN_POINT('',(0.600000000000001,-2.1,-34.29)) ;
#142440=CARTESIAN_POINT('',(0.600000000000001,-2.9,-35.565)) ;
#142441=CARTESIAN_POINT('',(0.600000000000001,-3.69904270612699E-17,-35.565)) ;
#142442=CARTESIAN_POINT('',(0.600000000000001,-2.9,-33.015)) ;
#142443=CARTESIAN_POINT('',(0.600000000000001,-2.9,-34.29)) ;
#142444=CARTESIAN_POINT('',(0.600000000000001,-2.1,-33.015)) ;
#142445=CARTESIAN_POINT('',(0.600000000000001,1.58165963986121E-16,-33.015)) ;
#142446=CARTESIAN_POINT('',(0.600000000000001,-2.1,-33.69)) ;
#142447=CARTESIAN_POINT('',(0.600000000000001,-2.1,-34.29)) ;
#142448=CARTESIAN_POINT('Origin',(0.600000000000001,-1.9,-33.69)) ;
#142449=CARTESIAN_POINT('Origin',(0.600000000000001,2.80617032878603E-17,
-30.48)) ;
#142450=CARTESIAN_POINT('',(0.600000000000001,-1.9,-30.08)) ;
#142451=CARTESIAN_POINT('',(0.600000000000001,-0.3,-30.08)) ;
#142452=CARTESIAN_POINT('',(0.600000000000001,-2.39800009914441E-17,-30.08)) ;
#142453=CARTESIAN_POINT('',(0.6,-0.4,-30.18)) ;
#142454=CARTESIAN_POINT('Origin',(0.6,-0.3,-30.18)) ;
#142455=CARTESIAN_POINT('',(0.6,-0.4,-30.78)) ;
#142456=CARTESIAN_POINT('',(0.6,-0.4,-30.08)) ;
#142457=CARTESIAN_POINT('Origin',(0.6,-0.3,-30.78)) ;
#142458=CARTESIAN_POINT('',(0.600000000000001,-2.1,-31.08)) ;
#142459=CARTESIAN_POINT('Origin',(0.600000000000001,-1.9,-31.08)) ;
#142460=CARTESIAN_POINT('',(0.600000000000001,-2.1,-31.755)) ;
#142461=CARTESIAN_POINT('',(0.600000000000001,-2.1,-30.48)) ;
#142462=CARTESIAN_POINT('',(0.600000000000001,-2.9,-31.755)) ;
#142463=CARTESIAN_POINT('',(0.600000000000001,-3.69904270612699E-17,-31.755)) ;
#142464=CARTESIAN_POINT('',(0.600000000000001,-2.9,-29.205)) ;
#142465=CARTESIAN_POINT('',(0.600000000000001,-2.9,-30.48)) ;
#142466=CARTESIAN_POINT('',(0.600000000000001,-2.1,-29.205)) ;
#142467=CARTESIAN_POINT('',(0.600000000000001,1.58165963986121E-16,-29.205)) ;
#142468=CARTESIAN_POINT('',(0.600000000000001,-2.1,-29.88)) ;
#142469=CARTESIAN_POINT('',(0.600000000000001,-2.1,-30.48)) ;
#142470=CARTESIAN_POINT('Origin',(0.600000000000001,-1.9,-29.88)) ;
#142471=CARTESIAN_POINT('Origin',(0.600000000000001,2.80617032878603E-17,
-26.67)) ;
#142472=CARTESIAN_POINT('',(0.600000000000001,-1.9,-26.27)) ;
#142473=CARTESIAN_POINT('',(0.600000000000001,-0.3,-26.27)) ;
#142474=CARTESIAN_POINT('',(0.600000000000001,-2.39800009914441E-17,-26.27)) ;
#142475=CARTESIAN_POINT('',(0.6,-0.4,-26.37)) ;
#142476=CARTESIAN_POINT('Origin',(0.6,-0.3,-26.37)) ;
#142477=CARTESIAN_POINT('',(0.6,-0.4,-26.97)) ;
#142478=CARTESIAN_POINT('',(0.6,-0.4,-26.27)) ;
#142479=CARTESIAN_POINT('Origin',(0.6,-0.3,-26.97)) ;
#142480=CARTESIAN_POINT('',(0.600000000000001,-2.1,-27.27)) ;
#142481=CARTESIAN_POINT('Origin',(0.600000000000001,-1.9,-27.27)) ;
#142482=CARTESIAN_POINT('',(0.600000000000001,-2.1,-27.945)) ;
#142483=CARTESIAN_POINT('',(0.600000000000001,-2.1,-26.67)) ;
#142484=CARTESIAN_POINT('',(0.600000000000001,-2.9,-27.945)) ;
#142485=CARTESIAN_POINT('',(0.600000000000001,-3.69904270612701E-17,-27.945)) ;
#142486=CARTESIAN_POINT('',(0.600000000000001,-2.9,-25.395)) ;
#142487=CARTESIAN_POINT('',(0.600000000000001,-2.9,-26.67)) ;
#142488=CARTESIAN_POINT('',(0.600000000000001,-2.1,-25.395)) ;
#142489=CARTESIAN_POINT('',(0.600000000000001,1.58165963986121E-16,-25.395)) ;
#142490=CARTESIAN_POINT('',(0.600000000000001,-2.1,-26.07)) ;
#142491=CARTESIAN_POINT('',(0.600000000000001,-2.1,-26.67)) ;
#142492=CARTESIAN_POINT('Origin',(0.600000000000001,-1.9,-26.07)) ;
#142493=CARTESIAN_POINT('Origin',(0.600000000000001,2.80617032878603E-17,
-22.86)) ;
#142494=CARTESIAN_POINT('',(0.600000000000001,-1.9,-22.46)) ;
#142495=CARTESIAN_POINT('',(0.600000000000001,-0.3,-22.46)) ;
#142496=CARTESIAN_POINT('',(0.600000000000001,-2.39800009914441E-17,-22.46)) ;
#142497=CARTESIAN_POINT('',(0.6,-0.4,-22.56)) ;
#142498=CARTESIAN_POINT('Origin',(0.6,-0.3,-22.56)) ;
#142499=CARTESIAN_POINT('',(0.6,-0.4,-23.16)) ;
#142500=CARTESIAN_POINT('',(0.6,-0.4,-22.46)) ;
#142501=CARTESIAN_POINT('Origin',(0.6,-0.3,-23.16)) ;
#142502=CARTESIAN_POINT('',(0.600000000000001,-2.1,-23.46)) ;
#142503=CARTESIAN_POINT('Origin',(0.600000000000001,-1.9,-23.46)) ;
#142504=CARTESIAN_POINT('',(0.600000000000001,-2.1,-24.135)) ;
#142505=CARTESIAN_POINT('',(0.600000000000001,-2.1,-22.86)) ;
#142506=CARTESIAN_POINT('',(0.600000000000001,-2.9,-24.135)) ;
#142507=CARTESIAN_POINT('',(0.600000000000001,-3.69904270612701E-17,-24.135)) ;
#142508=CARTESIAN_POINT('',(0.600000000000001,-2.9,-21.585)) ;
#142509=CARTESIAN_POINT('',(0.600000000000001,-2.9,-22.86)) ;
#142510=CARTESIAN_POINT('',(0.600000000000001,-2.1,-21.585)) ;
#142511=CARTESIAN_POINT('',(0.600000000000001,1.58165963986121E-16,-21.585)) ;
#142512=CARTESIAN_POINT('',(0.600000000000001,-2.1,-22.26)) ;
#142513=CARTESIAN_POINT('',(0.600000000000001,-2.1,-22.86)) ;
#142514=CARTESIAN_POINT('Origin',(0.600000000000001,-1.9,-22.26)) ;
#142515=CARTESIAN_POINT('Origin',(0.600000000000001,2.80617032878603E-17,
-19.05)) ;
#142516=CARTESIAN_POINT('',(0.600000000000001,-1.9,-18.65)) ;
#142517=CARTESIAN_POINT('',(0.600000000000001,-0.3,-18.65)) ;
#142518=CARTESIAN_POINT('',(0.600000000000001,-2.39800009914441E-17,-18.65)) ;
#142519=CARTESIAN_POINT('',(0.6,-0.4,-18.75)) ;
#142520=CARTESIAN_POINT('Origin',(0.6,-0.3,-18.75)) ;
#142521=CARTESIAN_POINT('',(0.6,-0.4,-19.35)) ;
#142522=CARTESIAN_POINT('',(0.6,-0.4,-18.65)) ;
#142523=CARTESIAN_POINT('Origin',(0.6,-0.3,-19.35)) ;
#142524=CARTESIAN_POINT('',(0.600000000000001,-2.1,-19.65)) ;
#142525=CARTESIAN_POINT('Origin',(0.600000000000001,-1.9,-19.65)) ;
#142526=CARTESIAN_POINT('',(0.600000000000001,-2.1,-20.325)) ;
#142527=CARTESIAN_POINT('',(0.600000000000001,-2.1,-19.05)) ;
#142528=CARTESIAN_POINT('',(0.600000000000001,-2.9,-20.325)) ;
#142529=CARTESIAN_POINT('',(0.600000000000001,-3.69904270612701E-17,-20.325)) ;
#142530=CARTESIAN_POINT('',(0.600000000000001,-2.9,-17.775)) ;
#142531=CARTESIAN_POINT('',(0.600000000000001,-2.9,-19.05)) ;
#142532=CARTESIAN_POINT('',(0.600000000000001,-2.1,-17.775)) ;
#142533=CARTESIAN_POINT('',(0.600000000000001,1.58165963986121E-16,-17.775)) ;
#142534=CARTESIAN_POINT('',(0.600000000000001,-2.1,-18.45)) ;
#142535=CARTESIAN_POINT('',(0.600000000000001,-2.1,-19.05)) ;
#142536=CARTESIAN_POINT('Origin',(0.600000000000001,-1.9,-18.45)) ;
#142537=CARTESIAN_POINT('Origin',(0.600000000000001,2.80617032878603E-17,
-15.24)) ;
#142538=CARTESIAN_POINT('',(0.600000000000001,-1.9,-14.84)) ;
#142539=CARTESIAN_POINT('',(0.600000000000001,-0.3,-14.84)) ;
#142540=CARTESIAN_POINT('',(0.600000000000001,-2.39800009914441E-17,-14.84)) ;
#142541=CARTESIAN_POINT('',(0.6,-0.4,-14.94)) ;
#142542=CARTESIAN_POINT('Origin',(0.6,-0.3,-14.94)) ;
#142543=CARTESIAN_POINT('',(0.6,-0.4,-15.54)) ;
#142544=CARTESIAN_POINT('',(0.6,-0.4,-14.84)) ;
#142545=CARTESIAN_POINT('Origin',(0.6,-0.3,-15.54)) ;
#142546=CARTESIAN_POINT('',(0.600000000000001,-2.1,-15.84)) ;
#142547=CARTESIAN_POINT('Origin',(0.600000000000001,-1.9,-15.84)) ;
#142548=CARTESIAN_POINT('',(0.600000000000001,-2.1,-16.515)) ;
#142549=CARTESIAN_POINT('',(0.600000000000001,-2.1,-15.24)) ;
#142550=CARTESIAN_POINT('',(0.600000000000001,-2.9,-16.515)) ;
#142551=CARTESIAN_POINT('',(0.600000000000001,-3.69904270612701E-17,-16.515)) ;
#142552=CARTESIAN_POINT('',(0.600000000000001,-2.9,-13.965)) ;
#142553=CARTESIAN_POINT('',(0.600000000000001,-2.9,-15.24)) ;
#142554=CARTESIAN_POINT('',(0.600000000000001,-2.1,-13.965)) ;
#142555=CARTESIAN_POINT('',(0.600000000000001,1.58165963986121E-16,-13.965)) ;
#142556=CARTESIAN_POINT('',(0.600000000000001,-2.1,-14.64)) ;
#142557=CARTESIAN_POINT('',(0.600000000000001,-2.1,-15.24)) ;
#142558=CARTESIAN_POINT('Origin',(0.600000000000001,-1.9,-14.64)) ;
#142559=CARTESIAN_POINT('Origin',(0.600000000000001,2.80617032878603E-17,
-11.43)) ;
#142560=CARTESIAN_POINT('',(0.600000000000001,-1.9,-11.03)) ;
#142561=CARTESIAN_POINT('',(0.600000000000001,-0.3,-11.03)) ;
#142562=CARTESIAN_POINT('',(0.600000000000001,-2.39800009914441E-17,-11.03)) ;
#142563=CARTESIAN_POINT('',(0.6,-0.4,-11.13)) ;
#142564=CARTESIAN_POINT('Origin',(0.6,-0.3,-11.13)) ;
#142565=CARTESIAN_POINT('',(0.6,-0.4,-11.73)) ;
#142566=CARTESIAN_POINT('',(0.6,-0.4,-11.03)) ;
#142567=CARTESIAN_POINT('Origin',(0.6,-0.3,-11.73)) ;
#142568=CARTESIAN_POINT('',(0.600000000000001,-2.1,-12.03)) ;
#142569=CARTESIAN_POINT('Origin',(0.600000000000001,-1.9,-12.03)) ;
#142570=CARTESIAN_POINT('',(0.600000000000001,-2.1,-12.705)) ;
#142571=CARTESIAN_POINT('',(0.600000000000001,-2.1,-11.43)) ;
#142572=CARTESIAN_POINT('',(0.600000000000001,-2.9,-12.705)) ;
#142573=CARTESIAN_POINT('',(0.600000000000001,-3.69904270612701E-17,-12.705)) ;
#142574=CARTESIAN_POINT('',(0.600000000000001,-2.9,-10.155)) ;
#142575=CARTESIAN_POINT('',(0.600000000000001,-2.9,-11.43)) ;
#142576=CARTESIAN_POINT('',(0.600000000000001,-2.1,-10.155)) ;
#142577=CARTESIAN_POINT('',(0.600000000000001,1.58165963986121E-16,-10.155)) ;
#142578=CARTESIAN_POINT('',(0.600000000000001,-2.1,-10.83)) ;
#142579=CARTESIAN_POINT('',(0.600000000000001,-2.1,-11.43)) ;
#142580=CARTESIAN_POINT('Origin',(0.600000000000001,-1.9,-10.83)) ;
#142581=CARTESIAN_POINT('Origin',(0.600000000000001,2.80617032878603E-17,
-7.62)) ;
#142582=CARTESIAN_POINT('',(0.600000000000001,-1.9,-7.22)) ;
#142583=CARTESIAN_POINT('',(0.600000000000001,-0.3,-7.22)) ;
#142584=CARTESIAN_POINT('',(0.600000000000001,-2.39800009914439E-17,-7.22)) ;
#142585=CARTESIAN_POINT('',(0.6,-0.4,-7.32)) ;
#142586=CARTESIAN_POINT('Origin',(0.6,-0.3,-7.32)) ;
#142587=CARTESIAN_POINT('',(0.6,-0.4,-7.92)) ;
#142588=CARTESIAN_POINT('',(0.6,-0.4,-7.22)) ;
#142589=CARTESIAN_POINT('Origin',(0.6,-0.3,-7.92)) ;
#142590=CARTESIAN_POINT('',(0.600000000000001,-2.1,-8.22)) ;
#142591=CARTESIAN_POINT('Origin',(0.600000000000001,-1.9,-8.22)) ;
#142592=CARTESIAN_POINT('',(0.600000000000001,-2.1,-8.895)) ;
#142593=CARTESIAN_POINT('',(0.600000000000001,-2.1,-7.62)) ;
#142594=CARTESIAN_POINT('',(0.600000000000001,-2.9,-8.895)) ;
#142595=CARTESIAN_POINT('',(0.600000000000001,-3.69904270612701E-17,-8.895)) ;
#142596=CARTESIAN_POINT('',(0.600000000000001,-2.9,-6.345)) ;
#142597=CARTESIAN_POINT('',(0.600000000000001,-2.9,-7.62)) ;
#142598=CARTESIAN_POINT('',(0.600000000000001,-2.1,-6.345)) ;
#142599=CARTESIAN_POINT('',(0.600000000000001,1.58165963986121E-16,-6.345)) ;
#142600=CARTESIAN_POINT('',(0.600000000000001,-2.1,-7.02)) ;
#142601=CARTESIAN_POINT('',(0.600000000000001,-2.1,-7.62)) ;
#142602=CARTESIAN_POINT('Origin',(0.600000000000001,-1.9,-7.02)) ;
#142603=CARTESIAN_POINT('Origin',(0.600000000000001,2.80617032878603E-17,
-3.81)) ;
#142604=CARTESIAN_POINT('',(0.600000000000001,-1.9,-3.41)) ;
#142605=CARTESIAN_POINT('',(0.600000000000001,-0.3,-3.41)) ;
#142606=CARTESIAN_POINT('',(0.600000000000001,-2.3980000991444E-17,-3.41)) ;
#142607=CARTESIAN_POINT('',(0.6,-0.4,-3.51)) ;
#142608=CARTESIAN_POINT('Origin',(0.6,-0.3,-3.51)) ;
#142609=CARTESIAN_POINT('',(0.6,-0.4,-4.11)) ;
#142610=CARTESIAN_POINT('',(0.6,-0.4,-3.41)) ;
#142611=CARTESIAN_POINT('Origin',(0.6,-0.3,-4.11)) ;
#142612=CARTESIAN_POINT('',(0.600000000000001,-2.1,-4.41)) ;
#142613=CARTESIAN_POINT('Origin',(0.600000000000001,-1.9,-4.41)) ;
#142614=CARTESIAN_POINT('',(0.600000000000001,-2.1,-5.085)) ;
#142615=CARTESIAN_POINT('',(0.600000000000001,-2.1,-3.81)) ;
#142616=CARTESIAN_POINT('',(0.600000000000001,-2.9,-5.085)) ;
#142617=CARTESIAN_POINT('',(0.600000000000001,-3.699042706127E-17,-5.085)) ;
#142618=CARTESIAN_POINT('',(0.600000000000001,-2.9,-2.535)) ;
#142619=CARTESIAN_POINT('',(0.600000000000001,-2.9,-3.81)) ;
#142620=CARTESIAN_POINT('',(0.600000000000001,-2.1,-2.535)) ;
#142621=CARTESIAN_POINT('',(0.600000000000001,1.58165963986121E-16,-2.535)) ;
#142622=CARTESIAN_POINT('',(0.600000000000001,-2.1,-3.21)) ;
#142623=CARTESIAN_POINT('',(0.600000000000001,-2.1,-3.81)) ;
#142624=CARTESIAN_POINT('Origin',(0.600000000000001,-1.9,-3.21)) ;
#142625=CARTESIAN_POINT('Origin',(-0.999999999999999,1.25,-35.665)) ;
#142626=CARTESIAN_POINT('',(-1.1,-1.9,-35.665)) ;
#142627=CARTESIAN_POINT('',(-0.899999999999999,-2.1,-35.665)) ;
#142628=CARTESIAN_POINT('Origin',(-0.899999999999999,-1.9,-35.665)) ;
#142629=CARTESIAN_POINT('',(-1.1,-2.9,-35.665)) ;
#142630=CARTESIAN_POINT('',(-1.1,-2.9,-35.665)) ;
#142631=CARTESIAN_POINT('',(0.500000000000001,-2.9,-35.665)) ;
#142632=CARTESIAN_POINT('',(0.600000000000001,-2.9,-35.665)) ;
#142633=CARTESIAN_POINT('',(0.500000000000001,-2.1,-35.665)) ;
#142634=CARTESIAN_POINT('',(0.5,1.25,-35.665)) ;
#142635=CARTESIAN_POINT('',(-0.999999999999999,-2.1,-35.665)) ;
#142636=CARTESIAN_POINT('Origin',(-0.999999999999999,1.25,-32.915)) ;
#142637=CARTESIAN_POINT('',(-0.899999999999999,-2.1,-32.915)) ;
#142638=CARTESIAN_POINT('',(-1.1,-1.9,-32.915)) ;
#142639=CARTESIAN_POINT('Origin',(-0.899999999999999,-1.9,-32.915)) ;
#142640=CARTESIAN_POINT('',(0.500000000000001,-2.1,-32.915)) ;
#142641=CARTESIAN_POINT('',(0.600000000000001,-2.1,-32.915)) ;
#142642=CARTESIAN_POINT('',(0.500000000000001,-2.9,-32.915)) ;
#142643=CARTESIAN_POINT('',(0.5,1.25,-32.915)) ;
#142644=CARTESIAN_POINT('',(-1.1,-2.9,-32.915)) ;
#142645=CARTESIAN_POINT('',(-1.1,-2.9,-32.915)) ;
#142646=CARTESIAN_POINT('',(-1.1,1.25,-32.915)) ;
#142647=CARTESIAN_POINT('Origin',(-0.999999999999999,1.25,-31.855)) ;
#142648=CARTESIAN_POINT('',(-1.1,-1.9,-31.855)) ;
#142649=CARTESIAN_POINT('',(-0.899999999999999,-2.1,-31.855)) ;
#142650=CARTESIAN_POINT('Origin',(-0.899999999999999,-1.9,-31.855)) ;
#142651=CARTESIAN_POINT('',(-1.1,-2.9,-31.855)) ;
#142652=CARTESIAN_POINT('',(-1.1,-2.9,-31.855)) ;
#142653=CARTESIAN_POINT('',(0.500000000000001,-2.9,-31.855)) ;
#142654=CARTESIAN_POINT('',(0.600000000000001,-2.9,-31.855)) ;
#142655=CARTESIAN_POINT('',(0.500000000000001,-2.1,-31.855)) ;
#142656=CARTESIAN_POINT('',(0.5,1.25,-31.855)) ;
#142657=CARTESIAN_POINT('',(-0.999999999999999,-2.1,-31.855)) ;
#142658=CARTESIAN_POINT('Origin',(-0.999999999999999,1.25,-29.105)) ;
#142659=CARTESIAN_POINT('',(-0.899999999999999,-2.1,-29.105)) ;
#142660=CARTESIAN_POINT('',(-1.1,-1.9,-29.105)) ;
#142661=CARTESIAN_POINT('Origin',(-0.899999999999999,-1.9,-29.105)) ;
#142662=CARTESIAN_POINT('',(0.500000000000001,-2.1,-29.105)) ;
#142663=CARTESIAN_POINT('',(0.600000000000001,-2.1,-29.105)) ;
#142664=CARTESIAN_POINT('',(0.500000000000001,-2.9,-29.105)) ;
#142665=CARTESIAN_POINT('',(0.5,1.25,-29.105)) ;
#142666=CARTESIAN_POINT('',(-1.1,-2.9,-29.105)) ;
#142667=CARTESIAN_POINT('',(-1.1,-2.9,-29.105)) ;
#142668=CARTESIAN_POINT('',(-1.1,1.25,-29.105)) ;
#142669=CARTESIAN_POINT('Origin',(-0.999999999999999,1.25,-28.045)) ;
#142670=CARTESIAN_POINT('',(-1.1,-1.9,-28.045)) ;
#142671=CARTESIAN_POINT('',(-0.899999999999999,-2.1,-28.045)) ;
#142672=CARTESIAN_POINT('Origin',(-0.899999999999999,-1.9,-28.045)) ;
#142673=CARTESIAN_POINT('',(-1.1,-2.9,-28.045)) ;
#142674=CARTESIAN_POINT('',(-1.1,-2.9,-28.045)) ;
#142675=CARTESIAN_POINT('',(0.500000000000001,-2.9,-28.045)) ;
#142676=CARTESIAN_POINT('',(0.600000000000001,-2.9,-28.045)) ;
#142677=CARTESIAN_POINT('',(0.500000000000001,-2.1,-28.045)) ;
#142678=CARTESIAN_POINT('',(0.5,1.25,-28.045)) ;
#142679=CARTESIAN_POINT('',(-0.999999999999999,-2.1,-28.045)) ;
#142680=CARTESIAN_POINT('Origin',(-0.999999999999999,1.25,-25.295)) ;
#142681=CARTESIAN_POINT('',(-0.899999999999999,-2.1,-25.295)) ;
#142682=CARTESIAN_POINT('',(-1.1,-1.9,-25.295)) ;
#142683=CARTESIAN_POINT('Origin',(-0.899999999999999,-1.9,-25.295)) ;
#142684=CARTESIAN_POINT('',(0.500000000000001,-2.1,-25.295)) ;
#142685=CARTESIAN_POINT('',(0.600000000000001,-2.1,-25.295)) ;
#142686=CARTESIAN_POINT('',(0.500000000000001,-2.9,-25.295)) ;
#142687=CARTESIAN_POINT('',(0.5,1.25,-25.295)) ;
#142688=CARTESIAN_POINT('',(-1.1,-2.9,-25.295)) ;
#142689=CARTESIAN_POINT('',(-1.1,-2.9,-25.295)) ;
#142690=CARTESIAN_POINT('',(-1.1,1.25,-25.295)) ;
#142691=CARTESIAN_POINT('Origin',(-0.999999999999999,1.25,-24.235)) ;
#142692=CARTESIAN_POINT('',(-1.1,-1.9,-24.235)) ;
#142693=CARTESIAN_POINT('',(-0.899999999999999,-2.1,-24.235)) ;
#142694=CARTESIAN_POINT('Origin',(-0.899999999999999,-1.9,-24.235)) ;
#142695=CARTESIAN_POINT('',(-1.1,-2.9,-24.235)) ;
#142696=CARTESIAN_POINT('',(-1.1,-2.9,-24.235)) ;
#142697=CARTESIAN_POINT('',(0.500000000000001,-2.9,-24.235)) ;
#142698=CARTESIAN_POINT('',(0.600000000000001,-2.9,-24.235)) ;
#142699=CARTESIAN_POINT('',(0.500000000000001,-2.1,-24.235)) ;
#142700=CARTESIAN_POINT('',(0.5,1.25,-24.235)) ;
#142701=CARTESIAN_POINT('',(-0.999999999999999,-2.1,-24.235)) ;
#142702=CARTESIAN_POINT('Origin',(-0.999999999999999,1.25,-21.485)) ;
#142703=CARTESIAN_POINT('',(-0.899999999999999,-2.1,-21.485)) ;
#142704=CARTESIAN_POINT('',(-1.1,-1.9,-21.485)) ;
#142705=CARTESIAN_POINT('Origin',(-0.899999999999999,-1.9,-21.485)) ;
#142706=CARTESIAN_POINT('',(0.500000000000001,-2.1,-21.485)) ;
#142707=CARTESIAN_POINT('',(0.600000000000001,-2.1,-21.485)) ;
#142708=CARTESIAN_POINT('',(0.500000000000001,-2.9,-21.485)) ;
#142709=CARTESIAN_POINT('',(0.5,1.25,-21.485)) ;
#142710=CARTESIAN_POINT('',(-1.1,-2.9,-21.485)) ;
#142711=CARTESIAN_POINT('',(-1.1,-2.9,-21.485)) ;
#142712=CARTESIAN_POINT('',(-1.1,1.25,-21.485)) ;
#142713=CARTESIAN_POINT('Origin',(-0.999999999999999,1.25,-20.425)) ;
#142714=CARTESIAN_POINT('',(-1.1,-1.9,-20.425)) ;
#142715=CARTESIAN_POINT('',(-0.899999999999999,-2.1,-20.425)) ;
#142716=CARTESIAN_POINT('Origin',(-0.899999999999999,-1.9,-20.425)) ;
#142717=CARTESIAN_POINT('',(-1.1,-2.9,-20.425)) ;
#142718=CARTESIAN_POINT('',(-1.1,-2.9,-20.425)) ;
#142719=CARTESIAN_POINT('',(0.500000000000001,-2.9,-20.425)) ;
#142720=CARTESIAN_POINT('',(0.600000000000001,-2.9,-20.425)) ;
#142721=CARTESIAN_POINT('',(0.500000000000001,-2.1,-20.425)) ;
#142722=CARTESIAN_POINT('',(0.5,1.25,-20.425)) ;
#142723=CARTESIAN_POINT('',(-0.999999999999999,-2.1,-20.425)) ;
#142724=CARTESIAN_POINT('Origin',(-0.999999999999999,1.25,-17.675)) ;
#142725=CARTESIAN_POINT('',(-0.899999999999999,-2.1,-17.675)) ;
#142726=CARTESIAN_POINT('',(-1.1,-1.9,-17.675)) ;
#142727=CARTESIAN_POINT('Origin',(-0.899999999999999,-1.9,-17.675)) ;
#142728=CARTESIAN_POINT('',(0.500000000000001,-2.1,-17.675)) ;
#142729=CARTESIAN_POINT('',(0.600000000000001,-2.1,-17.675)) ;
#142730=CARTESIAN_POINT('',(0.500000000000001,-2.9,-17.675)) ;
#142731=CARTESIAN_POINT('',(0.5,1.25,-17.675)) ;
#142732=CARTESIAN_POINT('',(-1.1,-2.9,-17.675)) ;
#142733=CARTESIAN_POINT('',(-1.1,-2.9,-17.675)) ;
#142734=CARTESIAN_POINT('',(-1.1,1.25,-17.675)) ;
#142735=CARTESIAN_POINT('Origin',(-0.999999999999999,1.25,-16.615)) ;
#142736=CARTESIAN_POINT('',(-1.1,-1.9,-16.615)) ;
#142737=CARTESIAN_POINT('',(-0.899999999999999,-2.1,-16.615)) ;
#142738=CARTESIAN_POINT('Origin',(-0.899999999999999,-1.9,-16.615)) ;
#142739=CARTESIAN_POINT('',(-1.1,-2.9,-16.615)) ;
#142740=CARTESIAN_POINT('',(-1.1,-2.9,-16.615)) ;
#142741=CARTESIAN_POINT('',(0.500000000000001,-2.9,-16.615)) ;
#142742=CARTESIAN_POINT('',(0.600000000000001,-2.9,-16.615)) ;
#142743=CARTESIAN_POINT('',(0.500000000000001,-2.1,-16.615)) ;
#142744=CARTESIAN_POINT('',(0.5,1.25,-16.615)) ;
#142745=CARTESIAN_POINT('',(-0.999999999999999,-2.1,-16.615)) ;
#142746=CARTESIAN_POINT('Origin',(-0.999999999999999,1.25,-13.865)) ;
#142747=CARTESIAN_POINT('',(-0.899999999999999,-2.1,-13.865)) ;
#142748=CARTESIAN_POINT('',(-1.1,-1.9,-13.865)) ;
#142749=CARTESIAN_POINT('Origin',(-0.899999999999999,-1.9,-13.865)) ;
#142750=CARTESIAN_POINT('',(0.500000000000001,-2.1,-13.865)) ;
#142751=CARTESIAN_POINT('',(0.600000000000001,-2.1,-13.865)) ;
#142752=CARTESIAN_POINT('',(0.500000000000001,-2.9,-13.865)) ;
#142753=CARTESIAN_POINT('',(0.5,1.25,-13.865)) ;
#142754=CARTESIAN_POINT('',(-1.1,-2.9,-13.865)) ;
#142755=CARTESIAN_POINT('',(-1.1,-2.9,-13.865)) ;
#142756=CARTESIAN_POINT('',(-1.1,1.25,-13.865)) ;
#142757=CARTESIAN_POINT('Origin',(-0.999999999999999,1.25,-12.805)) ;
#142758=CARTESIAN_POINT('',(-1.1,-1.9,-12.805)) ;
#142759=CARTESIAN_POINT('',(-0.899999999999999,-2.1,-12.805)) ;
#142760=CARTESIAN_POINT('Origin',(-0.899999999999999,-1.9,-12.805)) ;
#142761=CARTESIAN_POINT('',(-1.1,-2.9,-12.805)) ;
#142762=CARTESIAN_POINT('',(-1.1,-2.9,-12.805)) ;
#142763=CARTESIAN_POINT('',(0.500000000000001,-2.9,-12.805)) ;
#142764=CARTESIAN_POINT('',(0.600000000000001,-2.9,-12.805)) ;
#142765=CARTESIAN_POINT('',(0.500000000000001,-2.1,-12.805)) ;
#142766=CARTESIAN_POINT('',(0.5,1.25,-12.805)) ;
#142767=CARTESIAN_POINT('',(-0.999999999999999,-2.1,-12.805)) ;
#142768=CARTESIAN_POINT('Origin',(-0.999999999999999,1.25,-10.055)) ;
#142769=CARTESIAN_POINT('',(-0.899999999999999,-2.1,-10.055)) ;
#142770=CARTESIAN_POINT('',(-1.1,-1.9,-10.055)) ;
#142771=CARTESIAN_POINT('Origin',(-0.899999999999999,-1.9,-10.055)) ;
#142772=CARTESIAN_POINT('',(0.500000000000001,-2.1,-10.055)) ;
#142773=CARTESIAN_POINT('',(0.600000000000001,-2.1,-10.055)) ;
#142774=CARTESIAN_POINT('',(0.500000000000001,-2.9,-10.055)) ;
#142775=CARTESIAN_POINT('',(0.5,1.25,-10.055)) ;
#142776=CARTESIAN_POINT('',(-1.1,-2.9,-10.055)) ;
#142777=CARTESIAN_POINT('',(-1.1,-2.9,-10.055)) ;
#142778=CARTESIAN_POINT('',(-1.1,1.25,-10.055)) ;
#142779=CARTESIAN_POINT('Origin',(-0.999999999999999,1.25,-8.995)) ;
#142780=CARTESIAN_POINT('',(-1.1,-1.9,-8.995)) ;
#142781=CARTESIAN_POINT('',(-0.899999999999999,-2.1,-8.995)) ;
#142782=CARTESIAN_POINT('Origin',(-0.899999999999999,-1.9,-8.995)) ;
#142783=CARTESIAN_POINT('',(-1.1,-2.9,-8.995)) ;
#142784=CARTESIAN_POINT('',(-1.1,-2.9,-8.995)) ;
#142785=CARTESIAN_POINT('',(0.500000000000001,-2.9,-8.995)) ;
#142786=CARTESIAN_POINT('',(0.600000000000001,-2.9,-8.995)) ;
#142787=CARTESIAN_POINT('',(0.500000000000001,-2.1,-8.995)) ;
#142788=CARTESIAN_POINT('',(0.5,1.25,-8.995)) ;
#142789=CARTESIAN_POINT('',(-0.999999999999999,-2.1,-8.995)) ;
#142790=CARTESIAN_POINT('Origin',(-0.999999999999999,1.25,-6.245)) ;
#142791=CARTESIAN_POINT('',(-0.899999999999999,-2.1,-6.245)) ;
#142792=CARTESIAN_POINT('',(-1.1,-1.9,-6.245)) ;
#142793=CARTESIAN_POINT('Origin',(-0.899999999999999,-1.9,-6.245)) ;
#142794=CARTESIAN_POINT('',(0.500000000000001,-2.1,-6.245)) ;
#142795=CARTESIAN_POINT('',(0.600000000000001,-2.1,-6.245)) ;
#142796=CARTESIAN_POINT('',(0.500000000000001,-2.9,-6.245)) ;
#142797=CARTESIAN_POINT('',(0.5,1.25,-6.245)) ;
#142798=CARTESIAN_POINT('',(-1.1,-2.9,-6.245)) ;
#142799=CARTESIAN_POINT('',(-1.1,-2.9,-6.245)) ;
#142800=CARTESIAN_POINT('',(-1.1,1.25,-6.245)) ;
#142801=CARTESIAN_POINT('Origin',(-0.999999999999999,1.25,-5.185)) ;
#142802=CARTESIAN_POINT('',(-1.1,-1.9,-5.185)) ;
#142803=CARTESIAN_POINT('',(-0.899999999999999,-2.1,-5.185)) ;
#142804=CARTESIAN_POINT('Origin',(-0.899999999999999,-1.9,-5.185)) ;
#142805=CARTESIAN_POINT('',(-1.1,-2.9,-5.185)) ;
#142806=CARTESIAN_POINT('',(-1.1,-2.9,-5.185)) ;
#142807=CARTESIAN_POINT('',(0.500000000000001,-2.9,-5.185)) ;
#142808=CARTESIAN_POINT('',(0.600000000000001,-2.9,-5.185)) ;
#142809=CARTESIAN_POINT('',(0.500000000000001,-2.1,-5.185)) ;
#142810=CARTESIAN_POINT('',(0.5,1.25,-5.185)) ;
#142811=CARTESIAN_POINT('',(-0.999999999999999,-2.1,-5.185)) ;
#142812=CARTESIAN_POINT('Origin',(-0.999999999999999,1.25,-2.435)) ;
#142813=CARTESIAN_POINT('',(-0.899999999999999,-2.1,-2.435)) ;
#142814=CARTESIAN_POINT('',(-1.1,-1.9,-2.435)) ;
#142815=CARTESIAN_POINT('Origin',(-0.899999999999999,-1.9,-2.435)) ;
#142816=CARTESIAN_POINT('',(0.500000000000001,-2.1,-2.435)) ;
#142817=CARTESIAN_POINT('',(0.600000000000001,-2.1,-2.435)) ;
#142818=CARTESIAN_POINT('',(0.500000000000001,-2.9,-2.435)) ;
#142819=CARTESIAN_POINT('',(0.5,1.25,-2.435)) ;
#142820=CARTESIAN_POINT('',(-1.1,-2.9,-2.435)) ;
#142821=CARTESIAN_POINT('',(-1.1,-2.9,-2.435)) ;
#142822=CARTESIAN_POINT('',(-1.1,1.25,-2.435)) ;
#142823=CARTESIAN_POINT('Origin',(-1.1,-2.9,-36.89)) ;
#142824=CARTESIAN_POINT('',(-1.2,-2.9,-2.335)) ;
#142825=CARTESIAN_POINT('',(-1.2,-2.9,-1.475)) ;
#142826=CARTESIAN_POINT('',(-1.2,-2.9,-36.89)) ;
#142827=CARTESIAN_POINT('',(-1.1,-3.,-2.335)) ;
#142828=CARTESIAN_POINT('Origin',(-1.1,-2.9,-2.335)) ;
#142829=CARTESIAN_POINT('',(-1.1,-3.,-1.475)) ;
#142830=CARTESIAN_POINT('',(-1.1,-3.,-36.89)) ;
#142831=CARTESIAN_POINT('Origin',(-1.1,-2.9,-1.475)) ;
#142832=CARTESIAN_POINT('Origin',(-1.1,-2.9,-36.89)) ;
#142833=CARTESIAN_POINT('',(-1.2,-2.9,-6.145)) ;
#142834=CARTESIAN_POINT('',(-1.2,-2.9,-5.285)) ;
#142835=CARTESIAN_POINT('',(-1.2,-2.9,-36.89)) ;
#142836=CARTESIAN_POINT('',(-1.1,-3.,-6.145)) ;
#142837=CARTESIAN_POINT('Origin',(-1.1,-2.9,-6.145)) ;
#142838=CARTESIAN_POINT('',(-1.1,-3.,-5.285)) ;
#142839=CARTESIAN_POINT('',(-1.1,-3.,-36.89)) ;
#142840=CARTESIAN_POINT('Origin',(-1.1,-2.9,-5.285)) ;
#142841=CARTESIAN_POINT('Origin',(-1.1,-2.9,-36.89)) ;
#142842=CARTESIAN_POINT('',(-1.2,-2.9,-9.955)) ;
#142843=CARTESIAN_POINT('',(-1.2,-2.9,-9.095)) ;
#142844=CARTESIAN_POINT('',(-1.2,-2.9,-36.89)) ;
#142845=CARTESIAN_POINT('',(-1.1,-3.,-9.955)) ;
#142846=CARTESIAN_POINT('Origin',(-1.1,-2.9,-9.955)) ;
#142847=CARTESIAN_POINT('',(-1.1,-3.,-9.095)) ;
#142848=CARTESIAN_POINT('',(-1.1,-3.,-36.89)) ;
#142849=CARTESIAN_POINT('Origin',(-1.1,-2.9,-9.095)) ;
#142850=CARTESIAN_POINT('Origin',(-1.1,-2.9,-36.89)) ;
#142851=CARTESIAN_POINT('',(-1.2,-2.9,-13.765)) ;
#142852=CARTESIAN_POINT('',(-1.2,-2.9,-12.905)) ;
#142853=CARTESIAN_POINT('',(-1.2,-2.9,-36.89)) ;
#142854=CARTESIAN_POINT('',(-1.1,-3.,-13.765)) ;
#142855=CARTESIAN_POINT('Origin',(-1.1,-2.9,-13.765)) ;
#142856=CARTESIAN_POINT('',(-1.1,-3.,-12.905)) ;
#142857=CARTESIAN_POINT('',(-1.1,-3.,-36.89)) ;
#142858=CARTESIAN_POINT('Origin',(-1.1,-2.9,-12.905)) ;
#142859=CARTESIAN_POINT('Origin',(-1.1,-2.9,-36.89)) ;
#142860=CARTESIAN_POINT('',(-1.2,-2.9,-17.575)) ;
#142861=CARTESIAN_POINT('',(-1.2,-2.9,-16.715)) ;
#142862=CARTESIAN_POINT('',(-1.2,-2.9,-36.89)) ;
#142863=CARTESIAN_POINT('',(-1.1,-3.,-17.575)) ;
#142864=CARTESIAN_POINT('Origin',(-1.1,-2.9,-17.575)) ;
#142865=CARTESIAN_POINT('',(-1.1,-3.,-16.715)) ;
#142866=CARTESIAN_POINT('',(-1.1,-3.,-36.89)) ;
#142867=CARTESIAN_POINT('Origin',(-1.1,-2.9,-16.715)) ;
#142868=CARTESIAN_POINT('Origin',(-1.1,-2.9,-36.89)) ;
#142869=CARTESIAN_POINT('',(-1.2,-2.9,-21.385)) ;
#142870=CARTESIAN_POINT('',(-1.2,-2.9,-20.525)) ;
#142871=CARTESIAN_POINT('',(-1.2,-2.9,-36.89)) ;
#142872=CARTESIAN_POINT('',(-1.1,-3.,-21.385)) ;
#142873=CARTESIAN_POINT('Origin',(-1.1,-2.9,-21.385)) ;
#142874=CARTESIAN_POINT('',(-1.1,-3.,-20.525)) ;
#142875=CARTESIAN_POINT('',(-1.1,-3.,-36.89)) ;
#142876=CARTESIAN_POINT('Origin',(-1.1,-2.9,-20.525)) ;
#142877=CARTESIAN_POINT('Origin',(-1.1,-2.9,-36.89)) ;
#142878=CARTESIAN_POINT('',(-1.2,-2.9,-25.195)) ;
#142879=CARTESIAN_POINT('',(-1.2,-2.9,-24.335)) ;
#142880=CARTESIAN_POINT('',(-1.2,-2.9,-36.89)) ;
#142881=CARTESIAN_POINT('',(-1.1,-3.,-25.195)) ;
#142882=CARTESIAN_POINT('Origin',(-1.1,-2.9,-25.195)) ;
#142883=CARTESIAN_POINT('',(-1.1,-3.,-24.335)) ;
#142884=CARTESIAN_POINT('',(-1.1,-3.,-36.89)) ;
#142885=CARTESIAN_POINT('Origin',(-1.1,-2.9,-24.335)) ;
#142886=CARTESIAN_POINT('Origin',(-1.1,-2.9,-36.89)) ;
#142887=CARTESIAN_POINT('',(-1.2,-2.9,-29.005)) ;
#142888=CARTESIAN_POINT('',(-1.2,-2.9,-28.145)) ;
#142889=CARTESIAN_POINT('',(-1.2,-2.9,-36.89)) ;
#142890=CARTESIAN_POINT('',(-1.1,-3.,-29.005)) ;
#142891=CARTESIAN_POINT('Origin',(-1.1,-2.9,-29.005)) ;
#142892=CARTESIAN_POINT('',(-1.1,-3.,-28.145)) ;
#142893=CARTESIAN_POINT('',(-1.1,-3.,-36.89)) ;
#142894=CARTESIAN_POINT('Origin',(-1.1,-2.9,-28.145)) ;
#142895=CARTESIAN_POINT('Origin',(-1.1,-2.9,-36.89)) ;
#142896=CARTESIAN_POINT('',(-1.2,-2.9,-32.815)) ;
#142897=CARTESIAN_POINT('',(-1.2,-2.9,-31.955)) ;
#142898=CARTESIAN_POINT('',(-1.2,-2.9,-36.89)) ;
#142899=CARTESIAN_POINT('',(-1.1,-3.,-32.815)) ;
#142900=CARTESIAN_POINT('Origin',(-1.1,-2.9,-32.815)) ;
#142901=CARTESIAN_POINT('',(-1.1,-3.,-31.955)) ;
#142902=CARTESIAN_POINT('',(-1.1,-3.,-36.89)) ;
#142903=CARTESIAN_POINT('Origin',(-1.1,-2.9,-31.955)) ;
#142904=CARTESIAN_POINT('Origin',(0.600000000000001,2.80617032878603E-17,
0.)) ;
#142905=CARTESIAN_POINT('',(0.600000000000001,-1.9,0.4)) ;
#142906=CARTESIAN_POINT('',(0.600000000000001,-0.3,0.4)) ;
#142907=CARTESIAN_POINT('',(0.600000000000001,-2.3980000991444E-17,0.4)) ;
#142908=CARTESIAN_POINT('',(0.6,-0.4,0.3)) ;
#142909=CARTESIAN_POINT('Origin',(0.6,-0.3,0.3)) ;
#142910=CARTESIAN_POINT('',(0.6,-0.4,-0.3)) ;
#142911=CARTESIAN_POINT('',(0.6,-0.4,0.4)) ;
#142912=CARTESIAN_POINT('Origin',(0.6,-0.3,-0.3)) ;
#142913=CARTESIAN_POINT('',(0.600000000000001,-2.1,-0.6)) ;
#142914=CARTESIAN_POINT('Origin',(0.600000000000001,-1.9,-0.6)) ;
#142915=CARTESIAN_POINT('',(0.600000000000001,-2.1,-1.275)) ;
#142916=CARTESIAN_POINT('',(0.600000000000001,-2.1,0.)) ;
#142917=CARTESIAN_POINT('',(0.600000000000001,-2.9,-1.275)) ;
#142918=CARTESIAN_POINT('',(0.600000000000001,-3.699042706127E-17,-1.275)) ;
#142919=CARTESIAN_POINT('',(0.600000000000001,-2.9,1.275)) ;
#142920=CARTESIAN_POINT('',(0.600000000000001,-2.9,0.)) ;
#142921=CARTESIAN_POINT('',(0.600000000000001,-2.1,1.275)) ;
#142922=CARTESIAN_POINT('',(0.600000000000001,1.58165963986121E-16,1.275)) ;
#142923=CARTESIAN_POINT('',(0.600000000000001,-2.1,0.6)) ;
#142924=CARTESIAN_POINT('',(0.600000000000001,-2.1,0.)) ;
#142925=CARTESIAN_POINT('Origin',(0.600000000000001,-1.9,0.6)) ;
#142926=CARTESIAN_POINT('Origin',(-0.999999999999999,1.25,-1.375)) ;
#142927=CARTESIAN_POINT('',(-1.1,-1.9,-1.375)) ;
#142928=CARTESIAN_POINT('',(-0.899999999999999,-2.1,-1.375)) ;
#142929=CARTESIAN_POINT('Origin',(-0.899999999999999,-1.9,-1.375)) ;
#142930=CARTESIAN_POINT('',(-1.1,-2.9,-1.375)) ;
#142931=CARTESIAN_POINT('',(-1.1,-2.9,-1.375)) ;
#142932=CARTESIAN_POINT('',(0.500000000000001,-2.9,-1.375)) ;
#142933=CARTESIAN_POINT('',(0.600000000000001,-2.9,-1.375)) ;
#142934=CARTESIAN_POINT('',(0.500000000000001,-2.1,-1.375)) ;
#142935=CARTESIAN_POINT('',(0.5,1.25,-1.375)) ;
#142936=CARTESIAN_POINT('',(-0.999999999999999,-2.1,-1.375)) ;
#142937=CARTESIAN_POINT('Origin',(-0.999999999999999,1.25,1.375)) ;
#142938=CARTESIAN_POINT('',(-0.899999999999999,-2.1,1.375)) ;
#142939=CARTESIAN_POINT('',(-1.1,-1.9,1.375)) ;
#142940=CARTESIAN_POINT('Origin',(-0.899999999999999,-1.9,1.375)) ;
#142941=CARTESIAN_POINT('',(0.500000000000001,-2.1,1.375)) ;
#142942=CARTESIAN_POINT('',(0.600000000000001,-2.1,1.375)) ;
#142943=CARTESIAN_POINT('',(0.500000000000001,-2.9,1.375)) ;
#142944=CARTESIAN_POINT('',(0.5,1.25,1.375)) ;
#142945=CARTESIAN_POINT('',(-1.1,-2.9,1.375)) ;
#142946=CARTESIAN_POINT('',(-1.1,-2.9,1.375)) ;
#142947=CARTESIAN_POINT('',(-1.1,1.25,1.375)) ;
#142948=CARTESIAN_POINT('Origin',(-1.1,-2.9,-36.89)) ;
#142949=CARTESIAN_POINT('',(-1.2,-2.9,1.475)) ;
#142950=CARTESIAN_POINT('',(-1.2,-2.9,2.5)) ;
#142951=CARTESIAN_POINT('',(-1.2,-2.9,-36.89)) ;
#142952=CARTESIAN_POINT('',(-1.1,-3.,1.475)) ;
#142953=CARTESIAN_POINT('Origin',(-1.1,-2.9,1.475)) ;
#142954=CARTESIAN_POINT('',(-1.1,-3.,2.5)) ;
#142955=CARTESIAN_POINT('',(-1.1,-3.,-36.89)) ;
#142956=CARTESIAN_POINT('Origin',(-1.1,-2.9,2.5)) ;
#142957=CARTESIAN_POINT('Origin',(7.9,-2.9,-36.89)) ;
#142958=CARTESIAN_POINT('',(7.9,-3.,-36.79)) ;
#142959=CARTESIAN_POINT('',(7.9,-3.,2.5)) ;
#142960=CARTESIAN_POINT('',(7.9,-3.,-36.89)) ;
#142961=CARTESIAN_POINT('',(8.,-2.9,-36.79)) ;
#142962=CARTESIAN_POINT('Origin',(7.9,-2.9,-36.79)) ;
#142963=CARTESIAN_POINT('',(8.,-2.9,2.5)) ;
#142964=CARTESIAN_POINT('',(8.,-2.9,-36.89)) ;
#142965=CARTESIAN_POINT('Origin',(7.9,-2.9,2.5)) ;
#142966=CARTESIAN_POINT('Origin',(-1.1,-3.,-36.89)) ;
#142967=CARTESIAN_POINT('',(0.500000000000001,-3.,-35.765)) ;
#142968=CARTESIAN_POINT('',(0.700000000000002,-3.,-35.565)) ;
#142969=CARTESIAN_POINT('Origin',(0.500000000000001,-3.,-35.565)) ;
#142970=CARTESIAN_POINT('',(-1.1,-3.,-35.765)) ;
#142971=CARTESIAN_POINT('',(-1.1,-3.,-35.765)) ;
#142972=CARTESIAN_POINT('',(-1.1,-3.,-36.79)) ;
#142973=CARTESIAN_POINT('',(-1.1,-3.,-36.89)) ;
#142974=CARTESIAN_POINT('',(7.9,-3.,-36.79)) ;
#142975=CARTESIAN_POINT('',(-1.1,-3.,2.5)) ;
#142976=CARTESIAN_POINT('',(0.500000000000001,-3.,1.475)) ;
#142977=CARTESIAN_POINT('',(0.600000000000001,-3.,1.475)) ;
#142978=CARTESIAN_POINT('',(0.700000000000002,-3.,1.275)) ;
#142979=CARTESIAN_POINT('Origin',(0.500000000000001,-3.,1.275)) ;
#142980=CARTESIAN_POINT('',(0.700000000000002,-3.,-1.275)) ;
#142981=CARTESIAN_POINT('',(0.700000000000002,-3.,-36.89)) ;
#142982=CARTESIAN_POINT('',(0.500000000000001,-3.,-1.475)) ;
#142983=CARTESIAN_POINT('Origin',(0.500000000000001,-3.,-1.275)) ;
#142984=CARTESIAN_POINT('',(-1.1,-3.,-1.475)) ;
#142985=CARTESIAN_POINT('',(0.500000000000001,-3.,-2.335)) ;
#142986=CARTESIAN_POINT('',(0.600000000000001,-3.,-2.335)) ;
#142987=CARTESIAN_POINT('',(0.700000000000002,-3.,-2.535)) ;
#142988=CARTESIAN_POINT('Origin',(0.500000000000001,-3.,-2.535)) ;
#142989=CARTESIAN_POINT('',(0.700000000000002,-3.,-5.085)) ;
#142990=CARTESIAN_POINT('',(0.700000000000002,-3.,-36.89)) ;
#142991=CARTESIAN_POINT('',(0.500000000000001,-3.,-5.285)) ;
#142992=CARTESIAN_POINT('Origin',(0.500000000000001,-3.,-5.085)) ;
#142993=CARTESIAN_POINT('',(-1.1,-3.,-5.285)) ;
#142994=CARTESIAN_POINT('',(0.500000000000001,-3.,-6.145)) ;
#142995=CARTESIAN_POINT('',(0.600000000000001,-3.,-6.145)) ;
#142996=CARTESIAN_POINT('',(0.700000000000002,-3.,-6.345)) ;
#142997=CARTESIAN_POINT('Origin',(0.500000000000001,-3.,-6.345)) ;
#142998=CARTESIAN_POINT('',(0.700000000000002,-3.,-8.895)) ;
#142999=CARTESIAN_POINT('',(0.700000000000002,-3.,-36.89)) ;
#143000=CARTESIAN_POINT('',(0.500000000000001,-3.,-9.095)) ;
#143001=CARTESIAN_POINT('Origin',(0.500000000000001,-3.,-8.895)) ;
#143002=CARTESIAN_POINT('',(-1.1,-3.,-9.095)) ;
#143003=CARTESIAN_POINT('',(0.500000000000001,-3.,-9.955)) ;
#143004=CARTESIAN_POINT('',(0.600000000000001,-3.,-9.955)) ;
#143005=CARTESIAN_POINT('',(0.700000000000002,-3.,-10.155)) ;
#143006=CARTESIAN_POINT('Origin',(0.500000000000001,-3.,-10.155)) ;
#143007=CARTESIAN_POINT('',(0.700000000000002,-3.,-12.705)) ;
#143008=CARTESIAN_POINT('',(0.700000000000002,-3.,-36.89)) ;
#143009=CARTESIAN_POINT('',(0.500000000000001,-3.,-12.905)) ;
#143010=CARTESIAN_POINT('Origin',(0.500000000000001,-3.,-12.705)) ;
#143011=CARTESIAN_POINT('',(-1.1,-3.,-12.905)) ;
#143012=CARTESIAN_POINT('',(0.500000000000001,-3.,-13.765)) ;
#143013=CARTESIAN_POINT('',(0.600000000000001,-3.,-13.765)) ;
#143014=CARTESIAN_POINT('',(0.700000000000002,-3.,-13.965)) ;
#143015=CARTESIAN_POINT('Origin',(0.500000000000001,-3.,-13.965)) ;
#143016=CARTESIAN_POINT('',(0.700000000000002,-3.,-16.515)) ;
#143017=CARTESIAN_POINT('',(0.700000000000002,-3.,-36.89)) ;
#143018=CARTESIAN_POINT('',(0.500000000000001,-3.,-16.715)) ;
#143019=CARTESIAN_POINT('Origin',(0.500000000000001,-3.,-16.515)) ;
#143020=CARTESIAN_POINT('',(-1.1,-3.,-16.715)) ;
#143021=CARTESIAN_POINT('',(0.500000000000001,-3.,-17.575)) ;
#143022=CARTESIAN_POINT('',(0.600000000000001,-3.,-17.575)) ;
#143023=CARTESIAN_POINT('',(0.700000000000002,-3.,-17.775)) ;
#143024=CARTESIAN_POINT('Origin',(0.500000000000001,-3.,-17.775)) ;
#143025=CARTESIAN_POINT('',(0.700000000000002,-3.,-20.325)) ;
#143026=CARTESIAN_POINT('',(0.700000000000002,-3.,-36.89)) ;
#143027=CARTESIAN_POINT('',(0.500000000000001,-3.,-20.525)) ;
#143028=CARTESIAN_POINT('Origin',(0.500000000000001,-3.,-20.325)) ;
#143029=CARTESIAN_POINT('',(-1.1,-3.,-20.525)) ;
#143030=CARTESIAN_POINT('',(0.500000000000001,-3.,-21.385)) ;
#143031=CARTESIAN_POINT('',(0.600000000000001,-3.,-21.385)) ;
#143032=CARTESIAN_POINT('',(0.700000000000002,-3.,-21.585)) ;
#143033=CARTESIAN_POINT('Origin',(0.500000000000001,-3.,-21.585)) ;
#143034=CARTESIAN_POINT('',(0.700000000000002,-3.,-24.135)) ;
#143035=CARTESIAN_POINT('',(0.700000000000002,-3.,-36.89)) ;
#143036=CARTESIAN_POINT('',(0.500000000000001,-3.,-24.335)) ;
#143037=CARTESIAN_POINT('Origin',(0.500000000000001,-3.,-24.135)) ;
#143038=CARTESIAN_POINT('',(-1.1,-3.,-24.335)) ;
#143039=CARTESIAN_POINT('',(0.500000000000001,-3.,-25.195)) ;
#143040=CARTESIAN_POINT('',(0.600000000000001,-3.,-25.195)) ;
#143041=CARTESIAN_POINT('',(0.700000000000002,-3.,-25.395)) ;
#143042=CARTESIAN_POINT('Origin',(0.500000000000001,-3.,-25.395)) ;
#143043=CARTESIAN_POINT('',(0.700000000000002,-3.,-27.945)) ;
#143044=CARTESIAN_POINT('',(0.700000000000002,-3.,-36.89)) ;
#143045=CARTESIAN_POINT('',(0.500000000000001,-3.,-28.145)) ;
#143046=CARTESIAN_POINT('Origin',(0.500000000000001,-3.,-27.945)) ;
#143047=CARTESIAN_POINT('',(-1.1,-3.,-28.145)) ;
#143048=CARTESIAN_POINT('',(0.500000000000001,-3.,-29.005)) ;
#143049=CARTESIAN_POINT('',(0.600000000000001,-3.,-29.005)) ;
#143050=CARTESIAN_POINT('',(0.700000000000002,-3.,-29.205)) ;
#143051=CARTESIAN_POINT('Origin',(0.500000000000001,-3.,-29.205)) ;
#143052=CARTESIAN_POINT('',(0.700000000000002,-3.,-31.755)) ;
#143053=CARTESIAN_POINT('',(0.700000000000002,-3.,-36.89)) ;
#143054=CARTESIAN_POINT('',(0.500000000000001,-3.,-31.955)) ;
#143055=CARTESIAN_POINT('Origin',(0.500000000000001,-3.,-31.755)) ;
#143056=CARTESIAN_POINT('',(-1.1,-3.,-31.955)) ;
#143057=CARTESIAN_POINT('',(0.500000000000001,-3.,-32.815)) ;
#143058=CARTESIAN_POINT('',(0.600000000000001,-3.,-32.815)) ;
#143059=CARTESIAN_POINT('',(0.700000000000002,-3.,-33.015)) ;
#143060=CARTESIAN_POINT('Origin',(0.500000000000001,-3.,-33.015)) ;
#143061=CARTESIAN_POINT('',(0.700000000000002,-3.,-36.89)) ;
#143062=CARTESIAN_POINT('Origin',(-1.1,-2.9,-36.89)) ;
#143063=CARTESIAN_POINT('',(-1.2,-2.9,-35.765)) ;
#143064=CARTESIAN_POINT('Origin',(-1.1,-2.9,-35.765)) ;
#143065=CARTESIAN_POINT('',(-1.2,-2.9,-36.79)) ;
#143066=CARTESIAN_POINT('',(-1.2,-2.9,-36.89)) ;
#143067=CARTESIAN_POINT('Origin',(-1.1,-2.9,-36.79)) ;
#143068=CARTESIAN_POINT('Origin',(-1.2,4.15,-36.89)) ;
#143069=CARTESIAN_POINT('',(-1.2,1.15,-32.815)) ;
#143070=CARTESIAN_POINT('',(-1.2,1.35,-33.015)) ;
#143071=CARTESIAN_POINT('Origin',(-1.2,1.15,-33.015)) ;
#143072=CARTESIAN_POINT('',(-1.2,-2.9,-32.815)) ;
#143073=CARTESIAN_POINT('',(-1.2,1.15,-31.955)) ;
#143074=CARTESIAN_POINT('',(-1.2,1.25,-31.955)) ;
#143075=CARTESIAN_POINT('',(-1.2,1.35,-31.755)) ;
#143076=CARTESIAN_POINT('Origin',(-1.2,1.15,-31.755)) ;
#143077=CARTESIAN_POINT('',(-1.2,1.35,-29.205)) ;
#143078=CARTESIAN_POINT('',(-1.2,1.35,-29.105)) ;
#143079=CARTESIAN_POINT('',(-1.2,1.15,-29.005)) ;
#143080=CARTESIAN_POINT('Origin',(-1.2,1.15,-29.205)) ;
#143081=CARTESIAN_POINT('',(-1.2,-2.9,-29.005)) ;
#143082=CARTESIAN_POINT('',(-1.2,1.15,-28.145)) ;
#143083=CARTESIAN_POINT('',(-1.2,1.25,-28.145)) ;
#143084=CARTESIAN_POINT('',(-1.2,1.35,-27.945)) ;
#143085=CARTESIAN_POINT('Origin',(-1.2,1.15,-27.945)) ;
#143086=CARTESIAN_POINT('',(-1.2,1.35,-25.395)) ;
#143087=CARTESIAN_POINT('',(-1.2,1.35,-25.295)) ;
#143088=CARTESIAN_POINT('',(-1.2,1.15,-25.195)) ;
#143089=CARTESIAN_POINT('Origin',(-1.2,1.15,-25.395)) ;
#143090=CARTESIAN_POINT('',(-1.2,-2.9,-25.195)) ;
#143091=CARTESIAN_POINT('',(-1.2,1.15,-24.335)) ;
#143092=CARTESIAN_POINT('',(-1.2,1.25,-24.335)) ;
#143093=CARTESIAN_POINT('',(-1.2,1.35,-24.135)) ;
#143094=CARTESIAN_POINT('Origin',(-1.2,1.15,-24.135)) ;
#143095=CARTESIAN_POINT('',(-1.2,1.35,-21.585)) ;
#143096=CARTESIAN_POINT('',(-1.2,1.35,-21.485)) ;
#143097=CARTESIAN_POINT('',(-1.2,1.15,-21.385)) ;
#143098=CARTESIAN_POINT('Origin',(-1.2,1.15,-21.585)) ;
#143099=CARTESIAN_POINT('',(-1.2,-2.9,-21.385)) ;
#143100=CARTESIAN_POINT('',(-1.2,1.15,-20.525)) ;
#143101=CARTESIAN_POINT('',(-1.2,1.25,-20.525)) ;
#143102=CARTESIAN_POINT('',(-1.2,1.35,-20.325)) ;
#143103=CARTESIAN_POINT('Origin',(-1.2,1.15,-20.325)) ;
#143104=CARTESIAN_POINT('',(-1.2,1.35,-17.775)) ;
#143105=CARTESIAN_POINT('',(-1.2,1.35,-17.675)) ;
#143106=CARTESIAN_POINT('',(-1.2,1.15,-17.575)) ;
#143107=CARTESIAN_POINT('Origin',(-1.2,1.15,-17.775)) ;
#143108=CARTESIAN_POINT('',(-1.2,-2.9,-17.575)) ;
#143109=CARTESIAN_POINT('',(-1.2,1.15,-16.715)) ;
#143110=CARTESIAN_POINT('',(-1.2,1.25,-16.715)) ;
#143111=CARTESIAN_POINT('',(-1.2,1.35,-16.515)) ;
#143112=CARTESIAN_POINT('Origin',(-1.2,1.15,-16.515)) ;
#143113=CARTESIAN_POINT('',(-1.2,1.35,-13.965)) ;
#143114=CARTESIAN_POINT('',(-1.2,1.35,-13.865)) ;
#143115=CARTESIAN_POINT('',(-1.2,1.15,-13.765)) ;
#143116=CARTESIAN_POINT('Origin',(-1.2,1.15,-13.965)) ;
#143117=CARTESIAN_POINT('',(-1.2,-2.9,-13.765)) ;
#143118=CARTESIAN_POINT('',(-1.2,1.15,-12.905)) ;
#143119=CARTESIAN_POINT('',(-1.2,1.25,-12.905)) ;
#143120=CARTESIAN_POINT('',(-1.2,1.35,-12.705)) ;
#143121=CARTESIAN_POINT('Origin',(-1.2,1.15,-12.705)) ;
#143122=CARTESIAN_POINT('',(-1.2,1.35,-10.155)) ;
#143123=CARTESIAN_POINT('',(-1.2,1.35,-10.055)) ;
#143124=CARTESIAN_POINT('',(-1.2,1.15,-9.955)) ;
#143125=CARTESIAN_POINT('Origin',(-1.2,1.15,-10.155)) ;
#143126=CARTESIAN_POINT('',(-1.2,-2.9,-9.955)) ;
#143127=CARTESIAN_POINT('',(-1.2,1.15,-9.095)) ;
#143128=CARTESIAN_POINT('',(-1.2,1.25,-9.095)) ;
#143129=CARTESIAN_POINT('',(-1.2,1.35,-8.895)) ;
#143130=CARTESIAN_POINT('Origin',(-1.2,1.15,-8.895)) ;
#143131=CARTESIAN_POINT('',(-1.2,1.35,-6.345)) ;
#143132=CARTESIAN_POINT('',(-1.2,1.35,-6.245)) ;
#143133=CARTESIAN_POINT('',(-1.2,1.15,-6.145)) ;
#143134=CARTESIAN_POINT('Origin',(-1.2,1.15,-6.345)) ;
#143135=CARTESIAN_POINT('',(-1.2,-2.9,-6.145)) ;
#143136=CARTESIAN_POINT('',(-1.2,1.15,-5.285)) ;
#143137=CARTESIAN_POINT('',(-1.2,1.25,-5.285)) ;
#143138=CARTESIAN_POINT('',(-1.2,1.35,-5.085)) ;
#143139=CARTESIAN_POINT('Origin',(-1.2,1.15,-5.085)) ;
#143140=CARTESIAN_POINT('',(-1.2,1.35,-2.535)) ;
#143141=CARTESIAN_POINT('',(-1.2,1.35,-2.435)) ;
#143142=CARTESIAN_POINT('',(-1.2,1.15,-2.335)) ;
#143143=CARTESIAN_POINT('Origin',(-1.2,1.15,-2.535)) ;
#143144=CARTESIAN_POINT('',(-1.2,-2.9,-2.335)) ;
#143145=CARTESIAN_POINT('',(-1.2,1.15,-1.475)) ;
#143146=CARTESIAN_POINT('',(-1.2,1.25,-1.475)) ;
#143147=CARTESIAN_POINT('',(-1.2,1.35,-1.275)) ;
#143148=CARTESIAN_POINT('Origin',(-1.2,1.15,-1.275)) ;
#143149=CARTESIAN_POINT('',(-1.2,1.35,1.275)) ;
#143150=CARTESIAN_POINT('',(-1.2,1.35,1.37499999999999)) ;
#143151=CARTESIAN_POINT('',(-1.2,1.15,1.475)) ;
#143152=CARTESIAN_POINT('Origin',(-1.2,1.15,1.275)) ;
#143153=CARTESIAN_POINT('',(-1.2,-2.9,1.475)) ;
#143154=CARTESIAN_POINT('',(-1.2,4.15,2.5)) ;
#143155=CARTESIAN_POINT('',(-1.2,4.15,2.5)) ;
#143156=CARTESIAN_POINT('',(-1.2,4.15,-36.79)) ;
#143157=CARTESIAN_POINT('',(-1.2,4.15,-36.89)) ;
#143158=CARTESIAN_POINT('',(-1.2,-2.9,-36.79)) ;
#143159=CARTESIAN_POINT('',(-1.2,1.15,-35.765)) ;
#143160=CARTESIAN_POINT('',(-1.2,1.25,-35.765)) ;
#143161=CARTESIAN_POINT('',(-1.2,1.35,-35.565)) ;
#143162=CARTESIAN_POINT('Origin',(-1.2,1.15,-35.565)) ;
#143163=CARTESIAN_POINT('',(-1.2,1.35,-32.915)) ;
#143164=CARTESIAN_POINT('Origin',(-1.1,4.15,-36.89)) ;
#143165=CARTESIAN_POINT('',(-1.1,4.25,-36.79)) ;
#143166=CARTESIAN_POINT('',(-1.1,4.25,2.5)) ;
#143167=CARTESIAN_POINT('',(-1.1,4.25,-36.89)) ;
#143168=CARTESIAN_POINT('Origin',(-1.1,4.15,-36.79)) ;
#143169=CARTESIAN_POINT('Origin',(-1.1,4.15,2.5)) ;
#143170=CARTESIAN_POINT('Origin',(-1.1,4.25,-36.89)) ;
#143171=CARTESIAN_POINT('',(4.35,4.25,-36.79)) ;
#143172=CARTESIAN_POINT('',(4.35,4.25,2.5)) ;
#143173=CARTESIAN_POINT('',(4.35,4.25,-36.89)) ;
#143174=CARTESIAN_POINT('',(-1.1,4.25,-36.79)) ;
#143175=CARTESIAN_POINT('',(-1.1,4.25,2.5)) ;
#143176=CARTESIAN_POINT('Origin',(4.35,4.35,-36.89)) ;
#143177=CARTESIAN_POINT('',(4.45,4.35,-36.79)) ;
#143178=CARTESIAN_POINT('',(4.45,4.35,2.5)) ;
#143179=CARTESIAN_POINT('',(4.45,4.35,-36.89)) ;
#143180=CARTESIAN_POINT('Origin',(4.35,4.35,-36.79)) ;
#143181=CARTESIAN_POINT('Origin',(4.35,4.35,2.5)) ;
#143182=CARTESIAN_POINT('Origin',(4.45,4.55,-36.89)) ;
#143183=CARTESIAN_POINT('',(4.45,4.55,-36.79)) ;
#143184=CARTESIAN_POINT('',(4.45,4.55,2.5)) ;
#143185=CARTESIAN_POINT('',(4.45,4.55,-36.89)) ;
#143186=CARTESIAN_POINT('',(4.45,4.35,-36.79)) ;
#143187=CARTESIAN_POINT('',(4.45,4.55,2.5)) ;
#143188=CARTESIAN_POINT('Origin',(4.55,4.55,-36.89)) ;
#143189=CARTESIAN_POINT('',(4.55,4.65,-36.79)) ;
#143190=CARTESIAN_POINT('',(4.55,4.65,2.5)) ;
#143191=CARTESIAN_POINT('',(4.55,4.65,-36.89)) ;
#143192=CARTESIAN_POINT('Origin',(4.55,4.55,-36.79)) ;
#143193=CARTESIAN_POINT('Origin',(4.55,4.55,2.5)) ;
#143194=CARTESIAN_POINT('Origin',(4.75,4.65,-36.89)) ;
#143195=CARTESIAN_POINT('',(4.75,4.65,-36.79)) ;
#143196=CARTESIAN_POINT('',(4.75,4.65,2.5)) ;
#143197=CARTESIAN_POINT('',(4.75,4.65,-36.89)) ;
#143198=CARTESIAN_POINT('',(4.55,4.65,-36.79)) ;
#143199=CARTESIAN_POINT('',(4.75,4.65,2.5)) ;
#143200=CARTESIAN_POINT('Origin',(4.75,4.55,-36.89)) ;
#143201=CARTESIAN_POINT('',(4.85,4.55,-36.79)) ;
#143202=CARTESIAN_POINT('',(4.85,4.55,2.5)) ;
#143203=CARTESIAN_POINT('',(4.85,4.55,-36.89)) ;
#143204=CARTESIAN_POINT('Origin',(4.75,4.55,-36.79)) ;
#143205=CARTESIAN_POINT('Origin',(4.75,4.55,2.5)) ;
#143206=CARTESIAN_POINT('Origin',(4.85,4.35,-36.89)) ;
#143207=CARTESIAN_POINT('',(4.85,4.35,-36.79)) ;
#143208=CARTESIAN_POINT('',(4.85,4.35,2.5)) ;
#143209=CARTESIAN_POINT('',(4.85,4.35,-36.89)) ;
#143210=CARTESIAN_POINT('',(4.85,4.55,-36.79)) ;
#143211=CARTESIAN_POINT('',(4.85,4.35,2.5)) ;
#143212=CARTESIAN_POINT('Origin',(4.95,4.35,-36.89)) ;
#143213=CARTESIAN_POINT('',(4.95,4.25,-36.79)) ;
#143214=CARTESIAN_POINT('',(4.95,4.25,2.5)) ;
#143215=CARTESIAN_POINT('',(4.95,4.25,-36.89)) ;
#143216=CARTESIAN_POINT('Origin',(4.95,4.35,-36.79)) ;
#143217=CARTESIAN_POINT('Origin',(4.95,4.35,2.5)) ;
#143218=CARTESIAN_POINT('Origin',(4.95,4.25,-36.89)) ;
#143219=CARTESIAN_POINT('',(7.9,4.25,-36.79)) ;
#143220=CARTESIAN_POINT('',(7.9,4.25,2.5)) ;
#143221=CARTESIAN_POINT('',(7.9,4.25,-36.89)) ;
#143222=CARTESIAN_POINT('',(4.95,4.25,-36.79)) ;
#143223=CARTESIAN_POINT('',(4.95,4.25,2.5)) ;
#143224=CARTESIAN_POINT('Origin',(7.9,4.15,-36.89)) ;
#143225=CARTESIAN_POINT('',(8.,4.15,-36.79)) ;
#143226=CARTESIAN_POINT('',(8.,4.15,2.5)) ;
#143227=CARTESIAN_POINT('',(8.,4.15,-36.89)) ;
#143228=CARTESIAN_POINT('Origin',(7.9,4.15,-36.79)) ;
#143229=CARTESIAN_POINT('Origin',(7.9,4.15,2.5)) ;
#143230=CARTESIAN_POINT('Origin',(8.,4.15,-36.89)) ;
#143231=CARTESIAN_POINT('',(8.,4.15,-36.79)) ;
#143232=CARTESIAN_POINT('',(8.,4.15,2.5)) ;
#143233=CARTESIAN_POINT('',(8.,1.9,-32.54)) ;
#143234=CARTESIAN_POINT('',(8.,2.1,-32.74)) ;
#143235=CARTESIAN_POINT('Origin',(8.,1.9,-32.74)) ;
#143236=CARTESIAN_POINT('',(8.,2.1,-33.69)) ;
#143237=CARTESIAN_POINT('',(8.,2.1,-33.69)) ;
#143238=CARTESIAN_POINT('',(8.,2.4,-33.69)) ;
#143239=CARTESIAN_POINT('',(8.,2.4,-33.69)) ;
#143240=CARTESIAN_POINT('',(8.,2.4,-33.5814213562373)) ;
#143241=CARTESIAN_POINT('',(8.,2.4,-33.5814213562373)) ;
#143242=CARTESIAN_POINT('',(8.,2.45857864376269,-33.44)) ;
#143243=CARTESIAN_POINT('Origin',(8.,2.6,-33.5814213562373)) ;
#143244=CARTESIAN_POINT('',(8.,3.00857864376269,-32.89)) ;
#143245=CARTESIAN_POINT('',(8.,3.00857864376269,-32.89)) ;
#143246=CARTESIAN_POINT('',(8.,3.35,-33.0314213562373)) ;
#143247=CARTESIAN_POINT('Origin',(8.,3.15,-33.0314213562373)) ;
#143248=CARTESIAN_POINT('',(8.,3.35,-35.5485786437627)) ;
#143249=CARTESIAN_POINT('',(8.,2.45857864376269,-35.14)) ;
#143250=CARTESIAN_POINT('',(8.,2.45857864376269,-35.14)) ;
#143251=CARTESIAN_POINT('',(8.,2.4,-34.9985786437627)) ;
#143252=CARTESIAN_POINT('Origin',(8.,2.6,-34.9985786437627)) ;
#143253=CARTESIAN_POINT('',(8.,2.4,-34.89)) ;
#143254=CARTESIAN_POINT('',(8.,2.4,-34.89)) ;
#143255=CARTESIAN_POINT('',(8.,2.1,-34.89)) ;
#143256=CARTESIAN_POINT('',(8.,2.1,-34.89)) ;
#143257=CARTESIAN_POINT('',(8.,2.1,-35.84)) ;
#143258=CARTESIAN_POINT('',(8.,2.1,-35.84)) ;
#143259=CARTESIAN_POINT('',(8.,1.9,-36.04)) ;
#143260=CARTESIAN_POINT('Origin',(8.,1.9,-35.84)) ;
#143261=CARTESIAN_POINT('',(8.,-2.15,-36.04)) ;
#143262=CARTESIAN_POINT('',(8.,-2.15,-36.04)) ;
#143263=CARTESIAN_POINT('',(8.,-2.35,-35.84)) ;
#143264=CARTESIAN_POINT('Origin',(8.,-2.15,-35.84)) ;
#143265=CARTESIAN_POINT('',(8.,-2.35,-35.1931195934094)) ;
#143266=CARTESIAN_POINT('',(8.,-2.35,-35.1931195934094)) ;
#143267=CARTESIAN_POINT('',(8.,-2.32153024911032,-35.0902732340176)) ;
#143268=CARTESIAN_POINT('Origin',(8.,-2.15,-35.1931195934094)) ;
#143269=CARTESIAN_POINT('',(8.,-2.32153024911033,-33.4897267659824)) ;
#143270=CARTESIAN_POINT('Origin',(8.,-3.65625,-34.29)) ;
#143271=CARTESIAN_POINT('',(8.,-2.35,-33.3868804065906)) ;
#143272=CARTESIAN_POINT('Origin',(8.,-2.15,-33.3868804065906)) ;
#143273=CARTESIAN_POINT('',(8.,-2.35,-32.74)) ;
#143274=CARTESIAN_POINT('',(8.,-2.35,-32.74)) ;
#143275=CARTESIAN_POINT('',(8.,-2.15,-32.54)) ;
#143276=CARTESIAN_POINT('Origin',(8.,-2.15,-32.74)) ;
#143277=CARTESIAN_POINT('',(8.,1.9,-32.54)) ;
#143278=CARTESIAN_POINT('',(8.,1.9,-28.73)) ;
#143279=CARTESIAN_POINT('',(8.,2.1,-28.93)) ;
#143280=CARTESIAN_POINT('Origin',(8.,1.9,-28.93)) ;
#143281=CARTESIAN_POINT('',(8.,2.1,-29.88)) ;
#143282=CARTESIAN_POINT('',(8.,2.1,-29.88)) ;
#143283=CARTESIAN_POINT('',(8.,2.4,-29.88)) ;
#143284=CARTESIAN_POINT('',(8.,2.4,-29.88)) ;
#143285=CARTESIAN_POINT('',(8.,2.4,-29.7714213562373)) ;
#143286=CARTESIAN_POINT('',(8.,2.4,-29.7714213562373)) ;
#143287=CARTESIAN_POINT('',(8.,2.45857864376269,-29.63)) ;
#143288=CARTESIAN_POINT('Origin',(8.,2.6,-29.7714213562373)) ;
#143289=CARTESIAN_POINT('',(8.,3.00857864376269,-29.08)) ;
#143290=CARTESIAN_POINT('',(8.,3.00857864376269,-29.08)) ;
#143291=CARTESIAN_POINT('',(8.,3.35,-29.2214213562373)) ;
#143292=CARTESIAN_POINT('Origin',(8.,3.15,-29.2214213562373)) ;
#143293=CARTESIAN_POINT('',(8.,3.35,-31.7385786437627)) ;
#143294=CARTESIAN_POINT('',(8.,2.45857864376269,-31.33)) ;
#143295=CARTESIAN_POINT('',(8.,2.45857864376269,-31.33)) ;
#143296=CARTESIAN_POINT('',(8.,2.4,-31.1885786437627)) ;
#143297=CARTESIAN_POINT('Origin',(8.,2.6,-31.1885786437627)) ;
#143298=CARTESIAN_POINT('',(8.,2.4,-31.08)) ;
#143299=CARTESIAN_POINT('',(8.,2.4,-31.08)) ;
#143300=CARTESIAN_POINT('',(8.,2.1,-31.08)) ;
#143301=CARTESIAN_POINT('',(8.,2.1,-31.08)) ;
#143302=CARTESIAN_POINT('',(8.,2.1,-32.03)) ;
#143303=CARTESIAN_POINT('',(8.,2.1,-32.03)) ;
#143304=CARTESIAN_POINT('',(8.,1.9,-32.23)) ;
#143305=CARTESIAN_POINT('Origin',(8.,1.9,-32.03)) ;
#143306=CARTESIAN_POINT('',(8.,-2.15,-32.23)) ;
#143307=CARTESIAN_POINT('',(8.,-2.15,-32.23)) ;
#143308=CARTESIAN_POINT('',(8.,-2.35,-32.03)) ;
#143309=CARTESIAN_POINT('Origin',(8.,-2.15,-32.03)) ;
#143310=CARTESIAN_POINT('',(8.,-2.35,-31.3831195934094)) ;
#143311=CARTESIAN_POINT('',(8.,-2.35,-31.3831195934094)) ;
#143312=CARTESIAN_POINT('',(8.,-2.32153024911032,-31.2802732340176)) ;
#143313=CARTESIAN_POINT('Origin',(8.,-2.15,-31.3831195934094)) ;
#143314=CARTESIAN_POINT('',(8.,-2.32153024911032,-29.6797267659824)) ;
#143315=CARTESIAN_POINT('Origin',(8.,-3.65625,-30.48)) ;
#143316=CARTESIAN_POINT('',(8.,-2.35,-29.5768804065906)) ;
#143317=CARTESIAN_POINT('Origin',(8.,-2.15,-29.5768804065906)) ;
#143318=CARTESIAN_POINT('',(8.,-2.35,-28.93)) ;
#143319=CARTESIAN_POINT('',(8.,-2.35,-28.93)) ;
#143320=CARTESIAN_POINT('',(8.,-2.15,-28.73)) ;
#143321=CARTESIAN_POINT('Origin',(8.,-2.15,-28.93)) ;
#143322=CARTESIAN_POINT('',(8.,1.9,-28.73)) ;
#143323=CARTESIAN_POINT('',(8.,1.9,-24.92)) ;
#143324=CARTESIAN_POINT('',(8.,2.1,-25.12)) ;
#143325=CARTESIAN_POINT('Origin',(8.,1.9,-25.12)) ;
#143326=CARTESIAN_POINT('',(8.,2.1,-26.07)) ;
#143327=CARTESIAN_POINT('',(8.,2.1,-26.07)) ;
#143328=CARTESIAN_POINT('',(8.,2.4,-26.07)) ;
#143329=CARTESIAN_POINT('',(8.,2.4,-26.07)) ;
#143330=CARTESIAN_POINT('',(8.,2.4,-25.9614213562373)) ;
#143331=CARTESIAN_POINT('',(8.,2.4,-25.9614213562373)) ;
#143332=CARTESIAN_POINT('',(8.,2.45857864376269,-25.82)) ;
#143333=CARTESIAN_POINT('Origin',(8.,2.6,-25.9614213562373)) ;
#143334=CARTESIAN_POINT('',(8.,3.00857864376269,-25.27)) ;
#143335=CARTESIAN_POINT('',(8.,3.00857864376269,-25.27)) ;
#143336=CARTESIAN_POINT('',(8.,3.35,-25.4114213562373)) ;
#143337=CARTESIAN_POINT('Origin',(8.,3.15,-25.4114213562373)) ;
#143338=CARTESIAN_POINT('',(8.,3.35,-27.9285786437627)) ;
#143339=CARTESIAN_POINT('',(8.,2.45857864376269,-27.52)) ;
#143340=CARTESIAN_POINT('',(8.,2.45857864376269,-27.52)) ;
#143341=CARTESIAN_POINT('',(8.,2.4,-27.3785786437627)) ;
#143342=CARTESIAN_POINT('Origin',(8.,2.6,-27.3785786437627)) ;
#143343=CARTESIAN_POINT('',(8.,2.4,-27.27)) ;
#143344=CARTESIAN_POINT('',(8.,2.4,-27.27)) ;
#143345=CARTESIAN_POINT('',(8.,2.1,-27.27)) ;
#143346=CARTESIAN_POINT('',(8.,2.1,-27.27)) ;
#143347=CARTESIAN_POINT('',(8.,2.1,-28.22)) ;
#143348=CARTESIAN_POINT('',(8.,2.1,-28.22)) ;
#143349=CARTESIAN_POINT('',(8.,1.9,-28.42)) ;
#143350=CARTESIAN_POINT('Origin',(8.,1.9,-28.22)) ;
#143351=CARTESIAN_POINT('',(8.,-2.15,-28.42)) ;
#143352=CARTESIAN_POINT('',(8.,-2.15,-28.42)) ;
#143353=CARTESIAN_POINT('',(8.,-2.35,-28.22)) ;
#143354=CARTESIAN_POINT('Origin',(8.,-2.15,-28.22)) ;
#143355=CARTESIAN_POINT('',(8.,-2.35,-27.5731195934094)) ;
#143356=CARTESIAN_POINT('',(8.,-2.35,-27.5731195934094)) ;
#143357=CARTESIAN_POINT('',(8.,-2.32153024911032,-27.4702732340176)) ;
#143358=CARTESIAN_POINT('Origin',(8.,-2.15,-27.5731195934094)) ;
#143359=CARTESIAN_POINT('',(8.,-2.32153024911032,-25.8697267659824)) ;
#143360=CARTESIAN_POINT('Origin',(8.,-3.65625,-26.67)) ;
#143361=CARTESIAN_POINT('',(8.,-2.35,-25.7668804065906)) ;
#143362=CARTESIAN_POINT('Origin',(8.,-2.15,-25.7668804065906)) ;
#143363=CARTESIAN_POINT('',(8.,-2.35,-25.12)) ;
#143364=CARTESIAN_POINT('',(8.,-2.35,-25.12)) ;
#143365=CARTESIAN_POINT('',(8.,-2.15,-24.92)) ;
#143366=CARTESIAN_POINT('Origin',(8.,-2.15,-25.12)) ;
#143367=CARTESIAN_POINT('',(8.,1.9,-24.92)) ;
#143368=CARTESIAN_POINT('',(8.,1.9,-21.11)) ;
#143369=CARTESIAN_POINT('',(8.,2.1,-21.31)) ;
#143370=CARTESIAN_POINT('Origin',(8.,1.9,-21.31)) ;
#143371=CARTESIAN_POINT('',(8.,2.1,-22.26)) ;
#143372=CARTESIAN_POINT('',(8.,2.1,-22.26)) ;
#143373=CARTESIAN_POINT('',(8.,2.4,-22.26)) ;
#143374=CARTESIAN_POINT('',(8.,2.4,-22.26)) ;
#143375=CARTESIAN_POINT('',(8.,2.4,-22.1514213562373)) ;
#143376=CARTESIAN_POINT('',(8.,2.4,-22.1514213562373)) ;
#143377=CARTESIAN_POINT('',(8.,2.45857864376269,-22.01)) ;
#143378=CARTESIAN_POINT('Origin',(8.,2.6,-22.1514213562373)) ;
#143379=CARTESIAN_POINT('',(8.,3.00857864376269,-21.46)) ;
#143380=CARTESIAN_POINT('',(8.,3.00857864376269,-21.46)) ;
#143381=CARTESIAN_POINT('',(8.,3.35,-21.6014213562373)) ;
#143382=CARTESIAN_POINT('Origin',(8.,3.15,-21.6014213562373)) ;
#143383=CARTESIAN_POINT('',(8.,3.35,-24.1185786437627)) ;
#143384=CARTESIAN_POINT('',(8.,2.45857864376269,-23.71)) ;
#143385=CARTESIAN_POINT('',(8.,2.45857864376269,-23.71)) ;
#143386=CARTESIAN_POINT('',(8.,2.4,-23.5685786437627)) ;
#143387=CARTESIAN_POINT('Origin',(8.,2.6,-23.5685786437627)) ;
#143388=CARTESIAN_POINT('',(8.,2.4,-23.46)) ;
#143389=CARTESIAN_POINT('',(8.,2.4,-23.46)) ;
#143390=CARTESIAN_POINT('',(8.,2.1,-23.46)) ;
#143391=CARTESIAN_POINT('',(8.,2.1,-23.46)) ;
#143392=CARTESIAN_POINT('',(8.,2.1,-24.41)) ;
#143393=CARTESIAN_POINT('',(8.,2.1,-24.41)) ;
#143394=CARTESIAN_POINT('',(8.,1.9,-24.61)) ;
#143395=CARTESIAN_POINT('Origin',(8.,1.9,-24.41)) ;
#143396=CARTESIAN_POINT('',(8.,-2.15,-24.61)) ;
#143397=CARTESIAN_POINT('',(8.,-2.15,-24.61)) ;
#143398=CARTESIAN_POINT('',(8.,-2.35,-24.41)) ;
#143399=CARTESIAN_POINT('Origin',(8.,-2.15,-24.41)) ;
#143400=CARTESIAN_POINT('',(8.,-2.35,-23.7631195934094)) ;
#143401=CARTESIAN_POINT('',(8.,-2.35,-23.7631195934094)) ;
#143402=CARTESIAN_POINT('',(8.,-2.32153024911032,-23.6602732340176)) ;
#143403=CARTESIAN_POINT('Origin',(8.,-2.15,-23.7631195934094)) ;
#143404=CARTESIAN_POINT('',(8.,-2.32153024911032,-22.0597267659824)) ;
#143405=CARTESIAN_POINT('Origin',(8.,-3.65625,-22.86)) ;
#143406=CARTESIAN_POINT('',(8.,-2.35,-21.9568804065906)) ;
#143407=CARTESIAN_POINT('Origin',(8.,-2.15,-21.9568804065906)) ;
#143408=CARTESIAN_POINT('',(8.,-2.35,-21.31)) ;
#143409=CARTESIAN_POINT('',(8.,-2.35,-21.31)) ;
#143410=CARTESIAN_POINT('',(8.,-2.15,-21.11)) ;
#143411=CARTESIAN_POINT('Origin',(8.,-2.15,-21.31)) ;
#143412=CARTESIAN_POINT('',(8.,1.9,-21.11)) ;
#143413=CARTESIAN_POINT('',(8.,1.9,-17.3)) ;
#143414=CARTESIAN_POINT('',(8.,2.1,-17.5)) ;
#143415=CARTESIAN_POINT('Origin',(8.,1.9,-17.5)) ;
#143416=CARTESIAN_POINT('',(8.,2.1,-18.45)) ;
#143417=CARTESIAN_POINT('',(8.,2.1,-18.45)) ;
#143418=CARTESIAN_POINT('',(8.,2.4,-18.45)) ;
#143419=CARTESIAN_POINT('',(8.,2.4,-18.45)) ;
#143420=CARTESIAN_POINT('',(8.,2.4,-18.3414213562373)) ;
#143421=CARTESIAN_POINT('',(8.,2.4,-18.3414213562373)) ;
#143422=CARTESIAN_POINT('',(8.,2.45857864376269,-18.2)) ;
#143423=CARTESIAN_POINT('Origin',(8.,2.6,-18.3414213562373)) ;
#143424=CARTESIAN_POINT('',(8.,3.00857864376269,-17.65)) ;
#143425=CARTESIAN_POINT('',(8.,3.00857864376269,-17.65)) ;
#143426=CARTESIAN_POINT('',(8.,3.35,-17.7914213562373)) ;
#143427=CARTESIAN_POINT('Origin',(8.,3.15,-17.7914213562373)) ;
#143428=CARTESIAN_POINT('',(8.,3.35,-20.3085786437627)) ;
#143429=CARTESIAN_POINT('',(8.,2.45857864376269,-19.9)) ;
#143430=CARTESIAN_POINT('',(8.,2.45857864376269,-19.9)) ;
#143431=CARTESIAN_POINT('',(8.,2.4,-19.7585786437627)) ;
#143432=CARTESIAN_POINT('Origin',(8.,2.6,-19.7585786437627)) ;
#143433=CARTESIAN_POINT('',(8.,2.4,-19.65)) ;
#143434=CARTESIAN_POINT('',(8.,2.4,-19.65)) ;
#143435=CARTESIAN_POINT('',(8.,2.1,-19.65)) ;
#143436=CARTESIAN_POINT('',(8.,2.1,-19.65)) ;
#143437=CARTESIAN_POINT('',(8.,2.1,-20.6)) ;
#143438=CARTESIAN_POINT('',(8.,2.1,-20.6)) ;
#143439=CARTESIAN_POINT('',(8.,1.9,-20.8)) ;
#143440=CARTESIAN_POINT('Origin',(8.,1.9,-20.6)) ;
#143441=CARTESIAN_POINT('',(8.,-2.15,-20.8)) ;
#143442=CARTESIAN_POINT('',(8.,-2.15,-20.8)) ;
#143443=CARTESIAN_POINT('',(8.,-2.35,-20.6)) ;
#143444=CARTESIAN_POINT('Origin',(8.,-2.15,-20.6)) ;
#143445=CARTESIAN_POINT('',(8.,-2.35,-19.9531195934094)) ;
#143446=CARTESIAN_POINT('',(8.,-2.35,-19.9531195934094)) ;
#143447=CARTESIAN_POINT('',(8.,-2.32153024911032,-19.8502732340176)) ;
#143448=CARTESIAN_POINT('Origin',(8.,-2.15,-19.9531195934094)) ;
#143449=CARTESIAN_POINT('',(8.,-2.32153024911032,-18.2497267659824)) ;
#143450=CARTESIAN_POINT('Origin',(8.,-3.65625,-19.05)) ;
#143451=CARTESIAN_POINT('',(8.,-2.35,-18.1468804065906)) ;
#143452=CARTESIAN_POINT('Origin',(8.,-2.15,-18.1468804065906)) ;
#143453=CARTESIAN_POINT('',(8.,-2.35,-17.5)) ;
#143454=CARTESIAN_POINT('',(8.,-2.35,-17.5)) ;
#143455=CARTESIAN_POINT('',(8.,-2.15,-17.3)) ;
#143456=CARTESIAN_POINT('Origin',(8.,-2.15,-17.5)) ;
#143457=CARTESIAN_POINT('',(8.,1.9,-17.3)) ;
#143458=CARTESIAN_POINT('',(8.,1.9,-13.49)) ;
#143459=CARTESIAN_POINT('',(8.,2.1,-13.69)) ;
#143460=CARTESIAN_POINT('Origin',(8.,1.9,-13.69)) ;
#143461=CARTESIAN_POINT('',(8.,2.1,-14.64)) ;
#143462=CARTESIAN_POINT('',(8.,2.1,-14.64)) ;
#143463=CARTESIAN_POINT('',(8.,2.4,-14.64)) ;
#143464=CARTESIAN_POINT('',(8.,2.4,-14.64)) ;
#143465=CARTESIAN_POINT('',(8.,2.4,-14.5314213562373)) ;
#143466=CARTESIAN_POINT('',(8.,2.4,-14.5314213562373)) ;
#143467=CARTESIAN_POINT('',(8.,2.45857864376269,-14.39)) ;
#143468=CARTESIAN_POINT('Origin',(8.,2.6,-14.5314213562373)) ;
#143469=CARTESIAN_POINT('',(8.,3.00857864376269,-13.84)) ;
#143470=CARTESIAN_POINT('',(8.,3.00857864376269,-13.84)) ;
#143471=CARTESIAN_POINT('',(8.,3.35,-13.9814213562373)) ;
#143472=CARTESIAN_POINT('Origin',(8.,3.15,-13.9814213562373)) ;
#143473=CARTESIAN_POINT('',(8.,3.35,-16.4985786437627)) ;
#143474=CARTESIAN_POINT('',(8.,2.45857864376269,-16.09)) ;
#143475=CARTESIAN_POINT('',(8.,2.45857864376269,-16.09)) ;
#143476=CARTESIAN_POINT('',(8.,2.4,-15.9485786437627)) ;
#143477=CARTESIAN_POINT('Origin',(8.,2.6,-15.9485786437627)) ;
#143478=CARTESIAN_POINT('',(8.,2.4,-15.84)) ;
#143479=CARTESIAN_POINT('',(8.,2.4,-15.84)) ;
#143480=CARTESIAN_POINT('',(8.,2.1,-15.84)) ;
#143481=CARTESIAN_POINT('',(8.,2.1,-15.84)) ;
#143482=CARTESIAN_POINT('',(8.,2.1,-16.79)) ;
#143483=CARTESIAN_POINT('',(8.,2.1,-16.79)) ;
#143484=CARTESIAN_POINT('',(8.,1.9,-16.99)) ;
#143485=CARTESIAN_POINT('Origin',(8.,1.9,-16.79)) ;
#143486=CARTESIAN_POINT('',(8.,-2.15,-16.99)) ;
#143487=CARTESIAN_POINT('',(8.,-2.15,-16.99)) ;
#143488=CARTESIAN_POINT('',(8.,-2.35,-16.79)) ;
#143489=CARTESIAN_POINT('Origin',(8.,-2.15,-16.79)) ;
#143490=CARTESIAN_POINT('',(8.,-2.35,-16.1431195934094)) ;
#143491=CARTESIAN_POINT('',(8.,-2.35,-16.1431195934094)) ;
#143492=CARTESIAN_POINT('',(8.,-2.32153024911032,-16.0402732340176)) ;
#143493=CARTESIAN_POINT('Origin',(8.,-2.15,-16.1431195934094)) ;
#143494=CARTESIAN_POINT('',(8.,-2.32153024911032,-14.4397267659824)) ;
#143495=CARTESIAN_POINT('Origin',(8.,-3.65625,-15.24)) ;
#143496=CARTESIAN_POINT('',(8.,-2.35,-14.3368804065906)) ;
#143497=CARTESIAN_POINT('Origin',(8.,-2.15,-14.3368804065906)) ;
#143498=CARTESIAN_POINT('',(8.,-2.35,-13.69)) ;
#143499=CARTESIAN_POINT('',(8.,-2.35,-13.69)) ;
#143500=CARTESIAN_POINT('',(8.,-2.15,-13.49)) ;
#143501=CARTESIAN_POINT('Origin',(8.,-2.15,-13.69)) ;
#143502=CARTESIAN_POINT('',(8.,1.9,-13.49)) ;
#143503=CARTESIAN_POINT('',(8.,1.9,-9.68)) ;
#143504=CARTESIAN_POINT('',(8.,2.1,-9.88)) ;
#143505=CARTESIAN_POINT('Origin',(8.,1.9,-9.88)) ;
#143506=CARTESIAN_POINT('',(8.,2.1,-10.83)) ;
#143507=CARTESIAN_POINT('',(8.,2.1,-10.83)) ;
#143508=CARTESIAN_POINT('',(8.,2.4,-10.83)) ;
#143509=CARTESIAN_POINT('',(8.,2.4,-10.83)) ;
#143510=CARTESIAN_POINT('',(8.,2.4,-10.7214213562373)) ;
#143511=CARTESIAN_POINT('',(8.,2.4,-10.7214213562373)) ;
#143512=CARTESIAN_POINT('',(8.,2.45857864376269,-10.58)) ;
#143513=CARTESIAN_POINT('Origin',(8.,2.6,-10.7214213562373)) ;
#143514=CARTESIAN_POINT('',(8.,3.00857864376269,-10.03)) ;
#143515=CARTESIAN_POINT('',(8.,3.00857864376269,-10.03)) ;
#143516=CARTESIAN_POINT('',(8.,3.35,-10.1714213562373)) ;
#143517=CARTESIAN_POINT('Origin',(8.,3.15,-10.1714213562373)) ;
#143518=CARTESIAN_POINT('',(8.,3.35,-12.6885786437627)) ;
#143519=CARTESIAN_POINT('',(8.,2.45857864376269,-12.28)) ;
#143520=CARTESIAN_POINT('',(8.,2.45857864376269,-12.28)) ;
#143521=CARTESIAN_POINT('',(8.,2.4,-12.1385786437627)) ;
#143522=CARTESIAN_POINT('Origin',(8.,2.6,-12.1385786437627)) ;
#143523=CARTESIAN_POINT('',(8.,2.4,-12.03)) ;
#143524=CARTESIAN_POINT('',(8.,2.4,-12.03)) ;
#143525=CARTESIAN_POINT('',(8.,2.1,-12.03)) ;
#143526=CARTESIAN_POINT('',(8.,2.1,-12.03)) ;
#143527=CARTESIAN_POINT('',(8.,2.1,-12.98)) ;
#143528=CARTESIAN_POINT('',(8.,2.1,-12.98)) ;
#143529=CARTESIAN_POINT('',(8.,1.9,-13.18)) ;
#143530=CARTESIAN_POINT('Origin',(8.,1.9,-12.98)) ;
#143531=CARTESIAN_POINT('',(8.,-2.15,-13.18)) ;
#143532=CARTESIAN_POINT('',(8.,-2.15,-13.18)) ;
#143533=CARTESIAN_POINT('',(8.,-2.35,-12.98)) ;
#143534=CARTESIAN_POINT('Origin',(8.,-2.15,-12.98)) ;
#143535=CARTESIAN_POINT('',(8.,-2.35,-12.3331195934094)) ;
#143536=CARTESIAN_POINT('',(8.,-2.35,-12.3331195934094)) ;
#143537=CARTESIAN_POINT('',(8.,-2.32153024911032,-12.2302732340176)) ;
#143538=CARTESIAN_POINT('Origin',(8.,-2.15,-12.3331195934094)) ;
#143539=CARTESIAN_POINT('',(8.,-2.32153024911032,-10.6297267659824)) ;
#143540=CARTESIAN_POINT('Origin',(8.,-3.65625,-11.43)) ;
#143541=CARTESIAN_POINT('',(8.,-2.35,-10.5268804065906)) ;
#143542=CARTESIAN_POINT('Origin',(8.,-2.15,-10.5268804065906)) ;
#143543=CARTESIAN_POINT('',(8.,-2.35,-9.88)) ;
#143544=CARTESIAN_POINT('',(8.,-2.35,-9.88)) ;
#143545=CARTESIAN_POINT('',(8.,-2.15,-9.68)) ;
#143546=CARTESIAN_POINT('Origin',(8.,-2.15,-9.88)) ;
#143547=CARTESIAN_POINT('',(8.,1.9,-9.68)) ;
#143548=CARTESIAN_POINT('',(8.,1.9,-5.87)) ;
#143549=CARTESIAN_POINT('',(8.,2.1,-6.07)) ;
#143550=CARTESIAN_POINT('Origin',(8.,1.9,-6.07)) ;
#143551=CARTESIAN_POINT('',(8.,2.1,-7.02)) ;
#143552=CARTESIAN_POINT('',(8.,2.1,-7.02)) ;
#143553=CARTESIAN_POINT('',(8.,2.4,-7.02)) ;
#143554=CARTESIAN_POINT('',(8.,2.4,-7.02)) ;
#143555=CARTESIAN_POINT('',(8.,2.4,-6.91142135623731)) ;
#143556=CARTESIAN_POINT('',(8.,2.4,-6.91142135623731)) ;
#143557=CARTESIAN_POINT('',(8.,2.45857864376269,-6.77)) ;
#143558=CARTESIAN_POINT('Origin',(8.,2.6,-6.91142135623731)) ;
#143559=CARTESIAN_POINT('',(8.,3.00857864376269,-6.22)) ;
#143560=CARTESIAN_POINT('',(8.,3.00857864376269,-6.22)) ;
#143561=CARTESIAN_POINT('',(8.,3.35,-6.36142135623731)) ;
#143562=CARTESIAN_POINT('Origin',(8.,3.15,-6.36142135623731)) ;
#143563=CARTESIAN_POINT('',(8.,3.35,-8.87857864376269)) ;
#143564=CARTESIAN_POINT('',(8.,2.45857864376269,-8.47)) ;
#143565=CARTESIAN_POINT('',(8.,2.45857864376269,-8.47)) ;
#143566=CARTESIAN_POINT('',(8.,2.4,-8.32857864376269)) ;
#143567=CARTESIAN_POINT('Origin',(8.,2.6,-8.32857864376269)) ;
#143568=CARTESIAN_POINT('',(8.,2.4,-8.22)) ;
#143569=CARTESIAN_POINT('',(8.,2.4,-8.22)) ;
#143570=CARTESIAN_POINT('',(8.,2.1,-8.22)) ;
#143571=CARTESIAN_POINT('',(8.,2.1,-8.22)) ;
#143572=CARTESIAN_POINT('',(8.,2.1,-9.17)) ;
#143573=CARTESIAN_POINT('',(8.,2.1,-9.17)) ;
#143574=CARTESIAN_POINT('',(8.,1.9,-9.37)) ;
#143575=CARTESIAN_POINT('Origin',(8.,1.9,-9.17)) ;
#143576=CARTESIAN_POINT('',(8.,-2.15,-9.37)) ;
#143577=CARTESIAN_POINT('',(8.,-2.15,-9.37)) ;
#143578=CARTESIAN_POINT('',(8.,-2.35,-9.17)) ;
#143579=CARTESIAN_POINT('Origin',(8.,-2.15,-9.17)) ;
#143580=CARTESIAN_POINT('',(8.,-2.35,-8.52311959340942)) ;
#143581=CARTESIAN_POINT('',(8.,-2.35,-8.52311959340942)) ;
#143582=CARTESIAN_POINT('',(8.,-2.32153024911032,-8.4202732340176)) ;
#143583=CARTESIAN_POINT('Origin',(8.,-2.15,-8.52311959340942)) ;
#143584=CARTESIAN_POINT('',(8.,-2.32153024911032,-6.8197267659824)) ;
#143585=CARTESIAN_POINT('Origin',(8.,-3.65625,-7.62)) ;
#143586=CARTESIAN_POINT('',(8.,-2.35,-6.71688040659058)) ;
#143587=CARTESIAN_POINT('Origin',(8.,-2.15,-6.71688040659058)) ;
#143588=CARTESIAN_POINT('',(8.,-2.35,-6.07)) ;
#143589=CARTESIAN_POINT('',(8.,-2.35,-6.07)) ;
#143590=CARTESIAN_POINT('',(8.,-2.15,-5.87)) ;
#143591=CARTESIAN_POINT('Origin',(8.,-2.15,-6.07)) ;
#143592=CARTESIAN_POINT('',(8.,1.9,-5.87)) ;
#143593=CARTESIAN_POINT('',(8.,1.9,-2.06)) ;
#143594=CARTESIAN_POINT('',(8.,2.1,-2.26)) ;
#143595=CARTESIAN_POINT('Origin',(8.,1.9,-2.26)) ;
#143596=CARTESIAN_POINT('',(8.,2.1,-3.21)) ;
#143597=CARTESIAN_POINT('',(8.,2.1,-3.21)) ;
#143598=CARTESIAN_POINT('',(8.,2.4,-3.21)) ;
#143599=CARTESIAN_POINT('',(8.,2.4,-3.21)) ;
#143600=CARTESIAN_POINT('',(8.,2.4,-3.10142135623731)) ;
#143601=CARTESIAN_POINT('',(8.,2.4,-3.10142135623731)) ;
#143602=CARTESIAN_POINT('',(8.,2.45857864376269,-2.96)) ;
#143603=CARTESIAN_POINT('Origin',(8.,2.6,-3.10142135623731)) ;
#143604=CARTESIAN_POINT('',(8.,3.00857864376269,-2.41)) ;
#143605=CARTESIAN_POINT('',(8.,3.00857864376269,-2.41)) ;
#143606=CARTESIAN_POINT('',(8.,3.35,-2.55142135623731)) ;
#143607=CARTESIAN_POINT('Origin',(8.,3.15,-2.55142135623731)) ;
#143608=CARTESIAN_POINT('',(8.,3.35,-5.06857864376269)) ;
#143609=CARTESIAN_POINT('',(8.,2.45857864376269,-4.66)) ;
#143610=CARTESIAN_POINT('',(8.,2.45857864376269,-4.66)) ;
#143611=CARTESIAN_POINT('',(8.,2.4,-4.51857864376269)) ;
#143612=CARTESIAN_POINT('Origin',(8.,2.6,-4.51857864376269)) ;
#143613=CARTESIAN_POINT('',(8.,2.4,-4.41)) ;
#143614=CARTESIAN_POINT('',(8.,2.4,-4.41)) ;
#143615=CARTESIAN_POINT('',(8.,2.1,-4.41)) ;
#143616=CARTESIAN_POINT('',(8.,2.1,-4.41)) ;
#143617=CARTESIAN_POINT('',(8.,2.1,-5.36)) ;
#143618=CARTESIAN_POINT('',(8.,2.1,-5.36)) ;
#143619=CARTESIAN_POINT('',(8.,1.9,-5.56)) ;
#143620=CARTESIAN_POINT('Origin',(8.,1.9,-5.36)) ;
#143621=CARTESIAN_POINT('',(8.,-2.15,-5.56)) ;
#143622=CARTESIAN_POINT('',(8.,-2.15,-5.56)) ;
#143623=CARTESIAN_POINT('',(8.,-2.35,-5.36)) ;
#143624=CARTESIAN_POINT('Origin',(8.,-2.15,-5.36)) ;
#143625=CARTESIAN_POINT('',(8.,-2.35,-4.71311959340942)) ;
#143626=CARTESIAN_POINT('',(8.,-2.35,-4.71311959340942)) ;
#143627=CARTESIAN_POINT('',(8.,-2.32153024911032,-4.6102732340176)) ;
#143628=CARTESIAN_POINT('Origin',(8.,-2.15,-4.71311959340942)) ;
#143629=CARTESIAN_POINT('',(8.,-2.32153024911032,-3.0097267659824)) ;
#143630=CARTESIAN_POINT('Origin',(8.,-3.65625,-3.81)) ;
#143631=CARTESIAN_POINT('',(8.,-2.35,-2.90688040659058)) ;
#143632=CARTESIAN_POINT('Origin',(8.,-2.15,-2.90688040659058)) ;
#143633=CARTESIAN_POINT('',(8.,-2.35,-2.26)) ;
#143634=CARTESIAN_POINT('',(8.,-2.35,-2.26)) ;
#143635=CARTESIAN_POINT('',(8.,-2.15,-2.06)) ;
#143636=CARTESIAN_POINT('Origin',(8.,-2.15,-2.26)) ;
#143637=CARTESIAN_POINT('',(8.,1.9,-2.06)) ;
#143638=CARTESIAN_POINT('',(8.,1.9,1.75)) ;
#143639=CARTESIAN_POINT('',(8.,2.1,1.55)) ;
#143640=CARTESIAN_POINT('Origin',(8.,1.9,1.55)) ;
#143641=CARTESIAN_POINT('',(8.,2.1,0.6)) ;
#143642=CARTESIAN_POINT('',(8.,2.1,0.600000000000003)) ;
#143643=CARTESIAN_POINT('',(8.,2.4,0.6)) ;
#143644=CARTESIAN_POINT('',(8.,2.4,0.6)) ;
#143645=CARTESIAN_POINT('',(8.,2.4,0.70857864376269)) ;
#143646=CARTESIAN_POINT('',(8.,2.4,0.70857864376269)) ;
#143647=CARTESIAN_POINT('',(8.,2.45857864376269,0.849999999999999)) ;
#143648=CARTESIAN_POINT('Origin',(8.,2.6,0.70857864376269)) ;
#143649=CARTESIAN_POINT('',(8.,3.00857864376269,1.4)) ;
#143650=CARTESIAN_POINT('',(8.,3.00857864376269,1.4)) ;
#143651=CARTESIAN_POINT('',(8.,3.35,1.25857864376269)) ;
#143652=CARTESIAN_POINT('Origin',(8.,3.15,1.25857864376269)) ;
#143653=CARTESIAN_POINT('',(8.,3.35,-1.25857864376269)) ;
#143654=CARTESIAN_POINT('',(8.,2.45857864376269,-0.850000000000001)) ;
#143655=CARTESIAN_POINT('',(8.,2.45857864376269,-0.85)) ;
#143656=CARTESIAN_POINT('',(8.,2.4,-0.70857864376269)) ;
#143657=CARTESIAN_POINT('Origin',(8.,2.6,-0.70857864376269)) ;
#143658=CARTESIAN_POINT('',(8.,2.4,-0.6)) ;
#143659=CARTESIAN_POINT('',(8.,2.4,-0.6)) ;
#143660=CARTESIAN_POINT('',(8.,2.1,-0.6)) ;
#143661=CARTESIAN_POINT('',(8.,2.1,-0.6)) ;
#143662=CARTESIAN_POINT('',(8.,2.1,-1.55)) ;
#143663=CARTESIAN_POINT('',(8.,2.1,-1.55)) ;
#143664=CARTESIAN_POINT('',(8.,1.9,-1.75)) ;
#143665=CARTESIAN_POINT('Origin',(8.,1.9,-1.55)) ;
#143666=CARTESIAN_POINT('',(8.,-2.15,-1.75)) ;
#143667=CARTESIAN_POINT('',(8.,-2.15,-1.75)) ;
#143668=CARTESIAN_POINT('',(8.,-2.35,-1.55)) ;
#143669=CARTESIAN_POINT('Origin',(8.,-2.15,-1.55)) ;
#143670=CARTESIAN_POINT('',(8.,-2.35,-0.903119593409422)) ;
#143671=CARTESIAN_POINT('',(8.,-2.35,-0.903119593409422)) ;
#143672=CARTESIAN_POINT('',(8.,-2.32153024911032,-0.800273234017602)) ;
#143673=CARTESIAN_POINT('Origin',(8.,-2.15,-0.903119593409422)) ;
#143674=CARTESIAN_POINT('',(8.,-2.32153024911032,0.800273234017602)) ;
#143675=CARTESIAN_POINT('Origin',(8.,-3.65625,0.)) ;
#143676=CARTESIAN_POINT('',(8.,-2.35,0.903119593409422)) ;
#143677=CARTESIAN_POINT('Origin',(8.,-2.15,0.903119593409422)) ;
#143678=CARTESIAN_POINT('',(8.,-2.35,1.55)) ;
#143679=CARTESIAN_POINT('',(8.,-2.35,1.55)) ;
#143680=CARTESIAN_POINT('',(8.,-2.15,1.75)) ;
#143681=CARTESIAN_POINT('Origin',(8.,-2.15,1.55)) ;
#143682=CARTESIAN_POINT('',(8.,1.9,1.75)) ;
#143683=CARTESIAN_POINT('Origin',(7.9,-2.9,-36.89)) ;
#143684=CARTESIAN_POINT('',(7.9,4.15,-36.89)) ;
#143685=CARTESIAN_POINT('',(7.9,-2.9,-36.89)) ;
#143686=CARTESIAN_POINT('',(7.9,-2.9,-36.89)) ;
#143687=CARTESIAN_POINT('',(-1.1,-2.9,-36.89)) ;
#143688=CARTESIAN_POINT('',(-1.1,-2.9,-36.89)) ;
#143689=CARTESIAN_POINT('',(-1.1,4.15,-36.89)) ;
#143690=CARTESIAN_POINT('',(-1.1,4.15,-36.89)) ;
#143691=CARTESIAN_POINT('',(4.35,4.15,-36.89)) ;
#143692=CARTESIAN_POINT('',(4.35,4.15,-36.89)) ;
#143693=CARTESIAN_POINT('',(4.55,4.35,-36.89)) ;
#143694=CARTESIAN_POINT('Origin',(4.35,4.35,-36.89)) ;
#143695=CARTESIAN_POINT('',(4.55,4.55,-36.89)) ;
#143696=CARTESIAN_POINT('',(4.55,4.55,-36.89)) ;
#143697=CARTESIAN_POINT('',(4.75,4.55,-36.89)) ;
#143698=CARTESIAN_POINT('',(4.75,4.55,-36.89)) ;
#143699=CARTESIAN_POINT('',(4.75,4.35,-36.89)) ;
#143700=CARTESIAN_POINT('',(4.75,4.35,-36.89)) ;
#143701=CARTESIAN_POINT('',(4.95,4.15,-36.89)) ;
#143702=CARTESIAN_POINT('Origin',(4.95,4.35,-36.89)) ;
#143703=CARTESIAN_POINT('',(7.9,4.15,-36.89)) ;
#143704=CARTESIAN_POINT('Origin',(7.9,-2.9,2.6)) ;
#143705=CARTESIAN_POINT('',(-1.1,4.15,2.6)) ;
#143706=CARTESIAN_POINT('',(-1.1,-2.9,2.6)) ;
#143707=CARTESIAN_POINT('',(-1.1,-2.9,2.6)) ;
#143708=CARTESIAN_POINT('',(7.9,-2.9,2.6)) ;
#143709=CARTESIAN_POINT('',(7.9,-2.9,2.6)) ;
#143710=CARTESIAN_POINT('',(7.9,4.15,2.6)) ;
#143711=CARTESIAN_POINT('',(7.9,-2.9,2.6)) ;
#143712=CARTESIAN_POINT('',(4.95,4.15,2.6)) ;
#143713=CARTESIAN_POINT('',(7.9,4.15,2.6)) ;
#143714=CARTESIAN_POINT('',(4.75,4.35,2.6)) ;
#143715=CARTESIAN_POINT('Origin',(4.95,4.35,2.6)) ;
#143716=CARTESIAN_POINT('',(4.75,4.55,2.6)) ;
#143717=CARTESIAN_POINT('',(4.74999999999997,-2.89999999999999,2.6)) ;
#143718=CARTESIAN_POINT('',(4.55,4.55,2.6)) ;
#143719=CARTESIAN_POINT('',(7.9,4.55,2.6)) ;
#143720=CARTESIAN_POINT('',(4.55,4.35,2.6)) ;
#143721=CARTESIAN_POINT('',(4.55,-2.9,2.6)) ;
#143722=CARTESIAN_POINT('',(4.35,4.15,2.6)) ;
#143723=CARTESIAN_POINT('Origin',(4.35,4.35,2.6)) ;
#143724=CARTESIAN_POINT('',(7.9,4.15,2.6)) ;
#143725=CARTESIAN_POINT('Origin',(-0.999999999999999,-1.59070596587277E-16,
0.)) ;
#143726=CARTESIAN_POINT('',(-0.999999999999999,-1.9,0.6)) ;
#143727=CARTESIAN_POINT('',(-0.999999999999999,-1.9,1.275)) ;
#143728=CARTESIAN_POINT('',(-0.999999999999999,-1.9,1.375)) ;
#143729=CARTESIAN_POINT('',(-0.999999999999999,1.15,1.275)) ;
#143730=CARTESIAN_POINT('',(-0.999999999999999,-2.89663358890161E-17,1.275)) ;
#143731=CARTESIAN_POINT('',(-0.999999999999999,1.15,-1.275)) ;
#143732=CARTESIAN_POINT('',(-0.999999999999999,1.15,0.)) ;
#143733=CARTESIAN_POINT('',(-0.999999999999999,-1.9,-1.275)) ;
#143734=CARTESIAN_POINT('',(-0.999999999999999,-2.24122726936407E-16,-1.275)) ;
#143735=CARTESIAN_POINT('',(-0.999999999999999,-1.9,-0.6)) ;
#143736=CARTESIAN_POINT('',(-0.999999999999999,-1.9,-0.5)) ;
#143737=CARTESIAN_POINT('',(-0.999999999999999,0.4,-0.6)) ;
#143738=CARTESIAN_POINT('',(-0.999999999999999,0.5,-0.6)) ;
#143739=CARTESIAN_POINT('',(-0.999999999999999,0.6,-0.4)) ;
#143740=CARTESIAN_POINT('Origin',(-0.999999999999999,0.4,-0.4)) ;
#143741=CARTESIAN_POINT('',(-0.999999999999999,0.6,0.4)) ;
#143742=CARTESIAN_POINT('',(-0.999999999999999,0.6,0.5)) ;
#143743=CARTESIAN_POINT('',(-0.999999999999999,0.4,0.6)) ;
#143744=CARTESIAN_POINT('Origin',(-0.999999999999999,0.4,0.4)) ;
#143745=CARTESIAN_POINT('',(-0.999999999999999,-2.,0.6)) ;
#143746=CARTESIAN_POINT('Origin',(0.600000000000001,-2.,-0.5)) ;
#143747=CARTESIAN_POINT('',(0.500000000000001,-2.,-0.6)) ;
#143748=CARTESIAN_POINT('',(-0.899999999999999,-2.,-0.6)) ;
#143749=CARTESIAN_POINT('',(0.600000000000001,-2.,-0.6)) ;
#143750=CARTESIAN_POINT('',(-0.899999999999999,-2.,-1.275)) ;
#143751=CARTESIAN_POINT('',(-0.899999999999999,-2.,-1.375)) ;
#143752=CARTESIAN_POINT('',(0.500000000000001,-2.,-1.275)) ;
#143753=CARTESIAN_POINT('',(0.600000000000001,-2.,-1.275)) ;
#143754=CARTESIAN_POINT('',(0.500000000000001,-2.,-0.5)) ;
#143755=CARTESIAN_POINT('Origin',(0.600000000000001,0.5,-0.5)) ;
#143756=CARTESIAN_POINT('',(-0.899999999999999,0.4,-0.5)) ;
#143757=CARTESIAN_POINT('',(-0.999999999999999,0.4,-0.5)) ;
#143758=CARTESIAN_POINT('',(-0.899999999999999,-1.9,-0.5)) ;
#143759=CARTESIAN_POINT('',(-0.899999999999999,-2.,-0.5)) ;
#143760=CARTESIAN_POINT('',(0.600000000000001,-1.9,-0.5)) ;
#143761=CARTESIAN_POINT('Origin',(0.600000000000001,0.5,0.5)) ;
#143762=CARTESIAN_POINT('',(0.500000000000001,0.5,0.4)) ;
#143763=CARTESIAN_POINT('',(-0.899999999999999,0.5,0.4)) ;
#143764=CARTESIAN_POINT('',(-0.999999999999999,0.5,0.4)) ;
#143765=CARTESIAN_POINT('',(-0.899999999999999,0.5,-0.4)) ;
#143766=CARTESIAN_POINT('',(-0.899999999999999,0.5,-0.5)) ;
#143767=CARTESIAN_POINT('',(0.500000000000001,0.5,-0.4)) ;
#143768=CARTESIAN_POINT('',(0.600000000000001,0.5,-0.4)) ;
#143769=CARTESIAN_POINT('',(0.500000000000001,0.5,0.5)) ;
#143770=CARTESIAN_POINT('Origin',(0.600000000000001,-2.,0.5)) ;
#143771=CARTESIAN_POINT('',(0.500000000000001,-1.9,0.5)) ;
#143772=CARTESIAN_POINT('',(-0.899999999999999,-1.9,0.5)) ;
#143773=CARTESIAN_POINT('',(0.600000000000001,-1.9,0.5)) ;
#143774=CARTESIAN_POINT('',(-0.899999999999999,0.4,0.5)) ;
#143775=CARTESIAN_POINT('',(-0.899999999999999,0.5,0.5)) ;
#143776=CARTESIAN_POINT('',(0.500000000000001,0.4,0.5)) ;
#143777=CARTESIAN_POINT('',(0.600000000000001,0.4,0.5)) ;
#143778=CARTESIAN_POINT('',(0.500000000000001,-2.,0.5)) ;
#143779=CARTESIAN_POINT('Origin',(0.600000000000001,-2.,1.375)) ;
#143780=CARTESIAN_POINT('',(0.500000000000001,-2.,1.275)) ;
#143781=CARTESIAN_POINT('',(-0.899999999999999,-2.,1.275)) ;
#143782=CARTESIAN_POINT('',(-0.999999999999999,-2.,1.275)) ;
#143783=CARTESIAN_POINT('',(-0.899999999999999,-2.,0.6)) ;
#143784=CARTESIAN_POINT('',(-0.899999999999999,-2.,0.5)) ;
#143785=CARTESIAN_POINT('',(0.500000000000001,-2.,0.6)) ;
#143786=CARTESIAN_POINT('',(0.600000000000001,-2.,0.6)) ;
#143787=CARTESIAN_POINT('',(0.500000000000001,-2.,1.375)) ;
#143788=CARTESIAN_POINT('Origin',(1.4,2.1,0.6)) ;
#143789=CARTESIAN_POINT('',(1.5,2.,0.6)) ;
#143790=CARTESIAN_POINT('',(7.9,2.,0.6)) ;
#143791=CARTESIAN_POINT('',(1.4,2.,0.6)) ;
#143792=CARTESIAN_POINT('',(1.5,2.1,0.5)) ;
#143793=CARTESIAN_POINT('Origin',(1.5,2.1,0.6)) ;
#143794=CARTESIAN_POINT('',(7.9,2.1,0.5)) ;
#143795=CARTESIAN_POINT('',(1.4,2.1,0.5)) ;
#143796=CARTESIAN_POINT('Origin',(7.9,2.1,0.6)) ;
#143797=CARTESIAN_POINT('Origin',(1.4,2.4,0.5)) ;
#143798=CARTESIAN_POINT('',(1.5,2.4,0.5)) ;
#143799=CARTESIAN_POINT('',(1.5,2.4,0.5)) ;
#143800=CARTESIAN_POINT('',(7.9,2.4,0.5)) ;
#143801=CARTESIAN_POINT('',(1.4,2.4,0.5)) ;
#143802=CARTESIAN_POINT('',(7.9,2.1,0.5)) ;
#143803=CARTESIAN_POINT('Origin',(1.4,2.4,0.6)) ;
#143804=CARTESIAN_POINT('',(1.5,2.5,0.6)) ;
#143805=CARTESIAN_POINT('Origin',(1.5,2.4,0.6)) ;
#143806=CARTESIAN_POINT('',(7.9,2.5,0.6)) ;
#143807=CARTESIAN_POINT('',(1.4,2.5,0.6)) ;
#143808=CARTESIAN_POINT('Origin',(7.9,2.4,0.6)) ;
#143809=CARTESIAN_POINT('Origin',(1.4,2.5,0.70857864376269)) ;
#143810=CARTESIAN_POINT('',(1.5,2.5,0.70857864376269)) ;
#143811=CARTESIAN_POINT('',(1.5,2.5,0.70857864376269)) ;
#143812=CARTESIAN_POINT('',(7.9,2.5,0.70857864376269)) ;
#143813=CARTESIAN_POINT('',(1.4,2.5,0.70857864376269)) ;
#143814=CARTESIAN_POINT('',(7.9,2.5,0.6)) ;
#143815=CARTESIAN_POINT('Origin',(1.4,2.6,0.70857864376269)) ;
#143816=CARTESIAN_POINT('',(1.5,2.52928932188135,0.779289321881344)) ;
#143817=CARTESIAN_POINT('Origin',(1.5,2.6,0.70857864376269)) ;
#143818=CARTESIAN_POINT('',(7.9,2.52928932188135,0.779289321881344)) ;
#143819=CARTESIAN_POINT('',(1.4,2.52928932188135,0.779289321881344)) ;
#143820=CARTESIAN_POINT('Origin',(7.9,2.6,0.70857864376269)) ;
#143821=CARTESIAN_POINT('Origin',(1.4,3.07928932188135,1.32928932188135)) ;
#143822=CARTESIAN_POINT('',(1.5,3.07928932188135,1.32928932188134)) ;
#143823=CARTESIAN_POINT('',(7.9,3.07928932188135,1.32928932188135)) ;
#143824=CARTESIAN_POINT('',(1.4,3.07928932188135,1.32928932188135)) ;
#143825=CARTESIAN_POINT('',(7.9,2.52928932188135,0.779289321881344)) ;
#143826=CARTESIAN_POINT('Origin',(1.4,3.15,1.25857864376269)) ;
#143827=CARTESIAN_POINT('',(7.9,3.25,1.25857864376269)) ;
#143828=CARTESIAN_POINT('',(1.4,3.25,1.25857864376269)) ;
#143829=CARTESIAN_POINT('Origin',(7.9,3.15,1.25857864376269)) ;
#143830=CARTESIAN_POINT('Origin',(1.4,3.25,-1.25857864376269)) ;
#143831=CARTESIAN_POINT('',(1.5,3.25,-1.25857864376269)) ;
#143832=CARTESIAN_POINT('',(7.9,3.25,1.25857864376269)) ;
#143833=CARTESIAN_POINT('Origin',(1.4,2.52928932188134,-0.779289321881346)) ;
#143834=CARTESIAN_POINT('',(1.5,2.52928932188134,-0.779289321881346)) ;
#143835=CARTESIAN_POINT('',(1.5,2.52928932188134,-0.779289321881346)) ;
#143836=CARTESIAN_POINT('',(7.9,2.52928932188134,-0.779289321881346)) ;
#143837=CARTESIAN_POINT('',(1.4,2.52928932188134,-0.779289321881346)) ;
#143838=CARTESIAN_POINT('',(7.9,3.07928932188135,-1.32928932188135)) ;
#143839=CARTESIAN_POINT('Origin',(1.4,2.6,-0.70857864376269)) ;
#143840=CARTESIAN_POINT('',(1.5,2.5,-0.70857864376269)) ;
#143841=CARTESIAN_POINT('Origin',(1.5,2.6,-0.70857864376269)) ;
#143842=CARTESIAN_POINT('',(7.9,2.5,-0.70857864376269)) ;
#143843=CARTESIAN_POINT('',(1.4,2.5,-0.70857864376269)) ;
#143844=CARTESIAN_POINT('Origin',(7.9,2.6,-0.70857864376269)) ;
#143845=CARTESIAN_POINT('Origin',(1.4,2.5,-0.6)) ;
#143846=CARTESIAN_POINT('',(1.5,2.5,-0.6)) ;
#143847=CARTESIAN_POINT('',(1.5,2.5,-0.6)) ;
#143848=CARTESIAN_POINT('',(7.9,2.5,-0.6)) ;
#143849=CARTESIAN_POINT('',(1.4,2.5,-0.6)) ;
#143850=CARTESIAN_POINT('',(7.9,2.5,-0.70857864376269)) ;
#143851=CARTESIAN_POINT('Origin',(1.4,2.4,-0.6)) ;
#143852=CARTESIAN_POINT('',(1.5,2.4,-0.5)) ;
#143853=CARTESIAN_POINT('Origin',(1.5,2.4,-0.6)) ;
#143854=CARTESIAN_POINT('',(7.9,2.4,-0.5)) ;
#143855=CARTESIAN_POINT('',(1.4,2.4,-0.5)) ;
#143856=CARTESIAN_POINT('Origin',(7.9,2.4,-0.6)) ;
#143857=CARTESIAN_POINT('Origin',(1.4,2.1,-0.5)) ;
#143858=CARTESIAN_POINT('',(1.5,2.1,-0.5)) ;
#143859=CARTESIAN_POINT('',(1.5,2.1,-0.5)) ;
#143860=CARTESIAN_POINT('',(7.9,2.1,-0.5)) ;
#143861=CARTESIAN_POINT('',(1.4,2.1,-0.5)) ;
#143862=CARTESIAN_POINT('',(7.9,2.4,-0.5)) ;
#143863=CARTESIAN_POINT('Origin',(1.4,2.1,-0.6)) ;
#143864=CARTESIAN_POINT('',(1.5,2.,-0.6)) ;
#143865=CARTESIAN_POINT('Origin',(1.5,2.1,-0.6)) ;
#143866=CARTESIAN_POINT('',(7.9,2.,-0.6)) ;
#143867=CARTESIAN_POINT('',(1.4,2.,-0.6)) ;
#143868=CARTESIAN_POINT('Origin',(7.9,2.1,-0.6)) ;
#143869=CARTESIAN_POINT('Origin',(1.4,2.,-0.6)) ;
#143870=CARTESIAN_POINT('',(1.5,2.,-1.55)) ;
#143871=CARTESIAN_POINT('',(1.5,2.,-1.55)) ;
#143872=CARTESIAN_POINT('',(7.9,2.,-1.55)) ;
#143873=CARTESIAN_POINT('',(1.4,2.,-1.55)) ;
#143874=CARTESIAN_POINT('',(7.9,2.,-0.6)) ;
#143875=CARTESIAN_POINT('Origin',(1.4,1.9,-1.55)) ;
#143876=CARTESIAN_POINT('',(1.5,1.9,-1.65)) ;
#143877=CARTESIAN_POINT('Origin',(1.5,1.9,-1.55)) ;
#143878=CARTESIAN_POINT('',(7.9,1.9,-1.65)) ;
#143879=CARTESIAN_POINT('',(1.4,1.9,-1.65)) ;
#143880=CARTESIAN_POINT('Origin',(7.9,1.9,-1.55)) ;
#143881=CARTESIAN_POINT('Origin',(1.4,1.9,-1.65)) ;
#143882=CARTESIAN_POINT('',(1.5,-2.15,-1.65)) ;
#143883=CARTESIAN_POINT('',(1.5,-2.15,-1.65)) ;
#143884=CARTESIAN_POINT('',(7.9,-2.15,-1.65)) ;
#143885=CARTESIAN_POINT('',(1.4,-2.15,-1.65)) ;
#143886=CARTESIAN_POINT('',(7.9,1.9,-1.65)) ;
#143887=CARTESIAN_POINT('Origin',(1.4,-2.15,-1.55)) ;
#143888=CARTESIAN_POINT('',(1.5,-2.25,-1.55)) ;
#143889=CARTESIAN_POINT('Origin',(1.5,-2.15,-1.55)) ;
#143890=CARTESIAN_POINT('',(7.9,-2.25,-1.55)) ;
#143891=CARTESIAN_POINT('',(1.4,-2.25,-1.55)) ;
#143892=CARTESIAN_POINT('Origin',(7.9,-2.15,-1.55)) ;
#143893=CARTESIAN_POINT('Origin',(1.4,-2.25,-0.903119593409422)) ;
#143894=CARTESIAN_POINT('',(1.5,-2.25,-0.903119593409422)) ;
#143895=CARTESIAN_POINT('',(1.5,-2.25,-0.903119593409423)) ;
#143896=CARTESIAN_POINT('',(7.9,-2.25,-0.903119593409422)) ;
#143897=CARTESIAN_POINT('',(1.4,-2.25,-0.903119593409422)) ;
#143898=CARTESIAN_POINT('',(7.9,-2.25,-1.55)) ;
#143899=CARTESIAN_POINT('Origin',(1.4,-2.15,-0.903119593409422)) ;
#143900=CARTESIAN_POINT('',(1.5,-2.23576512455516,-0.851696413713512)) ;
#143901=CARTESIAN_POINT('Origin',(1.5,-2.15,-0.903119593409422)) ;
#143902=CARTESIAN_POINT('',(7.9,-2.23576512455516,-0.851696413713512)) ;
#143903=CARTESIAN_POINT('',(1.4,-2.23576512455516,-0.851696413713512)) ;
#143904=CARTESIAN_POINT('Origin',(7.9,-2.15,-0.903119593409422)) ;
#143905=CARTESIAN_POINT('Origin',(1.4,-3.65625,0.)) ;
#143906=CARTESIAN_POINT('',(1.5,-2.23576512455516,0.851696413713512)) ;
#143907=CARTESIAN_POINT('Origin',(1.5,-3.65625,0.)) ;
#143908=CARTESIAN_POINT('',(7.9,-2.23576512455516,0.851696413713512)) ;
#143909=CARTESIAN_POINT('',(1.4,-2.23576512455516,0.851696413713512)) ;
#143910=CARTESIAN_POINT('Origin',(7.9,-3.65625,0.)) ;
#143911=CARTESIAN_POINT('Origin',(1.4,-2.15,0.903119593409422)) ;
#143912=CARTESIAN_POINT('',(1.5,-2.25,0.903119593409422)) ;
#143913=CARTESIAN_POINT('Origin',(1.5,-2.15,0.903119593409422)) ;
#143914=CARTESIAN_POINT('',(7.9,-2.25,0.903119593409422)) ;
#143915=CARTESIAN_POINT('',(1.4,-2.25,0.903119593409422)) ;
#143916=CARTESIAN_POINT('Origin',(7.9,-2.15,0.903119593409422)) ;
#143917=CARTESIAN_POINT('Origin',(1.4,-2.25,1.55)) ;
#143918=CARTESIAN_POINT('',(1.5,-2.25,1.55)) ;
#143919=CARTESIAN_POINT('',(1.5,-2.25,1.55)) ;
#143920=CARTESIAN_POINT('',(7.9,-2.25,1.55)) ;
#143921=CARTESIAN_POINT('',(1.4,-2.25,1.55)) ;
#143922=CARTESIAN_POINT('',(7.9,-2.25,0.903119593409422)) ;
#143923=CARTESIAN_POINT('Origin',(1.4,-2.15,1.55)) ;
#143924=CARTESIAN_POINT('',(1.5,-2.15,1.65)) ;
#143925=CARTESIAN_POINT('Origin',(1.5,-2.15,1.55)) ;
#143926=CARTESIAN_POINT('',(7.9,-2.15,1.65)) ;
#143927=CARTESIAN_POINT('',(1.4,-2.15,1.65)) ;
#143928=CARTESIAN_POINT('Origin',(7.9,-2.15,1.55)) ;
#143929=CARTESIAN_POINT('Origin',(1.4,1.9,1.65)) ;
#143930=CARTESIAN_POINT('',(1.5,1.9,1.65)) ;
#143931=CARTESIAN_POINT('',(1.5,1.9,1.65)) ;
#143932=CARTESIAN_POINT('',(7.9,1.9,1.65)) ;
#143933=CARTESIAN_POINT('',(1.4,1.9,1.65)) ;
#143934=CARTESIAN_POINT('',(7.9,-2.15,1.65)) ;
#143935=CARTESIAN_POINT('Origin',(1.4,1.9,1.55)) ;
#143936=CARTESIAN_POINT('',(1.5,2.,1.55)) ;
#143937=CARTESIAN_POINT('Origin',(1.5,1.9,1.55)) ;
#143938=CARTESIAN_POINT('',(7.9,2.,1.55)) ;
#143939=CARTESIAN_POINT('',(1.4,2.,1.55)) ;
#143940=CARTESIAN_POINT('Origin',(7.9,1.9,1.55)) ;
#143941=CARTESIAN_POINT('Origin',(1.4,2.,1.55)) ;
#143942=CARTESIAN_POINT('',(1.5,2.,0.6)) ;
#143943=CARTESIAN_POINT('',(7.9,2.,1.55)) ;
#143944=CARTESIAN_POINT('Origin',(1.4,2.1,0.6)) ;
#143945=CARTESIAN_POINT('',(1.4,2.6,0.6)) ;
#143946=CARTESIAN_POINT('',(1.4,2.4,0.4)) ;
#143947=CARTESIAN_POINT('Origin',(1.4,2.4,0.6)) ;
#143948=CARTESIAN_POINT('',(1.4,2.1,0.4)) ;
#143949=CARTESIAN_POINT('',(1.4,2.1,0.4)) ;
#143950=CARTESIAN_POINT('',(1.4,1.9,0.6)) ;
#143951=CARTESIAN_POINT('Origin',(1.4,2.1,0.6)) ;
#143952=CARTESIAN_POINT('',(1.4,1.9,1.55)) ;
#143953=CARTESIAN_POINT('',(1.4,1.9,1.55)) ;
#143954=CARTESIAN_POINT('',(1.4,-2.15,1.55)) ;
#143955=CARTESIAN_POINT('',(1.4,-2.15,1.55)) ;
#143956=CARTESIAN_POINT('',(1.4,-2.15,0.903119593409422)) ;
#143957=CARTESIAN_POINT('',(1.4,-2.15,0.903119593409422)) ;
#143958=CARTESIAN_POINT('',(1.4,-2.15,-0.903119593409422)) ;
#143959=CARTESIAN_POINT('Origin',(1.4,-3.65625,0.)) ;
#143960=CARTESIAN_POINT('',(1.4,-2.15,-1.55)) ;
#143961=CARTESIAN_POINT('',(1.4,-2.15,-1.55)) ;
#143962=CARTESIAN_POINT('',(1.4,1.9,-1.55)) ;
#143963=CARTESIAN_POINT('',(1.4,1.9,-1.55)) ;
#143964=CARTESIAN_POINT('',(1.4,1.9,-0.6)) ;
#143965=CARTESIAN_POINT('',(1.4,1.9,-0.6)) ;
#143966=CARTESIAN_POINT('',(1.4,2.1,-0.4)) ;
#143967=CARTESIAN_POINT('Origin',(1.4,2.1,-0.6)) ;
#143968=CARTESIAN_POINT('',(1.4,2.4,-0.4)) ;
#143969=CARTESIAN_POINT('',(1.4,2.4,-0.4)) ;
#143970=CARTESIAN_POINT('',(1.4,2.6,-0.6)) ;
#143971=CARTESIAN_POINT('Origin',(1.4,2.4,-0.6)) ;
#143972=CARTESIAN_POINT('',(1.4,2.6,-0.70857864376269)) ;
#143973=CARTESIAN_POINT('',(1.4,2.6,-0.70857864376269)) ;
#143974=CARTESIAN_POINT('',(1.4,3.15,-1.25857864376269)) ;
#143975=CARTESIAN_POINT('',(1.4,3.15,-1.25857864376269)) ;
#143976=CARTESIAN_POINT('',(1.4,3.15,1.25857864376269)) ;
#143977=CARTESIAN_POINT('',(1.4,2.6,0.708578643762689)) ;
#143978=CARTESIAN_POINT('',(1.4,2.6,0.708578643762689)) ;
#143979=CARTESIAN_POINT('',(1.4,2.6,0.6)) ;
#143980=CARTESIAN_POINT('Origin',(2.4,0.,0.)) ;
#143981=CARTESIAN_POINT('',(2.4,0.3,0.4)) ;
#143982=CARTESIAN_POINT('',(2.4,-0.3,0.4)) ;
#143983=CARTESIAN_POINT('',(2.4,0.,0.4)) ;
#143984=CARTESIAN_POINT('',(2.4,0.4,0.3)) ;
#143985=CARTESIAN_POINT('Origin',(2.4,0.3,0.3)) ;
#143986=CARTESIAN_POINT('',(2.4,0.4,-0.3)) ;
#143987=CARTESIAN_POINT('',(2.4,0.4,0.)) ;
#143988=CARTESIAN_POINT('',(2.4,0.3,-0.4)) ;
#143989=CARTESIAN_POINT('Origin',(2.4,0.3,-0.3)) ;
#143990=CARTESIAN_POINT('',(2.4,-0.3,-0.4)) ;
#143991=CARTESIAN_POINT('',(2.4,0.,-0.4)) ;
#143992=CARTESIAN_POINT('',(2.4,-0.4,-0.3)) ;
#143993=CARTESIAN_POINT('Origin',(2.4,-0.3,-0.3)) ;
#143994=CARTESIAN_POINT('',(2.4,-0.4,0.3)) ;
#143995=CARTESIAN_POINT('',(2.4,-0.4,0.)) ;
#143996=CARTESIAN_POINT('Origin',(2.4,-0.3,0.3)) ;
#143997=CARTESIAN_POINT('Origin',(-0.899999999999999,-2.,0.6)) ;
#143998=CARTESIAN_POINT('Origin',(-0.899999999999999,0.4,0.6)) ;
#143999=CARTESIAN_POINT('Origin',(-0.899999999999999,-1.9,0.6)) ;
#144000=CARTESIAN_POINT('Origin',(0.600000000000001,0.4,0.4)) ;
#144001=CARTESIAN_POINT('Origin',(0.500000000000001,0.4,0.4)) ;
#144002=CARTESIAN_POINT('Origin',(-0.899999999999999,0.4,0.4)) ;
#144003=CARTESIAN_POINT('Origin',(0.500000000000001,0.4,0.4)) ;
#144004=CARTESIAN_POINT('',(0.600000000000001,0.4,0.4)) ;
#144005=CARTESIAN_POINT('Origin',(0.500000000000001,0.4,0.4)) ;
#144006=CARTESIAN_POINT('Origin',(0.500000000000001,0.4,0.4)) ;
#144007=CARTESIAN_POINT('Origin',(-0.899999999999999,-1.9,0.6)) ;
#144008=CARTESIAN_POINT('Origin',(-0.899999999999999,-1.9,0.6)) ;
#144009=CARTESIAN_POINT('Origin',(-0.899999999999999,-1.9,0.6)) ;
#144010=CARTESIAN_POINT('Origin',(-0.899999999999999,0.4,0.4)) ;
#144011=CARTESIAN_POINT('Origin',(-0.899999999999999,0.6,0.4)) ;
#144012=CARTESIAN_POINT('Origin',(0.500000000000001,0.4,0.)) ;
#144013=CARTESIAN_POINT('Origin',(0.500000000000001,0.4,-0.4)) ;
#144014=CARTESIAN_POINT('',(0.600000000000001,0.4,-0.3)) ;
#144015=CARTESIAN_POINT('Ctrl Pts',(0.595612997216081,0.370705721320403,
-0.370705721320403)) ;
#144016=CARTESIAN_POINT('Ctrl Pts',(0.596180587760892,0.372558268494357,
-0.368855498832167)) ;
#144017=CARTESIAN_POINT('Ctrl Pts',(0.596672461925686,0.374355839771985,
-0.36691417986631)) ;
#144018=CARTESIAN_POINT('Ctrl Pts',(0.599015141889212,0.383869350930065,
-0.355764993656267)) ;
#144019=CARTESIAN_POINT('Ctrl Pts',(0.599609996542525,0.390224332900451,
-0.34497260265412)) ;
#144020=CARTESIAN_POINT('Ctrl Pts',(0.600050586298726,0.398117439141561,
-0.32233105320467)) ;
#144021=CARTESIAN_POINT('Ctrl Pts',(0.600000000000001,0.399999999999999,
-0.311201250633524)) ;
#144022=CARTESIAN_POINT('Ctrl Pts',(0.600000000000001,0.399999999999999,
-0.3)) ;
#144023=CARTESIAN_POINT('',(0.600000000000001,0.4,0.)) ;
#144024=CARTESIAN_POINT('Origin',(0.500000000000001,-4.5664044441154E-17,
0.4)) ;
#144025=CARTESIAN_POINT('',(0.500000000000001,0.394987437106619,0.3)) ;
#144026=CARTESIAN_POINT('Ctrl Pts',(0.500000000000001,0.394987437106619,
0.3)) ;
#144027=CARTESIAN_POINT('Ctrl Pts',(0.505940567948951,0.3955844866499,0.3)) ;
#144028=CARTESIAN_POINT('Ctrl Pts',(0.511931971019139,0.396132036079018,
0.300533699672039)) ;
#144029=CARTESIAN_POINT('Ctrl Pts',(0.517829015308548,0.396618246075354,
0.301602204226276)) ;
#144030=CARTESIAN_POINT('Ctrl Pts',(0.522982218721202,0.397043126556053,
0.30253592984289)) ;
#144031=CARTESIAN_POINT('Ctrl Pts',(0.528062648970231,0.397421319341388,
0.303877173202936)) ;
#144032=CARTESIAN_POINT('Ctrl Pts',(0.532978106724001,0.397751505046071,
0.305594256123367)) ;
#144033=CARTESIAN_POINT('Ctrl Pts',(0.538583536338965,0.398128038182999,
0.307552362150451)) ;
#144034=CARTESIAN_POINT('Ctrl Pts',(0.544059405914892,0.398447721828296,
0.310029991688954)) ;
#144035=CARTESIAN_POINT('Ctrl Pts',(0.549268572255782,0.398712331108984,
0.312979268057107)) ;
#144036=CARTESIAN_POINT('Ctrl Pts',(0.553856850427146,0.398945401221756,
0.315577015853159)) ;
#144037=CARTESIAN_POINT('Ctrl Pts',(0.558237825069326,0.399135987683843,
0.318539615020013)) ;
#144038=CARTESIAN_POINT('Ctrl Pts',(0.562333836086213,0.399290378266507,
0.32180477713583)) ;
#144039=CARTESIAN_POINT('Ctrl Pts',(0.566990328957893,0.399465895042381,
0.325516731047696)) ;
#144040=CARTESIAN_POINT('Ctrl Pts',(0.571349096493423,0.399597278936107,
0.329677193515201)) ;
#144041=CARTESIAN_POINT('Ctrl Pts',(0.575296920056712,0.399694832180837,
0.334194424020656)) ;
#144042=CARTESIAN_POINT('Ctrl Pts',(0.578744263667908,0.399780018245913,
0.338138988784921)) ;
#144043=CARTESIAN_POINT('Ctrl Pts',(0.58187831456043,0.399839626289636,
0.342354478157894)) ;
#144044=CARTESIAN_POINT('Ctrl Pts',(0.584648147334856,0.399882153365958,
0.346758182292707)) ;
#144045=CARTESIAN_POINT('Ctrl Pts',(0.587839270208173,0.399931148788079,
0.351831687495501)) ;
#144046=CARTESIAN_POINT('Ctrl Pts',(0.590595054415093,0.399958289583404,
0.357233363755549)) ;
#144047=CARTESIAN_POINT('Ctrl Pts',(0.592838618943104,0.399974357003159,
0.362838314990607)) ;
#144048=CARTESIAN_POINT('Ctrl Pts',(0.594777336851655,0.399988241245861,
0.367681687757603)) ;
#144049=CARTESIAN_POINT('Ctrl Pts',(0.596334051506189,0.399993946552814,
0.372675833772872)) ;
#144050=CARTESIAN_POINT('Ctrl Pts',(0.597488309822308,0.39999684570125,
0.377728281431604)) ;
#144051=CARTESIAN_POINT('Ctrl Pts',(0.598804024094401,0.400000150378306,
0.383487458039442)) ;
#144052=CARTESIAN_POINT('Ctrl Pts',(0.599612685195431,0.399999963509465,
0.389397156109403)) ;
#144053=CARTESIAN_POINT('Ctrl Pts',(0.599890230999721,0.399999993975383,
0.395315797738928)) ;
#144054=CARTESIAN_POINT('Ctrl Pts',(0.5999634645494,0.400000002014155,0.396877497210183)) ;
#144055=CARTESIAN_POINT('Ctrl Pts',(0.600000000000001,0.399999999999999,
0.398439778490821)) ;
#144056=CARTESIAN_POINT('Ctrl Pts',(0.600000000000001,0.399999999999999,
0.4)) ;
#144057=CARTESIAN_POINT('',(0.600000000000001,0.299999999999999,0.4)) ;
#144058=CARTESIAN_POINT('Ctrl Pts',(0.500000000000001,0.394987437106619,
0.3)) ;
#144059=CARTESIAN_POINT('Ctrl Pts',(0.500454935589698,0.395033159853734,
0.3)) ;
#144060=CARTESIAN_POINT('Ctrl Pts',(0.500909898680399,0.395078570329052,
0.300003104508874)) ;
#144061=CARTESIAN_POINT('Ctrl Pts',(0.502892456245148,0.395275075889088,
0.300030166058056)) ;
#144062=CARTESIAN_POINT('Ctrl Pts',(0.504418747482362,0.395422812032197,
0.300086014579005)) ;
#144063=CARTESIAN_POINT('Ctrl Pts',(0.508462199543372,0.395804395682036,
0.300326718943359)) ;
#144064=CARTESIAN_POINT('Ctrl Pts',(0.510974953343318,0.396031485023319,
0.300572060854946)) ;
#144065=CARTESIAN_POINT('Ctrl Pts',(0.521160739721334,0.396903453186241,
0.301957205508451)) ;
#144066=CARTESIAN_POINT('Ctrl Pts',(0.528708678528457,0.397444933153163,
0.303895782295333)) ;
#144067=CARTESIAN_POINT('Ctrl Pts',(0.54594320635814,0.398105551684111,
0.310535360548881)) ;
#144068=CARTESIAN_POINT('Ctrl Pts',(0.555229535466871,0.397987646678423,
0.315964641164077)) ;
#144069=CARTESIAN_POINT('Ctrl Pts',(0.571394604995807,0.395490482808029,
0.329224486636193)) ;
#144070=CARTESIAN_POINT('Ctrl Pts',(0.578055313702881,0.393198948698321,
0.336759254368297)) ;
#144071=CARTESIAN_POINT('Ctrl Pts',(0.58855913220255,0.385442756729278,
0.352607766016028)) ;
#144072=CARTESIAN_POINT('Ctrl Pts',(0.592167355639995,0.380240075126846,
0.360451734393248)) ;
#144073=CARTESIAN_POINT('Ctrl Pts',(0.597496615531129,0.365892753466911,
0.376074478204782)) ;
#144074=CARTESIAN_POINT('Ctrl Pts',(0.598734255154207,0.356660564300593,
0.38322725827313)) ;
#144075=CARTESIAN_POINT('Ctrl Pts',(0.600012754681692,0.335223914398488,
0.394417694134416)) ;
#144076=CARTESIAN_POINT('Ctrl Pts',(0.59999390055981,0.32265503709182,0.398338480634425)) ;
#144077=CARTESIAN_POINT('Ctrl Pts',(0.600000296204999,0.306106913582345,
0.399860373652956)) ;
#144078=CARTESIAN_POINT('Ctrl Pts',(0.600000000000001,0.303050992413431,
0.4)) ;
#144079=CARTESIAN_POINT('Ctrl Pts',(0.600000000000001,0.299999999999999,
0.4)) ;
#144080=CARTESIAN_POINT('',(0.600000000000001,-2.3980000991444E-17,0.4)) ;
#144081=CARTESIAN_POINT('Origin',(0.500000000000001,-1.9,0.4)) ;
#144082=CARTESIAN_POINT('Origin',(0.600000000000001,-1.9,0.6)) ;
#144083=CARTESIAN_POINT('Origin',(0.500000000000001,-1.9,0.6)) ;
#144084=CARTESIAN_POINT('Origin',(-0.899999999999999,-1.9,1.375)) ;
#144085=CARTESIAN_POINT('Origin',(-0.899999999999999,-1.9,1.275)) ;
#144086=CARTESIAN_POINT('Origin',(-0.899999999999999,0.6,0.5)) ;
#144087=CARTESIAN_POINT('Origin',(-0.899999999999999,0.6,-0.4)) ;
#144088=CARTESIAN_POINT('Origin',(0.600000000000001,0.4,-0.4)) ;
#144089=CARTESIAN_POINT('Origin',(0.500000000000001,0.4,-0.4)) ;
#144090=CARTESIAN_POINT('Origin',(-0.899999999999999,0.4,-0.4)) ;
#144091=CARTESIAN_POINT('Origin',(0.500000000000001,0.4,-0.4)) ;
#144092=CARTESIAN_POINT('Origin',(0.500000000000001,-1.9,0.6)) ;
#144093=CARTESIAN_POINT('Origin',(0.500000000000001,-2.1,0.6)) ;
#144094=CARTESIAN_POINT('Origin',(-0.899999999999999,-1.9,1.275)) ;
#144095=CARTESIAN_POINT('Origin',(-1.1,-1.9,1.275)) ;
#144096=CARTESIAN_POINT('Origin',(-0.899999999999999,-2.1,1.275)) ;
#144097=CARTESIAN_POINT('Origin',(-0.899999999999999,0.4,-0.4)) ;
#144098=CARTESIAN_POINT('Origin',(-0.899999999999999,0.4,-0.6)) ;
#144099=CARTESIAN_POINT('Origin',(0.500000000000001,-2.1,0.)) ;
#144100=CARTESIAN_POINT('Origin',(0.500000000000001,-2.1,1.275)) ;
#144101=CARTESIAN_POINT('Origin',(0.600000000000001,-2.1,1.275)) ;
#144102=CARTESIAN_POINT('Origin',(0.500000000000001,-2.1,1.275)) ;
#144103=CARTESIAN_POINT('Origin',(-1.1,-4.42727195005762E-17,1.275)) ;
#144104=CARTESIAN_POINT('',(-1.1,1.15,1.375)) ;
#144105=CARTESIAN_POINT('',(-1.1,1.25,1.375)) ;
#144106=CARTESIAN_POINT('Origin',(-1.1,1.15,1.275)) ;
#144107=CARTESIAN_POINT('Origin',(-0.899999999999999,0.5,-0.6)) ;
#144108=CARTESIAN_POINT('Origin',(-0.899999999999999,-1.9,-0.6)) ;
#144109=CARTESIAN_POINT('Origin',(0.600000000000001,-1.9,-0.6)) ;
#144110=CARTESIAN_POINT('Origin',(0.500000000000001,-1.9,-0.6)) ;
#144111=CARTESIAN_POINT('Origin',(-0.899999999999999,-1.9,-0.6)) ;
#144112=CARTESIAN_POINT('Origin',(0.500000000000001,-1.9,-0.6)) ;
#144113=CARTESIAN_POINT('Origin',(0.500000000000001,-2.1,-0.6)) ;
#144114=CARTESIAN_POINT('Origin',(0.500000000000001,-2.1,1.275)) ;
#144115=CARTESIAN_POINT('Origin',(0.500000000000001,-2.1,1.275)) ;
#144116=CARTESIAN_POINT('Origin',(-1.1,-2.9,1.475)) ;
#144117=CARTESIAN_POINT('Origin',(-1.1,-2.9,1.475)) ;
#144118=CARTESIAN_POINT('Origin',(-1.1,-2.9,1.475)) ;
#144119=CARTESIAN_POINT('Origin',(-1.1,1.25,1.475)) ;
#144120=CARTESIAN_POINT('Origin',(-1.1,1.15,1.475)) ;
#144121=CARTESIAN_POINT('Origin',(-1.1,1.15,1.275)) ;
#144122=CARTESIAN_POINT('',(-1.1,1.25,1.275)) ;
#144123=CARTESIAN_POINT('Origin',(-1.1,1.15,1.275)) ;
#144124=CARTESIAN_POINT('Origin',(-1.1,1.15,1.275)) ;
#144125=CARTESIAN_POINT('Origin',(-0.899999999999999,-1.9,-0.6)) ;
#144126=CARTESIAN_POINT('Origin',(-0.899999999999999,-1.9,-0.6)) ;
#144127=CARTESIAN_POINT('Origin',(0.500000000000001,-2.1,0.)) ;
#144128=CARTESIAN_POINT('Origin',(0.500000000000001,-2.1,-1.275)) ;
#144129=CARTESIAN_POINT('Origin',(0.500000000000001,1.36481920536411E-16,
1.275)) ;
#144130=CARTESIAN_POINT('Origin',(0.500000000000001,-2.9,1.275)) ;
#144131=CARTESIAN_POINT('Origin',(-0.999999999999999,-2.9,1.475)) ;
#144132=CARTESIAN_POINT('Origin',(0.500000000000001,-2.9,1.475)) ;
#144133=CARTESIAN_POINT('Origin',(-1.1,1.15,1.275)) ;
#144134=CARTESIAN_POINT('Origin',(-1.1,1.35,1.275)) ;
#144135=CARTESIAN_POINT('Origin',(-1.1,1.15,0.)) ;
#144136=CARTESIAN_POINT('',(-1.1,1.25,-1.275)) ;
#144137=CARTESIAN_POINT('',(-1.1,1.25,-1.375)) ;
#144138=CARTESIAN_POINT('Origin',(-1.1,1.15,-1.275)) ;
#144139=CARTESIAN_POINT('Origin',(-0.899999999999999,-1.9,-0.5)) ;
#144140=CARTESIAN_POINT('Origin',(-0.899999999999999,-1.9,-1.275)) ;
#144141=CARTESIAN_POINT('Origin',(-0.999999999999999,-2.1,-1.275)) ;
#144142=CARTESIAN_POINT('Origin',(0.500000000000001,-2.1,-1.275)) ;
#144143=CARTESIAN_POINT('Origin',(-0.899999999999999,-2.1,-1.275)) ;
#144144=CARTESIAN_POINT('Origin',(0.500000000000001,-2.1,-1.275)) ;
#144145=CARTESIAN_POINT('Origin',(0.500000000000001,-2.1,-1.275)) ;
#144146=CARTESIAN_POINT('Origin',(0.500000000000001,-2.9,1.275)) ;
#144147=CARTESIAN_POINT('Origin',(0.700000000000002,-2.9,1.275)) ;
#144148=CARTESIAN_POINT('Origin',(-1.1,1.35,-1.375)) ;
#144149=CARTESIAN_POINT('Origin',(-1.1,1.35,-1.275)) ;
#144150=CARTESIAN_POINT('Origin',(-1.1,1.15,-1.275)) ;
#144151=CARTESIAN_POINT('',(-1.1,1.15,-1.375)) ;
#144152=CARTESIAN_POINT('Origin',(-1.1,1.15,-1.275)) ;
#144153=CARTESIAN_POINT('Origin',(-1.1,1.15,-1.275)) ;
#144154=CARTESIAN_POINT('Origin',(-0.899999999999999,-1.9,-1.275)) ;
#144155=CARTESIAN_POINT('Origin',(-1.1,-1.9,-1.275)) ;
#144156=CARTESIAN_POINT('Origin',(0.500000000000001,-5.86744705109801E-17,
-1.275)) ;
#144157=CARTESIAN_POINT('Origin',(0.500000000000001,-2.9,-1.275)) ;
#144158=CARTESIAN_POINT('Origin',(0.700000000000002,-2.9,0.)) ;
#144159=CARTESIAN_POINT('Origin',(0.700000000000002,-2.9,-1.275)) ;
#144160=CARTESIAN_POINT('Origin',(-1.1,1.15,-1.275)) ;
#144161=CARTESIAN_POINT('Origin',(-1.1,1.15,-1.475)) ;
#144162=CARTESIAN_POINT('Origin',(-1.1,-2.39429110547967E-16,-1.275)) ;
#144163=CARTESIAN_POINT('',(-1.1,1.25,-1.375)) ;
#144164=CARTESIAN_POINT('Origin',(0.500000000000001,-2.9,-1.275)) ;
#144165=CARTESIAN_POINT('Origin',(0.500000000000001,-2.9,-1.475)) ;
#144166=CARTESIAN_POINT('Origin',(-1.1,1.25,-1.475)) ;
#144167=CARTESIAN_POINT('Origin',(-1.1,-2.9,-1.475)) ;
#144168=CARTESIAN_POINT('Origin',(-1.1,-2.9,-1.475)) ;
#144169=CARTESIAN_POINT('Origin',(-1.1,-2.9,-1.475)) ;
#144170=CARTESIAN_POINT('Origin',(-1.1,-2.9,-1.475)) ;
#144171=CARTESIAN_POINT('Origin',(4.55,4.55,-36.79)) ;
#144172=CARTESIAN_POINT('Origin',(4.55,4.55,-36.79)) ;
#144173=CARTESIAN_POINT('Origin',(4.55,4.55,-36.79)) ;
#144174=CARTESIAN_POINT('Origin',(4.55,4.55,-36.79)) ;
#144175=CARTESIAN_POINT('Origin',(4.55,4.35,-36.79)) ;
#144176=CARTESIAN_POINT('Origin',(4.75,4.55,-36.79)) ;
#144177=CARTESIAN_POINT('Origin',(4.75,4.55,-36.79)) ;
#144178=CARTESIAN_POINT('Origin',(4.35,4.35,-36.79)) ;
#144179=CARTESIAN_POINT('Origin',(4.35,4.15,-36.79)) ;
#144180=CARTESIAN_POINT('Origin',(4.75,4.55,-36.79)) ;
#144181=CARTESIAN_POINT('Origin',(4.75,4.55,-36.79)) ;
#144182=CARTESIAN_POINT('Origin',(-1.1,4.15,-36.79)) ;
#144183=CARTESIAN_POINT('Origin',(-1.1,4.15,-36.79)) ;
#144184=CARTESIAN_POINT('Origin',(4.75,4.35,-36.79)) ;
#144185=CARTESIAN_POINT('Origin',(4.75,4.35,-36.79)) ;
#144186=CARTESIAN_POINT('Origin',(-1.1,4.15,-36.79)) ;
#144187=CARTESIAN_POINT('Origin',(-1.1,4.15,-36.79)) ;
#144188=CARTESIAN_POINT('Origin',(4.95,4.35,-36.79)) ;
#144189=CARTESIAN_POINT('Origin',(4.95,4.15,-36.79)) ;
#144190=CARTESIAN_POINT('Origin',(-1.1,4.15,-36.79)) ;
#144191=CARTESIAN_POINT('Origin',(-1.1,-2.9,-36.79)) ;
#144192=CARTESIAN_POINT('Origin',(4.95,4.15,-36.79)) ;
#144193=CARTESIAN_POINT('Origin',(7.9,4.15,-36.79)) ;
#144194=CARTESIAN_POINT('Origin',(-1.1,-2.9,-36.79)) ;
#144195=CARTESIAN_POINT('Origin',(-1.1,-2.9,-36.79)) ;
#144196=CARTESIAN_POINT('Origin',(7.9,4.15,-36.79)) ;
#144197=CARTESIAN_POINT('Origin',(7.9,4.15,-36.79)) ;
#144198=CARTESIAN_POINT('Origin',(-1.1,-2.9,-36.79)) ;
#144199=CARTESIAN_POINT('Origin',(7.9,-2.9,-36.79)) ;
#144200=CARTESIAN_POINT('Origin',(7.9,4.15,-36.79)) ;
#144201=CARTESIAN_POINT('Origin',(7.9,-2.9,-36.79)) ;
#144202=CARTESIAN_POINT('Origin',(7.9,-2.9,-36.79)) ;
#144203=CARTESIAN_POINT('Origin',(4.55,4.55,2.5)) ;
#144204=CARTESIAN_POINT('Origin',(4.55,4.55,2.5)) ;
#144205=CARTESIAN_POINT('Origin',(4.55,4.55,2.5)) ;
#144206=CARTESIAN_POINT('Origin',(4.55,-2.9,2.5)) ;
#144207=CARTESIAN_POINT('Origin',(4.55,4.35,2.5)) ;
#144208=CARTESIAN_POINT('Origin',(7.9,4.55,2.5)) ;
#144209=CARTESIAN_POINT('Origin',(4.75,4.55,2.5)) ;
#144210=CARTESIAN_POINT('Origin',(4.35,4.35,2.5)) ;
#144211=CARTESIAN_POINT('Origin',(4.35,4.15,2.5)) ;
#144212=CARTESIAN_POINT('Origin',(4.75,4.55,2.5)) ;
#144213=CARTESIAN_POINT('Origin',(4.75,4.55,2.5)) ;
#144214=CARTESIAN_POINT('Origin',(7.9,4.15,2.5)) ;
#144215=CARTESIAN_POINT('Origin',(-1.1,4.15,2.5)) ;
#144216=CARTESIAN_POINT('Origin',(4.74999999999997,-2.89999999999999,2.5)) ;
#144217=CARTESIAN_POINT('Origin',(4.75,4.35,2.5)) ;
#144218=CARTESIAN_POINT('Origin',(-1.1,4.15,2.5)) ;
#144219=CARTESIAN_POINT('Origin',(-1.1,4.15,2.5)) ;
#144220=CARTESIAN_POINT('Origin',(4.95,4.35,2.5)) ;
#144221=CARTESIAN_POINT('Origin',(4.95,4.15,2.5)) ;
#144222=CARTESIAN_POINT('Origin',(-1.1,-2.9,2.5)) ;
#144223=CARTESIAN_POINT('Origin',(-1.1,-2.9,2.5)) ;
#144224=CARTESIAN_POINT('Origin',(7.9,4.15,2.5)) ;
#144225=CARTESIAN_POINT('Origin',(7.9,4.15,2.5)) ;
#144226=CARTESIAN_POINT('Origin',(-1.1,-2.9,2.5)) ;
#144227=CARTESIAN_POINT('Origin',(-1.1,-2.9,2.5)) ;
#144228=CARTESIAN_POINT('Origin',(7.9,4.15,2.5)) ;
#144229=CARTESIAN_POINT('Origin',(7.9,4.15,2.5)) ;
#144230=CARTESIAN_POINT('Origin',(7.9,-2.9,2.5)) ;
#144231=CARTESIAN_POINT('Origin',(7.9,-2.9,2.5)) ;
#144232=CARTESIAN_POINT('Origin',(7.9,-2.9,2.5)) ;
#144233=CARTESIAN_POINT('Origin',(7.9,-2.9,2.5)) ;
#144234=CARTESIAN_POINT('Origin',(7.9,-2.9,2.5)) ;
#144235=CARTESIAN_POINT('Origin',(1.5,1.9,0.6)) ;
#144236=CARTESIAN_POINT('Origin',(1.5,1.9,-1.55)) ;
#144237=CARTESIAN_POINT('Origin',(1.5,1.9,-0.6)) ;
#144238=CARTESIAN_POINT('Origin',(1.5,2.1,-0.6)) ;
#144239=CARTESIAN_POINT('Origin',(1.5,2.1,-0.4)) ;
#144240=CARTESIAN_POINT('Origin',(1.5,1.9,-1.55)) ;
#144241=CARTESIAN_POINT('Origin',(1.5,1.9,-1.55)) ;
#144242=CARTESIAN_POINT('Origin',(1.5,2.1,-0.4)) ;
#144243=CARTESIAN_POINT('Origin',(1.5,2.4,-0.4)) ;
#144244=CARTESIAN_POINT('Origin',(1.5,2.1,-1.55)) ;
#144245=CARTESIAN_POINT('Origin',(1.5,-2.15,-1.55)) ;
#144246=CARTESIAN_POINT('Origin',(1.5,2.4,-0.6)) ;
#144247=CARTESIAN_POINT('Origin',(1.5,2.6,-0.6)) ;
#144248=CARTESIAN_POINT('Origin',(1.5,-2.15,-1.55)) ;
#144249=CARTESIAN_POINT('Origin',(1.5,-2.15,-1.55)) ;
#144250=CARTESIAN_POINT('Origin',(1.5,2.6,0.6)) ;
#144251=CARTESIAN_POINT('Origin',(1.5,2.6,-0.70857864376269)) ;
#144252=CARTESIAN_POINT('Origin',(1.5,-2.15,0.6)) ;
#144253=CARTESIAN_POINT('Origin',(1.5,-2.15,-0.903119593409422)) ;
#144254=CARTESIAN_POINT('Origin',(1.5,2.6,-0.70857864376269)) ;
#144255=CARTESIAN_POINT('Origin',(1.5,2.6,-0.70857864376269)) ;
#144256=CARTESIAN_POINT('Origin',(1.5,-2.15,-0.903119593409422)) ;
#144257=CARTESIAN_POINT('Origin',(1.5,-2.15,-0.903119593409422)) ;
#144258=CARTESIAN_POINT('Origin',(1.5,1.69571067811865,0.195710678118654)) ;
#144259=CARTESIAN_POINT('Origin',(1.5,3.15,-1.25857864376269)) ;
#144260=CARTESIAN_POINT('Origin',(1.5,-3.65625,0.)) ;
#144261=CARTESIAN_POINT('Origin',(1.5,-2.15,0.903119593409423)) ;
#144262=CARTESIAN_POINT('Origin',(1.5,3.15,-1.25857864376269)) ;
#144263=CARTESIAN_POINT('Origin',(1.5,3.15,-1.25857864376269)) ;
#144264=CARTESIAN_POINT('Origin',(1.5,-2.15,0.903119593409422)) ;
#144265=CARTESIAN_POINT('Origin',(1.5,-2.15,0.903119593409422)) ;
#144266=CARTESIAN_POINT('Origin',(1.5,3.15,0.6)) ;
#144267=CARTESIAN_POINT('Origin',(1.5,-2.15,0.6)) ;
#144268=CARTESIAN_POINT('Origin',(1.5,-2.15,1.55)) ;
#144269=CARTESIAN_POINT('Origin',(1.5,-2.15,1.55)) ;
#144270=CARTESIAN_POINT('Origin',(1.5,-2.15,1.55)) ;
#144271=CARTESIAN_POINT('Origin',(1.5,2.29571067811866,0.404289321881344)) ;
#144272=CARTESIAN_POINT('Origin',(1.5,2.6,0.708578643762689)) ;
#144273=CARTESIAN_POINT('Origin',(1.5,2.1,1.55)) ;
#144274=CARTESIAN_POINT('Origin',(1.5,1.9,1.55)) ;
#144275=CARTESIAN_POINT('Origin',(1.5,2.6,0.70857864376269)) ;
#144276=CARTESIAN_POINT('Origin',(1.5,2.6,0.70857864376269)) ;
#144277=CARTESIAN_POINT('Origin',(1.5,1.9,1.55)) ;
#144278=CARTESIAN_POINT('Origin',(1.5,1.9,1.55)) ;
#144279=CARTESIAN_POINT('Origin',(1.5,2.6,0.599999999999998)) ;
#144280=CARTESIAN_POINT('Origin',(1.5,2.6,0.6)) ;
#144281=CARTESIAN_POINT('Origin',(1.5,1.9,0.6)) ;
#144282=CARTESIAN_POINT('Origin',(1.5,1.9,0.6)) ;
#144283=CARTESIAN_POINT('Origin',(1.5,2.4,0.6)) ;
#144284=CARTESIAN_POINT('Origin',(1.5,2.4,0.4)) ;
#144285=CARTESIAN_POINT('Origin',(1.5,2.1,0.6)) ;
#144286=CARTESIAN_POINT('Origin',(1.5,2.1,0.4)) ;
#144287=CARTESIAN_POINT('Origin',(1.5,2.1,0.4)) ;
#144288=CARTESIAN_POINT('Origin',(7.9,2.1,-0.6)) ;
#144289=CARTESIAN_POINT('Origin',(7.9,2.4,-0.6)) ;
#144290=CARTESIAN_POINT('Origin',(7.9,2.1,-0.6)) ;
#144291=CARTESIAN_POINT('Origin',(7.9,2.4,-0.6)) ;
#144292=CARTESIAN_POINT('Origin',(7.9,2.4,-0.6)) ;
#144293=CARTESIAN_POINT('Origin',(7.9,2.1,-0.6)) ;
#144294=CARTESIAN_POINT('Origin',(7.9,2.1,-0.6)) ;
#144295=CARTESIAN_POINT('Origin',(7.9,2.4,-0.6)) ;
#144296=CARTESIAN_POINT('Origin',(7.9,2.4,-0.70857864376269)) ;
#144297=CARTESIAN_POINT('Origin',(7.9,2.1,-0.6)) ;
#144298=CARTESIAN_POINT('Origin',(7.9,2.1,-1.55)) ;
#144299=CARTESIAN_POINT('Origin',(7.9,2.6,-0.70857864376269)) ;
#144300=CARTESIAN_POINT('Origin',(7.9,2.45857864376269,-0.85)) ;
#144301=CARTESIAN_POINT('Origin',(7.9,1.9,-1.55)) ;
#144302=CARTESIAN_POINT('Origin',(7.9,1.9,-1.75)) ;
#144303=CARTESIAN_POINT('Origin',(7.9,2.45857864376269,-0.85)) ;
#144304=CARTESIAN_POINT('Origin',(7.9,1.9,-1.75)) ;
#144305=CARTESIAN_POINT('Origin',(7.9,-2.15,-1.75)) ;
#144306=CARTESIAN_POINT('Origin',(7.9,-2.15,-1.55)) ;
#144307=CARTESIAN_POINT('Origin',(7.9,-2.35,-1.55)) ;
#144308=CARTESIAN_POINT('Origin',(7.9,3.35,-1.25857864376269)) ;
#144309=CARTESIAN_POINT('Origin',(7.9,3.35,1.25857864376269)) ;
#144310=CARTESIAN_POINT('Origin',(7.9,-2.35,-0.903119593409422)) ;
#144311=CARTESIAN_POINT('Origin',(7.9,-2.35,-0.903119593409422)) ;
#144312=CARTESIAN_POINT('Origin',(7.9,3.15,1.25857864376269)) ;
#144313=CARTESIAN_POINT('Origin',(7.9,3.00857864376269,1.4)) ;
#144314=CARTESIAN_POINT('Origin',(7.9,-2.15,-0.903119593409422)) ;
#144315=CARTESIAN_POINT('Origin',(7.9,-2.32153024911032,-0.800273234017602)) ;
#144316=CARTESIAN_POINT('Origin',(7.9,3.00857864376269,1.4)) ;
#144317=CARTESIAN_POINT('Origin',(7.9,2.45857864376269,0.849999999999999)) ;
#144318=CARTESIAN_POINT('Origin',(7.9,-3.65625,0.)) ;
#144319=CARTESIAN_POINT('Origin',(7.9,-2.32153024911032,0.800273234017602)) ;
#144320=CARTESIAN_POINT('Origin',(7.9,2.6,0.70857864376269)) ;
#144321=CARTESIAN_POINT('Origin',(7.9,2.4,0.70857864376269)) ;
#144322=CARTESIAN_POINT('Origin',(7.9,-2.15,0.903119593409422)) ;
#144323=CARTESIAN_POINT('Origin',(7.9,-2.35,0.903119593409422)) ;
#144324=CARTESIAN_POINT('Origin',(7.9,2.4,0.70857864376269)) ;
#144325=CARTESIAN_POINT('Origin',(7.9,2.4,0.600000000000001)) ;
#144326=CARTESIAN_POINT('Origin',(7.9,-2.35,1.55)) ;
#144327=CARTESIAN_POINT('Origin',(7.9,-2.35,1.55)) ;
#144328=CARTESIAN_POINT('Origin',(7.9,2.4,0.6)) ;
#144329=CARTESIAN_POINT('Origin',(7.9,2.4,0.6)) ;
#144330=CARTESIAN_POINT('Origin',(7.9,-2.15,1.55)) ;
#144331=CARTESIAN_POINT('Origin',(7.9,-2.15,1.75)) ;
#144332=CARTESIAN_POINT('Origin',(7.9,2.4,0.6)) ;
#144333=CARTESIAN_POINT('Origin',(7.9,2.1,0.6)) ;
#144334=CARTESIAN_POINT('Origin',(7.9,1.9,1.75)) ;
#144335=CARTESIAN_POINT('Origin',(7.9,1.9,1.75)) ;
#144336=CARTESIAN_POINT('Origin',(7.9,2.1,0.6)) ;
#144337=CARTESIAN_POINT('Origin',(7.9,2.1,0.6)) ;
#144338=CARTESIAN_POINT('Origin',(7.9,1.9,1.55)) ;
#144339=CARTESIAN_POINT('Origin',(7.9,2.1,1.55)) ;
#144340=CARTESIAN_POINT('Origin',(7.9,2.1,1.55)) ;
#144341=CARTESIAN_POINT('Origin',(-0.4,-0.600000000000001,0.4)) ;
#144342=CARTESIAN_POINT('',(-0.4,-0.600000000000001,0.3)) ;
#144343=CARTESIAN_POINT('',(-0.4,-0.600000000000001,-0.3)) ;
#144344=CARTESIAN_POINT('',(-0.4,-0.600000000000001,0.4)) ;
#144345=CARTESIAN_POINT('',(-0.4,-6.05857864376269,-0.3)) ;
#144346=CARTESIAN_POINT('',(-0.4,-0.600000000000001,-0.3)) ;
#144347=CARTESIAN_POINT('',(-0.4,-6.05857864376269,0.3)) ;
#144348=CARTESIAN_POINT('',(-0.4,-6.05857864376269,0.4)) ;
#144349=CARTESIAN_POINT('',(-0.4,-0.600000000000001,0.3)) ;
#144350=CARTESIAN_POINT('Origin',(-0.4,-6.1,0.4)) ;
#144351=CARTESIAN_POINT('',(-0.129289321881346,-6.37071067811866,-0.0585786437626899)) ;
#144352=CARTESIAN_POINT('',(-0.129289321881346,-6.37071067811866,0.0585786437626899)) ;
#144353=CARTESIAN_POINT('',(-0.129289321881346,-6.37071067811866,0.4)) ;
#144354=CARTESIAN_POINT('',(-0.370710678118655,-6.12928932188134,0.3)) ;
#144355=CARTESIAN_POINT('',(-0.423570226039552,-6.07642977396045,0.352859547920897)) ;
#144356=CARTESIAN_POINT('',(-0.370710678118655,-6.12928932188134,-0.3)) ;
#144357=CARTESIAN_POINT('',(-0.370710678118655,-6.12928932188134,0.4)) ;
#144358=CARTESIAN_POINT('',(-0.156903559372884,-6.34309644062712,-0.0861928812542289)) ;
#144359=CARTESIAN_POINT('Origin',(-0.1,-6.4,0.4)) ;
#144360=CARTESIAN_POINT('',(0.0585786437626908,-6.4,-0.0585786437626897)) ;
#144361=CARTESIAN_POINT('',(0.0585786437626908,-6.4,0.0585786437626898)) ;
#144362=CARTESIAN_POINT('',(0.0585786437626908,-6.4,0.4)) ;
#144363=CARTESIAN_POINT('',(-0.0585786437626908,-6.4,0.0585786437626898)) ;
#144364=CARTESIAN_POINT('',(-0.1,-6.4,0.0585786437626898)) ;
#144365=CARTESIAN_POINT('',(-0.0585786437626908,-6.4,-0.0585786437626897)) ;
#144366=CARTESIAN_POINT('',(-0.0585786437626908,-6.4,0.4)) ;
#144367=CARTESIAN_POINT('',(-0.1,-6.4,-0.0585786437626898)) ;
#144368=CARTESIAN_POINT('Origin',(0.1,-6.4,0.4)) ;
#144369=CARTESIAN_POINT('',(0.370710678118655,-6.12928932188134,-0.3)) ;
#144370=CARTESIAN_POINT('',(0.370710678118655,-6.12928932188134,0.299999999999999)) ;
#144371=CARTESIAN_POINT('',(0.370710678118655,-6.12928932188134,0.4)) ;
#144372=CARTESIAN_POINT('',(0.129289321881346,-6.37071067811866,0.0585786437626892)) ;
#144373=CARTESIAN_POINT('',(0.223570226039552,-6.27642977396045,0.152859547920897)) ;
#144374=CARTESIAN_POINT('',(0.129289321881346,-6.37071067811866,-0.05857864376269)) ;
#144375=CARTESIAN_POINT('',(0.129289321881346,-6.37071067811866,0.4)) ;
#144376=CARTESIAN_POINT('',(-0.0430964406271149,-6.54309644062712,0.113807118745771)) ;
#144377=CARTESIAN_POINT('Origin',(0.4,-6.1,0.4)) ;
#144378=CARTESIAN_POINT('',(0.4,-6.05857864376269,0.3)) ;
#144379=CARTESIAN_POINT('',(0.4,-6.05857864376269,-0.3)) ;
#144380=CARTESIAN_POINT('',(0.4,-6.05857864376269,0.4)) ;
#144381=CARTESIAN_POINT('',(0.4,-0.6,-0.3)) ;
#144382=CARTESIAN_POINT('',(0.4,-6.1,-0.3)) ;
#144383=CARTESIAN_POINT('',(0.4,-0.6,0.3)) ;
#144384=CARTESIAN_POINT('',(0.4,-0.6,0.4)) ;
#144385=CARTESIAN_POINT('',(0.4,-6.05857864376269,0.3)) ;
#144386=CARTESIAN_POINT('Origin',(0.6,-0.600000000000001,0.4)) ;
#144387=CARTESIAN_POINT('',(0.3,-6.05857864376269,0.4)) ;
#144388=CARTESIAN_POINT('',(0.3,-0.6,0.4)) ;
#144389=CARTESIAN_POINT('',(0.3,-0.6,0.4)) ;
#144390=CARTESIAN_POINT('Origin',(0.6,-0.6,0.4)) ;
#144391=CARTESIAN_POINT('',(-0.3,-0.600000000000001,0.4)) ;
#144392=CARTESIAN_POINT('Origin',(0.6,-0.600000000000001,0.4)) ;
#144393=CARTESIAN_POINT('',(-0.3,-6.05857864376269,0.4)) ;
#144394=CARTESIAN_POINT('',(-0.3,-0.600000000000001,0.4)) ;
#144395=CARTESIAN_POINT('',(0.4,-6.05857864376269,0.4)) ;
#144396=CARTESIAN_POINT('Origin',(0.6,-0.600000000000001,-0.4)) ;
#144397=CARTESIAN_POINT('',(-0.3,-6.05857864376269,-0.4)) ;
#144398=CARTESIAN_POINT('',(-0.3,-0.600000000000001,-0.4)) ;
#144399=CARTESIAN_POINT('',(-0.3,-0.600000000000001,-0.4)) ;
#144400=CARTESIAN_POINT('Origin',(0.6,-0.600000000000001,-0.4)) ;
#144401=CARTESIAN_POINT('',(0.3,-0.6,-0.4)) ;
#144402=CARTESIAN_POINT('Origin',(0.6,-0.6,-0.4)) ;
#144403=CARTESIAN_POINT('',(0.3,-6.05857864376269,-0.4)) ;
#144404=CARTESIAN_POINT('',(0.3,-0.600000000000001,-0.4)) ;
#144405=CARTESIAN_POINT('',(0.6,-6.05857864376269,-0.4)) ;
#144406=CARTESIAN_POINT('Origin',(0.6,-0.600000000000001,0.4)) ;
#144407=CARTESIAN_POINT('Origin',(0.6,-0.600000000000001,-0.3)) ;
#144408=CARTESIAN_POINT('Origin',(0.6,-0.600000000000001,0.3)) ;
#144409=CARTESIAN_POINT('Origin',(0.6,-0.6,0.4)) ;
#144410=CARTESIAN_POINT('Origin',(0.6,-0.6,-0.3)) ;
#144411=CARTESIAN_POINT('Origin',(0.6,-0.6,0.3)) ;
#144412=CARTESIAN_POINT('Origin',(7.,0.1,0.4)) ;
#144413=CARTESIAN_POINT('',(6.72928932188135,0.370710678118655,-0.3)) ;
#144414=CARTESIAN_POINT('',(6.72928932188135,0.370710678118655,0.3)) ;
#144415=CARTESIAN_POINT('',(6.72928932188135,0.370710678118655,0.4)) ;
#144416=CARTESIAN_POINT('',(6.97071067811866,0.129289321881346,0.0585786437626902)) ;
#144417=CARTESIAN_POINT('',(6.87642977396045,0.223570226039552,0.152859547920897)) ;
#144418=CARTESIAN_POINT('',(6.97071067811866,0.129289321881346,-0.0585786437626903)) ;
#144419=CARTESIAN_POINT('',(6.97071067811866,0.129289321881346,0.4)) ;
#144420=CARTESIAN_POINT('',(7.14309644062712,-0.043096440627115,0.11380711874577)) ;
#144421=CARTESIAN_POINT('Origin',(6.7,0.400000000000001,0.4)) ;
#144422=CARTESIAN_POINT('',(6.65857864376269,0.400000000000001,0.3)) ;
#144423=CARTESIAN_POINT('',(6.65857864376269,0.400000000000001,-0.3)) ;
#144424=CARTESIAN_POINT('',(6.65857864376269,0.400000000000001,0.4)) ;
#144425=CARTESIAN_POINT('',(6.7,0.400000000000001,-0.3)) ;
#144426=CARTESIAN_POINT('',(6.65857864376269,0.400000000000001,0.3)) ;
#144427=CARTESIAN_POINT('Origin',(0.6,-0.4,0.4)) ;
#144428=CARTESIAN_POINT('',(6.65857864376269,-0.400000000000001,-0.3)) ;
#144429=CARTESIAN_POINT('',(0.6,-0.4,-0.3)) ;
#144430=CARTESIAN_POINT('',(6.65857864376269,-0.400000000000001,0.3)) ;
#144431=CARTESIAN_POINT('',(6.65857864376269,-0.400000000000001,0.4)) ;
#144432=CARTESIAN_POINT('',(2.4,-0.4,0.3)) ;
#144433=CARTESIAN_POINT('Origin',(6.7,-0.400000000000001,0.4)) ;
#144434=CARTESIAN_POINT('',(6.97071067811866,-0.129289321881346,-0.0585786437626903)) ;
#144435=CARTESIAN_POINT('',(6.97071067811866,-0.129289321881346,0.0585786437626901)) ;
#144436=CARTESIAN_POINT('',(6.97071067811866,-0.129289321881346,0.4)) ;
#144437=CARTESIAN_POINT('',(6.72928932188135,-0.370710678118655,0.3)) ;
#144438=CARTESIAN_POINT('',(6.67642977396045,-0.423570226039552,0.352859547920897)) ;
#144439=CARTESIAN_POINT('',(6.72928932188135,-0.370710678118655,-0.3)) ;
#144440=CARTESIAN_POINT('',(6.72928932188135,-0.370710678118655,0.4)) ;
#144441=CARTESIAN_POINT('',(6.94309644062712,-0.156903559372885,-0.0861928812542298)) ;
#144442=CARTESIAN_POINT('Origin',(7.,-0.1,0.4)) ;
#144443=CARTESIAN_POINT('',(7.,-0.0585786437626909,0.0585786437626901)) ;
#144444=CARTESIAN_POINT('',(7.,-0.0585786437626909,-0.05857864376269)) ;
#144445=CARTESIAN_POINT('',(7.,-0.0585786437626909,0.4)) ;
#144446=CARTESIAN_POINT('',(7.,0.0585786437626909,-0.05857864376269)) ;
#144447=CARTESIAN_POINT('',(7.,-0.1,-0.05857864376269)) ;
#144448=CARTESIAN_POINT('',(7.,0.0585786437626909,0.05857864376269)) ;
#144449=CARTESIAN_POINT('',(7.,0.0585786437626909,0.4)) ;
#144450=CARTESIAN_POINT('',(7.,-0.1,0.0585786437626901)) ;
#144451=CARTESIAN_POINT('Origin',(0.6,-0.600000000000001,0.4)) ;
#144452=CARTESIAN_POINT('',(6.65857864376269,-0.300000000000001,0.4)) ;
#144453=CARTESIAN_POINT('',(6.65857864376269,0.300000000000001,0.4)) ;
#144454=CARTESIAN_POINT('',(6.65857864376269,-0.399999999999999,0.4)) ;
#144455=CARTESIAN_POINT('',(2.4,0.3,0.4)) ;
#144456=CARTESIAN_POINT('',(6.65857864376269,-0.300000000000001,0.4)) ;
#144457=CARTESIAN_POINT('Origin',(0.6,-0.600000000000001,-0.4)) ;
#144458=CARTESIAN_POINT('',(6.65857864376269,0.300000000000001,-0.4)) ;
#144459=CARTESIAN_POINT('',(0.6,0.299999999999999,-0.4)) ;
#144460=CARTESIAN_POINT('',(6.65857864376269,-0.300000000000001,-0.4)) ;
#144461=CARTESIAN_POINT('',(6.65857864376269,-0.6,-0.4)) ;
#144462=CARTESIAN_POINT('',(0.6,-0.3,-0.4)) ;
#144463=CARTESIAN_POINT('Origin',(0.4,-6.4,-0.0999999999999988)) ;
#144464=CARTESIAN_POINT('',(-0.0585786437626909,-6.37071067811866,-0.129289321881344)) ;
#144465=CARTESIAN_POINT('',(-0.3,-6.12928932188134,-0.370710678118655)) ;
#144466=CARTESIAN_POINT('',(0.113807118745769,-6.54309644062712,0.0430964406271166)) ;
#144467=CARTESIAN_POINT('',(0.3,-6.12928932188134,-0.370710678118655)) ;
#144468=CARTESIAN_POINT('',(0.4,-6.12928932188134,-0.370710678118654)) ;
#144469=CARTESIAN_POINT('',(0.058578643762691,-6.37071067811866,-0.129289321881344)) ;
#144470=CARTESIAN_POINT('',(0.152859547920897,-6.27642977396045,-0.22357022603955)) ;
#144471=CARTESIAN_POINT('',(0.4,-6.37071067811866,-0.129289321881344)) ;
#144472=CARTESIAN_POINT('Origin',(0.4,-6.1,0.4)) ;
#144473=CARTESIAN_POINT('',(0.0585786437626902,-6.37071067811866,0.129289321881344)) ;
#144474=CARTESIAN_POINT('',(0.299999999999999,-6.12928932188134,0.370710678118655)) ;
#144475=CARTESIAN_POINT('',(0.352859547920896,-6.07642977396045,0.423570226039552)) ;
#144476=CARTESIAN_POINT('',(-0.3,-6.12928932188134,0.370710678118655)) ;
#144477=CARTESIAN_POINT('',(0.4,-6.12928932188134,0.370710678118654)) ;
#144478=CARTESIAN_POINT('',(-0.058578643762691,-6.37071067811866,0.129289321881344)) ;
#144479=CARTESIAN_POINT('',(-0.086192881254231,-6.34309644062712,0.156903559372885)) ;
#144480=CARTESIAN_POINT('',(0.4,-6.37071067811866,0.129289321881344)) ;
#144481=CARTESIAN_POINT('Origin',(6.7,-0.399999999999999,-0.4)) ;
#144482=CARTESIAN_POINT('',(6.97071067811866,-0.0585786437626912,-0.129289321881345)) ;
#144483=CARTESIAN_POINT('',(6.72928932188135,-0.300000000000001,-0.370710678118655)) ;
#144484=CARTESIAN_POINT('',(6.67642977396045,-0.352859547920897,-0.423570226039551)) ;
#144485=CARTESIAN_POINT('',(6.72928932188135,0.300000000000001,-0.370710678118655)) ;
#144486=CARTESIAN_POINT('',(6.72928932188135,-0.399999999999999,-0.370710678118655)) ;
#144487=CARTESIAN_POINT('',(6.97071067811866,0.0585786437626912,-0.129289321881345)) ;
#144488=CARTESIAN_POINT('',(6.94309644062712,0.0861928812542309,-0.156903559372884)) ;
#144489=CARTESIAN_POINT('',(6.97071067811866,-0.4,-0.129289321881345)) ;
#144490=CARTESIAN_POINT('Origin',(7.,-0.399999999999999,0.0999999999999993)) ;
#144491=CARTESIAN_POINT('',(6.97071067811866,0.0585786437626911,0.129289321881345)) ;
#144492=CARTESIAN_POINT('',(6.72928932188135,0.300000000000001,0.370710678118655)) ;
#144493=CARTESIAN_POINT('',(7.14309644062712,-0.113807118745769,-0.043096440627116)) ;
#144494=CARTESIAN_POINT('',(6.72928932188135,-0.300000000000001,0.370710678118655)) ;
#144495=CARTESIAN_POINT('',(6.72928932188135,-0.399999999999999,0.370710678118655)) ;
#144496=CARTESIAN_POINT('',(6.97071067811866,-0.0585786437626911,0.129289321881345)) ;
#144497=CARTESIAN_POINT('',(6.87642977396045,-0.152859547920897,0.223570226039551)) ;
#144498=CARTESIAN_POINT('',(6.97071067811866,-0.399999999999999,0.129289321881345)) ;
#144499=CARTESIAN_POINT('Origin',(-0.11380711874577,-6.47238576250846,0.113807118745771)) ;
#144500=CARTESIAN_POINT('Origin',(0.3,-6.05857864376269,-0.3)) ;
#144501=CARTESIAN_POINT('Origin',(0.058578643762691,-6.3,-0.0585786437626897)) ;
#144502=CARTESIAN_POINT('Origin',(0.3,-6.05857864376269,0.4)) ;
#144503=CARTESIAN_POINT('Origin',(0.3,-6.05857864376269,-0.3)) ;
#144504=CARTESIAN_POINT('Origin',(0.3,-6.05857864376269,0.3)) ;
#144505=CARTESIAN_POINT('Origin',(0.0585786437626908,-6.3,-0.0585786437626897)) ;
#144506=CARTESIAN_POINT('Origin',(0.0585786437626908,-6.3,-0.0585786437626897)) ;
#144507=CARTESIAN_POINT('Origin',(0.0585786437626908,-6.3,-0.05857864376269)) ;
#144508=CARTESIAN_POINT('Origin',(0.152859547920897,-6.20571909584179,0.152859547920897)) ;
#144509=CARTESIAN_POINT('Origin',(0.3,-6.05857864376269,0.3)) ;
#144510=CARTESIAN_POINT('Origin',(0.0585786437626908,-6.3,0.0585786437626892)) ;
#144511=CARTESIAN_POINT('Origin',(0.0585786437626908,-6.3,0.4)) ;
#144512=CARTESIAN_POINT('Origin',(0.0585786437626908,-6.3,0.0585786437626898)) ;
#144513=CARTESIAN_POINT('Origin',(0.4,-6.3,-0.0585786437626897)) ;
#144514=CARTESIAN_POINT('Origin',(-0.0585786437626909,-6.3,-0.0585786437626897)) ;
#144515=CARTESIAN_POINT('Origin',(0.0585786437626908,-6.3,0.0585786437626898)) ;
#144516=CARTESIAN_POINT('Origin',(0.0585786437626902,-6.3,0.0585786437626897)) ;
#144517=CARTESIAN_POINT('Origin',(-0.0585786437626908,-6.3,-0.0585786437626897)) ;
#144518=CARTESIAN_POINT('Origin',(-0.0585786437626908,-6.3,-0.0585786437626899)) ;
#144519=CARTESIAN_POINT('Origin',(-0.0585786437626908,-6.3,-0.0585786437626897)) ;
#144520=CARTESIAN_POINT('Origin',(-0.1,-6.3,0.0585786437626898)) ;
#144521=CARTESIAN_POINT('Origin',(-0.0585786437626908,-6.3,0.0585786437626898)) ;
#144522=CARTESIAN_POINT('Origin',(-0.0585786437626908,-6.3,0.4)) ;
#144523=CARTESIAN_POINT('Origin',(-0.0585786437626908,-6.3,0.0585786437626899)) ;
#144524=CARTESIAN_POINT('Origin',(-0.0861928812542298,-6.27238576250846,
-0.0861928812542288)) ;
#144525=CARTESIAN_POINT('Origin',(-0.3,-6.05857864376269,-0.3)) ;
#144526=CARTESIAN_POINT('Origin',(-0.0585786437626909,-6.3,0.0585786437626898)) ;
#144527=CARTESIAN_POINT('Origin',(-0.058578643762691,-6.3,0.0585786437626897)) ;
#144528=CARTESIAN_POINT('Origin',(-0.3,-6.05857864376269,0.4)) ;
#144529=CARTESIAN_POINT('Origin',(-0.3,-6.05857864376269,-0.3)) ;
#144530=CARTESIAN_POINT('Origin',(-0.3,-6.05857864376269,0.3)) ;
#144531=CARTESIAN_POINT('Origin',(-0.352859547920897,-6.00571909584179,
0.352859547920897)) ;
#144532=CARTESIAN_POINT('Origin',(-0.3,-6.05857864376269,0.3)) ;
#144533=CARTESIAN_POINT('Origin',(7.07238576250846,-0.11380711874577,0.113807118745771)) ;
#144534=CARTESIAN_POINT('Origin',(6.65857864376269,0.300000000000001,-0.3)) ;
#144535=CARTESIAN_POINT('Origin',(6.9,0.0585786437626912,-0.05857864376269)) ;
#144536=CARTESIAN_POINT('Origin',(6.65857864376269,0.300000000000001,0.4)) ;
#144537=CARTESIAN_POINT('Origin',(6.65857864376269,0.300000000000001,-0.3)) ;
#144538=CARTESIAN_POINT('Origin',(6.65857864376269,0.300000000000001,0.3)) ;
#144539=CARTESIAN_POINT('Origin',(6.9,0.0585786437626909,-0.05857864376269)) ;
#144540=CARTESIAN_POINT('Origin',(6.9,0.0585786437626909,-0.05857864376269)) ;
#144541=CARTESIAN_POINT('Origin',(6.9,0.0585786437626909,-0.0585786437626903)) ;
#144542=CARTESIAN_POINT('Origin',(6.80571909584179,0.152859547920897,0.152859547920897)) ;
#144543=CARTESIAN_POINT('Origin',(6.65857864376269,0.300000000000001,0.3)) ;
#144544=CARTESIAN_POINT('Origin',(6.9,0.0585786437626909,0.0585786437626902)) ;
#144545=CARTESIAN_POINT('Origin',(6.9,0.0585786437626909,0.4)) ;
#144546=CARTESIAN_POINT('Origin',(6.9,0.0585786437626909,0.05857864376269)) ;
#144547=CARTESIAN_POINT('Origin',(6.9,-0.1,-0.05857864376269)) ;
#144548=CARTESIAN_POINT('Origin',(6.9,-0.0585786437626912,-0.05857864376269)) ;
#144549=CARTESIAN_POINT('Origin',(6.9,0.0585786437626909,0.05857864376269)) ;
#144550=CARTESIAN_POINT('Origin',(6.9,0.0585786437626911,0.05857864376269)) ;
#144551=CARTESIAN_POINT('Origin',(6.9,-0.058578643762691,-0.0585786437626901)) ;
#144552=CARTESIAN_POINT('Origin',(6.9,-0.0585786437626909,-0.0585786437626903)) ;
#144553=CARTESIAN_POINT('Origin',(6.9,-0.0585786437626909,-0.05857864376269)) ;
#144554=CARTESIAN_POINT('Origin',(6.9,-0.399999999999999,0.0585786437626901)) ;
#144555=CARTESIAN_POINT('Origin',(6.9,-0.0585786437626909,0.0585786437626901)) ;
#144556=CARTESIAN_POINT('Origin',(6.9,-0.0585786437626909,0.4)) ;
#144557=CARTESIAN_POINT('Origin',(6.9,-0.0585786437626909,0.0585786437626901)) ;
#144558=CARTESIAN_POINT('Origin',(6.87238576250846,-0.0861928812542305,
-0.0861928812542296)) ;
#144559=CARTESIAN_POINT('Origin',(6.65857864376269,-0.300000000000001,-0.3)) ;
#144560=CARTESIAN_POINT('Origin',(6.9,-0.058578643762691,0.0585786437626901)) ;
#144561=CARTESIAN_POINT('Origin',(6.9,-0.0585786437626911,0.05857864376269)) ;
#144562=CARTESIAN_POINT('Origin',(6.65857864376269,-0.300000000000001,0.4)) ;
#144563=CARTESIAN_POINT('Origin',(6.65857864376269,-0.300000000000001,-0.3)) ;
#144564=CARTESIAN_POINT('Origin',(6.65857864376269,-0.300000000000001,0.3)) ;
#144565=CARTESIAN_POINT('Origin',(6.60571909584179,-0.352859547920898,0.352859547920897)) ;
#144566=CARTESIAN_POINT('Origin',(6.65857864376269,-0.300000000000001,0.3)) ;
#144567=CARTESIAN_POINT('Origin',(0.6,-0.6,-0.3)) ;
#144568=CARTESIAN_POINT('Origin',(0.3,-0.6,-0.3)) ;
#144569=CARTESIAN_POINT('Origin',(0.3,-6.1,-0.3)) ;
#144570=CARTESIAN_POINT('Origin',(0.3,-6.05857864376269,-0.3)) ;
#144571=CARTESIAN_POINT('Origin',(0.3,-6.05857864376269,-0.3)) ;
#144572=CARTESIAN_POINT('Origin',(0.3,-6.05857864376269,-0.3)) ;
#144573=CARTESIAN_POINT('Origin',(0.4,-6.05857864376269,-0.3)) ;
#144574=CARTESIAN_POINT('Origin',(-0.3,-6.05857864376269,-0.3)) ;
#144575=CARTESIAN_POINT('Origin',(-0.3,-6.05857864376269,-0.3)) ;
#144576=CARTESIAN_POINT('Origin',(-0.3,-6.05857864376269,-0.3)) ;
#144577=CARTESIAN_POINT('Origin',(-0.3,-0.600000000000001,-0.3)) ;
#144578=CARTESIAN_POINT('Origin',(-0.3,-0.600000000000001,-0.3)) ;
#144579=CARTESIAN_POINT('Origin',(0.6,-0.600000000000001,-0.3)) ;
#144580=CARTESIAN_POINT('Origin',(0.6,-0.600000000000001,0.3)) ;
#144581=CARTESIAN_POINT('Origin',(-0.3,-0.600000000000001,0.3)) ;
#144582=CARTESIAN_POINT('Origin',(-0.3,-0.600000000000001,0.3)) ;
#144583=CARTESIAN_POINT('Origin',(-0.3,-6.05857864376269,0.3)) ;
#144584=CARTESIAN_POINT('Origin',(-0.3,-6.05857864376269,0.3)) ;
#144585=CARTESIAN_POINT('Origin',(-0.3,-6.05857864376269,0.3)) ;
#144586=CARTESIAN_POINT('Origin',(0.4,-6.05857864376269,0.3)) ;
#144587=CARTESIAN_POINT('Origin',(0.299999999999999,-6.05857864376269,0.3)) ;
#144588=CARTESIAN_POINT('Origin',(0.3,-6.05857864376269,0.3)) ;
#144589=CARTESIAN_POINT('Origin',(0.3,-6.05857864376269,0.3)) ;
#144590=CARTESIAN_POINT('Origin',(0.3,-0.600000000000001,0.3)) ;
#144591=CARTESIAN_POINT('Origin',(0.3,-0.6,0.3)) ;
#144592=CARTESIAN_POINT('Origin',(0.6,-0.6,0.3)) ;
#144593=CARTESIAN_POINT('Origin',(6.7,0.300000000000001,-0.3)) ;
#144594=CARTESIAN_POINT('Origin',(6.65857864376269,0.300000000000001,-0.3)) ;
#144595=CARTESIAN_POINT('Origin',(6.65857864376269,0.300000000000001,-0.3)) ;
#144596=CARTESIAN_POINT('Origin',(6.65857864376269,0.300000000000001,-0.3)) ;
#144597=CARTESIAN_POINT('Origin',(6.65857864376269,-0.399999999999999,-0.3)) ;
#144598=CARTESIAN_POINT('Origin',(6.65857864376269,-0.300000000000001,-0.3)) ;
#144599=CARTESIAN_POINT('Origin',(6.65857864376269,-0.300000000000001,-0.3)) ;
#144600=CARTESIAN_POINT('Origin',(6.65857864376269,-0.300000000000001,-0.3)) ;
#144601=CARTESIAN_POINT('Origin',(0.6,-0.3,-0.3)) ;
#144602=CARTESIAN_POINT('Origin',(0.6,0.299999999999999,0.3)) ;
#144603=CARTESIAN_POINT('Origin',(6.65857864376269,0.300000000000001,0.3)) ;
#144604=CARTESIAN_POINT('Origin',(6.65857864376269,0.300000000000001,0.3)) ;
#144605=CARTESIAN_POINT('Origin',(6.65857864376269,0.300000000000001,0.3)) ;
#144606=CARTESIAN_POINT('Origin',(6.65857864376269,-0.399999999999999,0.3)) ;
#144607=CARTESIAN_POINT('Origin',(6.65857864376269,-0.300000000000001,0.3)) ;
#144608=CARTESIAN_POINT('Origin',(0.6,-0.3,0.3)) ;
#144609=CARTESIAN_POINT('Origin',(6.65857864376269,-0.300000000000001,0.3)) ;
#144610=CARTESIAN_POINT('Origin',(6.65857864376269,-0.300000000000001,0.3)) ;
#144611=CARTESIAN_POINT('Origin',(-0.999999999999999,-1.59070596587277E-16,
-34.29)) ;
#144612=CARTESIAN_POINT('',(-0.999999999999999,-1.9,-33.69)) ;
#144613=CARTESIAN_POINT('',(-0.999999999999999,-1.9,-33.015)) ;
#144614=CARTESIAN_POINT('',(-0.999999999999999,-1.9,-32.915)) ;
#144615=CARTESIAN_POINT('',(-0.999999999999999,1.15,-33.015)) ;
#144616=CARTESIAN_POINT('',(-0.999999999999999,-2.89663358890162E-17,-33.015)) ;
#144617=CARTESIAN_POINT('',(-0.999999999999999,1.15,-35.565)) ;
#144618=CARTESIAN_POINT('',(-0.999999999999999,1.15,-34.29)) ;
#144619=CARTESIAN_POINT('',(-0.999999999999999,-1.9,-35.565)) ;
#144620=CARTESIAN_POINT('',(-0.999999999999999,-2.24122726936407E-16,-35.565)) ;
#144621=CARTESIAN_POINT('',(-0.999999999999999,-1.9,-34.89)) ;
#144622=CARTESIAN_POINT('',(-0.999999999999999,-1.9,-34.79)) ;
#144623=CARTESIAN_POINT('',(-0.999999999999999,0.4,-34.89)) ;
#144624=CARTESIAN_POINT('',(-0.999999999999999,0.5,-34.89)) ;
#144625=CARTESIAN_POINT('',(-0.999999999999999,0.6,-34.69)) ;
#144626=CARTESIAN_POINT('Origin',(-0.999999999999999,0.4,-34.69)) ;
#144627=CARTESIAN_POINT('',(-0.999999999999999,0.6,-33.89)) ;
#144628=CARTESIAN_POINT('',(-0.999999999999999,0.6,-33.79)) ;
#144629=CARTESIAN_POINT('',(-0.999999999999999,0.4,-33.69)) ;
#144630=CARTESIAN_POINT('Origin',(-0.999999999999999,0.4,-33.89)) ;
#144631=CARTESIAN_POINT('',(-0.999999999999999,-2.,-33.69)) ;
#144632=CARTESIAN_POINT('Origin',(-0.999999999999999,-1.59070596587277E-16,
-30.48)) ;
#144633=CARTESIAN_POINT('',(-0.999999999999999,-1.9,-29.88)) ;
#144634=CARTESIAN_POINT('',(-0.999999999999999,-1.9,-29.205)) ;
#144635=CARTESIAN_POINT('',(-0.999999999999999,-1.9,-29.105)) ;
#144636=CARTESIAN_POINT('',(-0.999999999999999,1.15,-29.205)) ;
#144637=CARTESIAN_POINT('',(-0.999999999999999,-2.89663358890162E-17,-29.205)) ;
#144638=CARTESIAN_POINT('',(-0.999999999999999,1.15,-31.755)) ;
#144639=CARTESIAN_POINT('',(-0.999999999999999,1.15,-30.48)) ;
#144640=CARTESIAN_POINT('',(-0.999999999999999,-1.9,-31.755)) ;
#144641=CARTESIAN_POINT('',(-0.999999999999999,-2.24122726936407E-16,-31.755)) ;
#144642=CARTESIAN_POINT('',(-0.999999999999999,-1.9,-31.08)) ;
#144643=CARTESIAN_POINT('',(-0.999999999999999,-1.9,-30.98)) ;
#144644=CARTESIAN_POINT('',(-0.999999999999999,0.4,-31.08)) ;
#144645=CARTESIAN_POINT('',(-0.999999999999999,0.5,-31.08)) ;
#144646=CARTESIAN_POINT('',(-0.999999999999999,0.6,-30.88)) ;
#144647=CARTESIAN_POINT('Origin',(-0.999999999999999,0.4,-30.88)) ;
#144648=CARTESIAN_POINT('',(-0.999999999999999,0.6,-30.08)) ;
#144649=CARTESIAN_POINT('',(-0.999999999999999,0.6,-29.98)) ;
#144650=CARTESIAN_POINT('',(-0.999999999999999,0.4,-29.88)) ;
#144651=CARTESIAN_POINT('Origin',(-0.999999999999999,0.4,-30.08)) ;
#144652=CARTESIAN_POINT('',(-0.999999999999999,-2.,-29.88)) ;
#144653=CARTESIAN_POINT('Origin',(-0.999999999999999,-1.59070596587277E-16,
-26.67)) ;
#144654=CARTESIAN_POINT('',(-0.999999999999999,-1.9,-26.07)) ;
#144655=CARTESIAN_POINT('',(-0.999999999999999,-1.9,-25.395)) ;
#144656=CARTESIAN_POINT('',(-0.999999999999999,-1.9,-25.295)) ;
#144657=CARTESIAN_POINT('',(-0.999999999999999,1.15,-25.395)) ;
#144658=CARTESIAN_POINT('',(-0.999999999999999,-2.89663358890162E-17,-25.395)) ;
#144659=CARTESIAN_POINT('',(-0.999999999999999,1.15,-27.945)) ;
#144660=CARTESIAN_POINT('',(-0.999999999999999,1.15,-26.67)) ;
#144661=CARTESIAN_POINT('',(-0.999999999999999,-1.9,-27.945)) ;
#144662=CARTESIAN_POINT('',(-0.999999999999999,-2.24122726936407E-16,-27.945)) ;
#144663=CARTESIAN_POINT('',(-0.999999999999999,-1.9,-27.27)) ;
#144664=CARTESIAN_POINT('',(-0.999999999999999,-1.9,-27.17)) ;
#144665=CARTESIAN_POINT('',(-0.999999999999999,0.4,-27.27)) ;
#144666=CARTESIAN_POINT('',(-0.999999999999999,0.5,-27.27)) ;
#144667=CARTESIAN_POINT('',(-0.999999999999999,0.6,-27.07)) ;
#144668=CARTESIAN_POINT('Origin',(-0.999999999999999,0.4,-27.07)) ;
#144669=CARTESIAN_POINT('',(-0.999999999999999,0.6,-26.27)) ;
#144670=CARTESIAN_POINT('',(-0.999999999999999,0.6,-26.17)) ;
#144671=CARTESIAN_POINT('',(-0.999999999999999,0.4,-26.07)) ;
#144672=CARTESIAN_POINT('Origin',(-0.999999999999999,0.4,-26.27)) ;
#144673=CARTESIAN_POINT('',(-0.999999999999999,-2.,-26.07)) ;
#144674=CARTESIAN_POINT('Origin',(-0.999999999999999,-1.59070596587277E-16,
-22.86)) ;
#144675=CARTESIAN_POINT('',(-0.999999999999999,-1.9,-22.26)) ;
#144676=CARTESIAN_POINT('',(-0.999999999999999,-1.9,-21.585)) ;
#144677=CARTESIAN_POINT('',(-0.999999999999999,-1.9,-21.485)) ;
#144678=CARTESIAN_POINT('',(-0.999999999999999,1.15,-21.585)) ;
#144679=CARTESIAN_POINT('',(-0.999999999999999,-2.89663358890162E-17,-21.585)) ;
#144680=CARTESIAN_POINT('',(-0.999999999999999,1.15,-24.135)) ;
#144681=CARTESIAN_POINT('',(-0.999999999999999,1.15,-22.86)) ;
#144682=CARTESIAN_POINT('',(-0.999999999999999,-1.9,-24.135)) ;
#144683=CARTESIAN_POINT('',(-0.999999999999999,-2.24122726936407E-16,-24.135)) ;
#144684=CARTESIAN_POINT('',(-0.999999999999999,-1.9,-23.46)) ;
#144685=CARTESIAN_POINT('',(-0.999999999999999,-1.9,-23.36)) ;
#144686=CARTESIAN_POINT('',(-0.999999999999999,0.4,-23.46)) ;
#144687=CARTESIAN_POINT('',(-0.999999999999999,0.5,-23.46)) ;
#144688=CARTESIAN_POINT('',(-0.999999999999999,0.6,-23.26)) ;
#144689=CARTESIAN_POINT('Origin',(-0.999999999999999,0.4,-23.26)) ;
#144690=CARTESIAN_POINT('',(-0.999999999999999,0.6,-22.46)) ;
#144691=CARTESIAN_POINT('',(-0.999999999999999,0.6,-22.36)) ;
#144692=CARTESIAN_POINT('',(-0.999999999999999,0.4,-22.26)) ;
#144693=CARTESIAN_POINT('Origin',(-0.999999999999999,0.4,-22.46)) ;
#144694=CARTESIAN_POINT('',(-0.999999999999999,-2.,-22.26)) ;
#144695=CARTESIAN_POINT('Origin',(-0.999999999999999,-1.59070596587277E-16,
-19.05)) ;
#144696=CARTESIAN_POINT('',(-0.999999999999999,-1.9,-18.45)) ;
#144697=CARTESIAN_POINT('',(-0.999999999999999,-1.9,-17.775)) ;
#144698=CARTESIAN_POINT('',(-0.999999999999999,-1.9,-17.675)) ;
#144699=CARTESIAN_POINT('',(-0.999999999999999,1.15,-17.775)) ;
#144700=CARTESIAN_POINT('',(-0.999999999999999,-2.89663358890162E-17,-17.775)) ;
#144701=CARTESIAN_POINT('',(-0.999999999999999,1.15,-20.325)) ;
#144702=CARTESIAN_POINT('',(-0.999999999999999,1.15,-19.05)) ;
#144703=CARTESIAN_POINT('',(-0.999999999999999,-1.9,-20.325)) ;
#144704=CARTESIAN_POINT('',(-0.999999999999999,-2.24122726936407E-16,-20.325)) ;
#144705=CARTESIAN_POINT('',(-0.999999999999999,-1.9,-19.65)) ;
#144706=CARTESIAN_POINT('',(-0.999999999999999,-1.9,-19.55)) ;
#144707=CARTESIAN_POINT('',(-0.999999999999999,0.4,-19.65)) ;
#144708=CARTESIAN_POINT('',(-0.999999999999999,0.5,-19.65)) ;
#144709=CARTESIAN_POINT('',(-0.999999999999999,0.6,-19.45)) ;
#144710=CARTESIAN_POINT('Origin',(-0.999999999999999,0.4,-19.45)) ;
#144711=CARTESIAN_POINT('',(-0.999999999999999,0.6,-18.65)) ;
#144712=CARTESIAN_POINT('',(-0.999999999999999,0.6,-18.55)) ;
#144713=CARTESIAN_POINT('',(-0.999999999999999,0.4,-18.45)) ;
#144714=CARTESIAN_POINT('Origin',(-0.999999999999999,0.4,-18.65)) ;
#144715=CARTESIAN_POINT('',(-0.999999999999999,-2.,-18.45)) ;
#144716=CARTESIAN_POINT('Origin',(-0.999999999999999,-1.59070596587277E-16,
-15.24)) ;
#144717=CARTESIAN_POINT('',(-0.999999999999999,-1.9,-14.64)) ;
#144718=CARTESIAN_POINT('',(-0.999999999999999,-1.9,-13.965)) ;
#144719=CARTESIAN_POINT('',(-0.999999999999999,-1.9,-13.865)) ;
#144720=CARTESIAN_POINT('',(-0.999999999999999,1.15,-13.965)) ;
#144721=CARTESIAN_POINT('',(-0.999999999999999,-2.8966335889016E-17,-13.965)) ;
#144722=CARTESIAN_POINT('',(-0.999999999999999,1.15,-16.515)) ;
#144723=CARTESIAN_POINT('',(-0.999999999999999,1.15,-15.24)) ;
#144724=CARTESIAN_POINT('',(-0.999999999999999,-1.9,-16.515)) ;
#144725=CARTESIAN_POINT('',(-0.999999999999999,-2.24122726936407E-16,-16.515)) ;
#144726=CARTESIAN_POINT('',(-0.999999999999999,-1.9,-15.84)) ;
#144727=CARTESIAN_POINT('',(-0.999999999999999,-1.9,-15.74)) ;
#144728=CARTESIAN_POINT('',(-0.999999999999999,0.4,-15.84)) ;
#144729=CARTESIAN_POINT('',(-0.999999999999999,0.5,-15.84)) ;
#144730=CARTESIAN_POINT('',(-0.999999999999999,0.6,-15.64)) ;
#144731=CARTESIAN_POINT('Origin',(-0.999999999999999,0.4,-15.64)) ;
#144732=CARTESIAN_POINT('',(-0.999999999999999,0.6,-14.84)) ;
#144733=CARTESIAN_POINT('',(-0.999999999999999,0.6,-14.74)) ;
#144734=CARTESIAN_POINT('',(-0.999999999999999,0.4,-14.64)) ;
#144735=CARTESIAN_POINT('Origin',(-0.999999999999999,0.4,-14.84)) ;
#144736=CARTESIAN_POINT('',(-0.999999999999999,-2.,-14.64)) ;
#144737=CARTESIAN_POINT('Origin',(-0.999999999999999,-1.59070596587277E-16,
-11.43)) ;
#144738=CARTESIAN_POINT('',(-0.999999999999999,-1.9,-10.83)) ;
#144739=CARTESIAN_POINT('',(-0.999999999999999,-1.9,-10.155)) ;
#144740=CARTESIAN_POINT('',(-0.999999999999999,-1.9,-10.055)) ;
#144741=CARTESIAN_POINT('',(-0.999999999999999,1.15,-10.155)) ;
#144742=CARTESIAN_POINT('',(-0.999999999999999,-2.8966335889016E-17,-10.155)) ;
#144743=CARTESIAN_POINT('',(-0.999999999999999,1.15,-12.705)) ;
#144744=CARTESIAN_POINT('',(-0.999999999999999,1.15,-11.43)) ;
#144745=CARTESIAN_POINT('',(-0.999999999999999,-1.9,-12.705)) ;
#144746=CARTESIAN_POINT('',(-0.999999999999999,-2.24122726936407E-16,-12.705)) ;
#144747=CARTESIAN_POINT('',(-0.999999999999999,-1.9,-12.03)) ;
#144748=CARTESIAN_POINT('',(-0.999999999999999,-1.9,-11.93)) ;
#144749=CARTESIAN_POINT('',(-0.999999999999999,0.4,-12.03)) ;
#144750=CARTESIAN_POINT('',(-0.999999999999999,0.5,-12.03)) ;
#144751=CARTESIAN_POINT('',(-0.999999999999999,0.6,-11.83)) ;
#144752=CARTESIAN_POINT('Origin',(-0.999999999999999,0.4,-11.83)) ;
#144753=CARTESIAN_POINT('',(-0.999999999999999,0.6,-11.03)) ;
#144754=CARTESIAN_POINT('',(-0.999999999999999,0.6,-10.93)) ;
#144755=CARTESIAN_POINT('',(-0.999999999999999,0.4,-10.83)) ;
#144756=CARTESIAN_POINT('Origin',(-0.999999999999999,0.4,-11.03)) ;
#144757=CARTESIAN_POINT('',(-0.999999999999999,-2.,-10.83)) ;
#144758=CARTESIAN_POINT('Origin',(-0.999999999999999,-1.59070596587277E-16,
-7.62)) ;
#144759=CARTESIAN_POINT('',(-0.999999999999999,-1.9,-7.02)) ;
#144760=CARTESIAN_POINT('',(-0.999999999999999,-1.9,-6.345)) ;
#144761=CARTESIAN_POINT('',(-0.999999999999999,-1.9,-6.245)) ;
#144762=CARTESIAN_POINT('',(-0.999999999999999,1.15,-6.345)) ;
#144763=CARTESIAN_POINT('',(-0.999999999999999,-2.89663358890161E-17,-6.345)) ;
#144764=CARTESIAN_POINT('',(-0.999999999999999,1.15,-8.895)) ;
#144765=CARTESIAN_POINT('',(-0.999999999999999,1.15,-7.62)) ;
#144766=CARTESIAN_POINT('',(-0.999999999999999,-1.9,-8.895)) ;
#144767=CARTESIAN_POINT('',(-0.999999999999999,-2.24122726936407E-16,-8.895)) ;
#144768=CARTESIAN_POINT('',(-0.999999999999999,-1.9,-8.22)) ;
#144769=CARTESIAN_POINT('',(-0.999999999999999,-1.9,-8.12)) ;
#144770=CARTESIAN_POINT('',(-0.999999999999999,0.4,-8.22)) ;
#144771=CARTESIAN_POINT('',(-0.999999999999999,0.5,-8.22)) ;
#144772=CARTESIAN_POINT('',(-0.999999999999999,0.6,-8.02)) ;
#144773=CARTESIAN_POINT('Origin',(-0.999999999999999,0.4,-8.02)) ;
#144774=CARTESIAN_POINT('',(-0.999999999999999,0.6,-7.22)) ;
#144775=CARTESIAN_POINT('',(-0.999999999999999,0.6,-7.12)) ;
#144776=CARTESIAN_POINT('',(-0.999999999999999,0.4,-7.02)) ;
#144777=CARTESIAN_POINT('Origin',(-0.999999999999999,0.4,-7.22)) ;
#144778=CARTESIAN_POINT('',(-0.999999999999999,-2.,-7.02)) ;
#144779=CARTESIAN_POINT('Origin',(-0.999999999999999,-1.59070596587277E-16,
-3.81)) ;
#144780=CARTESIAN_POINT('',(-0.999999999999999,-1.9,-3.21)) ;
#144781=CARTESIAN_POINT('',(-0.999999999999999,-1.9,-2.535)) ;
#144782=CARTESIAN_POINT('',(-0.999999999999999,-1.9,-2.435)) ;
#144783=CARTESIAN_POINT('',(-0.999999999999999,1.15,-2.535)) ;
#144784=CARTESIAN_POINT('',(-0.999999999999999,-2.89663358890161E-17,-2.535)) ;
#144785=CARTESIAN_POINT('',(-0.999999999999999,1.15,-5.085)) ;
#144786=CARTESIAN_POINT('',(-0.999999999999999,1.15,-3.81)) ;
#144787=CARTESIAN_POINT('',(-0.999999999999999,-1.9,-5.085)) ;
#144788=CARTESIAN_POINT('',(-0.999999999999999,-2.24122726936407E-16,-5.085)) ;
#144789=CARTESIAN_POINT('',(-0.999999999999999,-1.9,-4.41)) ;
#144790=CARTESIAN_POINT('',(-0.999999999999999,-1.9,-4.31)) ;
#144791=CARTESIAN_POINT('',(-0.999999999999999,0.4,-4.41)) ;
#144792=CARTESIAN_POINT('',(-0.999999999999999,0.5,-4.41)) ;
#144793=CARTESIAN_POINT('',(-0.999999999999999,0.6,-4.21)) ;
#144794=CARTESIAN_POINT('Origin',(-0.999999999999999,0.4,-4.21)) ;
#144795=CARTESIAN_POINT('',(-0.999999999999999,0.6,-3.41)) ;
#144796=CARTESIAN_POINT('',(-0.999999999999999,0.6,-3.31)) ;
#144797=CARTESIAN_POINT('',(-0.999999999999999,0.4,-3.21)) ;
#144798=CARTESIAN_POINT('Origin',(-0.999999999999999,0.4,-3.41)) ;
#144799=CARTESIAN_POINT('',(-0.999999999999999,-2.,-3.21)) ;
#144800=CARTESIAN_POINT('Origin',(0.600000000000001,-2.,-4.31)) ;
#144801=CARTESIAN_POINT('',(0.500000000000001,-2.,-4.41)) ;
#144802=CARTESIAN_POINT('',(-0.899999999999999,-2.,-4.41)) ;
#144803=CARTESIAN_POINT('',(0.600000000000001,-2.,-4.41)) ;
#144804=CARTESIAN_POINT('',(-0.899999999999999,-2.,-5.085)) ;
#144805=CARTESIAN_POINT('',(-0.899999999999999,-2.,-5.185)) ;
#144806=CARTESIAN_POINT('',(0.500000000000001,-2.,-5.085)) ;
#144807=CARTESIAN_POINT('',(0.600000000000001,-2.,-5.085)) ;
#144808=CARTESIAN_POINT('',(0.500000000000001,-2.,-4.31)) ;
#144809=CARTESIAN_POINT('Origin',(0.600000000000001,0.5,-4.31)) ;
#144810=CARTESIAN_POINT('',(-0.899999999999999,0.4,-4.31)) ;
#144811=CARTESIAN_POINT('',(-0.999999999999999,0.4,-4.31)) ;
#144812=CARTESIAN_POINT('',(-0.899999999999999,-1.9,-4.31)) ;
#144813=CARTESIAN_POINT('',(-0.899999999999999,-2.,-4.31)) ;
#144814=CARTESIAN_POINT('',(0.600000000000001,-1.9,-4.31)) ;
#144815=CARTESIAN_POINT('Origin',(0.600000000000001,0.5,-3.31)) ;
#144816=CARTESIAN_POINT('',(0.500000000000001,0.5,-3.41)) ;
#144817=CARTESIAN_POINT('',(-0.899999999999999,0.5,-3.41)) ;
#144818=CARTESIAN_POINT('',(-0.999999999999999,0.5,-3.41)) ;
#144819=CARTESIAN_POINT('',(-0.899999999999999,0.5,-4.21)) ;
#144820=CARTESIAN_POINT('',(-0.899999999999999,0.5,-4.31)) ;
#144821=CARTESIAN_POINT('',(0.500000000000001,0.5,-4.21)) ;
#144822=CARTESIAN_POINT('',(0.600000000000001,0.5,-4.21)) ;
#144823=CARTESIAN_POINT('',(0.500000000000001,0.5,-3.31)) ;
#144824=CARTESIAN_POINT('Origin',(0.600000000000001,-2.,-3.31)) ;
#144825=CARTESIAN_POINT('',(0.500000000000001,-1.9,-3.31)) ;
#144826=CARTESIAN_POINT('',(-0.899999999999999,-1.9,-3.31)) ;
#144827=CARTESIAN_POINT('',(0.600000000000001,-1.9,-3.31)) ;
#144828=CARTESIAN_POINT('',(-0.899999999999999,0.4,-3.31)) ;
#144829=CARTESIAN_POINT('',(-0.899999999999999,0.5,-3.31)) ;
#144830=CARTESIAN_POINT('',(0.500000000000001,0.4,-3.31)) ;
#144831=CARTESIAN_POINT('',(0.600000000000001,0.4,-3.31)) ;
#144832=CARTESIAN_POINT('',(0.500000000000001,-2.,-3.31)) ;
#144833=CARTESIAN_POINT('Origin',(0.600000000000001,-2.,-2.435)) ;
#144834=CARTESIAN_POINT('',(0.500000000000001,-2.,-2.535)) ;
#144835=CARTESIAN_POINT('',(-0.899999999999999,-2.,-2.535)) ;
#144836=CARTESIAN_POINT('',(-0.999999999999999,-2.,-2.535)) ;
#144837=CARTESIAN_POINT('',(-0.899999999999999,-2.,-3.21)) ;
#144838=CARTESIAN_POINT('',(-0.899999999999999,-2.,-3.31)) ;
#144839=CARTESIAN_POINT('',(0.500000000000001,-2.,-3.21)) ;
#144840=CARTESIAN_POINT('',(0.600000000000001,-2.,-3.21)) ;
#144841=CARTESIAN_POINT('',(0.500000000000001,-2.,-2.435)) ;
#144842=CARTESIAN_POINT('Origin',(0.600000000000001,-2.,-8.12)) ;
#144843=CARTESIAN_POINT('',(0.500000000000001,-2.,-8.22)) ;
#144844=CARTESIAN_POINT('',(-0.899999999999999,-2.,-8.22)) ;
#144845=CARTESIAN_POINT('',(0.600000000000001,-2.,-8.22)) ;
#144846=CARTESIAN_POINT('',(-0.899999999999999,-2.,-8.895)) ;
#144847=CARTESIAN_POINT('',(-0.899999999999999,-2.,-8.995)) ;
#144848=CARTESIAN_POINT('',(0.500000000000001,-2.,-8.895)) ;
#144849=CARTESIAN_POINT('',(0.600000000000001,-2.,-8.895)) ;
#144850=CARTESIAN_POINT('',(0.500000000000001,-2.,-8.12)) ;
#144851=CARTESIAN_POINT('Origin',(0.600000000000001,0.5,-8.12)) ;
#144852=CARTESIAN_POINT('',(-0.899999999999999,0.4,-8.12)) ;
#144853=CARTESIAN_POINT('',(-0.999999999999999,0.4,-8.12)) ;
#144854=CARTESIAN_POINT('',(-0.899999999999999,-1.9,-8.12)) ;
#144855=CARTESIAN_POINT('',(-0.899999999999999,-2.,-8.12)) ;
#144856=CARTESIAN_POINT('',(0.600000000000001,-1.9,-8.12)) ;
#144857=CARTESIAN_POINT('Origin',(0.600000000000001,0.5,-7.12)) ;
#144858=CARTESIAN_POINT('',(0.500000000000001,0.5,-7.22)) ;
#144859=CARTESIAN_POINT('',(-0.899999999999999,0.5,-7.22)) ;
#144860=CARTESIAN_POINT('',(-0.999999999999999,0.5,-7.22)) ;
#144861=CARTESIAN_POINT('',(-0.899999999999999,0.5,-8.02)) ;
#144862=CARTESIAN_POINT('',(-0.899999999999999,0.5,-8.12)) ;
#144863=CARTESIAN_POINT('',(0.500000000000001,0.5,-8.02)) ;
#144864=CARTESIAN_POINT('',(0.600000000000001,0.5,-8.02)) ;
#144865=CARTESIAN_POINT('',(0.500000000000001,0.5,-7.12)) ;
#144866=CARTESIAN_POINT('Origin',(0.600000000000001,-2.,-7.12)) ;
#144867=CARTESIAN_POINT('',(0.500000000000001,-1.9,-7.12)) ;
#144868=CARTESIAN_POINT('',(-0.899999999999999,-1.9,-7.12)) ;
#144869=CARTESIAN_POINT('',(0.600000000000001,-1.9,-7.12)) ;
#144870=CARTESIAN_POINT('',(-0.899999999999999,0.4,-7.12)) ;
#144871=CARTESIAN_POINT('',(-0.899999999999999,0.5,-7.12)) ;
#144872=CARTESIAN_POINT('',(0.500000000000001,0.4,-7.12)) ;
#144873=CARTESIAN_POINT('',(0.600000000000001,0.4,-7.12)) ;
#144874=CARTESIAN_POINT('',(0.500000000000001,-2.,-7.12)) ;
#144875=CARTESIAN_POINT('Origin',(0.600000000000001,-2.,-6.245)) ;
#144876=CARTESIAN_POINT('',(0.500000000000001,-2.,-6.345)) ;
#144877=CARTESIAN_POINT('',(-0.899999999999999,-2.,-6.345)) ;
#144878=CARTESIAN_POINT('',(-0.999999999999999,-2.,-6.345)) ;
#144879=CARTESIAN_POINT('',(-0.899999999999999,-2.,-7.02)) ;
#144880=CARTESIAN_POINT('',(-0.899999999999999,-2.,-7.12)) ;
#144881=CARTESIAN_POINT('',(0.500000000000001,-2.,-7.02)) ;
#144882=CARTESIAN_POINT('',(0.600000000000001,-2.,-7.02)) ;
#144883=CARTESIAN_POINT('',(0.500000000000001,-2.,-6.245)) ;
#144884=CARTESIAN_POINT('Origin',(0.600000000000001,-2.,-11.93)) ;
#144885=CARTESIAN_POINT('',(0.500000000000001,-2.,-12.03)) ;
#144886=CARTESIAN_POINT('',(-0.899999999999999,-2.,-12.03)) ;
#144887=CARTESIAN_POINT('',(0.600000000000001,-2.,-12.03)) ;
#144888=CARTESIAN_POINT('',(-0.899999999999999,-2.,-12.705)) ;
#144889=CARTESIAN_POINT('',(-0.899999999999999,-2.,-12.805)) ;
#144890=CARTESIAN_POINT('',(0.500000000000001,-2.,-12.705)) ;
#144891=CARTESIAN_POINT('',(0.600000000000001,-2.,-12.705)) ;
#144892=CARTESIAN_POINT('',(0.500000000000001,-2.,-11.93)) ;
#144893=CARTESIAN_POINT('Origin',(0.600000000000001,0.5,-11.93)) ;
#144894=CARTESIAN_POINT('',(-0.899999999999999,0.4,-11.93)) ;
#144895=CARTESIAN_POINT('',(-0.999999999999999,0.4,-11.93)) ;
#144896=CARTESIAN_POINT('',(-0.899999999999999,-1.9,-11.93)) ;
#144897=CARTESIAN_POINT('',(-0.899999999999999,-2.,-11.93)) ;
#144898=CARTESIAN_POINT('',(0.600000000000001,-1.9,-11.93)) ;
#144899=CARTESIAN_POINT('Origin',(0.600000000000001,0.5,-10.93)) ;
#144900=CARTESIAN_POINT('',(0.500000000000001,0.5,-11.03)) ;
#144901=CARTESIAN_POINT('',(-0.899999999999999,0.5,-11.03)) ;
#144902=CARTESIAN_POINT('',(-0.999999999999999,0.5,-11.03)) ;
#144903=CARTESIAN_POINT('',(-0.899999999999999,0.5,-11.83)) ;
#144904=CARTESIAN_POINT('',(-0.899999999999999,0.5,-11.93)) ;
#144905=CARTESIAN_POINT('',(0.500000000000001,0.5,-11.83)) ;
#144906=CARTESIAN_POINT('',(0.600000000000001,0.5,-11.83)) ;
#144907=CARTESIAN_POINT('',(0.500000000000001,0.5,-10.93)) ;
#144908=CARTESIAN_POINT('Origin',(0.600000000000001,-2.,-10.93)) ;
#144909=CARTESIAN_POINT('',(0.500000000000001,-1.9,-10.93)) ;
#144910=CARTESIAN_POINT('',(-0.899999999999999,-1.9,-10.93)) ;
#144911=CARTESIAN_POINT('',(0.600000000000001,-1.9,-10.93)) ;
#144912=CARTESIAN_POINT('',(-0.899999999999999,0.4,-10.93)) ;
#144913=CARTESIAN_POINT('',(-0.899999999999999,0.5,-10.93)) ;
#144914=CARTESIAN_POINT('',(0.500000000000001,0.4,-10.93)) ;
#144915=CARTESIAN_POINT('',(0.600000000000001,0.4,-10.93)) ;
#144916=CARTESIAN_POINT('',(0.500000000000001,-2.,-10.93)) ;
#144917=CARTESIAN_POINT('Origin',(0.600000000000001,-2.,-10.055)) ;
#144918=CARTESIAN_POINT('',(0.500000000000001,-2.,-10.155)) ;
#144919=CARTESIAN_POINT('',(-0.899999999999999,-2.,-10.155)) ;
#144920=CARTESIAN_POINT('',(-0.999999999999999,-2.,-10.155)) ;
#144921=CARTESIAN_POINT('',(-0.899999999999999,-2.,-10.83)) ;
#144922=CARTESIAN_POINT('',(-0.899999999999999,-2.,-10.93)) ;
#144923=CARTESIAN_POINT('',(0.500000000000001,-2.,-10.83)) ;
#144924=CARTESIAN_POINT('',(0.600000000000001,-2.,-10.83)) ;
#144925=CARTESIAN_POINT('',(0.500000000000001,-2.,-10.055)) ;
#144926=CARTESIAN_POINT('Origin',(0.600000000000001,-2.,-15.74)) ;
#144927=CARTESIAN_POINT('',(0.500000000000001,-2.,-15.84)) ;
#144928=CARTESIAN_POINT('',(-0.899999999999999,-2.,-15.84)) ;
#144929=CARTESIAN_POINT('',(0.600000000000001,-2.,-15.84)) ;
#144930=CARTESIAN_POINT('',(-0.899999999999999,-2.,-16.515)) ;
#144931=CARTESIAN_POINT('',(-0.899999999999999,-2.,-16.615)) ;
#144932=CARTESIAN_POINT('',(0.500000000000001,-2.,-16.515)) ;
#144933=CARTESIAN_POINT('',(0.600000000000001,-2.,-16.515)) ;
#144934=CARTESIAN_POINT('',(0.500000000000001,-2.,-15.74)) ;
#144935=CARTESIAN_POINT('Origin',(0.600000000000001,0.5,-15.74)) ;
#144936=CARTESIAN_POINT('',(-0.899999999999999,0.4,-15.74)) ;
#144937=CARTESIAN_POINT('',(-0.999999999999999,0.4,-15.74)) ;
#144938=CARTESIAN_POINT('',(-0.899999999999999,-1.9,-15.74)) ;
#144939=CARTESIAN_POINT('',(-0.899999999999999,-2.,-15.74)) ;
#144940=CARTESIAN_POINT('',(0.600000000000001,-1.9,-15.74)) ;
#144941=CARTESIAN_POINT('Origin',(0.600000000000001,0.5,-14.74)) ;
#144942=CARTESIAN_POINT('',(0.500000000000001,0.5,-14.84)) ;
#144943=CARTESIAN_POINT('',(-0.899999999999999,0.5,-14.84)) ;
#144944=CARTESIAN_POINT('',(-0.999999999999999,0.5,-14.84)) ;
#144945=CARTESIAN_POINT('',(-0.899999999999999,0.5,-15.64)) ;
#144946=CARTESIAN_POINT('',(-0.899999999999999,0.5,-15.74)) ;
#144947=CARTESIAN_POINT('',(0.500000000000001,0.5,-15.64)) ;
#144948=CARTESIAN_POINT('',(0.600000000000001,0.5,-15.64)) ;
#144949=CARTESIAN_POINT('',(0.500000000000001,0.5,-14.74)) ;
#144950=CARTESIAN_POINT('Origin',(0.600000000000001,-2.,-14.74)) ;
#144951=CARTESIAN_POINT('',(0.500000000000001,-1.9,-14.74)) ;
#144952=CARTESIAN_POINT('',(-0.899999999999999,-1.9,-14.74)) ;
#144953=CARTESIAN_POINT('',(0.600000000000001,-1.9,-14.74)) ;
#144954=CARTESIAN_POINT('',(-0.899999999999999,0.4,-14.74)) ;
#144955=CARTESIAN_POINT('',(-0.899999999999999,0.5,-14.74)) ;
#144956=CARTESIAN_POINT('',(0.500000000000001,0.4,-14.74)) ;
#144957=CARTESIAN_POINT('',(0.600000000000001,0.4,-14.74)) ;
#144958=CARTESIAN_POINT('',(0.500000000000001,-2.,-14.74)) ;
#144959=CARTESIAN_POINT('Origin',(0.600000000000001,-2.,-13.865)) ;
#144960=CARTESIAN_POINT('',(0.500000000000001,-2.,-13.965)) ;
#144961=CARTESIAN_POINT('',(-0.899999999999999,-2.,-13.965)) ;
#144962=CARTESIAN_POINT('',(-0.999999999999999,-2.,-13.965)) ;
#144963=CARTESIAN_POINT('',(-0.899999999999999,-2.,-14.64)) ;
#144964=CARTESIAN_POINT('',(-0.899999999999999,-2.,-14.74)) ;
#144965=CARTESIAN_POINT('',(0.500000000000001,-2.,-14.64)) ;
#144966=CARTESIAN_POINT('',(0.600000000000001,-2.,-14.64)) ;
#144967=CARTESIAN_POINT('',(0.500000000000001,-2.,-13.865)) ;
#144968=CARTESIAN_POINT('Origin',(0.600000000000001,-2.,-19.55)) ;
#144969=CARTESIAN_POINT('',(0.500000000000001,-2.,-19.65)) ;
#144970=CARTESIAN_POINT('',(-0.899999999999999,-2.,-19.65)) ;
#144971=CARTESIAN_POINT('',(0.600000000000001,-2.,-19.65)) ;
#144972=CARTESIAN_POINT('',(-0.899999999999999,-2.,-20.325)) ;
#144973=CARTESIAN_POINT('',(-0.899999999999999,-2.,-20.425)) ;
#144974=CARTESIAN_POINT('',(0.500000000000001,-2.,-20.325)) ;
#144975=CARTESIAN_POINT('',(0.600000000000001,-2.,-20.325)) ;
#144976=CARTESIAN_POINT('',(0.500000000000001,-2.,-19.55)) ;
#144977=CARTESIAN_POINT('Origin',(0.600000000000001,0.5,-19.55)) ;
#144978=CARTESIAN_POINT('',(-0.899999999999999,0.4,-19.55)) ;
#144979=CARTESIAN_POINT('',(-0.999999999999999,0.4,-19.55)) ;
#144980=CARTESIAN_POINT('',(-0.899999999999999,-1.9,-19.55)) ;
#144981=CARTESIAN_POINT('',(-0.899999999999999,-2.,-19.55)) ;
#144982=CARTESIAN_POINT('',(0.600000000000001,-1.9,-19.55)) ;
#144983=CARTESIAN_POINT('Origin',(0.600000000000001,0.5,-18.55)) ;
#144984=CARTESIAN_POINT('',(0.500000000000001,0.5,-18.65)) ;
#144985=CARTESIAN_POINT('',(-0.899999999999999,0.5,-18.65)) ;
#144986=CARTESIAN_POINT('',(-0.999999999999999,0.5,-18.65)) ;
#144987=CARTESIAN_POINT('',(-0.899999999999999,0.5,-19.45)) ;
#144988=CARTESIAN_POINT('',(-0.899999999999999,0.5,-19.55)) ;
#144989=CARTESIAN_POINT('',(0.500000000000001,0.5,-19.45)) ;
#144990=CARTESIAN_POINT('',(0.600000000000001,0.5,-19.45)) ;
#144991=CARTESIAN_POINT('',(0.500000000000001,0.5,-18.55)) ;
#144992=CARTESIAN_POINT('Origin',(0.600000000000001,-2.,-18.55)) ;
#144993=CARTESIAN_POINT('',(0.500000000000001,-1.9,-18.55)) ;
#144994=CARTESIAN_POINT('',(-0.899999999999999,-1.9,-18.55)) ;
#144995=CARTESIAN_POINT('',(0.600000000000001,-1.9,-18.55)) ;
#144996=CARTESIAN_POINT('',(-0.899999999999999,0.4,-18.55)) ;
#144997=CARTESIAN_POINT('',(-0.899999999999999,0.5,-18.55)) ;
#144998=CARTESIAN_POINT('',(0.500000000000001,0.4,-18.55)) ;
#144999=CARTESIAN_POINT('',(0.600000000000001,0.4,-18.55)) ;
#145000=CARTESIAN_POINT('',(0.500000000000001,-2.,-18.55)) ;
#145001=CARTESIAN_POINT('Origin',(0.600000000000001,-2.,-17.675)) ;
#145002=CARTESIAN_POINT('',(0.500000000000001,-2.,-17.775)) ;
#145003=CARTESIAN_POINT('',(-0.899999999999999,-2.,-17.775)) ;
#145004=CARTESIAN_POINT('',(-0.999999999999999,-2.,-17.775)) ;
#145005=CARTESIAN_POINT('',(-0.899999999999999,-2.,-18.45)) ;
#145006=CARTESIAN_POINT('',(-0.899999999999999,-2.,-18.55)) ;
#145007=CARTESIAN_POINT('',(0.500000000000001,-2.,-18.45)) ;
#145008=CARTESIAN_POINT('',(0.600000000000001,-2.,-18.45)) ;
#145009=CARTESIAN_POINT('',(0.500000000000001,-2.,-17.675)) ;
#145010=CARTESIAN_POINT('Origin',(0.600000000000001,-2.,-23.36)) ;
#145011=CARTESIAN_POINT('',(0.500000000000001,-2.,-23.46)) ;
#145012=CARTESIAN_POINT('',(-0.899999999999999,-2.,-23.46)) ;
#145013=CARTESIAN_POINT('',(0.600000000000001,-2.,-23.46)) ;
#145014=CARTESIAN_POINT('',(-0.899999999999999,-2.,-24.135)) ;
#145015=CARTESIAN_POINT('',(-0.899999999999999,-2.,-24.235)) ;
#145016=CARTESIAN_POINT('',(0.500000000000001,-2.,-24.135)) ;
#145017=CARTESIAN_POINT('',(0.600000000000001,-2.,-24.135)) ;
#145018=CARTESIAN_POINT('',(0.500000000000001,-2.,-23.36)) ;
#145019=CARTESIAN_POINT('Origin',(0.600000000000001,0.5,-23.36)) ;
#145020=CARTESIAN_POINT('',(-0.899999999999999,0.4,-23.36)) ;
#145021=CARTESIAN_POINT('',(-0.999999999999999,0.4,-23.36)) ;
#145022=CARTESIAN_POINT('',(-0.899999999999999,-1.9,-23.36)) ;
#145023=CARTESIAN_POINT('',(-0.899999999999999,-2.,-23.36)) ;
#145024=CARTESIAN_POINT('',(0.600000000000001,-1.9,-23.36)) ;
#145025=CARTESIAN_POINT('Origin',(0.600000000000001,0.5,-22.36)) ;
#145026=CARTESIAN_POINT('',(0.500000000000001,0.5,-22.46)) ;
#145027=CARTESIAN_POINT('',(-0.899999999999999,0.5,-22.46)) ;
#145028=CARTESIAN_POINT('',(-0.999999999999999,0.5,-22.46)) ;
#145029=CARTESIAN_POINT('',(-0.899999999999999,0.5,-23.26)) ;
#145030=CARTESIAN_POINT('',(-0.899999999999999,0.5,-23.36)) ;
#145031=CARTESIAN_POINT('',(0.500000000000001,0.5,-23.26)) ;
#145032=CARTESIAN_POINT('',(0.600000000000001,0.5,-23.26)) ;
#145033=CARTESIAN_POINT('',(0.500000000000001,0.5,-22.36)) ;
#145034=CARTESIAN_POINT('Origin',(0.600000000000001,-2.,-22.36)) ;
#145035=CARTESIAN_POINT('',(0.500000000000001,-1.9,-22.36)) ;
#145036=CARTESIAN_POINT('',(-0.899999999999999,-1.9,-22.36)) ;
#145037=CARTESIAN_POINT('',(0.600000000000001,-1.9,-22.36)) ;
#145038=CARTESIAN_POINT('',(-0.899999999999999,0.4,-22.36)) ;
#145039=CARTESIAN_POINT('',(-0.899999999999999,0.5,-22.36)) ;
#145040=CARTESIAN_POINT('',(0.500000000000001,0.4,-22.36)) ;
#145041=CARTESIAN_POINT('',(0.600000000000001,0.4,-22.36)) ;
#145042=CARTESIAN_POINT('',(0.500000000000001,-2.,-22.36)) ;
#145043=CARTESIAN_POINT('Origin',(0.600000000000001,-2.,-21.485)) ;
#145044=CARTESIAN_POINT('',(0.500000000000001,-2.,-21.585)) ;
#145045=CARTESIAN_POINT('',(-0.899999999999999,-2.,-21.585)) ;
#145046=CARTESIAN_POINT('',(-0.999999999999999,-2.,-21.585)) ;
#145047=CARTESIAN_POINT('',(-0.899999999999999,-2.,-22.26)) ;
#145048=CARTESIAN_POINT('',(-0.899999999999999,-2.,-22.36)) ;
#145049=CARTESIAN_POINT('',(0.500000000000001,-2.,-22.26)) ;
#145050=CARTESIAN_POINT('',(0.600000000000001,-2.,-22.26)) ;
#145051=CARTESIAN_POINT('',(0.500000000000001,-2.,-21.485)) ;
#145052=CARTESIAN_POINT('Origin',(0.600000000000001,-2.,-27.17)) ;
#145053=CARTESIAN_POINT('',(0.500000000000001,-2.,-27.27)) ;
#145054=CARTESIAN_POINT('',(-0.899999999999999,-2.,-27.27)) ;
#145055=CARTESIAN_POINT('',(0.600000000000001,-2.,-27.27)) ;
#145056=CARTESIAN_POINT('',(-0.899999999999999,-2.,-27.945)) ;
#145057=CARTESIAN_POINT('',(-0.899999999999999,-2.,-28.045)) ;
#145058=CARTESIAN_POINT('',(0.500000000000001,-2.,-27.945)) ;
#145059=CARTESIAN_POINT('',(0.600000000000001,-2.,-27.945)) ;
#145060=CARTESIAN_POINT('',(0.500000000000001,-2.,-27.17)) ;
#145061=CARTESIAN_POINT('Origin',(0.600000000000001,0.5,-27.17)) ;
#145062=CARTESIAN_POINT('',(-0.899999999999999,0.4,-27.17)) ;
#145063=CARTESIAN_POINT('',(-0.999999999999999,0.4,-27.17)) ;
#145064=CARTESIAN_POINT('',(-0.899999999999999,-1.9,-27.17)) ;
#145065=CARTESIAN_POINT('',(-0.899999999999999,-2.,-27.17)) ;
#145066=CARTESIAN_POINT('',(0.600000000000001,-1.9,-27.17)) ;
#145067=CARTESIAN_POINT('Origin',(0.600000000000001,0.5,-26.17)) ;
#145068=CARTESIAN_POINT('',(0.500000000000001,0.5,-26.27)) ;
#145069=CARTESIAN_POINT('',(-0.899999999999999,0.5,-26.27)) ;
#145070=CARTESIAN_POINT('',(-0.999999999999999,0.5,-26.27)) ;
#145071=CARTESIAN_POINT('',(-0.899999999999999,0.5,-27.07)) ;
#145072=CARTESIAN_POINT('',(-0.899999999999999,0.5,-27.17)) ;
#145073=CARTESIAN_POINT('',(0.500000000000001,0.5,-27.07)) ;
#145074=CARTESIAN_POINT('',(0.600000000000001,0.5,-27.07)) ;
#145075=CARTESIAN_POINT('',(0.500000000000001,0.5,-26.17)) ;
#145076=CARTESIAN_POINT('Origin',(0.600000000000001,-2.,-26.17)) ;
#145077=CARTESIAN_POINT('',(0.500000000000001,-1.9,-26.17)) ;
#145078=CARTESIAN_POINT('',(-0.899999999999999,-1.9,-26.17)) ;
#145079=CARTESIAN_POINT('',(0.600000000000001,-1.9,-26.17)) ;
#145080=CARTESIAN_POINT('',(-0.899999999999999,0.4,-26.17)) ;
#145081=CARTESIAN_POINT('',(-0.899999999999999,0.5,-26.17)) ;
#145082=CARTESIAN_POINT('',(0.500000000000001,0.4,-26.17)) ;
#145083=CARTESIAN_POINT('',(0.600000000000001,0.4,-26.17)) ;
#145084=CARTESIAN_POINT('',(0.500000000000001,-2.,-26.17)) ;
#145085=CARTESIAN_POINT('Origin',(0.600000000000001,-2.,-25.295)) ;
#145086=CARTESIAN_POINT('',(0.500000000000001,-2.,-25.395)) ;
#145087=CARTESIAN_POINT('',(-0.899999999999999,-2.,-25.395)) ;
#145088=CARTESIAN_POINT('',(-0.999999999999999,-2.,-25.395)) ;
#145089=CARTESIAN_POINT('',(-0.899999999999999,-2.,-26.07)) ;
#145090=CARTESIAN_POINT('',(-0.899999999999999,-2.,-26.17)) ;
#145091=CARTESIAN_POINT('',(0.500000000000001,-2.,-26.07)) ;
#145092=CARTESIAN_POINT('',(0.600000000000001,-2.,-26.07)) ;
#145093=CARTESIAN_POINT('',(0.500000000000001,-2.,-25.295)) ;
#145094=CARTESIAN_POINT('Origin',(0.600000000000001,-2.,-30.98)) ;
#145095=CARTESIAN_POINT('',(0.500000000000001,-2.,-31.08)) ;
#145096=CARTESIAN_POINT('',(-0.899999999999999,-2.,-31.08)) ;
#145097=CARTESIAN_POINT('',(0.600000000000001,-2.,-31.08)) ;
#145098=CARTESIAN_POINT('',(-0.899999999999999,-2.,-31.755)) ;
#145099=CARTESIAN_POINT('',(-0.899999999999999,-2.,-31.855)) ;
#145100=CARTESIAN_POINT('',(0.500000000000001,-2.,-31.755)) ;
#145101=CARTESIAN_POINT('',(0.600000000000001,-2.,-31.755)) ;
#145102=CARTESIAN_POINT('',(0.500000000000001,-2.,-30.98)) ;
#145103=CARTESIAN_POINT('Origin',(0.600000000000001,0.5,-30.98)) ;
#145104=CARTESIAN_POINT('',(-0.899999999999999,0.4,-30.98)) ;
#145105=CARTESIAN_POINT('',(-0.999999999999999,0.4,-30.98)) ;
#145106=CARTESIAN_POINT('',(-0.899999999999999,-1.9,-30.98)) ;
#145107=CARTESIAN_POINT('',(-0.899999999999999,-2.,-30.98)) ;
#145108=CARTESIAN_POINT('',(0.600000000000001,-1.9,-30.98)) ;
#145109=CARTESIAN_POINT('Origin',(0.600000000000001,0.5,-29.98)) ;
#145110=CARTESIAN_POINT('',(0.500000000000001,0.5,-30.08)) ;
#145111=CARTESIAN_POINT('',(-0.899999999999999,0.5,-30.08)) ;
#145112=CARTESIAN_POINT('',(-0.999999999999999,0.5,-30.08)) ;
#145113=CARTESIAN_POINT('',(-0.899999999999999,0.5,-30.88)) ;
#145114=CARTESIAN_POINT('',(-0.899999999999999,0.5,-30.98)) ;
#145115=CARTESIAN_POINT('',(0.500000000000001,0.5,-30.88)) ;
#145116=CARTESIAN_POINT('',(0.600000000000001,0.5,-30.88)) ;
#145117=CARTESIAN_POINT('',(0.500000000000001,0.5,-29.98)) ;
#145118=CARTESIAN_POINT('Origin',(0.600000000000001,-2.,-29.98)) ;
#145119=CARTESIAN_POINT('',(0.500000000000001,-1.9,-29.98)) ;
#145120=CARTESIAN_POINT('',(-0.899999999999999,-1.9,-29.98)) ;
#145121=CARTESIAN_POINT('',(0.600000000000001,-1.9,-29.98)) ;
#145122=CARTESIAN_POINT('',(-0.899999999999999,0.4,-29.98)) ;
#145123=CARTESIAN_POINT('',(-0.899999999999999,0.5,-29.98)) ;
#145124=CARTESIAN_POINT('',(0.500000000000001,0.4,-29.98)) ;
#145125=CARTESIAN_POINT('',(0.600000000000001,0.4,-29.98)) ;
#145126=CARTESIAN_POINT('',(0.500000000000001,-2.,-29.98)) ;
#145127=CARTESIAN_POINT('Origin',(0.600000000000001,-2.,-29.105)) ;
#145128=CARTESIAN_POINT('',(0.500000000000001,-2.,-29.205)) ;
#145129=CARTESIAN_POINT('',(-0.899999999999999,-2.,-29.205)) ;
#145130=CARTESIAN_POINT('',(-0.999999999999999,-2.,-29.205)) ;
#145131=CARTESIAN_POINT('',(-0.899999999999999,-2.,-29.88)) ;
#145132=CARTESIAN_POINT('',(-0.899999999999999,-2.,-29.98)) ;
#145133=CARTESIAN_POINT('',(0.500000000000001,-2.,-29.88)) ;
#145134=CARTESIAN_POINT('',(0.600000000000001,-2.,-29.88)) ;
#145135=CARTESIAN_POINT('',(0.500000000000001,-2.,-29.105)) ;
#145136=CARTESIAN_POINT('Origin',(0.600000000000001,-2.,-34.79)) ;
#145137=CARTESIAN_POINT('',(0.500000000000001,-2.,-34.89)) ;
#145138=CARTESIAN_POINT('',(-0.899999999999999,-2.,-34.89)) ;
#145139=CARTESIAN_POINT('',(0.600000000000001,-2.,-34.89)) ;
#145140=CARTESIAN_POINT('',(-0.899999999999999,-2.,-35.565)) ;
#145141=CARTESIAN_POINT('',(-0.899999999999999,-2.,-35.665)) ;
#145142=CARTESIAN_POINT('',(0.500000000000001,-2.,-35.565)) ;
#145143=CARTESIAN_POINT('',(0.600000000000001,-2.,-35.565)) ;
#145144=CARTESIAN_POINT('',(0.500000000000001,-2.,-34.79)) ;
#145145=CARTESIAN_POINT('Origin',(0.600000000000001,0.5,-34.79)) ;
#145146=CARTESIAN_POINT('',(-0.899999999999999,0.4,-34.79)) ;
#145147=CARTESIAN_POINT('',(-0.999999999999999,0.4,-34.79)) ;
#145148=CARTESIAN_POINT('',(-0.899999999999999,-1.9,-34.79)) ;
#145149=CARTESIAN_POINT('',(-0.899999999999999,-2.,-34.79)) ;
#145150=CARTESIAN_POINT('',(0.600000000000001,-1.9,-34.79)) ;
#145151=CARTESIAN_POINT('Origin',(0.600000000000001,0.5,-33.79)) ;
#145152=CARTESIAN_POINT('',(0.500000000000001,0.5,-33.89)) ;
#145153=CARTESIAN_POINT('',(-0.899999999999999,0.5,-33.89)) ;
#145154=CARTESIAN_POINT('',(-0.999999999999999,0.5,-33.89)) ;
#145155=CARTESIAN_POINT('',(-0.899999999999999,0.5,-34.69)) ;
#145156=CARTESIAN_POINT('',(-0.899999999999999,0.5,-34.79)) ;
#145157=CARTESIAN_POINT('',(0.500000000000001,0.5,-34.69)) ;
#145158=CARTESIAN_POINT('',(0.600000000000001,0.5,-34.69)) ;
#145159=CARTESIAN_POINT('',(0.500000000000001,0.5,-33.79)) ;
#145160=CARTESIAN_POINT('Origin',(0.600000000000001,-2.,-33.79)) ;
#145161=CARTESIAN_POINT('',(0.500000000000001,-1.9,-33.79)) ;
#145162=CARTESIAN_POINT('',(-0.899999999999999,-1.9,-33.79)) ;
#145163=CARTESIAN_POINT('',(0.600000000000001,-1.9,-33.79)) ;
#145164=CARTESIAN_POINT('',(-0.899999999999999,0.4,-33.79)) ;
#145165=CARTESIAN_POINT('',(-0.899999999999999,0.5,-33.79)) ;
#145166=CARTESIAN_POINT('',(0.500000000000001,0.4,-33.79)) ;
#145167=CARTESIAN_POINT('',(0.600000000000001,0.4,-33.79)) ;
#145168=CARTESIAN_POINT('',(0.500000000000001,-2.,-33.79)) ;
#145169=CARTESIAN_POINT('Origin',(0.600000000000001,-2.,-32.915)) ;
#145170=CARTESIAN_POINT('',(0.500000000000001,-2.,-33.015)) ;
#145171=CARTESIAN_POINT('',(-0.899999999999999,-2.,-33.015)) ;
#145172=CARTESIAN_POINT('',(-0.999999999999999,-2.,-33.015)) ;
#145173=CARTESIAN_POINT('',(-0.899999999999999,-2.,-33.69)) ;
#145174=CARTESIAN_POINT('',(-0.899999999999999,-2.,-33.79)) ;
#145175=CARTESIAN_POINT('',(0.500000000000001,-2.,-33.69)) ;
#145176=CARTESIAN_POINT('',(0.600000000000001,-2.,-33.69)) ;
#145177=CARTESIAN_POINT('',(0.500000000000001,-2.,-32.915)) ;
#145178=CARTESIAN_POINT('Origin',(1.4,2.1,-33.69)) ;
#145179=CARTESIAN_POINT('',(1.5,2.,-33.69)) ;
#145180=CARTESIAN_POINT('',(7.9,2.,-33.69)) ;
#145181=CARTESIAN_POINT('',(1.4,2.,-33.69)) ;
#145182=CARTESIAN_POINT('',(1.5,2.1,-33.79)) ;
#145183=CARTESIAN_POINT('Origin',(1.5,2.1,-33.69)) ;
#145184=CARTESIAN_POINT('',(7.9,2.1,-33.79)) ;
#145185=CARTESIAN_POINT('',(1.4,2.1,-33.79)) ;
#145186=CARTESIAN_POINT('Origin',(7.9,2.1,-33.69)) ;
#145187=CARTESIAN_POINT('Origin',(1.4,2.4,-33.79)) ;
#145188=CARTESIAN_POINT('',(1.5,2.4,-33.79)) ;
#145189=CARTESIAN_POINT('',(1.5,2.4,-33.79)) ;
#145190=CARTESIAN_POINT('',(7.9,2.4,-33.79)) ;
#145191=CARTESIAN_POINT('',(1.4,2.4,-33.79)) ;
#145192=CARTESIAN_POINT('',(7.9,2.1,-33.79)) ;
#145193=CARTESIAN_POINT('Origin',(1.4,2.4,-33.69)) ;
#145194=CARTESIAN_POINT('',(1.5,2.5,-33.69)) ;
#145195=CARTESIAN_POINT('Origin',(1.5,2.4,-33.69)) ;
#145196=CARTESIAN_POINT('',(7.9,2.5,-33.69)) ;
#145197=CARTESIAN_POINT('',(1.4,2.5,-33.69)) ;
#145198=CARTESIAN_POINT('Origin',(7.9,2.4,-33.69)) ;
#145199=CARTESIAN_POINT('Origin',(1.4,2.5,-33.5814213562373)) ;
#145200=CARTESIAN_POINT('',(1.5,2.5,-33.5814213562373)) ;
#145201=CARTESIAN_POINT('',(1.5,2.5,-33.5814213562373)) ;
#145202=CARTESIAN_POINT('',(7.9,2.5,-33.5814213562373)) ;
#145203=CARTESIAN_POINT('',(1.4,2.5,-33.5814213562373)) ;
#145204=CARTESIAN_POINT('',(7.9,2.5,-33.69)) ;
#145205=CARTESIAN_POINT('Origin',(1.4,2.6,-33.5814213562373)) ;
#145206=CARTESIAN_POINT('',(1.5,2.52928932188135,-33.5107106781187)) ;
#145207=CARTESIAN_POINT('Origin',(1.5,2.6,-33.5814213562373)) ;
#145208=CARTESIAN_POINT('',(7.9,2.52928932188135,-33.5107106781187)) ;
#145209=CARTESIAN_POINT('',(1.4,2.52928932188135,-33.5107106781187)) ;
#145210=CARTESIAN_POINT('Origin',(7.9,2.6,-33.5814213562373)) ;
#145211=CARTESIAN_POINT('Origin',(1.4,3.07928932188135,-32.9607106781187)) ;
#145212=CARTESIAN_POINT('',(1.5,3.07928932188135,-32.9607106781187)) ;
#145213=CARTESIAN_POINT('',(7.9,3.07928932188135,-32.9607106781187)) ;
#145214=CARTESIAN_POINT('',(1.4,3.07928932188135,-32.9607106781187)) ;
#145215=CARTESIAN_POINT('',(7.9,2.52928932188135,-33.5107106781187)) ;
#145216=CARTESIAN_POINT('Origin',(1.4,3.15,-33.0314213562373)) ;
#145217=CARTESIAN_POINT('',(7.9,3.25,-33.0314213562373)) ;
#145218=CARTESIAN_POINT('',(1.4,3.25,-33.0314213562373)) ;
#145219=CARTESIAN_POINT('Origin',(7.9,3.15,-33.0314213562373)) ;
#145220=CARTESIAN_POINT('Origin',(1.4,3.25,-35.5485786437627)) ;
#145221=CARTESIAN_POINT('',(1.5,3.25,-35.5485786437627)) ;
#145222=CARTESIAN_POINT('',(7.9,3.25,-33.0314213562373)) ;
#145223=CARTESIAN_POINT('Origin',(1.4,2.52928932188134,-35.0692893218813)) ;
#145224=CARTESIAN_POINT('',(1.5,2.52928932188134,-35.0692893218813)) ;
#145225=CARTESIAN_POINT('',(1.5,2.52928932188134,-35.0692893218813)) ;
#145226=CARTESIAN_POINT('',(7.9,2.52928932188134,-35.0692893218813)) ;
#145227=CARTESIAN_POINT('',(1.4,2.52928932188134,-35.0692893218813)) ;
#145228=CARTESIAN_POINT('',(7.9,3.07928932188135,-35.6192893218813)) ;
#145229=CARTESIAN_POINT('Origin',(1.4,2.6,-34.9985786437627)) ;
#145230=CARTESIAN_POINT('',(1.5,2.5,-34.9985786437627)) ;
#145231=CARTESIAN_POINT('Origin',(1.5,2.6,-34.9985786437627)) ;
#145232=CARTESIAN_POINT('',(7.9,2.5,-34.9985786437627)) ;
#145233=CARTESIAN_POINT('',(1.4,2.5,-34.9985786437627)) ;
#145234=CARTESIAN_POINT('Origin',(7.9,2.6,-34.9985786437627)) ;
#145235=CARTESIAN_POINT('Origin',(1.4,2.5,-34.89)) ;
#145236=CARTESIAN_POINT('',(1.5,2.5,-34.89)) ;
#145237=CARTESIAN_POINT('',(1.5,2.5,-34.89)) ;
#145238=CARTESIAN_POINT('',(7.9,2.5,-34.89)) ;
#145239=CARTESIAN_POINT('',(1.4,2.5,-34.89)) ;
#145240=CARTESIAN_POINT('',(7.9,2.5,-34.9985786437627)) ;
#145241=CARTESIAN_POINT('Origin',(1.4,2.4,-34.89)) ;
#145242=CARTESIAN_POINT('',(1.5,2.4,-34.79)) ;
#145243=CARTESIAN_POINT('Origin',(1.5,2.4,-34.89)) ;
#145244=CARTESIAN_POINT('',(7.9,2.4,-34.79)) ;
#145245=CARTESIAN_POINT('',(1.4,2.4,-34.79)) ;
#145246=CARTESIAN_POINT('Origin',(7.9,2.4,-34.89)) ;
#145247=CARTESIAN_POINT('Origin',(1.4,2.1,-34.79)) ;
#145248=CARTESIAN_POINT('',(1.5,2.1,-34.79)) ;
#145249=CARTESIAN_POINT('',(1.5,2.1,-34.79)) ;
#145250=CARTESIAN_POINT('',(7.9,2.1,-34.79)) ;
#145251=CARTESIAN_POINT('',(1.4,2.1,-34.79)) ;
#145252=CARTESIAN_POINT('',(7.9,2.4,-34.79)) ;
#145253=CARTESIAN_POINT('Origin',(1.4,2.1,-34.89)) ;
#145254=CARTESIAN_POINT('',(1.5,2.,-34.89)) ;
#145255=CARTESIAN_POINT('Origin',(1.5,2.1,-34.89)) ;
#145256=CARTESIAN_POINT('',(7.9,2.,-34.89)) ;
#145257=CARTESIAN_POINT('',(1.4,2.,-34.89)) ;
#145258=CARTESIAN_POINT('Origin',(7.9,2.1,-34.89)) ;
#145259=CARTESIAN_POINT('Origin',(1.4,2.,-34.89)) ;
#145260=CARTESIAN_POINT('',(1.5,2.,-35.84)) ;
#145261=CARTESIAN_POINT('',(1.5,2.,-35.84)) ;
#145262=CARTESIAN_POINT('',(7.9,2.,-35.84)) ;
#145263=CARTESIAN_POINT('',(1.4,2.,-35.84)) ;
#145264=CARTESIAN_POINT('',(7.9,2.,-34.89)) ;
#145265=CARTESIAN_POINT('Origin',(1.4,1.9,-35.84)) ;
#145266=CARTESIAN_POINT('',(1.5,1.9,-35.94)) ;
#145267=CARTESIAN_POINT('Origin',(1.5,1.9,-35.84)) ;
#145268=CARTESIAN_POINT('',(7.9,1.9,-35.94)) ;
#145269=CARTESIAN_POINT('',(1.4,1.9,-35.94)) ;
#145270=CARTESIAN_POINT('Origin',(7.9,1.9,-35.84)) ;
#145271=CARTESIAN_POINT('Origin',(1.4,1.9,-35.94)) ;
#145272=CARTESIAN_POINT('',(1.5,-2.15,-35.94)) ;
#145273=CARTESIAN_POINT('',(1.5,-2.15,-35.94)) ;
#145274=CARTESIAN_POINT('',(7.9,-2.15,-35.94)) ;
#145275=CARTESIAN_POINT('',(1.4,-2.15,-35.94)) ;
#145276=CARTESIAN_POINT('',(7.9,1.9,-35.94)) ;
#145277=CARTESIAN_POINT('Origin',(1.4,-2.15,-35.84)) ;
#145278=CARTESIAN_POINT('',(1.5,-2.25,-35.84)) ;
#145279=CARTESIAN_POINT('Origin',(1.5,-2.15,-35.84)) ;
#145280=CARTESIAN_POINT('',(7.9,-2.25,-35.84)) ;
#145281=CARTESIAN_POINT('',(1.4,-2.25,-35.84)) ;
#145282=CARTESIAN_POINT('Origin',(7.9,-2.15,-35.84)) ;
#145283=CARTESIAN_POINT('Origin',(1.4,-2.25,-35.1931195934094)) ;
#145284=CARTESIAN_POINT('',(1.5,-2.25,-35.1931195934094)) ;
#145285=CARTESIAN_POINT('',(1.5,-2.25,-35.1931195934094)) ;
#145286=CARTESIAN_POINT('',(7.9,-2.25,-35.1931195934094)) ;
#145287=CARTESIAN_POINT('',(1.4,-2.25,-35.1931195934094)) ;
#145288=CARTESIAN_POINT('',(7.9,-2.25,-35.84)) ;
#145289=CARTESIAN_POINT('Origin',(1.4,-2.15,-35.1931195934094)) ;
#145290=CARTESIAN_POINT('',(1.5,-2.23576512455516,-35.1416964137135)) ;
#145291=CARTESIAN_POINT('Origin',(1.5,-2.15,-35.1931195934094)) ;
#145292=CARTESIAN_POINT('',(7.9,-2.23576512455516,-35.1416964137135)) ;
#145293=CARTESIAN_POINT('',(1.4,-2.23576512455516,-35.1416964137135)) ;
#145294=CARTESIAN_POINT('Origin',(7.9,-2.15,-35.1931195934094)) ;
#145295=CARTESIAN_POINT('Origin',(1.4,-3.65625,-34.29)) ;
#145296=CARTESIAN_POINT('',(1.5,-2.23576512455516,-33.4383035862865)) ;
#145297=CARTESIAN_POINT('Origin',(1.5,-3.65625,-34.29)) ;
#145298=CARTESIAN_POINT('',(7.9,-2.23576512455516,-33.4383035862865)) ;
#145299=CARTESIAN_POINT('',(1.4,-2.23576512455516,-33.4383035862865)) ;
#145300=CARTESIAN_POINT('Origin',(7.9,-3.65625,-34.29)) ;
#145301=CARTESIAN_POINT('Origin',(1.4,-2.15,-33.3868804065906)) ;
#145302=CARTESIAN_POINT('',(1.5,-2.25,-33.3868804065906)) ;
#145303=CARTESIAN_POINT('Origin',(1.5,-2.15,-33.3868804065906)) ;
#145304=CARTESIAN_POINT('',(7.9,-2.25,-33.3868804065906)) ;
#145305=CARTESIAN_POINT('',(1.4,-2.25,-33.3868804065906)) ;
#145306=CARTESIAN_POINT('Origin',(7.9,-2.15,-33.3868804065906)) ;
#145307=CARTESIAN_POINT('Origin',(1.4,-2.25,-32.74)) ;
#145308=CARTESIAN_POINT('',(1.5,-2.25,-32.74)) ;
#145309=CARTESIAN_POINT('',(1.5,-2.25,-32.74)) ;
#145310=CARTESIAN_POINT('',(7.9,-2.25,-32.74)) ;
#145311=CARTESIAN_POINT('',(1.4,-2.25,-32.74)) ;
#145312=CARTESIAN_POINT('',(7.9,-2.25,-33.3868804065906)) ;
#145313=CARTESIAN_POINT('Origin',(1.4,-2.15,-32.74)) ;
#145314=CARTESIAN_POINT('',(1.5,-2.15,-32.64)) ;
#145315=CARTESIAN_POINT('Origin',(1.5,-2.15,-32.74)) ;
#145316=CARTESIAN_POINT('',(7.9,-2.15,-32.64)) ;
#145317=CARTESIAN_POINT('',(1.4,-2.15,-32.64)) ;
#145318=CARTESIAN_POINT('Origin',(7.9,-2.15,-32.74)) ;
#145319=CARTESIAN_POINT('Origin',(1.4,1.9,-32.64)) ;
#145320=CARTESIAN_POINT('',(1.5,1.9,-32.64)) ;
#145321=CARTESIAN_POINT('',(1.5,1.9,-32.64)) ;
#145322=CARTESIAN_POINT('',(7.9,1.9,-32.64)) ;
#145323=CARTESIAN_POINT('',(1.4,1.9,-32.64)) ;
#145324=CARTESIAN_POINT('',(7.9,-2.15,-32.64)) ;
#145325=CARTESIAN_POINT('Origin',(1.4,1.9,-32.74)) ;
#145326=CARTESIAN_POINT('',(1.5,2.,-32.74)) ;
#145327=CARTESIAN_POINT('Origin',(1.5,1.9,-32.74)) ;
#145328=CARTESIAN_POINT('',(7.9,2.,-32.74)) ;
#145329=CARTESIAN_POINT('',(1.4,2.,-32.74)) ;
#145330=CARTESIAN_POINT('Origin',(7.9,1.9,-32.74)) ;
#145331=CARTESIAN_POINT('Origin',(1.4,2.,-32.74)) ;
#145332=CARTESIAN_POINT('',(1.5,2.,-33.69)) ;
#145333=CARTESIAN_POINT('',(7.9,2.,-32.74)) ;
#145334=CARTESIAN_POINT('Origin',(1.4,2.1,-33.69)) ;
#145335=CARTESIAN_POINT('',(1.4,2.6,-33.69)) ;
#145336=CARTESIAN_POINT('',(1.4,2.4,-33.89)) ;
#145337=CARTESIAN_POINT('Origin',(1.4,2.4,-33.69)) ;
#145338=CARTESIAN_POINT('',(1.4,2.1,-33.89)) ;
#145339=CARTESIAN_POINT('',(1.4,2.1,-33.89)) ;
#145340=CARTESIAN_POINT('',(1.4,1.9,-33.69)) ;
#145341=CARTESIAN_POINT('Origin',(1.4,2.1,-33.69)) ;
#145342=CARTESIAN_POINT('',(1.4,1.9,-32.74)) ;
#145343=CARTESIAN_POINT('',(1.4,1.9,-32.74)) ;
#145344=CARTESIAN_POINT('',(1.4,-2.15,-32.74)) ;
#145345=CARTESIAN_POINT('',(1.4,-2.15,-32.74)) ;
#145346=CARTESIAN_POINT('',(1.4,-2.15,-33.3868804065906)) ;
#145347=CARTESIAN_POINT('',(1.4,-2.15,-33.3868804065906)) ;
#145348=CARTESIAN_POINT('',(1.4,-2.15,-35.1931195934094)) ;
#145349=CARTESIAN_POINT('Origin',(1.4,-3.65625,-34.29)) ;
#145350=CARTESIAN_POINT('',(1.4,-2.15,-35.84)) ;
#145351=CARTESIAN_POINT('',(1.4,-2.15,-35.84)) ;
#145352=CARTESIAN_POINT('',(1.4,1.9,-35.84)) ;
#145353=CARTESIAN_POINT('',(1.4,1.9,-35.84)) ;
#145354=CARTESIAN_POINT('',(1.4,1.9,-34.89)) ;
#145355=CARTESIAN_POINT('',(1.4,1.9,-34.89)) ;
#145356=CARTESIAN_POINT('',(1.4,2.1,-34.69)) ;
#145357=CARTESIAN_POINT('Origin',(1.4,2.1,-34.89)) ;
#145358=CARTESIAN_POINT('',(1.4,2.4,-34.69)) ;
#145359=CARTESIAN_POINT('',(1.4,2.4,-34.69)) ;
#145360=CARTESIAN_POINT('',(1.4,2.6,-34.89)) ;
#145361=CARTESIAN_POINT('Origin',(1.4,2.4,-34.89)) ;
#145362=CARTESIAN_POINT('',(1.4,2.6,-34.9985786437627)) ;
#145363=CARTESIAN_POINT('',(1.4,2.6,-34.9985786437627)) ;
#145364=CARTESIAN_POINT('',(1.4,3.15,-35.5485786437627)) ;
#145365=CARTESIAN_POINT('',(1.4,3.15,-35.5485786437627)) ;
#145366=CARTESIAN_POINT('',(1.4,3.15,-33.0314213562373)) ;
#145367=CARTESIAN_POINT('',(1.4,2.6,-33.5814213562373)) ;
#145368=CARTESIAN_POINT('',(1.4,2.6,-33.5814213562373)) ;
#145369=CARTESIAN_POINT('',(1.4,2.6,-33.69)) ;
#145370=CARTESIAN_POINT('Origin',(1.4,2.1,-29.88)) ;
#145371=CARTESIAN_POINT('',(1.5,2.,-29.88)) ;
#145372=CARTESIAN_POINT('',(7.9,2.,-29.88)) ;
#145373=CARTESIAN_POINT('',(1.4,2.,-29.88)) ;
#145374=CARTESIAN_POINT('',(1.5,2.1,-29.98)) ;
#145375=CARTESIAN_POINT('Origin',(1.5,2.1,-29.88)) ;
#145376=CARTESIAN_POINT('',(7.9,2.1,-29.98)) ;
#145377=CARTESIAN_POINT('',(1.4,2.1,-29.98)) ;
#145378=CARTESIAN_POINT('Origin',(7.9,2.1,-29.88)) ;
#145379=CARTESIAN_POINT('Origin',(1.4,2.4,-29.98)) ;
#145380=CARTESIAN_POINT('',(1.5,2.4,-29.98)) ;
#145381=CARTESIAN_POINT('',(1.5,2.4,-29.98)) ;
#145382=CARTESIAN_POINT('',(7.9,2.4,-29.98)) ;
#145383=CARTESIAN_POINT('',(1.4,2.4,-29.98)) ;
#145384=CARTESIAN_POINT('',(7.9,2.1,-29.98)) ;
#145385=CARTESIAN_POINT('Origin',(1.4,2.4,-29.88)) ;
#145386=CARTESIAN_POINT('',(1.5,2.5,-29.88)) ;
#145387=CARTESIAN_POINT('Origin',(1.5,2.4,-29.88)) ;
#145388=CARTESIAN_POINT('',(7.9,2.5,-29.88)) ;
#145389=CARTESIAN_POINT('',(1.4,2.5,-29.88)) ;
#145390=CARTESIAN_POINT('Origin',(7.9,2.4,-29.88)) ;
#145391=CARTESIAN_POINT('Origin',(1.4,2.5,-29.7714213562373)) ;
#145392=CARTESIAN_POINT('',(1.5,2.5,-29.7714213562373)) ;
#145393=CARTESIAN_POINT('',(1.5,2.5,-29.7714213562373)) ;
#145394=CARTESIAN_POINT('',(7.9,2.5,-29.7714213562373)) ;
#145395=CARTESIAN_POINT('',(1.4,2.5,-29.7714213562373)) ;
#145396=CARTESIAN_POINT('',(7.9,2.5,-29.88)) ;
#145397=CARTESIAN_POINT('Origin',(1.4,2.6,-29.7714213562373)) ;
#145398=CARTESIAN_POINT('',(1.5,2.52928932188135,-29.7007106781187)) ;
#145399=CARTESIAN_POINT('Origin',(1.5,2.6,-29.7714213562373)) ;
#145400=CARTESIAN_POINT('',(7.9,2.52928932188135,-29.7007106781187)) ;
#145401=CARTESIAN_POINT('',(1.4,2.52928932188135,-29.7007106781187)) ;
#145402=CARTESIAN_POINT('Origin',(7.9,2.6,-29.7714213562373)) ;
#145403=CARTESIAN_POINT('Origin',(1.4,3.07928932188135,-29.1507106781187)) ;
#145404=CARTESIAN_POINT('',(1.5,3.07928932188135,-29.1507106781187)) ;
#145405=CARTESIAN_POINT('',(7.9,3.07928932188135,-29.1507106781187)) ;
#145406=CARTESIAN_POINT('',(1.4,3.07928932188135,-29.1507106781187)) ;
#145407=CARTESIAN_POINT('',(7.9,2.52928932188135,-29.7007106781187)) ;
#145408=CARTESIAN_POINT('Origin',(1.4,3.15,-29.2214213562373)) ;
#145409=CARTESIAN_POINT('',(7.9,3.25,-29.2214213562373)) ;
#145410=CARTESIAN_POINT('',(1.4,3.25,-29.2214213562373)) ;
#145411=CARTESIAN_POINT('Origin',(7.9,3.15,-29.2214213562373)) ;
#145412=CARTESIAN_POINT('Origin',(1.4,3.25,-31.7385786437627)) ;
#145413=CARTESIAN_POINT('',(1.5,3.25,-31.7385786437627)) ;
#145414=CARTESIAN_POINT('',(7.9,3.25,-29.2214213562373)) ;
#145415=CARTESIAN_POINT('Origin',(1.4,2.52928932188134,-31.2592893218813)) ;
#145416=CARTESIAN_POINT('',(1.5,2.52928932188134,-31.2592893218813)) ;
#145417=CARTESIAN_POINT('',(1.5,2.52928932188135,-31.2592893218813)) ;
#145418=CARTESIAN_POINT('',(7.9,2.52928932188134,-31.2592893218813)) ;
#145419=CARTESIAN_POINT('',(1.4,2.52928932188134,-31.2592893218813)) ;
#145420=CARTESIAN_POINT('',(7.9,3.07928932188135,-31.8092893218813)) ;
#145421=CARTESIAN_POINT('Origin',(1.4,2.6,-31.1885786437627)) ;
#145422=CARTESIAN_POINT('',(1.5,2.5,-31.1885786437627)) ;
#145423=CARTESIAN_POINT('Origin',(1.5,2.6,-31.1885786437627)) ;
#145424=CARTESIAN_POINT('',(7.9,2.5,-31.1885786437627)) ;
#145425=CARTESIAN_POINT('',(1.4,2.5,-31.1885786437627)) ;
#145426=CARTESIAN_POINT('Origin',(7.9,2.6,-31.1885786437627)) ;
#145427=CARTESIAN_POINT('Origin',(1.4,2.5,-31.08)) ;
#145428=CARTESIAN_POINT('',(1.5,2.5,-31.08)) ;
#145429=CARTESIAN_POINT('',(1.5,2.5,-31.08)) ;
#145430=CARTESIAN_POINT('',(7.9,2.5,-31.08)) ;
#145431=CARTESIAN_POINT('',(1.4,2.5,-31.08)) ;
#145432=CARTESIAN_POINT('',(7.9,2.5,-31.1885786437627)) ;
#145433=CARTESIAN_POINT('Origin',(1.4,2.4,-31.08)) ;
#145434=CARTESIAN_POINT('',(1.5,2.4,-30.98)) ;
#145435=CARTESIAN_POINT('Origin',(1.5,2.4,-31.08)) ;
#145436=CARTESIAN_POINT('',(7.9,2.4,-30.98)) ;
#145437=CARTESIAN_POINT('',(1.4,2.4,-30.98)) ;
#145438=CARTESIAN_POINT('Origin',(7.9,2.4,-31.08)) ;
#145439=CARTESIAN_POINT('Origin',(1.4,2.1,-30.98)) ;
#145440=CARTESIAN_POINT('',(1.5,2.1,-30.98)) ;
#145441=CARTESIAN_POINT('',(1.5,2.1,-30.98)) ;
#145442=CARTESIAN_POINT('',(7.9,2.1,-30.98)) ;
#145443=CARTESIAN_POINT('',(1.4,2.1,-30.98)) ;
#145444=CARTESIAN_POINT('',(7.9,2.4,-30.98)) ;
#145445=CARTESIAN_POINT('Origin',(1.4,2.1,-31.08)) ;
#145446=CARTESIAN_POINT('',(1.5,2.,-31.08)) ;
#145447=CARTESIAN_POINT('Origin',(1.5,2.1,-31.08)) ;
#145448=CARTESIAN_POINT('',(7.9,2.,-31.08)) ;
#145449=CARTESIAN_POINT('',(1.4,2.,-31.08)) ;
#145450=CARTESIAN_POINT('Origin',(7.9,2.1,-31.08)) ;
#145451=CARTESIAN_POINT('Origin',(1.4,2.,-31.08)) ;
#145452=CARTESIAN_POINT('',(1.5,2.,-32.03)) ;
#145453=CARTESIAN_POINT('',(1.5,2.,-32.03)) ;
#145454=CARTESIAN_POINT('',(7.9,2.,-32.03)) ;
#145455=CARTESIAN_POINT('',(1.4,2.,-32.03)) ;
#145456=CARTESIAN_POINT('',(7.9,2.,-31.08)) ;
#145457=CARTESIAN_POINT('Origin',(1.4,1.9,-32.03)) ;
#145458=CARTESIAN_POINT('',(1.5,1.9,-32.13)) ;
#145459=CARTESIAN_POINT('Origin',(1.5,1.9,-32.03)) ;
#145460=CARTESIAN_POINT('',(7.9,1.9,-32.13)) ;
#145461=CARTESIAN_POINT('',(1.4,1.9,-32.13)) ;
#145462=CARTESIAN_POINT('Origin',(7.9,1.9,-32.03)) ;
#145463=CARTESIAN_POINT('Origin',(1.4,1.9,-32.13)) ;
#145464=CARTESIAN_POINT('',(1.5,-2.15,-32.13)) ;
#145465=CARTESIAN_POINT('',(1.5,-2.15,-32.13)) ;
#145466=CARTESIAN_POINT('',(7.9,-2.15,-32.13)) ;
#145467=CARTESIAN_POINT('',(1.4,-2.15,-32.13)) ;
#145468=CARTESIAN_POINT('',(7.9,1.9,-32.13)) ;
#145469=CARTESIAN_POINT('Origin',(1.4,-2.15,-32.03)) ;
#145470=CARTESIAN_POINT('',(1.5,-2.25,-32.03)) ;
#145471=CARTESIAN_POINT('Origin',(1.5,-2.15,-32.03)) ;
#145472=CARTESIAN_POINT('',(7.9,-2.25,-32.03)) ;
#145473=CARTESIAN_POINT('',(1.4,-2.25,-32.03)) ;
#145474=CARTESIAN_POINT('Origin',(7.9,-2.15,-32.03)) ;
#145475=CARTESIAN_POINT('Origin',(1.4,-2.25,-31.3831195934094)) ;
#145476=CARTESIAN_POINT('',(1.5,-2.25,-31.3831195934094)) ;
#145477=CARTESIAN_POINT('',(1.5,-2.25,-31.3831195934094)) ;
#145478=CARTESIAN_POINT('',(7.9,-2.25,-31.3831195934094)) ;
#145479=CARTESIAN_POINT('',(1.4,-2.25,-31.3831195934094)) ;
#145480=CARTESIAN_POINT('',(7.9,-2.25,-32.03)) ;
#145481=CARTESIAN_POINT('Origin',(1.4,-2.15,-31.3831195934094)) ;
#145482=CARTESIAN_POINT('',(1.5,-2.23576512455516,-31.3316964137135)) ;
#145483=CARTESIAN_POINT('Origin',(1.5,-2.15,-31.3831195934094)) ;
#145484=CARTESIAN_POINT('',(7.9,-2.23576512455516,-31.3316964137135)) ;
#145485=CARTESIAN_POINT('',(1.4,-2.23576512455516,-31.3316964137135)) ;
#145486=CARTESIAN_POINT('Origin',(7.9,-2.15,-31.3831195934094)) ;
#145487=CARTESIAN_POINT('Origin',(1.4,-3.65625,-30.48)) ;
#145488=CARTESIAN_POINT('',(1.5,-2.23576512455516,-29.6283035862865)) ;
#145489=CARTESIAN_POINT('Origin',(1.5,-3.65625,-30.48)) ;
#145490=CARTESIAN_POINT('',(7.9,-2.23576512455516,-29.6283035862865)) ;
#145491=CARTESIAN_POINT('',(1.4,-2.23576512455516,-29.6283035862865)) ;
#145492=CARTESIAN_POINT('Origin',(7.9,-3.65625,-30.48)) ;
#145493=CARTESIAN_POINT('Origin',(1.4,-2.15,-29.5768804065906)) ;
#145494=CARTESIAN_POINT('',(1.5,-2.25,-29.5768804065906)) ;
#145495=CARTESIAN_POINT('Origin',(1.5,-2.15,-29.5768804065906)) ;
#145496=CARTESIAN_POINT('',(7.9,-2.25,-29.5768804065906)) ;
#145497=CARTESIAN_POINT('',(1.4,-2.25,-29.5768804065906)) ;
#145498=CARTESIAN_POINT('Origin',(7.9,-2.15,-29.5768804065906)) ;
#145499=CARTESIAN_POINT('Origin',(1.4,-2.25,-28.93)) ;
#145500=CARTESIAN_POINT('',(1.5,-2.25,-28.93)) ;
#145501=CARTESIAN_POINT('',(1.5,-2.25,-28.93)) ;
#145502=CARTESIAN_POINT('',(7.9,-2.25,-28.93)) ;
#145503=CARTESIAN_POINT('',(1.4,-2.25,-28.93)) ;
#145504=CARTESIAN_POINT('',(7.9,-2.25,-29.5768804065906)) ;
#145505=CARTESIAN_POINT('Origin',(1.4,-2.15,-28.93)) ;
#145506=CARTESIAN_POINT('',(1.5,-2.15,-28.83)) ;
#145507=CARTESIAN_POINT('Origin',(1.5,-2.15,-28.93)) ;
#145508=CARTESIAN_POINT('',(7.9,-2.15,-28.83)) ;
#145509=CARTESIAN_POINT('',(1.4,-2.15,-28.83)) ;
#145510=CARTESIAN_POINT('Origin',(7.9,-2.15,-28.93)) ;
#145511=CARTESIAN_POINT('Origin',(1.4,1.9,-28.83)) ;
#145512=CARTESIAN_POINT('',(1.5,1.9,-28.83)) ;
#145513=CARTESIAN_POINT('',(1.5,1.9,-28.83)) ;
#145514=CARTESIAN_POINT('',(7.9,1.9,-28.83)) ;
#145515=CARTESIAN_POINT('',(1.4,1.9,-28.83)) ;
#145516=CARTESIAN_POINT('',(7.9,-2.15,-28.83)) ;
#145517=CARTESIAN_POINT('Origin',(1.4,1.9,-28.93)) ;
#145518=CARTESIAN_POINT('',(1.5,2.,-28.93)) ;
#145519=CARTESIAN_POINT('Origin',(1.5,1.9,-28.93)) ;
#145520=CARTESIAN_POINT('',(7.9,2.,-28.93)) ;
#145521=CARTESIAN_POINT('',(1.4,2.,-28.93)) ;
#145522=CARTESIAN_POINT('Origin',(7.9,1.9,-28.93)) ;
#145523=CARTESIAN_POINT('Origin',(1.4,2.,-28.93)) ;
#145524=CARTESIAN_POINT('',(1.5,2.,-29.88)) ;
#145525=CARTESIAN_POINT('',(7.9,2.,-28.93)) ;
#145526=CARTESIAN_POINT('Origin',(1.4,2.1,-29.88)) ;
#145527=CARTESIAN_POINT('',(1.4,2.6,-29.88)) ;
#145528=CARTESIAN_POINT('',(1.4,2.4,-30.08)) ;
#145529=CARTESIAN_POINT('Origin',(1.4,2.4,-29.88)) ;
#145530=CARTESIAN_POINT('',(1.4,2.1,-30.08)) ;
#145531=CARTESIAN_POINT('',(1.4,2.1,-30.08)) ;
#145532=CARTESIAN_POINT('',(1.4,1.9,-29.88)) ;
#145533=CARTESIAN_POINT('Origin',(1.4,2.1,-29.88)) ;
#145534=CARTESIAN_POINT('',(1.4,1.9,-28.93)) ;
#145535=CARTESIAN_POINT('',(1.4,1.9,-28.93)) ;
#145536=CARTESIAN_POINT('',(1.4,-2.15,-28.93)) ;
#145537=CARTESIAN_POINT('',(1.4,-2.15,-28.93)) ;
#145538=CARTESIAN_POINT('',(1.4,-2.15,-29.5768804065906)) ;
#145539=CARTESIAN_POINT('',(1.4,-2.15,-29.5768804065906)) ;
#145540=CARTESIAN_POINT('',(1.4,-2.15,-31.3831195934094)) ;
#145541=CARTESIAN_POINT('Origin',(1.4,-3.65625,-30.48)) ;
#145542=CARTESIAN_POINT('',(1.4,-2.15,-32.03)) ;
#145543=CARTESIAN_POINT('',(1.4,-2.15,-32.03)) ;
#145544=CARTESIAN_POINT('',(1.4,1.9,-32.03)) ;
#145545=CARTESIAN_POINT('',(1.4,1.9,-32.03)) ;
#145546=CARTESIAN_POINT('',(1.4,1.9,-31.08)) ;
#145547=CARTESIAN_POINT('',(1.4,1.9,-31.08)) ;
#145548=CARTESIAN_POINT('',(1.4,2.1,-30.88)) ;
#145549=CARTESIAN_POINT('Origin',(1.4,2.1,-31.08)) ;
#145550=CARTESIAN_POINT('',(1.4,2.4,-30.88)) ;
#145551=CARTESIAN_POINT('',(1.4,2.4,-30.88)) ;
#145552=CARTESIAN_POINT('',(1.4,2.6,-31.08)) ;
#145553=CARTESIAN_POINT('Origin',(1.4,2.4,-31.08)) ;
#145554=CARTESIAN_POINT('',(1.4,2.6,-31.1885786437627)) ;
#145555=CARTESIAN_POINT('',(1.4,2.6,-31.1885786437627)) ;
#145556=CARTESIAN_POINT('',(1.4,3.15,-31.7385786437627)) ;
#145557=CARTESIAN_POINT('',(1.4,3.15,-31.7385786437627)) ;
#145558=CARTESIAN_POINT('',(1.4,3.15,-29.2214213562373)) ;
#145559=CARTESIAN_POINT('',(1.4,2.6,-29.7714213562373)) ;
#145560=CARTESIAN_POINT('',(1.4,2.6,-29.7714213562373)) ;
#145561=CARTESIAN_POINT('',(1.4,2.6,-29.88)) ;
#145562=CARTESIAN_POINT('Origin',(1.4,2.1,-26.07)) ;
#145563=CARTESIAN_POINT('',(1.5,2.,-26.07)) ;
#145564=CARTESIAN_POINT('',(7.9,2.,-26.07)) ;
#145565=CARTESIAN_POINT('',(1.4,2.,-26.07)) ;
#145566=CARTESIAN_POINT('',(1.5,2.1,-26.17)) ;
#145567=CARTESIAN_POINT('Origin',(1.5,2.1,-26.07)) ;
#145568=CARTESIAN_POINT('',(7.9,2.1,-26.17)) ;
#145569=CARTESIAN_POINT('',(1.4,2.1,-26.17)) ;
#145570=CARTESIAN_POINT('Origin',(7.9,2.1,-26.07)) ;
#145571=CARTESIAN_POINT('Origin',(1.4,2.4,-26.17)) ;
#145572=CARTESIAN_POINT('',(1.5,2.4,-26.17)) ;
#145573=CARTESIAN_POINT('',(1.5,2.4,-26.17)) ;
#145574=CARTESIAN_POINT('',(7.9,2.4,-26.17)) ;
#145575=CARTESIAN_POINT('',(1.4,2.4,-26.17)) ;
#145576=CARTESIAN_POINT('',(7.9,2.1,-26.17)) ;
#145577=CARTESIAN_POINT('Origin',(1.4,2.4,-26.07)) ;
#145578=CARTESIAN_POINT('',(1.5,2.5,-26.07)) ;
#145579=CARTESIAN_POINT('Origin',(1.5,2.4,-26.07)) ;
#145580=CARTESIAN_POINT('',(7.9,2.5,-26.07)) ;
#145581=CARTESIAN_POINT('',(1.4,2.5,-26.07)) ;
#145582=CARTESIAN_POINT('Origin',(7.9,2.4,-26.07)) ;
#145583=CARTESIAN_POINT('Origin',(1.4,2.5,-25.9614213562373)) ;
#145584=CARTESIAN_POINT('',(1.5,2.5,-25.9614213562373)) ;
#145585=CARTESIAN_POINT('',(1.5,2.5,-25.9614213562373)) ;
#145586=CARTESIAN_POINT('',(7.9,2.5,-25.9614213562373)) ;
#145587=CARTESIAN_POINT('',(1.4,2.5,-25.9614213562373)) ;
#145588=CARTESIAN_POINT('',(7.9,2.5,-26.07)) ;
#145589=CARTESIAN_POINT('Origin',(1.4,2.6,-25.9614213562373)) ;
#145590=CARTESIAN_POINT('',(1.5,2.52928932188135,-25.8907106781187)) ;
#145591=CARTESIAN_POINT('Origin',(1.5,2.6,-25.9614213562373)) ;
#145592=CARTESIAN_POINT('',(7.9,2.52928932188135,-25.8907106781187)) ;
#145593=CARTESIAN_POINT('',(1.4,2.52928932188135,-25.8907106781187)) ;
#145594=CARTESIAN_POINT('Origin',(7.9,2.6,-25.9614213562373)) ;
#145595=CARTESIAN_POINT('Origin',(1.4,3.07928932188135,-25.3407106781187)) ;
#145596=CARTESIAN_POINT('',(1.5,3.07928932188135,-25.3407106781187)) ;
#145597=CARTESIAN_POINT('',(7.9,3.07928932188135,-25.3407106781187)) ;
#145598=CARTESIAN_POINT('',(1.4,3.07928932188135,-25.3407106781187)) ;
#145599=CARTESIAN_POINT('',(7.9,2.52928932188135,-25.8907106781187)) ;
#145600=CARTESIAN_POINT('Origin',(1.4,3.15,-25.4114213562373)) ;
#145601=CARTESIAN_POINT('',(7.9,3.25,-25.4114213562373)) ;
#145602=CARTESIAN_POINT('',(1.4,3.25,-25.4114213562373)) ;
#145603=CARTESIAN_POINT('Origin',(7.9,3.15,-25.4114213562373)) ;
#145604=CARTESIAN_POINT('Origin',(1.4,3.25,-27.9285786437627)) ;
#145605=CARTESIAN_POINT('',(1.5,3.25,-27.9285786437627)) ;
#145606=CARTESIAN_POINT('',(7.9,3.25,-25.4114213562373)) ;
#145607=CARTESIAN_POINT('Origin',(1.4,2.52928932188134,-27.4492893218813)) ;
#145608=CARTESIAN_POINT('',(1.5,2.52928932188134,-27.4492893218813)) ;
#145609=CARTESIAN_POINT('',(1.5,2.52928932188135,-27.4492893218813)) ;
#145610=CARTESIAN_POINT('',(7.9,2.52928932188134,-27.4492893218813)) ;
#145611=CARTESIAN_POINT('',(1.4,2.52928932188134,-27.4492893218813)) ;
#145612=CARTESIAN_POINT('',(7.9,3.07928932188134,-27.9992893218813)) ;
#145613=CARTESIAN_POINT('Origin',(1.4,2.6,-27.3785786437627)) ;
#145614=CARTESIAN_POINT('',(1.5,2.5,-27.3785786437627)) ;
#145615=CARTESIAN_POINT('Origin',(1.5,2.6,-27.3785786437627)) ;
#145616=CARTESIAN_POINT('',(7.9,2.5,-27.3785786437627)) ;
#145617=CARTESIAN_POINT('',(1.4,2.5,-27.3785786437627)) ;
#145618=CARTESIAN_POINT('Origin',(7.9,2.6,-27.3785786437627)) ;
#145619=CARTESIAN_POINT('Origin',(1.4,2.5,-27.27)) ;
#145620=CARTESIAN_POINT('',(1.5,2.5,-27.27)) ;
#145621=CARTESIAN_POINT('',(1.5,2.5,-27.27)) ;
#145622=CARTESIAN_POINT('',(7.9,2.5,-27.27)) ;
#145623=CARTESIAN_POINT('',(1.4,2.5,-27.27)) ;
#145624=CARTESIAN_POINT('',(7.9,2.5,-27.3785786437627)) ;
#145625=CARTESIAN_POINT('Origin',(1.4,2.4,-27.27)) ;
#145626=CARTESIAN_POINT('',(1.5,2.4,-27.17)) ;
#145627=CARTESIAN_POINT('Origin',(1.5,2.4,-27.27)) ;
#145628=CARTESIAN_POINT('',(7.9,2.4,-27.17)) ;
#145629=CARTESIAN_POINT('',(1.4,2.4,-27.17)) ;
#145630=CARTESIAN_POINT('Origin',(7.9,2.4,-27.27)) ;
#145631=CARTESIAN_POINT('Origin',(1.4,2.1,-27.17)) ;
#145632=CARTESIAN_POINT('',(1.5,2.1,-27.17)) ;
#145633=CARTESIAN_POINT('',(1.5,2.1,-27.17)) ;
#145634=CARTESIAN_POINT('',(7.9,2.1,-27.17)) ;
#145635=CARTESIAN_POINT('',(1.4,2.1,-27.17)) ;
#145636=CARTESIAN_POINT('',(7.9,2.4,-27.17)) ;
#145637=CARTESIAN_POINT('Origin',(1.4,2.1,-27.27)) ;
#145638=CARTESIAN_POINT('',(1.5,2.,-27.27)) ;
#145639=CARTESIAN_POINT('Origin',(1.5,2.1,-27.27)) ;
#145640=CARTESIAN_POINT('',(7.9,2.,-27.27)) ;
#145641=CARTESIAN_POINT('',(1.4,2.,-27.27)) ;
#145642=CARTESIAN_POINT('Origin',(7.9,2.1,-27.27)) ;
#145643=CARTESIAN_POINT('Origin',(1.4,2.,-27.27)) ;
#145644=CARTESIAN_POINT('',(1.5,2.,-28.22)) ;
#145645=CARTESIAN_POINT('',(1.5,2.,-28.22)) ;
#145646=CARTESIAN_POINT('',(7.9,2.,-28.22)) ;
#145647=CARTESIAN_POINT('',(1.4,2.,-28.22)) ;
#145648=CARTESIAN_POINT('',(7.9,2.,-27.27)) ;
#145649=CARTESIAN_POINT('Origin',(1.4,1.9,-28.22)) ;
#145650=CARTESIAN_POINT('',(1.5,1.9,-28.32)) ;
#145651=CARTESIAN_POINT('Origin',(1.5,1.9,-28.22)) ;
#145652=CARTESIAN_POINT('',(7.9,1.9,-28.32)) ;
#145653=CARTESIAN_POINT('',(1.4,1.9,-28.32)) ;
#145654=CARTESIAN_POINT('Origin',(7.9,1.9,-28.22)) ;
#145655=CARTESIAN_POINT('Origin',(1.4,1.9,-28.32)) ;
#145656=CARTESIAN_POINT('',(1.5,-2.15,-28.32)) ;
#145657=CARTESIAN_POINT('',(1.5,-2.15,-28.32)) ;
#145658=CARTESIAN_POINT('',(7.9,-2.15,-28.32)) ;
#145659=CARTESIAN_POINT('',(1.4,-2.15,-28.32)) ;
#145660=CARTESIAN_POINT('',(7.9,1.9,-28.32)) ;
#145661=CARTESIAN_POINT('Origin',(1.4,-2.15,-28.22)) ;
#145662=CARTESIAN_POINT('',(1.5,-2.25,-28.22)) ;
#145663=CARTESIAN_POINT('Origin',(1.5,-2.15,-28.22)) ;
#145664=CARTESIAN_POINT('',(7.9,-2.25,-28.22)) ;
#145665=CARTESIAN_POINT('',(1.4,-2.25,-28.22)) ;
#145666=CARTESIAN_POINT('Origin',(7.9,-2.15,-28.22)) ;
#145667=CARTESIAN_POINT('Origin',(1.4,-2.25,-27.5731195934094)) ;
#145668=CARTESIAN_POINT('',(1.5,-2.25,-27.5731195934094)) ;
#145669=CARTESIAN_POINT('',(1.5,-2.25,-27.5731195934094)) ;
#145670=CARTESIAN_POINT('',(7.9,-2.25,-27.5731195934094)) ;
#145671=CARTESIAN_POINT('',(1.4,-2.25,-27.5731195934094)) ;
#145672=CARTESIAN_POINT('',(7.9,-2.25,-28.22)) ;
#145673=CARTESIAN_POINT('Origin',(1.4,-2.15,-27.5731195934094)) ;
#145674=CARTESIAN_POINT('',(1.5,-2.23576512455516,-27.5216964137135)) ;
#145675=CARTESIAN_POINT('Origin',(1.5,-2.15,-27.5731195934094)) ;
#145676=CARTESIAN_POINT('',(7.9,-2.23576512455516,-27.5216964137135)) ;
#145677=CARTESIAN_POINT('',(1.4,-2.23576512455516,-27.5216964137135)) ;
#145678=CARTESIAN_POINT('Origin',(7.9,-2.15,-27.5731195934094)) ;
#145679=CARTESIAN_POINT('Origin',(1.4,-3.65625,-26.67)) ;
#145680=CARTESIAN_POINT('',(1.5,-2.23576512455516,-25.8183035862865)) ;
#145681=CARTESIAN_POINT('Origin',(1.5,-3.65625,-26.67)) ;
#145682=CARTESIAN_POINT('',(7.9,-2.23576512455516,-25.8183035862865)) ;
#145683=CARTESIAN_POINT('',(1.4,-2.23576512455516,-25.8183035862865)) ;
#145684=CARTESIAN_POINT('Origin',(7.9,-3.65625,-26.67)) ;
#145685=CARTESIAN_POINT('Origin',(1.4,-2.15,-25.7668804065906)) ;
#145686=CARTESIAN_POINT('',(1.5,-2.25,-25.7668804065906)) ;
#145687=CARTESIAN_POINT('Origin',(1.5,-2.15,-25.7668804065906)) ;
#145688=CARTESIAN_POINT('',(7.9,-2.25,-25.7668804065906)) ;
#145689=CARTESIAN_POINT('',(1.4,-2.25,-25.7668804065906)) ;
#145690=CARTESIAN_POINT('Origin',(7.9,-2.15,-25.7668804065906)) ;
#145691=CARTESIAN_POINT('Origin',(1.4,-2.25,-25.12)) ;
#145692=CARTESIAN_POINT('',(1.5,-2.25,-25.12)) ;
#145693=CARTESIAN_POINT('',(1.5,-2.25,-25.12)) ;
#145694=CARTESIAN_POINT('',(7.9,-2.25,-25.12)) ;
#145695=CARTESIAN_POINT('',(1.4,-2.25,-25.12)) ;
#145696=CARTESIAN_POINT('',(7.9,-2.25,-25.7668804065906)) ;
#145697=CARTESIAN_POINT('Origin',(1.4,-2.15,-25.12)) ;
#145698=CARTESIAN_POINT('',(1.5,-2.15,-25.02)) ;
#145699=CARTESIAN_POINT('Origin',(1.5,-2.15,-25.12)) ;
#145700=CARTESIAN_POINT('',(7.9,-2.15,-25.02)) ;
#145701=CARTESIAN_POINT('',(1.4,-2.15,-25.02)) ;
#145702=CARTESIAN_POINT('Origin',(7.9,-2.15,-25.12)) ;
#145703=CARTESIAN_POINT('Origin',(1.4,1.9,-25.02)) ;
#145704=CARTESIAN_POINT('',(1.5,1.9,-25.02)) ;
#145705=CARTESIAN_POINT('',(1.5,1.9,-25.02)) ;
#145706=CARTESIAN_POINT('',(7.9,1.9,-25.02)) ;
#145707=CARTESIAN_POINT('',(1.4,1.9,-25.02)) ;
#145708=CARTESIAN_POINT('',(7.9,-2.15,-25.02)) ;
#145709=CARTESIAN_POINT('Origin',(1.4,1.9,-25.12)) ;
#145710=CARTESIAN_POINT('',(1.5,2.,-25.12)) ;
#145711=CARTESIAN_POINT('Origin',(1.5,1.9,-25.12)) ;
#145712=CARTESIAN_POINT('',(7.9,2.,-25.12)) ;
#145713=CARTESIAN_POINT('',(1.4,2.,-25.12)) ;
#145714=CARTESIAN_POINT('Origin',(7.9,1.9,-25.12)) ;
#145715=CARTESIAN_POINT('Origin',(1.4,2.,-25.12)) ;
#145716=CARTESIAN_POINT('',(1.5,2.,-26.07)) ;
#145717=CARTESIAN_POINT('',(7.9,2.,-25.12)) ;
#145718=CARTESIAN_POINT('Origin',(1.4,2.1,-26.07)) ;
#145719=CARTESIAN_POINT('',(1.4,2.6,-26.07)) ;
#145720=CARTESIAN_POINT('',(1.4,2.4,-26.27)) ;
#145721=CARTESIAN_POINT('Origin',(1.4,2.4,-26.07)) ;
#145722=CARTESIAN_POINT('',(1.4,2.1,-26.27)) ;
#145723=CARTESIAN_POINT('',(1.4,2.1,-26.27)) ;
#145724=CARTESIAN_POINT('',(1.4,1.9,-26.07)) ;
#145725=CARTESIAN_POINT('Origin',(1.4,2.1,-26.07)) ;
#145726=CARTESIAN_POINT('',(1.4,1.9,-25.12)) ;
#145727=CARTESIAN_POINT('',(1.4,1.9,-25.12)) ;
#145728=CARTESIAN_POINT('',(1.4,-2.15,-25.12)) ;
#145729=CARTESIAN_POINT('',(1.4,-2.15,-25.12)) ;
#145730=CARTESIAN_POINT('',(1.4,-2.15,-25.7668804065906)) ;
#145731=CARTESIAN_POINT('',(1.4,-2.15,-25.7668804065906)) ;
#145732=CARTESIAN_POINT('',(1.4,-2.15,-27.5731195934094)) ;
#145733=CARTESIAN_POINT('Origin',(1.4,-3.65625,-26.67)) ;
#145734=CARTESIAN_POINT('',(1.4,-2.15,-28.22)) ;
#145735=CARTESIAN_POINT('',(1.4,-2.15,-28.22)) ;
#145736=CARTESIAN_POINT('',(1.4,1.9,-28.22)) ;
#145737=CARTESIAN_POINT('',(1.4,1.9,-28.22)) ;
#145738=CARTESIAN_POINT('',(1.4,1.9,-27.27)) ;
#145739=CARTESIAN_POINT('',(1.4,1.9,-27.27)) ;
#145740=CARTESIAN_POINT('',(1.4,2.1,-27.07)) ;
#145741=CARTESIAN_POINT('Origin',(1.4,2.1,-27.27)) ;
#145742=CARTESIAN_POINT('',(1.4,2.4,-27.07)) ;
#145743=CARTESIAN_POINT('',(1.4,2.4,-27.07)) ;
#145744=CARTESIAN_POINT('',(1.4,2.6,-27.27)) ;
#145745=CARTESIAN_POINT('Origin',(1.4,2.4,-27.27)) ;
#145746=CARTESIAN_POINT('',(1.4,2.6,-27.3785786437627)) ;
#145747=CARTESIAN_POINT('',(1.4,2.6,-27.3785786437627)) ;
#145748=CARTESIAN_POINT('',(1.4,3.15,-27.9285786437627)) ;
#145749=CARTESIAN_POINT('',(1.4,3.15,-27.9285786437627)) ;
#145750=CARTESIAN_POINT('',(1.4,3.15,-25.4114213562373)) ;
#145751=CARTESIAN_POINT('',(1.4,2.6,-25.9614213562373)) ;
#145752=CARTESIAN_POINT('',(1.4,2.6,-25.9614213562373)) ;
#145753=CARTESIAN_POINT('',(1.4,2.6,-26.07)) ;
#145754=CARTESIAN_POINT('Origin',(1.4,2.1,-22.26)) ;
#145755=CARTESIAN_POINT('',(1.5,2.,-22.26)) ;
#145756=CARTESIAN_POINT('',(7.9,2.,-22.26)) ;
#145757=CARTESIAN_POINT('',(1.4,2.,-22.26)) ;
#145758=CARTESIAN_POINT('',(1.5,2.1,-22.36)) ;
#145759=CARTESIAN_POINT('Origin',(1.5,2.1,-22.26)) ;
#145760=CARTESIAN_POINT('',(7.9,2.1,-22.36)) ;
#145761=CARTESIAN_POINT('',(1.4,2.1,-22.36)) ;
#145762=CARTESIAN_POINT('Origin',(7.9,2.1,-22.26)) ;
#145763=CARTESIAN_POINT('Origin',(1.4,2.4,-22.36)) ;
#145764=CARTESIAN_POINT('',(1.5,2.4,-22.36)) ;
#145765=CARTESIAN_POINT('',(1.5,2.4,-22.36)) ;
#145766=CARTESIAN_POINT('',(7.9,2.4,-22.36)) ;
#145767=CARTESIAN_POINT('',(1.4,2.4,-22.36)) ;
#145768=CARTESIAN_POINT('',(7.9,2.1,-22.36)) ;
#145769=CARTESIAN_POINT('Origin',(1.4,2.4,-22.26)) ;
#145770=CARTESIAN_POINT('',(1.5,2.5,-22.26)) ;
#145771=CARTESIAN_POINT('Origin',(1.5,2.4,-22.26)) ;
#145772=CARTESIAN_POINT('',(7.9,2.5,-22.26)) ;
#145773=CARTESIAN_POINT('',(1.4,2.5,-22.26)) ;
#145774=CARTESIAN_POINT('Origin',(7.9,2.4,-22.26)) ;
#145775=CARTESIAN_POINT('Origin',(1.4,2.5,-22.1514213562373)) ;
#145776=CARTESIAN_POINT('',(1.5,2.5,-22.1514213562373)) ;
#145777=CARTESIAN_POINT('',(1.5,2.5,-22.1514213562373)) ;
#145778=CARTESIAN_POINT('',(7.9,2.5,-22.1514213562373)) ;
#145779=CARTESIAN_POINT('',(1.4,2.5,-22.1514213562373)) ;
#145780=CARTESIAN_POINT('',(7.9,2.5,-22.26)) ;
#145781=CARTESIAN_POINT('Origin',(1.4,2.6,-22.1514213562373)) ;
#145782=CARTESIAN_POINT('',(1.5,2.52928932188135,-22.0807106781187)) ;
#145783=CARTESIAN_POINT('Origin',(1.5,2.6,-22.1514213562373)) ;
#145784=CARTESIAN_POINT('',(7.9,2.52928932188135,-22.0807106781187)) ;
#145785=CARTESIAN_POINT('',(1.4,2.52928932188135,-22.0807106781187)) ;
#145786=CARTESIAN_POINT('Origin',(7.9,2.6,-22.1514213562373)) ;
#145787=CARTESIAN_POINT('Origin',(1.4,3.07928932188135,-21.5307106781187)) ;
#145788=CARTESIAN_POINT('',(1.5,3.07928932188135,-21.5307106781187)) ;
#145789=CARTESIAN_POINT('',(7.9,3.07928932188135,-21.5307106781187)) ;
#145790=CARTESIAN_POINT('',(1.4,3.07928932188135,-21.5307106781187)) ;
#145791=CARTESIAN_POINT('',(7.9,2.52928932188135,-22.0807106781187)) ;
#145792=CARTESIAN_POINT('Origin',(1.4,3.15,-21.6014213562373)) ;
#145793=CARTESIAN_POINT('',(7.9,3.25,-21.6014213562373)) ;
#145794=CARTESIAN_POINT('',(1.4,3.25,-21.6014213562373)) ;
#145795=CARTESIAN_POINT('Origin',(7.9,3.15,-21.6014213562373)) ;
#145796=CARTESIAN_POINT('Origin',(1.4,3.25,-24.1185786437627)) ;
#145797=CARTESIAN_POINT('',(1.5,3.25,-24.1185786437627)) ;
#145798=CARTESIAN_POINT('',(7.9,3.25,-21.6014213562373)) ;
#145799=CARTESIAN_POINT('Origin',(1.4,2.52928932188134,-23.6392893218813)) ;
#145800=CARTESIAN_POINT('',(1.5,2.52928932188134,-23.6392893218813)) ;
#145801=CARTESIAN_POINT('',(1.5,2.52928932188135,-23.6392893218813)) ;
#145802=CARTESIAN_POINT('',(7.9,2.52928932188134,-23.6392893218813)) ;
#145803=CARTESIAN_POINT('',(1.4,2.52928932188134,-23.6392893218813)) ;
#145804=CARTESIAN_POINT('',(7.9,3.07928932188134,-24.1892893218813)) ;
#145805=CARTESIAN_POINT('Origin',(1.4,2.6,-23.5685786437627)) ;
#145806=CARTESIAN_POINT('',(1.5,2.5,-23.5685786437627)) ;
#145807=CARTESIAN_POINT('Origin',(1.5,2.6,-23.5685786437627)) ;
#145808=CARTESIAN_POINT('',(7.9,2.5,-23.5685786437627)) ;
#145809=CARTESIAN_POINT('',(1.4,2.5,-23.5685786437627)) ;
#145810=CARTESIAN_POINT('Origin',(7.9,2.6,-23.5685786437627)) ;
#145811=CARTESIAN_POINT('Origin',(1.4,2.5,-23.46)) ;
#145812=CARTESIAN_POINT('',(1.5,2.5,-23.46)) ;
#145813=CARTESIAN_POINT('',(1.5,2.5,-23.46)) ;
#145814=CARTESIAN_POINT('',(7.9,2.5,-23.46)) ;
#145815=CARTESIAN_POINT('',(1.4,2.5,-23.46)) ;
#145816=CARTESIAN_POINT('',(7.9,2.5,-23.5685786437627)) ;
#145817=CARTESIAN_POINT('Origin',(1.4,2.4,-23.46)) ;
#145818=CARTESIAN_POINT('',(1.5,2.4,-23.36)) ;
#145819=CARTESIAN_POINT('Origin',(1.5,2.4,-23.46)) ;
#145820=CARTESIAN_POINT('',(7.9,2.4,-23.36)) ;
#145821=CARTESIAN_POINT('',(1.4,2.4,-23.36)) ;
#145822=CARTESIAN_POINT('Origin',(7.9,2.4,-23.46)) ;
#145823=CARTESIAN_POINT('Origin',(1.4,2.1,-23.36)) ;
#145824=CARTESIAN_POINT('',(1.5,2.1,-23.36)) ;
#145825=CARTESIAN_POINT('',(1.5,2.1,-23.36)) ;
#145826=CARTESIAN_POINT('',(7.9,2.1,-23.36)) ;
#145827=CARTESIAN_POINT('',(1.4,2.1,-23.36)) ;
#145828=CARTESIAN_POINT('',(7.9,2.4,-23.36)) ;
#145829=CARTESIAN_POINT('Origin',(1.4,2.1,-23.46)) ;
#145830=CARTESIAN_POINT('',(1.5,2.,-23.46)) ;
#145831=CARTESIAN_POINT('Origin',(1.5,2.1,-23.46)) ;
#145832=CARTESIAN_POINT('',(7.9,2.,-23.46)) ;
#145833=CARTESIAN_POINT('',(1.4,2.,-23.46)) ;
#145834=CARTESIAN_POINT('Origin',(7.9,2.1,-23.46)) ;
#145835=CARTESIAN_POINT('Origin',(1.4,2.,-23.46)) ;
#145836=CARTESIAN_POINT('',(1.5,2.,-24.41)) ;
#145837=CARTESIAN_POINT('',(1.5,2.,-24.41)) ;
#145838=CARTESIAN_POINT('',(7.9,2.,-24.41)) ;
#145839=CARTESIAN_POINT('',(1.4,2.,-24.41)) ;
#145840=CARTESIAN_POINT('',(7.9,2.,-23.46)) ;
#145841=CARTESIAN_POINT('Origin',(1.4,1.9,-24.41)) ;
#145842=CARTESIAN_POINT('',(1.5,1.9,-24.51)) ;
#145843=CARTESIAN_POINT('Origin',(1.5,1.9,-24.41)) ;
#145844=CARTESIAN_POINT('',(7.9,1.9,-24.51)) ;
#145845=CARTESIAN_POINT('',(1.4,1.9,-24.51)) ;
#145846=CARTESIAN_POINT('Origin',(7.9,1.9,-24.41)) ;
#145847=CARTESIAN_POINT('Origin',(1.4,1.9,-24.51)) ;
#145848=CARTESIAN_POINT('',(1.5,-2.15,-24.51)) ;
#145849=CARTESIAN_POINT('',(1.5,-2.15,-24.51)) ;
#145850=CARTESIAN_POINT('',(7.9,-2.15,-24.51)) ;
#145851=CARTESIAN_POINT('',(1.4,-2.15,-24.51)) ;
#145852=CARTESIAN_POINT('',(7.9,1.9,-24.51)) ;
#145853=CARTESIAN_POINT('Origin',(1.4,-2.15,-24.41)) ;
#145854=CARTESIAN_POINT('',(1.5,-2.25,-24.41)) ;
#145855=CARTESIAN_POINT('Origin',(1.5,-2.15,-24.41)) ;
#145856=CARTESIAN_POINT('',(7.9,-2.25,-24.41)) ;
#145857=CARTESIAN_POINT('',(1.4,-2.25,-24.41)) ;
#145858=CARTESIAN_POINT('Origin',(7.9,-2.15,-24.41)) ;
#145859=CARTESIAN_POINT('Origin',(1.4,-2.25,-23.7631195934094)) ;
#145860=CARTESIAN_POINT('',(1.5,-2.25,-23.7631195934094)) ;
#145861=CARTESIAN_POINT('',(1.5,-2.25,-23.7631195934094)) ;
#145862=CARTESIAN_POINT('',(7.9,-2.25,-23.7631195934094)) ;
#145863=CARTESIAN_POINT('',(1.4,-2.25,-23.7631195934094)) ;
#145864=CARTESIAN_POINT('',(7.9,-2.25,-24.41)) ;
#145865=CARTESIAN_POINT('Origin',(1.4,-2.15,-23.7631195934094)) ;
#145866=CARTESIAN_POINT('',(1.5,-2.23576512455516,-23.7116964137135)) ;
#145867=CARTESIAN_POINT('Origin',(1.5,-2.15,-23.7631195934094)) ;
#145868=CARTESIAN_POINT('',(7.9,-2.23576512455516,-23.7116964137135)) ;
#145869=CARTESIAN_POINT('',(1.4,-2.23576512455516,-23.7116964137135)) ;
#145870=CARTESIAN_POINT('Origin',(7.9,-2.15,-23.7631195934094)) ;
#145871=CARTESIAN_POINT('Origin',(1.4,-3.65625,-22.86)) ;
#145872=CARTESIAN_POINT('',(1.5,-2.23576512455516,-22.0083035862865)) ;
#145873=CARTESIAN_POINT('Origin',(1.5,-3.65625,-22.86)) ;
#145874=CARTESIAN_POINT('',(7.9,-2.23576512455516,-22.0083035862865)) ;
#145875=CARTESIAN_POINT('',(1.4,-2.23576512455516,-22.0083035862865)) ;
#145876=CARTESIAN_POINT('Origin',(7.9,-3.65625,-22.86)) ;
#145877=CARTESIAN_POINT('Origin',(1.4,-2.15,-21.9568804065906)) ;
#145878=CARTESIAN_POINT('',(1.5,-2.25,-21.9568804065906)) ;
#145879=CARTESIAN_POINT('Origin',(1.5,-2.15,-21.9568804065906)) ;
#145880=CARTESIAN_POINT('',(7.9,-2.25,-21.9568804065906)) ;
#145881=CARTESIAN_POINT('',(1.4,-2.25,-21.9568804065906)) ;
#145882=CARTESIAN_POINT('Origin',(7.9,-2.15,-21.9568804065906)) ;
#145883=CARTESIAN_POINT('Origin',(1.4,-2.25,-21.31)) ;
#145884=CARTESIAN_POINT('',(1.5,-2.25,-21.31)) ;
#145885=CARTESIAN_POINT('',(1.5,-2.25,-21.31)) ;
#145886=CARTESIAN_POINT('',(7.9,-2.25,-21.31)) ;
#145887=CARTESIAN_POINT('',(1.4,-2.25,-21.31)) ;
#145888=CARTESIAN_POINT('',(7.9,-2.25,-21.9568804065906)) ;
#145889=CARTESIAN_POINT('Origin',(1.4,-2.15,-21.31)) ;
#145890=CARTESIAN_POINT('',(1.5,-2.15,-21.21)) ;
#145891=CARTESIAN_POINT('Origin',(1.5,-2.15,-21.31)) ;
#145892=CARTESIAN_POINT('',(7.9,-2.15,-21.21)) ;
#145893=CARTESIAN_POINT('',(1.4,-2.15,-21.21)) ;
#145894=CARTESIAN_POINT('Origin',(7.9,-2.15,-21.31)) ;
#145895=CARTESIAN_POINT('Origin',(1.4,1.9,-21.21)) ;
#145896=CARTESIAN_POINT('',(1.5,1.9,-21.21)) ;
#145897=CARTESIAN_POINT('',(1.5,1.9,-21.21)) ;
#145898=CARTESIAN_POINT('',(7.9,1.9,-21.21)) ;
#145899=CARTESIAN_POINT('',(1.4,1.9,-21.21)) ;
#145900=CARTESIAN_POINT('',(7.9,-2.15,-21.21)) ;
#145901=CARTESIAN_POINT('Origin',(1.4,1.9,-21.31)) ;
#145902=CARTESIAN_POINT('',(1.5,2.,-21.31)) ;
#145903=CARTESIAN_POINT('Origin',(1.5,1.9,-21.31)) ;
#145904=CARTESIAN_POINT('',(7.9,2.,-21.31)) ;
#145905=CARTESIAN_POINT('',(1.4,2.,-21.31)) ;
#145906=CARTESIAN_POINT('Origin',(7.9,1.9,-21.31)) ;
#145907=CARTESIAN_POINT('Origin',(1.4,2.,-21.31)) ;
#145908=CARTESIAN_POINT('',(1.5,2.,-22.26)) ;
#145909=CARTESIAN_POINT('',(7.9,2.,-21.31)) ;
#145910=CARTESIAN_POINT('Origin',(1.4,2.1,-22.26)) ;
#145911=CARTESIAN_POINT('',(1.4,2.6,-22.26)) ;
#145912=CARTESIAN_POINT('',(1.4,2.4,-22.46)) ;
#145913=CARTESIAN_POINT('Origin',(1.4,2.4,-22.26)) ;
#145914=CARTESIAN_POINT('',(1.4,2.1,-22.46)) ;
#145915=CARTESIAN_POINT('',(1.4,2.1,-22.46)) ;
#145916=CARTESIAN_POINT('',(1.4,1.9,-22.26)) ;
#145917=CARTESIAN_POINT('Origin',(1.4,2.1,-22.26)) ;
#145918=CARTESIAN_POINT('',(1.4,1.9,-21.31)) ;
#145919=CARTESIAN_POINT('',(1.4,1.9,-21.31)) ;
#145920=CARTESIAN_POINT('',(1.4,-2.15,-21.31)) ;
#145921=CARTESIAN_POINT('',(1.4,-2.15,-21.31)) ;
#145922=CARTESIAN_POINT('',(1.4,-2.15,-21.9568804065906)) ;
#145923=CARTESIAN_POINT('',(1.4,-2.15,-21.9568804065906)) ;
#145924=CARTESIAN_POINT('',(1.4,-2.15,-23.7631195934094)) ;
#145925=CARTESIAN_POINT('Origin',(1.4,-3.65625,-22.86)) ;
#145926=CARTESIAN_POINT('',(1.4,-2.15,-24.41)) ;
#145927=CARTESIAN_POINT('',(1.4,-2.15,-24.41)) ;
#145928=CARTESIAN_POINT('',(1.4,1.9,-24.41)) ;
#145929=CARTESIAN_POINT('',(1.4,1.9,-24.41)) ;
#145930=CARTESIAN_POINT('',(1.4,1.9,-23.46)) ;
#145931=CARTESIAN_POINT('',(1.4,1.9,-23.46)) ;
#145932=CARTESIAN_POINT('',(1.4,2.1,-23.26)) ;
#145933=CARTESIAN_POINT('Origin',(1.4,2.1,-23.46)) ;
#145934=CARTESIAN_POINT('',(1.4,2.4,-23.26)) ;
#145935=CARTESIAN_POINT('',(1.4,2.4,-23.26)) ;
#145936=CARTESIAN_POINT('',(1.4,2.6,-23.46)) ;
#145937=CARTESIAN_POINT('Origin',(1.4,2.4,-23.46)) ;
#145938=CARTESIAN_POINT('',(1.4,2.6,-23.5685786437627)) ;
#145939=CARTESIAN_POINT('',(1.4,2.6,-23.5685786437627)) ;
#145940=CARTESIAN_POINT('',(1.4,3.15,-24.1185786437627)) ;
#145941=CARTESIAN_POINT('',(1.4,3.15,-24.1185786437627)) ;
#145942=CARTESIAN_POINT('',(1.4,3.15,-21.6014213562373)) ;
#145943=CARTESIAN_POINT('',(1.4,2.6,-22.1514213562373)) ;
#145944=CARTESIAN_POINT('',(1.4,2.6,-22.1514213562373)) ;
#145945=CARTESIAN_POINT('',(1.4,2.6,-22.26)) ;
#145946=CARTESIAN_POINT('Origin',(1.4,2.1,-18.45)) ;
#145947=CARTESIAN_POINT('',(1.5,2.,-18.45)) ;
#145948=CARTESIAN_POINT('',(7.9,2.,-18.45)) ;
#145949=CARTESIAN_POINT('',(1.4,2.,-18.45)) ;
#145950=CARTESIAN_POINT('',(1.5,2.1,-18.55)) ;
#145951=CARTESIAN_POINT('Origin',(1.5,2.1,-18.45)) ;
#145952=CARTESIAN_POINT('',(7.9,2.1,-18.55)) ;
#145953=CARTESIAN_POINT('',(1.4,2.1,-18.55)) ;
#145954=CARTESIAN_POINT('Origin',(7.9,2.1,-18.45)) ;
#145955=CARTESIAN_POINT('Origin',(1.4,2.4,-18.55)) ;
#145956=CARTESIAN_POINT('',(1.5,2.4,-18.55)) ;
#145957=CARTESIAN_POINT('',(1.5,2.4,-18.55)) ;
#145958=CARTESIAN_POINT('',(7.9,2.4,-18.55)) ;
#145959=CARTESIAN_POINT('',(1.4,2.4,-18.55)) ;
#145960=CARTESIAN_POINT('',(7.9,2.1,-18.55)) ;
#145961=CARTESIAN_POINT('Origin',(1.4,2.4,-18.45)) ;
#145962=CARTESIAN_POINT('',(1.5,2.5,-18.45)) ;
#145963=CARTESIAN_POINT('Origin',(1.5,2.4,-18.45)) ;
#145964=CARTESIAN_POINT('',(7.9,2.5,-18.45)) ;
#145965=CARTESIAN_POINT('',(1.4,2.5,-18.45)) ;
#145966=CARTESIAN_POINT('Origin',(7.9,2.4,-18.45)) ;
#145967=CARTESIAN_POINT('Origin',(1.4,2.5,-18.3414213562373)) ;
#145968=CARTESIAN_POINT('',(1.5,2.5,-18.3414213562373)) ;
#145969=CARTESIAN_POINT('',(1.5,2.5,-18.3414213562373)) ;
#145970=CARTESIAN_POINT('',(7.9,2.5,-18.3414213562373)) ;
#145971=CARTESIAN_POINT('',(1.4,2.5,-18.3414213562373)) ;
#145972=CARTESIAN_POINT('',(7.9,2.5,-18.45)) ;
#145973=CARTESIAN_POINT('Origin',(1.4,2.6,-18.3414213562373)) ;
#145974=CARTESIAN_POINT('',(1.5,2.52928932188135,-18.2707106781187)) ;
#145975=CARTESIAN_POINT('Origin',(1.5,2.6,-18.3414213562373)) ;
#145976=CARTESIAN_POINT('',(7.9,2.52928932188135,-18.2707106781187)) ;
#145977=CARTESIAN_POINT('',(1.4,2.52928932188135,-18.2707106781187)) ;
#145978=CARTESIAN_POINT('Origin',(7.9,2.6,-18.3414213562373)) ;
#145979=CARTESIAN_POINT('Origin',(1.4,3.07928932188135,-17.7207106781187)) ;
#145980=CARTESIAN_POINT('',(1.5,3.07928932188135,-17.7207106781187)) ;
#145981=CARTESIAN_POINT('',(7.9,3.07928932188135,-17.7207106781187)) ;
#145982=CARTESIAN_POINT('',(1.4,3.07928932188135,-17.7207106781187)) ;
#145983=CARTESIAN_POINT('',(7.9,2.52928932188135,-18.2707106781187)) ;
#145984=CARTESIAN_POINT('Origin',(1.4,3.15,-17.7914213562373)) ;
#145985=CARTESIAN_POINT('',(7.9,3.25,-17.7914213562373)) ;
#145986=CARTESIAN_POINT('',(1.4,3.25,-17.7914213562373)) ;
#145987=CARTESIAN_POINT('Origin',(7.9,3.15,-17.7914213562373)) ;
#145988=CARTESIAN_POINT('Origin',(1.4,3.25,-20.3085786437627)) ;
#145989=CARTESIAN_POINT('',(1.5,3.25,-20.3085786437627)) ;
#145990=CARTESIAN_POINT('',(7.9,3.25,-17.7914213562373)) ;
#145991=CARTESIAN_POINT('Origin',(1.4,2.52928932188134,-19.8292893218813)) ;
#145992=CARTESIAN_POINT('',(1.5,2.52928932188134,-19.8292893218813)) ;
#145993=CARTESIAN_POINT('',(1.5,2.52928932188135,-19.8292893218813)) ;
#145994=CARTESIAN_POINT('',(7.9,2.52928932188134,-19.8292893218813)) ;
#145995=CARTESIAN_POINT('',(1.4,2.52928932188134,-19.8292893218813)) ;
#145996=CARTESIAN_POINT('',(7.9,3.07928932188134,-20.3792893218813)) ;
#145997=CARTESIAN_POINT('Origin',(1.4,2.6,-19.7585786437627)) ;
#145998=CARTESIAN_POINT('',(1.5,2.5,-19.7585786437627)) ;
#145999=CARTESIAN_POINT('Origin',(1.5,2.6,-19.7585786437627)) ;
#146000=CARTESIAN_POINT('',(7.9,2.5,-19.7585786437627)) ;
#146001=CARTESIAN_POINT('',(1.4,2.5,-19.7585786437627)) ;
#146002=CARTESIAN_POINT('Origin',(7.9,2.6,-19.7585786437627)) ;
#146003=CARTESIAN_POINT('Origin',(1.4,2.5,-19.65)) ;
#146004=CARTESIAN_POINT('',(1.5,2.5,-19.65)) ;
#146005=CARTESIAN_POINT('',(1.5,2.5,-19.65)) ;
#146006=CARTESIAN_POINT('',(7.9,2.5,-19.65)) ;
#146007=CARTESIAN_POINT('',(1.4,2.5,-19.65)) ;
#146008=CARTESIAN_POINT('',(7.9,2.5,-19.7585786437627)) ;
#146009=CARTESIAN_POINT('Origin',(1.4,2.4,-19.65)) ;
#146010=CARTESIAN_POINT('',(1.5,2.4,-19.55)) ;
#146011=CARTESIAN_POINT('Origin',(1.5,2.4,-19.65)) ;
#146012=CARTESIAN_POINT('',(7.9,2.4,-19.55)) ;
#146013=CARTESIAN_POINT('',(1.4,2.4,-19.55)) ;
#146014=CARTESIAN_POINT('Origin',(7.9,2.4,-19.65)) ;
#146015=CARTESIAN_POINT('Origin',(1.4,2.1,-19.55)) ;
#146016=CARTESIAN_POINT('',(1.5,2.1,-19.55)) ;
#146017=CARTESIAN_POINT('',(1.5,2.1,-19.55)) ;
#146018=CARTESIAN_POINT('',(7.9,2.1,-19.55)) ;
#146019=CARTESIAN_POINT('',(1.4,2.1,-19.55)) ;
#146020=CARTESIAN_POINT('',(7.9,2.4,-19.55)) ;
#146021=CARTESIAN_POINT('Origin',(1.4,2.1,-19.65)) ;
#146022=CARTESIAN_POINT('',(1.5,2.,-19.65)) ;
#146023=CARTESIAN_POINT('Origin',(1.5,2.1,-19.65)) ;
#146024=CARTESIAN_POINT('',(7.9,2.,-19.65)) ;
#146025=CARTESIAN_POINT('',(1.4,2.,-19.65)) ;
#146026=CARTESIAN_POINT('Origin',(7.9,2.1,-19.65)) ;
#146027=CARTESIAN_POINT('Origin',(1.4,2.,-19.65)) ;
#146028=CARTESIAN_POINT('',(1.5,2.,-20.6)) ;
#146029=CARTESIAN_POINT('',(1.5,2.,-20.6)) ;
#146030=CARTESIAN_POINT('',(7.9,2.,-20.6)) ;
#146031=CARTESIAN_POINT('',(1.4,2.,-20.6)) ;
#146032=CARTESIAN_POINT('',(7.9,2.,-19.65)) ;
#146033=CARTESIAN_POINT('Origin',(1.4,1.9,-20.6)) ;
#146034=CARTESIAN_POINT('',(1.5,1.9,-20.7)) ;
#146035=CARTESIAN_POINT('Origin',(1.5,1.9,-20.6)) ;
#146036=CARTESIAN_POINT('',(7.9,1.9,-20.7)) ;
#146037=CARTESIAN_POINT('',(1.4,1.9,-20.7)) ;
#146038=CARTESIAN_POINT('Origin',(7.9,1.9,-20.6)) ;
#146039=CARTESIAN_POINT('Origin',(1.4,1.9,-20.7)) ;
#146040=CARTESIAN_POINT('',(1.5,-2.15,-20.7)) ;
#146041=CARTESIAN_POINT('',(1.5,-2.15,-20.7)) ;
#146042=CARTESIAN_POINT('',(7.9,-2.15,-20.7)) ;
#146043=CARTESIAN_POINT('',(1.4,-2.15,-20.7)) ;
#146044=CARTESIAN_POINT('',(7.9,1.9,-20.7)) ;
#146045=CARTESIAN_POINT('Origin',(1.4,-2.15,-20.6)) ;
#146046=CARTESIAN_POINT('',(1.5,-2.25,-20.6)) ;
#146047=CARTESIAN_POINT('Origin',(1.5,-2.15,-20.6)) ;
#146048=CARTESIAN_POINT('',(7.9,-2.25,-20.6)) ;
#146049=CARTESIAN_POINT('',(1.4,-2.25,-20.6)) ;
#146050=CARTESIAN_POINT('Origin',(7.9,-2.15,-20.6)) ;
#146051=CARTESIAN_POINT('Origin',(1.4,-2.25,-19.9531195934094)) ;
#146052=CARTESIAN_POINT('',(1.5,-2.25,-19.9531195934094)) ;
#146053=CARTESIAN_POINT('',(1.5,-2.25,-19.9531195934094)) ;
#146054=CARTESIAN_POINT('',(7.9,-2.25,-19.9531195934094)) ;
#146055=CARTESIAN_POINT('',(1.4,-2.25,-19.9531195934094)) ;
#146056=CARTESIAN_POINT('',(7.9,-2.25,-20.6)) ;
#146057=CARTESIAN_POINT('Origin',(1.4,-2.15,-19.9531195934094)) ;
#146058=CARTESIAN_POINT('',(1.5,-2.23576512455516,-19.9016964137135)) ;
#146059=CARTESIAN_POINT('Origin',(1.5,-2.15,-19.9531195934094)) ;
#146060=CARTESIAN_POINT('',(7.9,-2.23576512455516,-19.9016964137135)) ;
#146061=CARTESIAN_POINT('',(1.4,-2.23576512455516,-19.9016964137135)) ;
#146062=CARTESIAN_POINT('Origin',(7.9,-2.15,-19.9531195934094)) ;
#146063=CARTESIAN_POINT('Origin',(1.4,-3.65625,-19.05)) ;
#146064=CARTESIAN_POINT('',(1.5,-2.23576512455516,-18.1983035862865)) ;
#146065=CARTESIAN_POINT('Origin',(1.5,-3.65625,-19.05)) ;
#146066=CARTESIAN_POINT('',(7.9,-2.23576512455516,-18.1983035862865)) ;
#146067=CARTESIAN_POINT('',(1.4,-2.23576512455516,-18.1983035862865)) ;
#146068=CARTESIAN_POINT('Origin',(7.9,-3.65625,-19.05)) ;
#146069=CARTESIAN_POINT('Origin',(1.4,-2.15,-18.1468804065906)) ;
#146070=CARTESIAN_POINT('',(1.5,-2.25,-18.1468804065906)) ;
#146071=CARTESIAN_POINT('Origin',(1.5,-2.15,-18.1468804065906)) ;
#146072=CARTESIAN_POINT('',(7.9,-2.25,-18.1468804065906)) ;
#146073=CARTESIAN_POINT('',(1.4,-2.25,-18.1468804065906)) ;
#146074=CARTESIAN_POINT('Origin',(7.9,-2.15,-18.1468804065906)) ;
#146075=CARTESIAN_POINT('Origin',(1.4,-2.25,-17.5)) ;
#146076=CARTESIAN_POINT('',(1.5,-2.25,-17.5)) ;
#146077=CARTESIAN_POINT('',(1.5,-2.25,-17.5)) ;
#146078=CARTESIAN_POINT('',(7.9,-2.25,-17.5)) ;
#146079=CARTESIAN_POINT('',(1.4,-2.25,-17.5)) ;
#146080=CARTESIAN_POINT('',(7.9,-2.25,-18.1468804065906)) ;
#146081=CARTESIAN_POINT('Origin',(1.4,-2.15,-17.5)) ;
#146082=CARTESIAN_POINT('',(1.5,-2.15,-17.4)) ;
#146083=CARTESIAN_POINT('Origin',(1.5,-2.15,-17.5)) ;
#146084=CARTESIAN_POINT('',(7.9,-2.15,-17.4)) ;
#146085=CARTESIAN_POINT('',(1.4,-2.15,-17.4)) ;
#146086=CARTESIAN_POINT('Origin',(7.9,-2.15,-17.5)) ;
#146087=CARTESIAN_POINT('Origin',(1.4,1.9,-17.4)) ;
#146088=CARTESIAN_POINT('',(1.5,1.9,-17.4)) ;
#146089=CARTESIAN_POINT('',(1.5,1.9,-17.4)) ;
#146090=CARTESIAN_POINT('',(7.9,1.9,-17.4)) ;
#146091=CARTESIAN_POINT('',(1.4,1.9,-17.4)) ;
#146092=CARTESIAN_POINT('',(7.9,-2.15,-17.4)) ;
#146093=CARTESIAN_POINT('Origin',(1.4,1.9,-17.5)) ;
#146094=CARTESIAN_POINT('',(1.5,2.,-17.5)) ;
#146095=CARTESIAN_POINT('Origin',(1.5,1.9,-17.5)) ;
#146096=CARTESIAN_POINT('',(7.9,2.,-17.5)) ;
#146097=CARTESIAN_POINT('',(1.4,2.,-17.5)) ;
#146098=CARTESIAN_POINT('Origin',(7.9,1.9,-17.5)) ;
#146099=CARTESIAN_POINT('Origin',(1.4,2.,-17.5)) ;
#146100=CARTESIAN_POINT('',(1.5,2.,-18.45)) ;
#146101=CARTESIAN_POINT('',(7.9,2.,-17.5)) ;
#146102=CARTESIAN_POINT('Origin',(1.4,2.1,-18.45)) ;
#146103=CARTESIAN_POINT('',(1.4,2.6,-18.45)) ;
#146104=CARTESIAN_POINT('',(1.4,2.4,-18.65)) ;
#146105=CARTESIAN_POINT('Origin',(1.4,2.4,-18.45)) ;
#146106=CARTESIAN_POINT('',(1.4,2.1,-18.65)) ;
#146107=CARTESIAN_POINT('',(1.4,2.1,-18.65)) ;
#146108=CARTESIAN_POINT('',(1.4,1.9,-18.45)) ;
#146109=CARTESIAN_POINT('Origin',(1.4,2.1,-18.45)) ;
#146110=CARTESIAN_POINT('',(1.4,1.9,-17.5)) ;
#146111=CARTESIAN_POINT('',(1.4,1.9,-17.5)) ;
#146112=CARTESIAN_POINT('',(1.4,-2.15,-17.5)) ;
#146113=CARTESIAN_POINT('',(1.4,-2.15,-17.5)) ;
#146114=CARTESIAN_POINT('',(1.4,-2.15,-18.1468804065906)) ;
#146115=CARTESIAN_POINT('',(1.4,-2.15,-18.1468804065906)) ;
#146116=CARTESIAN_POINT('',(1.4,-2.15,-19.9531195934094)) ;
#146117=CARTESIAN_POINT('Origin',(1.4,-3.65625,-19.05)) ;
#146118=CARTESIAN_POINT('',(1.4,-2.15,-20.6)) ;
#146119=CARTESIAN_POINT('',(1.4,-2.15,-20.6)) ;
#146120=CARTESIAN_POINT('',(1.4,1.9,-20.6)) ;
#146121=CARTESIAN_POINT('',(1.4,1.9,-20.6)) ;
#146122=CARTESIAN_POINT('',(1.4,1.9,-19.65)) ;
#146123=CARTESIAN_POINT('',(1.4,1.9,-19.65)) ;
#146124=CARTESIAN_POINT('',(1.4,2.1,-19.45)) ;
#146125=CARTESIAN_POINT('Origin',(1.4,2.1,-19.65)) ;
#146126=CARTESIAN_POINT('',(1.4,2.4,-19.45)) ;
#146127=CARTESIAN_POINT('',(1.4,2.4,-19.45)) ;
#146128=CARTESIAN_POINT('',(1.4,2.6,-19.65)) ;
#146129=CARTESIAN_POINT('Origin',(1.4,2.4,-19.65)) ;
#146130=CARTESIAN_POINT('',(1.4,2.6,-19.7585786437627)) ;
#146131=CARTESIAN_POINT('',(1.4,2.6,-19.7585786437627)) ;
#146132=CARTESIAN_POINT('',(1.4,3.15,-20.3085786437627)) ;
#146133=CARTESIAN_POINT('',(1.4,3.15,-20.3085786437627)) ;
#146134=CARTESIAN_POINT('',(1.4,3.15,-17.7914213562373)) ;
#146135=CARTESIAN_POINT('',(1.4,2.6,-18.3414213562373)) ;
#146136=CARTESIAN_POINT('',(1.4,2.6,-18.3414213562373)) ;
#146137=CARTESIAN_POINT('',(1.4,2.6,-18.45)) ;
#146138=CARTESIAN_POINT('Origin',(1.4,2.1,-14.64)) ;
#146139=CARTESIAN_POINT('',(1.5,2.,-14.64)) ;
#146140=CARTESIAN_POINT('',(7.9,2.,-14.64)) ;
#146141=CARTESIAN_POINT('',(1.4,2.,-14.64)) ;
#146142=CARTESIAN_POINT('',(1.5,2.1,-14.74)) ;
#146143=CARTESIAN_POINT('Origin',(1.5,2.1,-14.64)) ;
#146144=CARTESIAN_POINT('',(7.9,2.1,-14.74)) ;
#146145=CARTESIAN_POINT('',(1.4,2.1,-14.74)) ;
#146146=CARTESIAN_POINT('Origin',(7.9,2.1,-14.64)) ;
#146147=CARTESIAN_POINT('Origin',(1.4,2.4,-14.74)) ;
#146148=CARTESIAN_POINT('',(1.5,2.4,-14.74)) ;
#146149=CARTESIAN_POINT('',(1.5,2.4,-14.74)) ;
#146150=CARTESIAN_POINT('',(7.9,2.4,-14.74)) ;
#146151=CARTESIAN_POINT('',(1.4,2.4,-14.74)) ;
#146152=CARTESIAN_POINT('',(7.9,2.1,-14.74)) ;
#146153=CARTESIAN_POINT('Origin',(1.4,2.4,-14.64)) ;
#146154=CARTESIAN_POINT('',(1.5,2.5,-14.64)) ;
#146155=CARTESIAN_POINT('Origin',(1.5,2.4,-14.64)) ;
#146156=CARTESIAN_POINT('',(7.9,2.5,-14.64)) ;
#146157=CARTESIAN_POINT('',(1.4,2.5,-14.64)) ;
#146158=CARTESIAN_POINT('Origin',(7.9,2.4,-14.64)) ;
#146159=CARTESIAN_POINT('Origin',(1.4,2.5,-14.5314213562373)) ;
#146160=CARTESIAN_POINT('',(1.5,2.5,-14.5314213562373)) ;
#146161=CARTESIAN_POINT('',(1.5,2.5,-14.5314213562373)) ;
#146162=CARTESIAN_POINT('',(7.9,2.5,-14.5314213562373)) ;
#146163=CARTESIAN_POINT('',(1.4,2.5,-14.5314213562373)) ;
#146164=CARTESIAN_POINT('',(7.9,2.5,-14.64)) ;
#146165=CARTESIAN_POINT('Origin',(1.4,2.6,-14.5314213562373)) ;
#146166=CARTESIAN_POINT('',(1.5,2.52928932188135,-14.4607106781187)) ;
#146167=CARTESIAN_POINT('Origin',(1.5,2.6,-14.5314213562373)) ;
#146168=CARTESIAN_POINT('',(7.9,2.52928932188135,-14.4607106781187)) ;
#146169=CARTESIAN_POINT('',(1.4,2.52928932188135,-14.4607106781187)) ;
#146170=CARTESIAN_POINT('Origin',(7.9,2.6,-14.5314213562373)) ;
#146171=CARTESIAN_POINT('Origin',(1.4,3.07928932188135,-13.9107106781187)) ;
#146172=CARTESIAN_POINT('',(1.5,3.07928932188135,-13.9107106781187)) ;
#146173=CARTESIAN_POINT('',(7.9,3.07928932188135,-13.9107106781187)) ;
#146174=CARTESIAN_POINT('',(1.4,3.07928932188135,-13.9107106781187)) ;
#146175=CARTESIAN_POINT('',(7.9,2.52928932188135,-14.4607106781187)) ;
#146176=CARTESIAN_POINT('Origin',(1.4,3.15,-13.9814213562373)) ;
#146177=CARTESIAN_POINT('',(7.9,3.25,-13.9814213562373)) ;
#146178=CARTESIAN_POINT('',(1.4,3.25,-13.9814213562373)) ;
#146179=CARTESIAN_POINT('Origin',(7.9,3.15,-13.9814213562373)) ;
#146180=CARTESIAN_POINT('Origin',(1.4,3.25,-16.4985786437627)) ;
#146181=CARTESIAN_POINT('',(1.5,3.25,-16.4985786437627)) ;
#146182=CARTESIAN_POINT('',(7.9,3.25,-13.9814213562373)) ;
#146183=CARTESIAN_POINT('Origin',(1.4,2.52928932188134,-16.0192893218813)) ;
#146184=CARTESIAN_POINT('',(1.5,2.52928932188134,-16.0192893218813)) ;
#146185=CARTESIAN_POINT('',(1.5,2.52928932188135,-16.0192893218813)) ;
#146186=CARTESIAN_POINT('',(7.9,2.52928932188134,-16.0192893218813)) ;
#146187=CARTESIAN_POINT('',(1.4,2.52928932188134,-16.0192893218813)) ;
#146188=CARTESIAN_POINT('',(7.9,3.07928932188134,-16.5692893218813)) ;
#146189=CARTESIAN_POINT('Origin',(1.4,2.6,-15.9485786437627)) ;
#146190=CARTESIAN_POINT('',(1.5,2.5,-15.9485786437627)) ;
#146191=CARTESIAN_POINT('Origin',(1.5,2.6,-15.9485786437627)) ;
#146192=CARTESIAN_POINT('',(7.9,2.5,-15.9485786437627)) ;
#146193=CARTESIAN_POINT('',(1.4,2.5,-15.9485786437627)) ;
#146194=CARTESIAN_POINT('Origin',(7.9,2.6,-15.9485786437627)) ;
#146195=CARTESIAN_POINT('Origin',(1.4,2.5,-15.84)) ;
#146196=CARTESIAN_POINT('',(1.5,2.5,-15.84)) ;
#146197=CARTESIAN_POINT('',(1.5,2.5,-15.84)) ;
#146198=CARTESIAN_POINT('',(7.9,2.5,-15.84)) ;
#146199=CARTESIAN_POINT('',(1.4,2.5,-15.84)) ;
#146200=CARTESIAN_POINT('',(7.9,2.5,-15.9485786437627)) ;
#146201=CARTESIAN_POINT('Origin',(1.4,2.4,-15.84)) ;
#146202=CARTESIAN_POINT('',(1.5,2.4,-15.74)) ;
#146203=CARTESIAN_POINT('Origin',(1.5,2.4,-15.84)) ;
#146204=CARTESIAN_POINT('',(7.9,2.4,-15.74)) ;
#146205=CARTESIAN_POINT('',(1.4,2.4,-15.74)) ;
#146206=CARTESIAN_POINT('Origin',(7.9,2.4,-15.84)) ;
#146207=CARTESIAN_POINT('Origin',(1.4,2.1,-15.74)) ;
#146208=CARTESIAN_POINT('',(1.5,2.1,-15.74)) ;
#146209=CARTESIAN_POINT('',(1.5,2.1,-15.74)) ;
#146210=CARTESIAN_POINT('',(7.9,2.1,-15.74)) ;
#146211=CARTESIAN_POINT('',(1.4,2.1,-15.74)) ;
#146212=CARTESIAN_POINT('',(7.9,2.4,-15.74)) ;
#146213=CARTESIAN_POINT('Origin',(1.4,2.1,-15.84)) ;
#146214=CARTESIAN_POINT('',(1.5,2.,-15.84)) ;
#146215=CARTESIAN_POINT('Origin',(1.5,2.1,-15.84)) ;
#146216=CARTESIAN_POINT('',(7.9,2.,-15.84)) ;
#146217=CARTESIAN_POINT('',(1.4,2.,-15.84)) ;
#146218=CARTESIAN_POINT('Origin',(7.9,2.1,-15.84)) ;
#146219=CARTESIAN_POINT('Origin',(1.4,2.,-15.84)) ;
#146220=CARTESIAN_POINT('',(1.5,2.,-16.79)) ;
#146221=CARTESIAN_POINT('',(1.5,2.,-16.79)) ;
#146222=CARTESIAN_POINT('',(7.9,2.,-16.79)) ;
#146223=CARTESIAN_POINT('',(1.4,2.,-16.79)) ;
#146224=CARTESIAN_POINT('',(7.9,2.,-15.84)) ;
#146225=CARTESIAN_POINT('Origin',(1.4,1.9,-16.79)) ;
#146226=CARTESIAN_POINT('',(1.5,1.9,-16.89)) ;
#146227=CARTESIAN_POINT('Origin',(1.5,1.9,-16.79)) ;
#146228=CARTESIAN_POINT('',(7.9,1.9,-16.89)) ;
#146229=CARTESIAN_POINT('',(1.4,1.9,-16.89)) ;
#146230=CARTESIAN_POINT('Origin',(7.9,1.9,-16.79)) ;
#146231=CARTESIAN_POINT('Origin',(1.4,1.9,-16.89)) ;
#146232=CARTESIAN_POINT('',(1.5,-2.15,-16.89)) ;
#146233=CARTESIAN_POINT('',(1.5,-2.15,-16.89)) ;
#146234=CARTESIAN_POINT('',(7.9,-2.15,-16.89)) ;
#146235=CARTESIAN_POINT('',(1.4,-2.15,-16.89)) ;
#146236=CARTESIAN_POINT('',(7.9,1.9,-16.89)) ;
#146237=CARTESIAN_POINT('Origin',(1.4,-2.15,-16.79)) ;
#146238=CARTESIAN_POINT('',(1.5,-2.25,-16.79)) ;
#146239=CARTESIAN_POINT('Origin',(1.5,-2.15,-16.79)) ;
#146240=CARTESIAN_POINT('',(7.9,-2.25,-16.79)) ;
#146241=CARTESIAN_POINT('',(1.4,-2.25,-16.79)) ;
#146242=CARTESIAN_POINT('Origin',(7.9,-2.15,-16.79)) ;
#146243=CARTESIAN_POINT('Origin',(1.4,-2.25,-16.1431195934094)) ;
#146244=CARTESIAN_POINT('',(1.5,-2.25,-16.1431195934094)) ;
#146245=CARTESIAN_POINT('',(1.5,-2.25,-16.1431195934094)) ;
#146246=CARTESIAN_POINT('',(7.9,-2.25,-16.1431195934094)) ;
#146247=CARTESIAN_POINT('',(1.4,-2.25,-16.1431195934094)) ;
#146248=CARTESIAN_POINT('',(7.9,-2.25,-16.79)) ;
#146249=CARTESIAN_POINT('Origin',(1.4,-2.15,-16.1431195934094)) ;
#146250=CARTESIAN_POINT('',(1.5,-2.23576512455516,-16.0916964137135)) ;
#146251=CARTESIAN_POINT('Origin',(1.5,-2.15,-16.1431195934094)) ;
#146252=CARTESIAN_POINT('',(7.9,-2.23576512455516,-16.0916964137135)) ;
#146253=CARTESIAN_POINT('',(1.4,-2.23576512455516,-16.0916964137135)) ;
#146254=CARTESIAN_POINT('Origin',(7.9,-2.15,-16.1431195934094)) ;
#146255=CARTESIAN_POINT('Origin',(1.4,-3.65625,-15.24)) ;
#146256=CARTESIAN_POINT('',(1.5,-2.23576512455516,-14.3883035862865)) ;
#146257=CARTESIAN_POINT('Origin',(1.5,-3.65625,-15.24)) ;
#146258=CARTESIAN_POINT('',(7.9,-2.23576512455516,-14.3883035862865)) ;
#146259=CARTESIAN_POINT('',(1.4,-2.23576512455516,-14.3883035862865)) ;
#146260=CARTESIAN_POINT('Origin',(7.9,-3.65625,-15.24)) ;
#146261=CARTESIAN_POINT('Origin',(1.4,-2.15,-14.3368804065906)) ;
#146262=CARTESIAN_POINT('',(1.5,-2.25,-14.3368804065906)) ;
#146263=CARTESIAN_POINT('Origin',(1.5,-2.15,-14.3368804065906)) ;
#146264=CARTESIAN_POINT('',(7.9,-2.25,-14.3368804065906)) ;
#146265=CARTESIAN_POINT('',(1.4,-2.25,-14.3368804065906)) ;
#146266=CARTESIAN_POINT('Origin',(7.9,-2.15,-14.3368804065906)) ;
#146267=CARTESIAN_POINT('Origin',(1.4,-2.25,-13.69)) ;
#146268=CARTESIAN_POINT('',(1.5,-2.25,-13.69)) ;
#146269=CARTESIAN_POINT('',(1.5,-2.25,-13.69)) ;
#146270=CARTESIAN_POINT('',(7.9,-2.25,-13.69)) ;
#146271=CARTESIAN_POINT('',(1.4,-2.25,-13.69)) ;
#146272=CARTESIAN_POINT('',(7.9,-2.25,-14.3368804065906)) ;
#146273=CARTESIAN_POINT('Origin',(1.4,-2.15,-13.69)) ;
#146274=CARTESIAN_POINT('',(1.5,-2.15,-13.59)) ;
#146275=CARTESIAN_POINT('Origin',(1.5,-2.15,-13.69)) ;
#146276=CARTESIAN_POINT('',(7.9,-2.15,-13.59)) ;
#146277=CARTESIAN_POINT('',(1.4,-2.15,-13.59)) ;
#146278=CARTESIAN_POINT('Origin',(7.9,-2.15,-13.69)) ;
#146279=CARTESIAN_POINT('Origin',(1.4,1.9,-13.59)) ;
#146280=CARTESIAN_POINT('',(1.5,1.9,-13.59)) ;
#146281=CARTESIAN_POINT('',(1.5,1.9,-13.59)) ;
#146282=CARTESIAN_POINT('',(7.9,1.9,-13.59)) ;
#146283=CARTESIAN_POINT('',(1.4,1.9,-13.59)) ;
#146284=CARTESIAN_POINT('',(7.9,-2.15,-13.59)) ;
#146285=CARTESIAN_POINT('Origin',(1.4,1.9,-13.69)) ;
#146286=CARTESIAN_POINT('',(1.5,2.,-13.69)) ;
#146287=CARTESIAN_POINT('Origin',(1.5,1.9,-13.69)) ;
#146288=CARTESIAN_POINT('',(7.9,2.,-13.69)) ;
#146289=CARTESIAN_POINT('',(1.4,2.,-13.69)) ;
#146290=CARTESIAN_POINT('Origin',(7.9,1.9,-13.69)) ;
#146291=CARTESIAN_POINT('Origin',(1.4,2.,-13.69)) ;
#146292=CARTESIAN_POINT('',(1.5,2.,-14.64)) ;
#146293=CARTESIAN_POINT('',(7.9,2.,-13.69)) ;
#146294=CARTESIAN_POINT('Origin',(1.4,2.1,-14.64)) ;
#146295=CARTESIAN_POINT('',(1.4,2.6,-14.64)) ;
#146296=CARTESIAN_POINT('',(1.4,2.4,-14.84)) ;
#146297=CARTESIAN_POINT('Origin',(1.4,2.4,-14.64)) ;
#146298=CARTESIAN_POINT('',(1.4,2.1,-14.84)) ;
#146299=CARTESIAN_POINT('',(1.4,2.1,-14.84)) ;
#146300=CARTESIAN_POINT('',(1.4,1.9,-14.64)) ;
#146301=CARTESIAN_POINT('Origin',(1.4,2.1,-14.64)) ;
#146302=CARTESIAN_POINT('',(1.4,1.9,-13.69)) ;
#146303=CARTESIAN_POINT('',(1.4,1.9,-13.69)) ;
#146304=CARTESIAN_POINT('',(1.4,-2.15,-13.69)) ;
#146305=CARTESIAN_POINT('',(1.4,-2.15,-13.69)) ;
#146306=CARTESIAN_POINT('',(1.4,-2.15,-14.3368804065906)) ;
#146307=CARTESIAN_POINT('',(1.4,-2.15,-14.3368804065906)) ;
#146308=CARTESIAN_POINT('',(1.4,-2.15,-16.1431195934094)) ;
#146309=CARTESIAN_POINT('Origin',(1.4,-3.65625,-15.24)) ;
#146310=CARTESIAN_POINT('',(1.4,-2.15,-16.79)) ;
#146311=CARTESIAN_POINT('',(1.4,-2.15,-16.79)) ;
#146312=CARTESIAN_POINT('',(1.4,1.9,-16.79)) ;
#146313=CARTESIAN_POINT('',(1.4,1.9,-16.79)) ;
#146314=CARTESIAN_POINT('',(1.4,1.9,-15.84)) ;
#146315=CARTESIAN_POINT('',(1.4,1.9,-15.84)) ;
#146316=CARTESIAN_POINT('',(1.4,2.1,-15.64)) ;
#146317=CARTESIAN_POINT('Origin',(1.4,2.1,-15.84)) ;
#146318=CARTESIAN_POINT('',(1.4,2.4,-15.64)) ;
#146319=CARTESIAN_POINT('',(1.4,2.4,-15.64)) ;
#146320=CARTESIAN_POINT('',(1.4,2.6,-15.84)) ;
#146321=CARTESIAN_POINT('Origin',(1.4,2.4,-15.84)) ;
#146322=CARTESIAN_POINT('',(1.4,2.6,-15.9485786437627)) ;
#146323=CARTESIAN_POINT('',(1.4,2.6,-15.9485786437627)) ;
#146324=CARTESIAN_POINT('',(1.4,3.15,-16.4985786437627)) ;
#146325=CARTESIAN_POINT('',(1.4,3.15,-16.4985786437627)) ;
#146326=CARTESIAN_POINT('',(1.4,3.15,-13.9814213562373)) ;
#146327=CARTESIAN_POINT('',(1.4,2.6,-14.5314213562373)) ;
#146328=CARTESIAN_POINT('',(1.4,2.6,-14.5314213562373)) ;
#146329=CARTESIAN_POINT('',(1.4,2.6,-14.64)) ;
#146330=CARTESIAN_POINT('Origin',(1.4,2.1,-10.83)) ;
#146331=CARTESIAN_POINT('',(1.5,2.,-10.83)) ;
#146332=CARTESIAN_POINT('',(7.9,2.,-10.83)) ;
#146333=CARTESIAN_POINT('',(1.4,2.,-10.83)) ;
#146334=CARTESIAN_POINT('',(1.5,2.1,-10.93)) ;
#146335=CARTESIAN_POINT('Origin',(1.5,2.1,-10.83)) ;
#146336=CARTESIAN_POINT('',(7.9,2.1,-10.93)) ;
#146337=CARTESIAN_POINT('',(1.4,2.1,-10.93)) ;
#146338=CARTESIAN_POINT('Origin',(7.9,2.1,-10.83)) ;
#146339=CARTESIAN_POINT('Origin',(1.4,2.4,-10.93)) ;
#146340=CARTESIAN_POINT('',(1.5,2.4,-10.93)) ;
#146341=CARTESIAN_POINT('',(1.5,2.4,-10.93)) ;
#146342=CARTESIAN_POINT('',(7.9,2.4,-10.93)) ;
#146343=CARTESIAN_POINT('',(1.4,2.4,-10.93)) ;
#146344=CARTESIAN_POINT('',(7.9,2.1,-10.93)) ;
#146345=CARTESIAN_POINT('Origin',(1.4,2.4,-10.83)) ;
#146346=CARTESIAN_POINT('',(1.5,2.5,-10.83)) ;
#146347=CARTESIAN_POINT('Origin',(1.5,2.4,-10.83)) ;
#146348=CARTESIAN_POINT('',(7.9,2.5,-10.83)) ;
#146349=CARTESIAN_POINT('',(1.4,2.5,-10.83)) ;
#146350=CARTESIAN_POINT('Origin',(7.9,2.4,-10.83)) ;
#146351=CARTESIAN_POINT('Origin',(1.4,2.5,-10.7214213562373)) ;
#146352=CARTESIAN_POINT('',(1.5,2.5,-10.7214213562373)) ;
#146353=CARTESIAN_POINT('',(1.5,2.5,-10.7214213562373)) ;
#146354=CARTESIAN_POINT('',(7.9,2.5,-10.7214213562373)) ;
#146355=CARTESIAN_POINT('',(1.4,2.5,-10.7214213562373)) ;
#146356=CARTESIAN_POINT('',(7.9,2.5,-10.83)) ;
#146357=CARTESIAN_POINT('Origin',(1.4,2.6,-10.7214213562373)) ;
#146358=CARTESIAN_POINT('',(1.5,2.52928932188135,-10.6507106781187)) ;
#146359=CARTESIAN_POINT('Origin',(1.5,2.6,-10.7214213562373)) ;
#146360=CARTESIAN_POINT('',(7.9,2.52928932188135,-10.6507106781187)) ;
#146361=CARTESIAN_POINT('',(1.4,2.52928932188135,-10.6507106781187)) ;
#146362=CARTESIAN_POINT('Origin',(7.9,2.6,-10.7214213562373)) ;
#146363=CARTESIAN_POINT('Origin',(1.4,3.07928932188135,-10.1007106781187)) ;
#146364=CARTESIAN_POINT('',(1.5,3.07928932188135,-10.1007106781187)) ;
#146365=CARTESIAN_POINT('',(7.9,3.07928932188135,-10.1007106781187)) ;
#146366=CARTESIAN_POINT('',(1.4,3.07928932188135,-10.1007106781187)) ;
#146367=CARTESIAN_POINT('',(7.9,2.52928932188135,-10.6507106781187)) ;
#146368=CARTESIAN_POINT('Origin',(1.4,3.15,-10.1714213562373)) ;
#146369=CARTESIAN_POINT('',(7.9,3.25,-10.1714213562373)) ;
#146370=CARTESIAN_POINT('',(1.4,3.25,-10.1714213562373)) ;
#146371=CARTESIAN_POINT('Origin',(7.9,3.15,-10.1714213562373)) ;
#146372=CARTESIAN_POINT('Origin',(1.4,3.25,-12.6885786437627)) ;
#146373=CARTESIAN_POINT('',(1.5,3.25,-12.6885786437627)) ;
#146374=CARTESIAN_POINT('',(7.9,3.25,-10.1714213562373)) ;
#146375=CARTESIAN_POINT('Origin',(1.4,2.52928932188134,-12.2092893218813)) ;
#146376=CARTESIAN_POINT('',(1.5,2.52928932188134,-12.2092893218813)) ;
#146377=CARTESIAN_POINT('',(1.5,2.52928932188134,-12.2092893218813)) ;
#146378=CARTESIAN_POINT('',(7.9,2.52928932188134,-12.2092893218813)) ;
#146379=CARTESIAN_POINT('',(1.4,2.52928932188134,-12.2092893218813)) ;
#146380=CARTESIAN_POINT('',(7.9,3.07928932188135,-12.7592893218813)) ;
#146381=CARTESIAN_POINT('Origin',(1.4,2.6,-12.1385786437627)) ;
#146382=CARTESIAN_POINT('',(1.5,2.5,-12.1385786437627)) ;
#146383=CARTESIAN_POINT('Origin',(1.5,2.6,-12.1385786437627)) ;
#146384=CARTESIAN_POINT('',(7.9,2.5,-12.1385786437627)) ;
#146385=CARTESIAN_POINT('',(1.4,2.5,-12.1385786437627)) ;
#146386=CARTESIAN_POINT('Origin',(7.9,2.6,-12.1385786437627)) ;
#146387=CARTESIAN_POINT('Origin',(1.4,2.5,-12.03)) ;
#146388=CARTESIAN_POINT('',(1.5,2.5,-12.03)) ;
#146389=CARTESIAN_POINT('',(1.5,2.5,-12.03)) ;
#146390=CARTESIAN_POINT('',(7.9,2.5,-12.03)) ;
#146391=CARTESIAN_POINT('',(1.4,2.5,-12.03)) ;
#146392=CARTESIAN_POINT('',(7.9,2.5,-12.1385786437627)) ;
#146393=CARTESIAN_POINT('Origin',(1.4,2.4,-12.03)) ;
#146394=CARTESIAN_POINT('',(1.5,2.4,-11.93)) ;
#146395=CARTESIAN_POINT('Origin',(1.5,2.4,-12.03)) ;
#146396=CARTESIAN_POINT('',(7.9,2.4,-11.93)) ;
#146397=CARTESIAN_POINT('',(1.4,2.4,-11.93)) ;
#146398=CARTESIAN_POINT('Origin',(7.9,2.4,-12.03)) ;
#146399=CARTESIAN_POINT('Origin',(1.4,2.1,-11.93)) ;
#146400=CARTESIAN_POINT('',(1.5,2.1,-11.93)) ;
#146401=CARTESIAN_POINT('',(1.5,2.1,-11.93)) ;
#146402=CARTESIAN_POINT('',(7.9,2.1,-11.93)) ;
#146403=CARTESIAN_POINT('',(1.4,2.1,-11.93)) ;
#146404=CARTESIAN_POINT('',(7.9,2.4,-11.93)) ;
#146405=CARTESIAN_POINT('Origin',(1.4,2.1,-12.03)) ;
#146406=CARTESIAN_POINT('',(1.5,2.,-12.03)) ;
#146407=CARTESIAN_POINT('Origin',(1.5,2.1,-12.03)) ;
#146408=CARTESIAN_POINT('',(7.9,2.,-12.03)) ;
#146409=CARTESIAN_POINT('',(1.4,2.,-12.03)) ;
#146410=CARTESIAN_POINT('Origin',(7.9,2.1,-12.03)) ;
#146411=CARTESIAN_POINT('Origin',(1.4,2.,-12.03)) ;
#146412=CARTESIAN_POINT('',(1.5,2.,-12.98)) ;
#146413=CARTESIAN_POINT('',(1.5,2.,-12.98)) ;
#146414=CARTESIAN_POINT('',(7.9,2.,-12.98)) ;
#146415=CARTESIAN_POINT('',(1.4,2.,-12.98)) ;
#146416=CARTESIAN_POINT('',(7.9,2.,-12.03)) ;
#146417=CARTESIAN_POINT('Origin',(1.4,1.9,-12.98)) ;
#146418=CARTESIAN_POINT('',(1.5,1.9,-13.08)) ;
#146419=CARTESIAN_POINT('Origin',(1.5,1.9,-12.98)) ;
#146420=CARTESIAN_POINT('',(7.9,1.9,-13.08)) ;
#146421=CARTESIAN_POINT('',(1.4,1.9,-13.08)) ;
#146422=CARTESIAN_POINT('Origin',(7.9,1.9,-12.98)) ;
#146423=CARTESIAN_POINT('Origin',(1.4,1.9,-13.08)) ;
#146424=CARTESIAN_POINT('',(1.5,-2.15,-13.08)) ;
#146425=CARTESIAN_POINT('',(1.5,-2.15,-13.08)) ;
#146426=CARTESIAN_POINT('',(7.9,-2.15,-13.08)) ;
#146427=CARTESIAN_POINT('',(1.4,-2.15,-13.08)) ;
#146428=CARTESIAN_POINT('',(7.9,1.9,-13.08)) ;
#146429=CARTESIAN_POINT('Origin',(1.4,-2.15,-12.98)) ;
#146430=CARTESIAN_POINT('',(1.5,-2.25,-12.98)) ;
#146431=CARTESIAN_POINT('Origin',(1.5,-2.15,-12.98)) ;
#146432=CARTESIAN_POINT('',(7.9,-2.25,-12.98)) ;
#146433=CARTESIAN_POINT('',(1.4,-2.25,-12.98)) ;
#146434=CARTESIAN_POINT('Origin',(7.9,-2.15,-12.98)) ;
#146435=CARTESIAN_POINT('Origin',(1.4,-2.25,-12.3331195934094)) ;
#146436=CARTESIAN_POINT('',(1.5,-2.25,-12.3331195934094)) ;
#146437=CARTESIAN_POINT('',(1.5,-2.25,-12.3331195934094)) ;
#146438=CARTESIAN_POINT('',(7.9,-2.25,-12.3331195934094)) ;
#146439=CARTESIAN_POINT('',(1.4,-2.25,-12.3331195934094)) ;
#146440=CARTESIAN_POINT('',(7.9,-2.25,-12.98)) ;
#146441=CARTESIAN_POINT('Origin',(1.4,-2.15,-12.3331195934094)) ;
#146442=CARTESIAN_POINT('',(1.5,-2.23576512455516,-12.2816964137135)) ;
#146443=CARTESIAN_POINT('Origin',(1.5,-2.15,-12.3331195934094)) ;
#146444=CARTESIAN_POINT('',(7.9,-2.23576512455516,-12.2816964137135)) ;
#146445=CARTESIAN_POINT('',(1.4,-2.23576512455516,-12.2816964137135)) ;
#146446=CARTESIAN_POINT('Origin',(7.9,-2.15,-12.3331195934094)) ;
#146447=CARTESIAN_POINT('Origin',(1.4,-3.65625,-11.43)) ;
#146448=CARTESIAN_POINT('',(1.5,-2.23576512455516,-10.5783035862865)) ;
#146449=CARTESIAN_POINT('Origin',(1.5,-3.65625,-11.43)) ;
#146450=CARTESIAN_POINT('',(7.9,-2.23576512455516,-10.5783035862865)) ;
#146451=CARTESIAN_POINT('',(1.4,-2.23576512455516,-10.5783035862865)) ;
#146452=CARTESIAN_POINT('Origin',(7.9,-3.65625,-11.43)) ;
#146453=CARTESIAN_POINT('Origin',(1.4,-2.15,-10.5268804065906)) ;
#146454=CARTESIAN_POINT('',(1.5,-2.25,-10.5268804065906)) ;
#146455=CARTESIAN_POINT('Origin',(1.5,-2.15,-10.5268804065906)) ;
#146456=CARTESIAN_POINT('',(7.9,-2.25,-10.5268804065906)) ;
#146457=CARTESIAN_POINT('',(1.4,-2.25,-10.5268804065906)) ;
#146458=CARTESIAN_POINT('Origin',(7.9,-2.15,-10.5268804065906)) ;
#146459=CARTESIAN_POINT('Origin',(1.4,-2.25,-9.88)) ;
#146460=CARTESIAN_POINT('',(1.5,-2.25,-9.88)) ;
#146461=CARTESIAN_POINT('',(1.5,-2.25,-9.88)) ;
#146462=CARTESIAN_POINT('',(7.9,-2.25,-9.88)) ;
#146463=CARTESIAN_POINT('',(1.4,-2.25,-9.88)) ;
#146464=CARTESIAN_POINT('',(7.9,-2.25,-10.5268804065906)) ;
#146465=CARTESIAN_POINT('Origin',(1.4,-2.15,-9.88)) ;
#146466=CARTESIAN_POINT('',(1.5,-2.15,-9.78)) ;
#146467=CARTESIAN_POINT('Origin',(1.5,-2.15,-9.88)) ;
#146468=CARTESIAN_POINT('',(7.9,-2.15,-9.78)) ;
#146469=CARTESIAN_POINT('',(1.4,-2.15,-9.78)) ;
#146470=CARTESIAN_POINT('Origin',(7.9,-2.15,-9.88)) ;
#146471=CARTESIAN_POINT('Origin',(1.4,1.9,-9.78)) ;
#146472=CARTESIAN_POINT('',(1.5,1.9,-9.78)) ;
#146473=CARTESIAN_POINT('',(1.5,1.9,-9.78)) ;
#146474=CARTESIAN_POINT('',(7.9,1.9,-9.78)) ;
#146475=CARTESIAN_POINT('',(1.4,1.9,-9.78)) ;
#146476=CARTESIAN_POINT('',(7.9,-2.15,-9.78)) ;
#146477=CARTESIAN_POINT('Origin',(1.4,1.9,-9.88)) ;
#146478=CARTESIAN_POINT('',(1.5,2.,-9.88)) ;
#146479=CARTESIAN_POINT('Origin',(1.5,1.9,-9.88)) ;
#146480=CARTESIAN_POINT('',(7.9,2.,-9.88)) ;
#146481=CARTESIAN_POINT('',(1.4,2.,-9.88)) ;
#146482=CARTESIAN_POINT('Origin',(7.9,1.9,-9.88)) ;
#146483=CARTESIAN_POINT('Origin',(1.4,2.,-9.88)) ;
#146484=CARTESIAN_POINT('',(1.5,2.,-10.83)) ;
#146485=CARTESIAN_POINT('',(7.9,2.,-9.88)) ;
#146486=CARTESIAN_POINT('Origin',(1.4,2.1,-10.83)) ;
#146487=CARTESIAN_POINT('',(1.4,2.6,-10.83)) ;
#146488=CARTESIAN_POINT('',(1.4,2.4,-11.03)) ;
#146489=CARTESIAN_POINT('Origin',(1.4,2.4,-10.83)) ;
#146490=CARTESIAN_POINT('',(1.4,2.1,-11.03)) ;
#146491=CARTESIAN_POINT('',(1.4,2.1,-11.03)) ;
#146492=CARTESIAN_POINT('',(1.4,1.9,-10.83)) ;
#146493=CARTESIAN_POINT('Origin',(1.4,2.1,-10.83)) ;
#146494=CARTESIAN_POINT('',(1.4,1.9,-9.88)) ;
#146495=CARTESIAN_POINT('',(1.4,1.9,-9.88)) ;
#146496=CARTESIAN_POINT('',(1.4,-2.15,-9.88)) ;
#146497=CARTESIAN_POINT('',(1.4,-2.15,-9.88)) ;
#146498=CARTESIAN_POINT('',(1.4,-2.15,-10.5268804065906)) ;
#146499=CARTESIAN_POINT('',(1.4,-2.15,-10.5268804065906)) ;
#146500=CARTESIAN_POINT('',(1.4,-2.15,-12.3331195934094)) ;
#146501=CARTESIAN_POINT('Origin',(1.4,-3.65625,-11.43)) ;
#146502=CARTESIAN_POINT('',(1.4,-2.15,-12.98)) ;
#146503=CARTESIAN_POINT('',(1.4,-2.15,-12.98)) ;
#146504=CARTESIAN_POINT('',(1.4,1.9,-12.98)) ;
#146505=CARTESIAN_POINT('',(1.4,1.9,-12.98)) ;
#146506=CARTESIAN_POINT('',(1.4,1.9,-12.03)) ;
#146507=CARTESIAN_POINT('',(1.4,1.9,-12.03)) ;
#146508=CARTESIAN_POINT('',(1.4,2.1,-11.83)) ;
#146509=CARTESIAN_POINT('Origin',(1.4,2.1,-12.03)) ;
#146510=CARTESIAN_POINT('',(1.4,2.4,-11.83)) ;
#146511=CARTESIAN_POINT('',(1.4,2.4,-11.83)) ;
#146512=CARTESIAN_POINT('',(1.4,2.6,-12.03)) ;
#146513=CARTESIAN_POINT('Origin',(1.4,2.4,-12.03)) ;
#146514=CARTESIAN_POINT('',(1.4,2.6,-12.1385786437627)) ;
#146515=CARTESIAN_POINT('',(1.4,2.6,-12.1385786437627)) ;
#146516=CARTESIAN_POINT('',(1.4,3.15,-12.6885786437627)) ;
#146517=CARTESIAN_POINT('',(1.4,3.15,-12.6885786437627)) ;
#146518=CARTESIAN_POINT('',(1.4,3.15,-10.1714213562373)) ;
#146519=CARTESIAN_POINT('',(1.4,2.6,-10.7214213562373)) ;
#146520=CARTESIAN_POINT('',(1.4,2.6,-10.7214213562373)) ;
#146521=CARTESIAN_POINT('',(1.4,2.6,-10.83)) ;
#146522=CARTESIAN_POINT('Origin',(1.4,2.1,-7.02)) ;
#146523=CARTESIAN_POINT('',(1.5,2.,-7.02)) ;
#146524=CARTESIAN_POINT('',(7.9,2.,-7.02)) ;
#146525=CARTESIAN_POINT('',(1.4,2.,-7.02)) ;
#146526=CARTESIAN_POINT('',(1.5,2.1,-7.12)) ;
#146527=CARTESIAN_POINT('Origin',(1.5,2.1,-7.02)) ;
#146528=CARTESIAN_POINT('',(7.9,2.1,-7.12)) ;
#146529=CARTESIAN_POINT('',(1.4,2.1,-7.12)) ;
#146530=CARTESIAN_POINT('Origin',(7.9,2.1,-7.02)) ;
#146531=CARTESIAN_POINT('Origin',(1.4,2.4,-7.12)) ;
#146532=CARTESIAN_POINT('',(1.5,2.4,-7.12)) ;
#146533=CARTESIAN_POINT('',(1.5,2.4,-7.12)) ;
#146534=CARTESIAN_POINT('',(7.9,2.4,-7.12)) ;
#146535=CARTESIAN_POINT('',(1.4,2.4,-7.12)) ;
#146536=CARTESIAN_POINT('',(7.9,2.1,-7.12)) ;
#146537=CARTESIAN_POINT('Origin',(1.4,2.4,-7.02)) ;
#146538=CARTESIAN_POINT('',(1.5,2.5,-7.02)) ;
#146539=CARTESIAN_POINT('Origin',(1.5,2.4,-7.02)) ;
#146540=CARTESIAN_POINT('',(7.9,2.5,-7.02)) ;
#146541=CARTESIAN_POINT('',(1.4,2.5,-7.02)) ;
#146542=CARTESIAN_POINT('Origin',(7.9,2.4,-7.02)) ;
#146543=CARTESIAN_POINT('Origin',(1.4,2.5,-6.91142135623731)) ;
#146544=CARTESIAN_POINT('',(1.5,2.5,-6.91142135623731)) ;
#146545=CARTESIAN_POINT('',(1.5,2.5,-6.91142135623731)) ;
#146546=CARTESIAN_POINT('',(7.9,2.5,-6.91142135623731)) ;
#146547=CARTESIAN_POINT('',(1.4,2.5,-6.91142135623731)) ;
#146548=CARTESIAN_POINT('',(7.9,2.5,-7.02)) ;
#146549=CARTESIAN_POINT('Origin',(1.4,2.6,-6.91142135623731)) ;
#146550=CARTESIAN_POINT('',(1.5,2.52928932188135,-6.84071067811866)) ;
#146551=CARTESIAN_POINT('Origin',(1.5,2.6,-6.91142135623731)) ;
#146552=CARTESIAN_POINT('',(7.9,2.52928932188135,-6.84071067811866)) ;
#146553=CARTESIAN_POINT('',(1.4,2.52928932188135,-6.84071067811866)) ;
#146554=CARTESIAN_POINT('Origin',(7.9,2.6,-6.91142135623731)) ;
#146555=CARTESIAN_POINT('Origin',(1.4,3.07928932188135,-6.29071067811866)) ;
#146556=CARTESIAN_POINT('',(1.5,3.07928932188135,-6.29071067811866)) ;
#146557=CARTESIAN_POINT('',(7.9,3.07928932188135,-6.29071067811866)) ;
#146558=CARTESIAN_POINT('',(1.4,3.07928932188135,-6.29071067811866)) ;
#146559=CARTESIAN_POINT('',(7.9,2.52928932188135,-6.84071067811866)) ;
#146560=CARTESIAN_POINT('Origin',(1.4,3.15,-6.36142135623731)) ;
#146561=CARTESIAN_POINT('',(7.9,3.25,-6.36142135623731)) ;
#146562=CARTESIAN_POINT('',(1.4,3.25,-6.36142135623731)) ;
#146563=CARTESIAN_POINT('Origin',(7.9,3.15,-6.36142135623731)) ;
#146564=CARTESIAN_POINT('Origin',(1.4,3.25,-8.87857864376269)) ;
#146565=CARTESIAN_POINT('',(1.5,3.25,-8.87857864376269)) ;
#146566=CARTESIAN_POINT('',(7.9,3.25,-6.36142135623731)) ;
#146567=CARTESIAN_POINT('Origin',(1.4,2.52928932188134,-8.39928932188135)) ;
#146568=CARTESIAN_POINT('',(1.5,2.52928932188134,-8.39928932188135)) ;
#146569=CARTESIAN_POINT('',(1.5,2.52928932188134,-8.39928932188135)) ;
#146570=CARTESIAN_POINT('',(7.9,2.52928932188134,-8.39928932188135)) ;
#146571=CARTESIAN_POINT('',(1.4,2.52928932188134,-8.39928932188135)) ;
#146572=CARTESIAN_POINT('',(7.9,3.07928932188135,-8.94928932188134)) ;
#146573=CARTESIAN_POINT('Origin',(1.4,2.6,-8.32857864376269)) ;
#146574=CARTESIAN_POINT('',(1.5,2.5,-8.32857864376269)) ;
#146575=CARTESIAN_POINT('Origin',(1.5,2.6,-8.32857864376269)) ;
#146576=CARTESIAN_POINT('',(7.9,2.5,-8.32857864376269)) ;
#146577=CARTESIAN_POINT('',(1.4,2.5,-8.32857864376269)) ;
#146578=CARTESIAN_POINT('Origin',(7.9,2.6,-8.32857864376269)) ;
#146579=CARTESIAN_POINT('Origin',(1.4,2.5,-8.22)) ;
#146580=CARTESIAN_POINT('',(1.5,2.5,-8.22)) ;
#146581=CARTESIAN_POINT('',(1.5,2.5,-8.22)) ;
#146582=CARTESIAN_POINT('',(7.9,2.5,-8.22)) ;
#146583=CARTESIAN_POINT('',(1.4,2.5,-8.22)) ;
#146584=CARTESIAN_POINT('',(7.9,2.5,-8.32857864376269)) ;
#146585=CARTESIAN_POINT('Origin',(1.4,2.4,-8.22)) ;
#146586=CARTESIAN_POINT('',(1.5,2.4,-8.12)) ;
#146587=CARTESIAN_POINT('Origin',(1.5,2.4,-8.22)) ;
#146588=CARTESIAN_POINT('',(7.9,2.4,-8.12)) ;
#146589=CARTESIAN_POINT('',(1.4,2.4,-8.12)) ;
#146590=CARTESIAN_POINT('Origin',(7.9,2.4,-8.22)) ;
#146591=CARTESIAN_POINT('Origin',(1.4,2.1,-8.12)) ;
#146592=CARTESIAN_POINT('',(1.5,2.1,-8.12)) ;
#146593=CARTESIAN_POINT('',(1.5,2.1,-8.12)) ;
#146594=CARTESIAN_POINT('',(7.9,2.1,-8.12)) ;
#146595=CARTESIAN_POINT('',(1.4,2.1,-8.12)) ;
#146596=CARTESIAN_POINT('',(7.9,2.4,-8.12)) ;
#146597=CARTESIAN_POINT('Origin',(1.4,2.1,-8.22)) ;
#146598=CARTESIAN_POINT('',(1.5,2.,-8.22)) ;
#146599=CARTESIAN_POINT('Origin',(1.5,2.1,-8.22)) ;
#146600=CARTESIAN_POINT('',(7.9,2.,-8.22)) ;
#146601=CARTESIAN_POINT('',(1.4,2.,-8.22)) ;
#146602=CARTESIAN_POINT('Origin',(7.9,2.1,-8.22)) ;
#146603=CARTESIAN_POINT('Origin',(1.4,2.,-8.22)) ;
#146604=CARTESIAN_POINT('',(1.5,2.,-9.17)) ;
#146605=CARTESIAN_POINT('',(1.5,2.,-9.17)) ;
#146606=CARTESIAN_POINT('',(7.9,2.,-9.17)) ;
#146607=CARTESIAN_POINT('',(1.4,2.,-9.17)) ;
#146608=CARTESIAN_POINT('',(7.9,2.,-8.22)) ;
#146609=CARTESIAN_POINT('Origin',(1.4,1.9,-9.17)) ;
#146610=CARTESIAN_POINT('',(1.5,1.9,-9.27)) ;
#146611=CARTESIAN_POINT('Origin',(1.5,1.9,-9.17)) ;
#146612=CARTESIAN_POINT('',(7.9,1.9,-9.27)) ;
#146613=CARTESIAN_POINT('',(1.4,1.9,-9.27)) ;
#146614=CARTESIAN_POINT('Origin',(7.9,1.9,-9.17)) ;
#146615=CARTESIAN_POINT('Origin',(1.4,1.9,-9.27)) ;
#146616=CARTESIAN_POINT('',(1.5,-2.15,-9.27)) ;
#146617=CARTESIAN_POINT('',(1.5,-2.15,-9.27)) ;
#146618=CARTESIAN_POINT('',(7.9,-2.15,-9.27)) ;
#146619=CARTESIAN_POINT('',(1.4,-2.15,-9.27)) ;
#146620=CARTESIAN_POINT('',(7.9,1.9,-9.27)) ;
#146621=CARTESIAN_POINT('Origin',(1.4,-2.15,-9.17)) ;
#146622=CARTESIAN_POINT('',(1.5,-2.25,-9.17)) ;
#146623=CARTESIAN_POINT('Origin',(1.5,-2.15,-9.17)) ;
#146624=CARTESIAN_POINT('',(7.9,-2.25,-9.17)) ;
#146625=CARTESIAN_POINT('',(1.4,-2.25,-9.17)) ;
#146626=CARTESIAN_POINT('Origin',(7.9,-2.15,-9.17)) ;
#146627=CARTESIAN_POINT('Origin',(1.4,-2.25,-8.52311959340942)) ;
#146628=CARTESIAN_POINT('',(1.5,-2.25,-8.52311959340942)) ;
#146629=CARTESIAN_POINT('',(1.5,-2.25,-8.52311959340942)) ;
#146630=CARTESIAN_POINT('',(7.9,-2.25,-8.52311959340942)) ;
#146631=CARTESIAN_POINT('',(1.4,-2.25,-8.52311959340942)) ;
#146632=CARTESIAN_POINT('',(7.9,-2.25,-9.17)) ;
#146633=CARTESIAN_POINT('Origin',(1.4,-2.15,-8.52311959340942)) ;
#146634=CARTESIAN_POINT('',(1.5,-2.23576512455516,-8.47169641371351)) ;
#146635=CARTESIAN_POINT('Origin',(1.5,-2.15,-8.52311959340942)) ;
#146636=CARTESIAN_POINT('',(7.9,-2.23576512455516,-8.47169641371351)) ;
#146637=CARTESIAN_POINT('',(1.4,-2.23576512455516,-8.47169641371351)) ;
#146638=CARTESIAN_POINT('Origin',(7.9,-2.15,-8.52311959340942)) ;
#146639=CARTESIAN_POINT('Origin',(1.4,-3.65625,-7.62)) ;
#146640=CARTESIAN_POINT('',(1.5,-2.23576512455516,-6.76830358628649)) ;
#146641=CARTESIAN_POINT('Origin',(1.5,-3.65625,-7.62)) ;
#146642=CARTESIAN_POINT('',(7.9,-2.23576512455516,-6.76830358628649)) ;
#146643=CARTESIAN_POINT('',(1.4,-2.23576512455516,-6.76830358628649)) ;
#146644=CARTESIAN_POINT('Origin',(7.9,-3.65625,-7.62)) ;
#146645=CARTESIAN_POINT('Origin',(1.4,-2.15,-6.71688040659058)) ;
#146646=CARTESIAN_POINT('',(1.5,-2.25,-6.71688040659058)) ;
#146647=CARTESIAN_POINT('Origin',(1.5,-2.15,-6.71688040659058)) ;
#146648=CARTESIAN_POINT('',(7.9,-2.25,-6.71688040659058)) ;
#146649=CARTESIAN_POINT('',(1.4,-2.25,-6.71688040659058)) ;
#146650=CARTESIAN_POINT('Origin',(7.9,-2.15,-6.71688040659058)) ;
#146651=CARTESIAN_POINT('Origin',(1.4,-2.25,-6.07)) ;
#146652=CARTESIAN_POINT('',(1.5,-2.25,-6.07)) ;
#146653=CARTESIAN_POINT('',(1.5,-2.25,-6.07)) ;
#146654=CARTESIAN_POINT('',(7.9,-2.25,-6.07)) ;
#146655=CARTESIAN_POINT('',(1.4,-2.25,-6.07)) ;
#146656=CARTESIAN_POINT('',(7.9,-2.25,-6.71688040659058)) ;
#146657=CARTESIAN_POINT('Origin',(1.4,-2.15,-6.07)) ;
#146658=CARTESIAN_POINT('',(1.5,-2.15,-5.97)) ;
#146659=CARTESIAN_POINT('Origin',(1.5,-2.15,-6.07)) ;
#146660=CARTESIAN_POINT('',(7.9,-2.15,-5.97)) ;
#146661=CARTESIAN_POINT('',(1.4,-2.15,-5.97)) ;
#146662=CARTESIAN_POINT('Origin',(7.9,-2.15,-6.07)) ;
#146663=CARTESIAN_POINT('Origin',(1.4,1.9,-5.97)) ;
#146664=CARTESIAN_POINT('',(1.5,1.9,-5.97)) ;
#146665=CARTESIAN_POINT('',(1.5,1.9,-5.97)) ;
#146666=CARTESIAN_POINT('',(7.9,1.9,-5.97)) ;
#146667=CARTESIAN_POINT('',(1.4,1.9,-5.97)) ;
#146668=CARTESIAN_POINT('',(7.9,-2.15,-5.97)) ;
#146669=CARTESIAN_POINT('Origin',(1.4,1.9,-6.07)) ;
#146670=CARTESIAN_POINT('',(1.5,2.,-6.07)) ;
#146671=CARTESIAN_POINT('Origin',(1.5,1.9,-6.07)) ;
#146672=CARTESIAN_POINT('',(7.9,2.,-6.07)) ;
#146673=CARTESIAN_POINT('',(1.4,2.,-6.07)) ;
#146674=CARTESIAN_POINT('Origin',(7.9,1.9,-6.07)) ;
#146675=CARTESIAN_POINT('Origin',(1.4,2.,-6.07)) ;
#146676=CARTESIAN_POINT('',(1.5,2.,-7.02)) ;
#146677=CARTESIAN_POINT('',(7.9,2.,-6.07)) ;
#146678=CARTESIAN_POINT('Origin',(1.4,2.1,-7.02)) ;
#146679=CARTESIAN_POINT('',(1.4,2.6,-7.02)) ;
#146680=CARTESIAN_POINT('',(1.4,2.4,-7.22)) ;
#146681=CARTESIAN_POINT('Origin',(1.4,2.4,-7.02)) ;
#146682=CARTESIAN_POINT('',(1.4,2.1,-7.22)) ;
#146683=CARTESIAN_POINT('',(1.4,2.1,-7.22)) ;
#146684=CARTESIAN_POINT('',(1.4,1.9,-7.02)) ;
#146685=CARTESIAN_POINT('Origin',(1.4,2.1,-7.02)) ;
#146686=CARTESIAN_POINT('',(1.4,1.9,-6.07)) ;
#146687=CARTESIAN_POINT('',(1.4,1.9,-6.07)) ;
#146688=CARTESIAN_POINT('',(1.4,-2.15,-6.07)) ;
#146689=CARTESIAN_POINT('',(1.4,-2.15,-6.07)) ;
#146690=CARTESIAN_POINT('',(1.4,-2.15,-6.71688040659058)) ;
#146691=CARTESIAN_POINT('',(1.4,-2.15,-6.71688040659058)) ;
#146692=CARTESIAN_POINT('',(1.4,-2.15,-8.52311959340942)) ;
#146693=CARTESIAN_POINT('Origin',(1.4,-3.65625,-7.62)) ;
#146694=CARTESIAN_POINT('',(1.4,-2.15,-9.17)) ;
#146695=CARTESIAN_POINT('',(1.4,-2.15,-9.17)) ;
#146696=CARTESIAN_POINT('',(1.4,1.9,-9.17)) ;
#146697=CARTESIAN_POINT('',(1.4,1.9,-9.17)) ;
#146698=CARTESIAN_POINT('',(1.4,1.9,-8.22)) ;
#146699=CARTESIAN_POINT('',(1.4,1.9,-8.22)) ;
#146700=CARTESIAN_POINT('',(1.4,2.1,-8.02)) ;
#146701=CARTESIAN_POINT('Origin',(1.4,2.1,-8.22)) ;
#146702=CARTESIAN_POINT('',(1.4,2.4,-8.02)) ;
#146703=CARTESIAN_POINT('',(1.4,2.4,-8.02)) ;
#146704=CARTESIAN_POINT('',(1.4,2.6,-8.22)) ;
#146705=CARTESIAN_POINT('Origin',(1.4,2.4,-8.22)) ;
#146706=CARTESIAN_POINT('',(1.4,2.6,-8.32857864376269)) ;
#146707=CARTESIAN_POINT('',(1.4,2.6,-8.32857864376269)) ;
#146708=CARTESIAN_POINT('',(1.4,3.15,-8.87857864376269)) ;
#146709=CARTESIAN_POINT('',(1.4,3.15,-8.87857864376269)) ;
#146710=CARTESIAN_POINT('',(1.4,3.15,-6.36142135623731)) ;
#146711=CARTESIAN_POINT('',(1.4,2.6,-6.91142135623731)) ;
#146712=CARTESIAN_POINT('',(1.4,2.6,-6.91142135623731)) ;
#146713=CARTESIAN_POINT('',(1.4,2.6,-7.02)) ;
#146714=CARTESIAN_POINT('Origin',(1.4,2.1,-3.21)) ;
#146715=CARTESIAN_POINT('',(1.5,2.,-3.21)) ;
#146716=CARTESIAN_POINT('',(7.9,2.,-3.21)) ;
#146717=CARTESIAN_POINT('',(1.4,2.,-3.21)) ;
#146718=CARTESIAN_POINT('',(1.5,2.1,-3.31)) ;
#146719=CARTESIAN_POINT('Origin',(1.5,2.1,-3.21)) ;
#146720=CARTESIAN_POINT('',(7.9,2.1,-3.31)) ;
#146721=CARTESIAN_POINT('',(1.4,2.1,-3.31)) ;
#146722=CARTESIAN_POINT('Origin',(7.9,2.1,-3.21)) ;
#146723=CARTESIAN_POINT('Origin',(1.4,2.4,-3.31)) ;
#146724=CARTESIAN_POINT('',(1.5,2.4,-3.31)) ;
#146725=CARTESIAN_POINT('',(1.5,2.4,-3.31)) ;
#146726=CARTESIAN_POINT('',(7.9,2.4,-3.31)) ;
#146727=CARTESIAN_POINT('',(1.4,2.4,-3.31)) ;
#146728=CARTESIAN_POINT('',(7.9,2.1,-3.31)) ;
#146729=CARTESIAN_POINT('Origin',(1.4,2.4,-3.21)) ;
#146730=CARTESIAN_POINT('',(1.5,2.5,-3.21)) ;
#146731=CARTESIAN_POINT('Origin',(1.5,2.4,-3.21)) ;
#146732=CARTESIAN_POINT('',(7.9,2.5,-3.21)) ;
#146733=CARTESIAN_POINT('',(1.4,2.5,-3.21)) ;
#146734=CARTESIAN_POINT('Origin',(7.9,2.4,-3.21)) ;
#146735=CARTESIAN_POINT('Origin',(1.4,2.5,-3.10142135623731)) ;
#146736=CARTESIAN_POINT('',(1.5,2.5,-3.10142135623731)) ;
#146737=CARTESIAN_POINT('',(1.5,2.5,-3.10142135623731)) ;
#146738=CARTESIAN_POINT('',(7.9,2.5,-3.10142135623731)) ;
#146739=CARTESIAN_POINT('',(1.4,2.5,-3.10142135623731)) ;
#146740=CARTESIAN_POINT('',(7.9,2.5,-3.21)) ;
#146741=CARTESIAN_POINT('Origin',(1.4,2.6,-3.10142135623731)) ;
#146742=CARTESIAN_POINT('',(1.5,2.52928932188135,-3.03071067811866)) ;
#146743=CARTESIAN_POINT('Origin',(1.5,2.6,-3.10142135623731)) ;
#146744=CARTESIAN_POINT('',(7.9,2.52928932188135,-3.03071067811866)) ;
#146745=CARTESIAN_POINT('',(1.4,2.52928932188135,-3.03071067811866)) ;
#146746=CARTESIAN_POINT('Origin',(7.9,2.6,-3.10142135623731)) ;
#146747=CARTESIAN_POINT('Origin',(1.4,3.07928932188135,-2.48071067811865)) ;
#146748=CARTESIAN_POINT('',(1.5,3.07928932188135,-2.48071067811865)) ;
#146749=CARTESIAN_POINT('',(7.9,3.07928932188135,-2.48071067811865)) ;
#146750=CARTESIAN_POINT('',(1.4,3.07928932188135,-2.48071067811865)) ;
#146751=CARTESIAN_POINT('',(7.9,2.52928932188135,-3.03071067811866)) ;
#146752=CARTESIAN_POINT('Origin',(1.4,3.15,-2.55142135623731)) ;
#146753=CARTESIAN_POINT('',(7.9,3.25,-2.55142135623731)) ;
#146754=CARTESIAN_POINT('',(1.4,3.25,-2.55142135623731)) ;
#146755=CARTESIAN_POINT('Origin',(7.9,3.15,-2.55142135623731)) ;
#146756=CARTESIAN_POINT('Origin',(1.4,3.25,-5.06857864376269)) ;
#146757=CARTESIAN_POINT('',(1.5,3.25,-5.06857864376269)) ;
#146758=CARTESIAN_POINT('',(7.9,3.25,-2.55142135623731)) ;
#146759=CARTESIAN_POINT('Origin',(1.4,2.52928932188134,-4.58928932188135)) ;
#146760=CARTESIAN_POINT('',(1.5,2.52928932188134,-4.58928932188135)) ;
#146761=CARTESIAN_POINT('',(1.5,2.52928932188134,-4.58928932188135)) ;
#146762=CARTESIAN_POINT('',(7.9,2.52928932188134,-4.58928932188135)) ;
#146763=CARTESIAN_POINT('',(1.4,2.52928932188134,-4.58928932188135)) ;
#146764=CARTESIAN_POINT('',(7.9,3.07928932188135,-5.13928932188135)) ;
#146765=CARTESIAN_POINT('Origin',(1.4,2.6,-4.51857864376269)) ;
#146766=CARTESIAN_POINT('',(1.5,2.5,-4.51857864376269)) ;
#146767=CARTESIAN_POINT('Origin',(1.5,2.6,-4.51857864376269)) ;
#146768=CARTESIAN_POINT('',(7.9,2.5,-4.51857864376269)) ;
#146769=CARTESIAN_POINT('',(1.4,2.5,-4.51857864376269)) ;
#146770=CARTESIAN_POINT('Origin',(7.9,2.6,-4.51857864376269)) ;
#146771=CARTESIAN_POINT('Origin',(1.4,2.5,-4.41)) ;
#146772=CARTESIAN_POINT('',(1.5,2.5,-4.41)) ;
#146773=CARTESIAN_POINT('',(1.5,2.5,-4.41)) ;
#146774=CARTESIAN_POINT('',(7.9,2.5,-4.41)) ;
#146775=CARTESIAN_POINT('',(1.4,2.5,-4.41)) ;
#146776=CARTESIAN_POINT('',(7.9,2.5,-4.51857864376269)) ;
#146777=CARTESIAN_POINT('Origin',(1.4,2.4,-4.41)) ;
#146778=CARTESIAN_POINT('',(1.5,2.4,-4.31)) ;
#146779=CARTESIAN_POINT('Origin',(1.5,2.4,-4.41)) ;
#146780=CARTESIAN_POINT('',(7.9,2.4,-4.31)) ;
#146781=CARTESIAN_POINT('',(1.4,2.4,-4.31)) ;
#146782=CARTESIAN_POINT('Origin',(7.9,2.4,-4.41)) ;
#146783=CARTESIAN_POINT('Origin',(1.4,2.1,-4.31)) ;
#146784=CARTESIAN_POINT('',(1.5,2.1,-4.31)) ;
#146785=CARTESIAN_POINT('',(1.5,2.1,-4.31)) ;
#146786=CARTESIAN_POINT('',(7.9,2.1,-4.31)) ;
#146787=CARTESIAN_POINT('',(1.4,2.1,-4.31)) ;
#146788=CARTESIAN_POINT('',(7.9,2.4,-4.31)) ;
#146789=CARTESIAN_POINT('Origin',(1.4,2.1,-4.41)) ;
#146790=CARTESIAN_POINT('',(1.5,2.,-4.41)) ;
#146791=CARTESIAN_POINT('Origin',(1.5,2.1,-4.41)) ;
#146792=CARTESIAN_POINT('',(7.9,2.,-4.41)) ;
#146793=CARTESIAN_POINT('',(1.4,2.,-4.41)) ;
#146794=CARTESIAN_POINT('Origin',(7.9,2.1,-4.41)) ;
#146795=CARTESIAN_POINT('Origin',(1.4,2.,-4.41)) ;
#146796=CARTESIAN_POINT('',(1.5,2.,-5.36)) ;
#146797=CARTESIAN_POINT('',(1.5,2.,-5.36)) ;
#146798=CARTESIAN_POINT('',(7.9,2.,-5.36)) ;
#146799=CARTESIAN_POINT('',(1.4,2.,-5.36)) ;
#146800=CARTESIAN_POINT('',(7.9,2.,-4.41)) ;
#146801=CARTESIAN_POINT('Origin',(1.4,1.9,-5.36)) ;
#146802=CARTESIAN_POINT('',(1.5,1.9,-5.46)) ;
#146803=CARTESIAN_POINT('Origin',(1.5,1.9,-5.36)) ;
#146804=CARTESIAN_POINT('',(7.9,1.9,-5.46)) ;
#146805=CARTESIAN_POINT('',(1.4,1.9,-5.46)) ;
#146806=CARTESIAN_POINT('Origin',(7.9,1.9,-5.36)) ;
#146807=CARTESIAN_POINT('Origin',(1.4,1.9,-5.46)) ;
#146808=CARTESIAN_POINT('',(1.5,-2.15,-5.46)) ;
#146809=CARTESIAN_POINT('',(1.5,-2.15,-5.46)) ;
#146810=CARTESIAN_POINT('',(7.9,-2.15,-5.46)) ;
#146811=CARTESIAN_POINT('',(1.4,-2.15,-5.46)) ;
#146812=CARTESIAN_POINT('',(7.9,1.9,-5.46)) ;
#146813=CARTESIAN_POINT('Origin',(1.4,-2.15,-5.36)) ;
#146814=CARTESIAN_POINT('',(1.5,-2.25,-5.36)) ;
#146815=CARTESIAN_POINT('Origin',(1.5,-2.15,-5.36)) ;
#146816=CARTESIAN_POINT('',(7.9,-2.25,-5.36)) ;
#146817=CARTESIAN_POINT('',(1.4,-2.25,-5.36)) ;
#146818=CARTESIAN_POINT('Origin',(7.9,-2.15,-5.36)) ;
#146819=CARTESIAN_POINT('Origin',(1.4,-2.25,-4.71311959340942)) ;
#146820=CARTESIAN_POINT('',(1.5,-2.25,-4.71311959340942)) ;
#146821=CARTESIAN_POINT('',(1.5,-2.25,-4.71311959340942)) ;
#146822=CARTESIAN_POINT('',(7.9,-2.25,-4.71311959340942)) ;
#146823=CARTESIAN_POINT('',(1.4,-2.25,-4.71311959340942)) ;
#146824=CARTESIAN_POINT('',(7.9,-2.25,-5.36)) ;
#146825=CARTESIAN_POINT('Origin',(1.4,-2.15,-4.71311959340942)) ;
#146826=CARTESIAN_POINT('',(1.5,-2.23576512455516,-4.66169641371351)) ;
#146827=CARTESIAN_POINT('Origin',(1.5,-2.15,-4.71311959340942)) ;
#146828=CARTESIAN_POINT('',(7.9,-2.23576512455516,-4.66169641371351)) ;
#146829=CARTESIAN_POINT('',(1.4,-2.23576512455516,-4.66169641371351)) ;
#146830=CARTESIAN_POINT('Origin',(7.9,-2.15,-4.71311959340942)) ;
#146831=CARTESIAN_POINT('Origin',(1.4,-3.65625,-3.81)) ;
#146832=CARTESIAN_POINT('',(1.5,-2.23576512455516,-2.95830358628649)) ;
#146833=CARTESIAN_POINT('Origin',(1.5,-3.65625,-3.81)) ;
#146834=CARTESIAN_POINT('',(7.9,-2.23576512455516,-2.95830358628649)) ;
#146835=CARTESIAN_POINT('',(1.4,-2.23576512455516,-2.95830358628649)) ;
#146836=CARTESIAN_POINT('Origin',(7.9,-3.65625,-3.81)) ;
#146837=CARTESIAN_POINT('Origin',(1.4,-2.15,-2.90688040659058)) ;
#146838=CARTESIAN_POINT('',(1.5,-2.25,-2.90688040659058)) ;
#146839=CARTESIAN_POINT('Origin',(1.5,-2.15,-2.90688040659058)) ;
#146840=CARTESIAN_POINT('',(7.9,-2.25,-2.90688040659058)) ;
#146841=CARTESIAN_POINT('',(1.4,-2.25,-2.90688040659058)) ;
#146842=CARTESIAN_POINT('Origin',(7.9,-2.15,-2.90688040659058)) ;
#146843=CARTESIAN_POINT('Origin',(1.4,-2.25,-2.26)) ;
#146844=CARTESIAN_POINT('',(1.5,-2.25,-2.26)) ;
#146845=CARTESIAN_POINT('',(1.5,-2.25,-2.26)) ;
#146846=CARTESIAN_POINT('',(7.9,-2.25,-2.26)) ;
#146847=CARTESIAN_POINT('',(1.4,-2.25,-2.26)) ;
#146848=CARTESIAN_POINT('',(7.9,-2.25,-2.90688040659058)) ;
#146849=CARTESIAN_POINT('Origin',(1.4,-2.15,-2.26)) ;
#146850=CARTESIAN_POINT('',(1.5,-2.15,-2.16)) ;
#146851=CARTESIAN_POINT('Origin',(1.5,-2.15,-2.26)) ;
#146852=CARTESIAN_POINT('',(7.9,-2.15,-2.16)) ;
#146853=CARTESIAN_POINT('',(1.4,-2.15,-2.16)) ;
#146854=CARTESIAN_POINT('Origin',(7.9,-2.15,-2.26)) ;
#146855=CARTESIAN_POINT('Origin',(1.4,1.9,-2.16)) ;
#146856=CARTESIAN_POINT('',(1.5,1.9,-2.16)) ;
#146857=CARTESIAN_POINT('',(1.5,1.9,-2.16)) ;
#146858=CARTESIAN_POINT('',(7.9,1.9,-2.16)) ;
#146859=CARTESIAN_POINT('',(1.4,1.9,-2.16)) ;
#146860=CARTESIAN_POINT('',(7.9,-2.15,-2.16)) ;
#146861=CARTESIAN_POINT('Origin',(1.4,1.9,-2.26)) ;
#146862=CARTESIAN_POINT('',(1.5,2.,-2.26)) ;
#146863=CARTESIAN_POINT('Origin',(1.5,1.9,-2.26)) ;
#146864=CARTESIAN_POINT('',(7.9,2.,-2.26)) ;
#146865=CARTESIAN_POINT('',(1.4,2.,-2.26)) ;
#146866=CARTESIAN_POINT('Origin',(7.9,1.9,-2.26)) ;
#146867=CARTESIAN_POINT('Origin',(1.4,2.,-2.26)) ;
#146868=CARTESIAN_POINT('',(1.5,2.,-3.21)) ;
#146869=CARTESIAN_POINT('',(7.9,2.,-2.26)) ;
#146870=CARTESIAN_POINT('Origin',(1.4,2.1,-3.21)) ;
#146871=CARTESIAN_POINT('',(1.4,2.6,-3.21)) ;
#146872=CARTESIAN_POINT('',(1.4,2.4,-3.41)) ;
#146873=CARTESIAN_POINT('Origin',(1.4,2.4,-3.21)) ;
#146874=CARTESIAN_POINT('',(1.4,2.1,-3.41)) ;
#146875=CARTESIAN_POINT('',(1.4,2.1,-3.41)) ;
#146876=CARTESIAN_POINT('',(1.4,1.9,-3.21)) ;
#146877=CARTESIAN_POINT('Origin',(1.4,2.1,-3.21)) ;
#146878=CARTESIAN_POINT('',(1.4,1.9,-2.26)) ;
#146879=CARTESIAN_POINT('',(1.4,1.9,-2.26)) ;
#146880=CARTESIAN_POINT('',(1.4,-2.15,-2.26)) ;
#146881=CARTESIAN_POINT('',(1.4,-2.15,-2.26)) ;
#146882=CARTESIAN_POINT('',(1.4,-2.15,-2.90688040659058)) ;
#146883=CARTESIAN_POINT('',(1.4,-2.15,-2.90688040659058)) ;
#146884=CARTESIAN_POINT('',(1.4,-2.15,-4.71311959340942)) ;
#146885=CARTESIAN_POINT('Origin',(1.4,-3.65625,-3.81)) ;
#146886=CARTESIAN_POINT('',(1.4,-2.15,-5.36)) ;
#146887=CARTESIAN_POINT('',(1.4,-2.15,-5.36)) ;
#146888=CARTESIAN_POINT('',(1.4,1.9,-5.36)) ;
#146889=CARTESIAN_POINT('',(1.4,1.9,-5.36)) ;
#146890=CARTESIAN_POINT('',(1.4,1.9,-4.41)) ;
#146891=CARTESIAN_POINT('',(1.4,1.9,-4.41)) ;
#146892=CARTESIAN_POINT('',(1.4,2.1,-4.21)) ;
#146893=CARTESIAN_POINT('Origin',(1.4,2.1,-4.41)) ;
#146894=CARTESIAN_POINT('',(1.4,2.4,-4.21)) ;
#146895=CARTESIAN_POINT('',(1.4,2.4,-4.21)) ;
#146896=CARTESIAN_POINT('',(1.4,2.6,-4.41)) ;
#146897=CARTESIAN_POINT('Origin',(1.4,2.4,-4.41)) ;
#146898=CARTESIAN_POINT('',(1.4,2.6,-4.51857864376269)) ;
#146899=CARTESIAN_POINT('',(1.4,2.6,-4.51857864376269)) ;
#146900=CARTESIAN_POINT('',(1.4,3.15,-5.06857864376269)) ;
#146901=CARTESIAN_POINT('',(1.4,3.15,-5.06857864376269)) ;
#146902=CARTESIAN_POINT('',(1.4,3.15,-2.55142135623731)) ;
#146903=CARTESIAN_POINT('',(1.4,2.6,-3.10142135623731)) ;
#146904=CARTESIAN_POINT('',(1.4,2.6,-3.10142135623731)) ;
#146905=CARTESIAN_POINT('',(1.4,2.6,-3.21)) ;
#146906=CARTESIAN_POINT('Origin',(2.4,0.,-3.81)) ;
#146907=CARTESIAN_POINT('',(2.4,0.3,-3.41)) ;
#146908=CARTESIAN_POINT('',(2.4,-0.3,-3.41)) ;
#146909=CARTESIAN_POINT('',(2.4,0.,-3.41)) ;
#146910=CARTESIAN_POINT('',(2.4,0.4,-3.51)) ;
#146911=CARTESIAN_POINT('Origin',(2.4,0.3,-3.51)) ;
#146912=CARTESIAN_POINT('',(2.4,0.4,-4.11)) ;
#146913=CARTESIAN_POINT('',(2.4,0.4,-3.81)) ;
#146914=CARTESIAN_POINT('',(2.4,0.3,-4.21)) ;
#146915=CARTESIAN_POINT('Origin',(2.4,0.3,-4.11)) ;
#146916=CARTESIAN_POINT('',(2.4,-0.3,-4.21)) ;
#146917=CARTESIAN_POINT('',(2.4,0.,-4.21)) ;
#146918=CARTESIAN_POINT('',(2.4,-0.4,-4.11)) ;
#146919=CARTESIAN_POINT('Origin',(2.4,-0.3,-4.11)) ;
#146920=CARTESIAN_POINT('',(2.4,-0.4,-3.51)) ;
#146921=CARTESIAN_POINT('',(2.4,-0.4,-3.81)) ;
#146922=CARTESIAN_POINT('Origin',(2.4,-0.3,-3.51)) ;
#146923=CARTESIAN_POINT('Origin',(2.4,0.,-7.62)) ;
#146924=CARTESIAN_POINT('',(2.4,0.3,-7.22)) ;
#146925=CARTESIAN_POINT('',(2.4,-0.3,-7.22)) ;
#146926=CARTESIAN_POINT('',(2.4,0.,-7.22)) ;
#146927=CARTESIAN_POINT('',(2.4,0.4,-7.32)) ;
#146928=CARTESIAN_POINT('Origin',(2.4,0.3,-7.32)) ;
#146929=CARTESIAN_POINT('',(2.4,0.4,-7.92)) ;
#146930=CARTESIAN_POINT('',(2.4,0.4,-7.62)) ;
#146931=CARTESIAN_POINT('',(2.4,0.3,-8.02)) ;
#146932=CARTESIAN_POINT('Origin',(2.4,0.3,-7.92)) ;
#146933=CARTESIAN_POINT('',(2.4,-0.3,-8.02)) ;
#146934=CARTESIAN_POINT('',(2.4,0.,-8.02)) ;
#146935=CARTESIAN_POINT('',(2.4,-0.4,-7.92)) ;
#146936=CARTESIAN_POINT('Origin',(2.4,-0.3,-7.92)) ;
#146937=CARTESIAN_POINT('',(2.4,-0.4,-7.32)) ;
#146938=CARTESIAN_POINT('',(2.4,-0.4,-7.62)) ;
#146939=CARTESIAN_POINT('Origin',(2.4,-0.3,-7.32)) ;
#146940=CARTESIAN_POINT('Origin',(2.4,0.,-11.43)) ;
#146941=CARTESIAN_POINT('',(2.4,0.3,-11.03)) ;
#146942=CARTESIAN_POINT('',(2.4,-0.3,-11.03)) ;
#146943=CARTESIAN_POINT('',(2.4,0.,-11.03)) ;
#146944=CARTESIAN_POINT('',(2.4,0.4,-11.13)) ;
#146945=CARTESIAN_POINT('Origin',(2.4,0.3,-11.13)) ;
#146946=CARTESIAN_POINT('',(2.4,0.4,-11.73)) ;
#146947=CARTESIAN_POINT('',(2.4,0.4,-11.43)) ;
#146948=CARTESIAN_POINT('',(2.4,0.3,-11.83)) ;
#146949=CARTESIAN_POINT('Origin',(2.4,0.3,-11.73)) ;
#146950=CARTESIAN_POINT('',(2.4,-0.3,-11.83)) ;
#146951=CARTESIAN_POINT('',(2.4,0.,-11.83)) ;
#146952=CARTESIAN_POINT('',(2.4,-0.4,-11.73)) ;
#146953=CARTESIAN_POINT('Origin',(2.4,-0.3,-11.73)) ;
#146954=CARTESIAN_POINT('',(2.4,-0.4,-11.13)) ;
#146955=CARTESIAN_POINT('',(2.4,-0.4,-11.43)) ;
#146956=CARTESIAN_POINT('Origin',(2.4,-0.3,-11.13)) ;
#146957=CARTESIAN_POINT('Origin',(2.4,0.,-15.24)) ;
#146958=CARTESIAN_POINT('',(2.4,0.3,-14.84)) ;
#146959=CARTESIAN_POINT('',(2.4,-0.3,-14.84)) ;
#146960=CARTESIAN_POINT('',(2.4,0.,-14.84)) ;
#146961=CARTESIAN_POINT('',(2.4,0.4,-14.94)) ;
#146962=CARTESIAN_POINT('Origin',(2.4,0.3,-14.94)) ;
#146963=CARTESIAN_POINT('',(2.4,0.4,-15.54)) ;
#146964=CARTESIAN_POINT('',(2.4,0.4,-15.24)) ;
#146965=CARTESIAN_POINT('',(2.4,0.3,-15.64)) ;
#146966=CARTESIAN_POINT('Origin',(2.4,0.3,-15.54)) ;
#146967=CARTESIAN_POINT('',(2.4,-0.3,-15.64)) ;
#146968=CARTESIAN_POINT('',(2.4,0.,-15.64)) ;
#146969=CARTESIAN_POINT('',(2.4,-0.4,-15.54)) ;
#146970=CARTESIAN_POINT('Origin',(2.4,-0.3,-15.54)) ;
#146971=CARTESIAN_POINT('',(2.4,-0.4,-14.94)) ;
#146972=CARTESIAN_POINT('',(2.4,-0.4,-15.24)) ;
#146973=CARTESIAN_POINT('Origin',(2.4,-0.3,-14.94)) ;
#146974=CARTESIAN_POINT('Origin',(2.4,0.,-19.05)) ;
#146975=CARTESIAN_POINT('',(2.4,0.3,-18.65)) ;
#146976=CARTESIAN_POINT('',(2.4,-0.3,-18.65)) ;
#146977=CARTESIAN_POINT('',(2.4,0.,-18.65)) ;
#146978=CARTESIAN_POINT('',(2.4,0.4,-18.75)) ;
#146979=CARTESIAN_POINT('Origin',(2.4,0.3,-18.75)) ;
#146980=CARTESIAN_POINT('',(2.4,0.4,-19.35)) ;
#146981=CARTESIAN_POINT('',(2.4,0.4,-19.05)) ;
#146982=CARTESIAN_POINT('',(2.4,0.3,-19.45)) ;
#146983=CARTESIAN_POINT('Origin',(2.4,0.3,-19.35)) ;
#146984=CARTESIAN_POINT('',(2.4,-0.3,-19.45)) ;
#146985=CARTESIAN_POINT('',(2.4,0.,-19.45)) ;
#146986=CARTESIAN_POINT('',(2.4,-0.4,-19.35)) ;
#146987=CARTESIAN_POINT('Origin',(2.4,-0.3,-19.35)) ;
#146988=CARTESIAN_POINT('',(2.4,-0.4,-18.75)) ;
#146989=CARTESIAN_POINT('',(2.4,-0.4,-19.05)) ;
#146990=CARTESIAN_POINT('Origin',(2.4,-0.3,-18.75)) ;
#146991=CARTESIAN_POINT('Origin',(2.4,0.,-22.86)) ;
#146992=CARTESIAN_POINT('',(2.4,0.3,-22.46)) ;
#146993=CARTESIAN_POINT('',(2.4,-0.3,-22.46)) ;
#146994=CARTESIAN_POINT('',(2.4,0.,-22.46)) ;
#146995=CARTESIAN_POINT('',(2.4,0.4,-22.56)) ;
#146996=CARTESIAN_POINT('Origin',(2.4,0.3,-22.56)) ;
#146997=CARTESIAN_POINT('',(2.4,0.4,-23.16)) ;
#146998=CARTESIAN_POINT('',(2.4,0.4,-22.86)) ;
#146999=CARTESIAN_POINT('',(2.4,0.3,-23.26)) ;
#147000=CARTESIAN_POINT('Origin',(2.4,0.3,-23.16)) ;
#147001=CARTESIAN_POINT('',(2.4,-0.3,-23.26)) ;
#147002=CARTESIAN_POINT('',(2.4,0.,-23.26)) ;
#147003=CARTESIAN_POINT('',(2.4,-0.4,-23.16)) ;
#147004=CARTESIAN_POINT('Origin',(2.4,-0.3,-23.16)) ;
#147005=CARTESIAN_POINT('',(2.4,-0.4,-22.56)) ;
#147006=CARTESIAN_POINT('',(2.4,-0.4,-22.86)) ;
#147007=CARTESIAN_POINT('Origin',(2.4,-0.3,-22.56)) ;
#147008=CARTESIAN_POINT('Origin',(2.4,0.,-26.67)) ;
#147009=CARTESIAN_POINT('',(2.4,0.3,-26.27)) ;
#147010=CARTESIAN_POINT('',(2.4,-0.3,-26.27)) ;
#147011=CARTESIAN_POINT('',(2.4,0.,-26.27)) ;
#147012=CARTESIAN_POINT('',(2.4,0.4,-26.37)) ;
#147013=CARTESIAN_POINT('Origin',(2.4,0.3,-26.37)) ;
#147014=CARTESIAN_POINT('',(2.4,0.4,-26.97)) ;
#147015=CARTESIAN_POINT('',(2.4,0.4,-26.67)) ;
#147016=CARTESIAN_POINT('',(2.4,0.3,-27.07)) ;
#147017=CARTESIAN_POINT('Origin',(2.4,0.3,-26.97)) ;
#147018=CARTESIAN_POINT('',(2.4,-0.3,-27.07)) ;
#147019=CARTESIAN_POINT('',(2.4,0.,-27.07)) ;
#147020=CARTESIAN_POINT('',(2.4,-0.4,-26.97)) ;
#147021=CARTESIAN_POINT('Origin',(2.4,-0.3,-26.97)) ;
#147022=CARTESIAN_POINT('',(2.4,-0.4,-26.37)) ;
#147023=CARTESIAN_POINT('',(2.4,-0.4,-26.67)) ;
#147024=CARTESIAN_POINT('Origin',(2.4,-0.3,-26.37)) ;
#147025=CARTESIAN_POINT('Origin',(2.4,0.,-30.48)) ;
#147026=CARTESIAN_POINT('',(2.4,0.3,-30.08)) ;
#147027=CARTESIAN_POINT('',(2.4,-0.3,-30.08)) ;
#147028=CARTESIAN_POINT('',(2.4,0.,-30.08)) ;
#147029=CARTESIAN_POINT('',(2.4,0.4,-30.18)) ;
#147030=CARTESIAN_POINT('Origin',(2.4,0.3,-30.18)) ;
#147031=CARTESIAN_POINT('',(2.4,0.4,-30.78)) ;
#147032=CARTESIAN_POINT('',(2.4,0.4,-30.48)) ;
#147033=CARTESIAN_POINT('',(2.4,0.3,-30.88)) ;
#147034=CARTESIAN_POINT('Origin',(2.4,0.3,-30.78)) ;
#147035=CARTESIAN_POINT('',(2.4,-0.3,-30.88)) ;
#147036=CARTESIAN_POINT('',(2.4,0.,-30.88)) ;
#147037=CARTESIAN_POINT('',(2.4,-0.4,-30.78)) ;
#147038=CARTESIAN_POINT('Origin',(2.4,-0.3,-30.78)) ;
#147039=CARTESIAN_POINT('',(2.4,-0.4,-30.18)) ;
#147040=CARTESIAN_POINT('',(2.4,-0.4,-30.48)) ;
#147041=CARTESIAN_POINT('Origin',(2.4,-0.3,-30.18)) ;
#147042=CARTESIAN_POINT('Origin',(2.4,0.,-34.29)) ;
#147043=CARTESIAN_POINT('',(2.4,0.3,-33.89)) ;
#147044=CARTESIAN_POINT('',(2.4,-0.3,-33.89)) ;
#147045=CARTESIAN_POINT('',(2.4,0.,-33.89)) ;
#147046=CARTESIAN_POINT('',(2.4,0.4,-33.99)) ;
#147047=CARTESIAN_POINT('Origin',(2.4,0.3,-33.99)) ;
#147048=CARTESIAN_POINT('',(2.4,0.4,-34.59)) ;
#147049=CARTESIAN_POINT('',(2.4,0.4,-34.29)) ;
#147050=CARTESIAN_POINT('',(2.4,0.3,-34.69)) ;
#147051=CARTESIAN_POINT('Origin',(2.4,0.3,-34.59)) ;
#147052=CARTESIAN_POINT('',(2.4,-0.3,-34.69)) ;
#147053=CARTESIAN_POINT('',(2.4,0.,-34.69)) ;
#147054=CARTESIAN_POINT('',(2.4,-0.4,-34.59)) ;
#147055=CARTESIAN_POINT('Origin',(2.4,-0.3,-34.59)) ;
#147056=CARTESIAN_POINT('',(2.4,-0.4,-33.99)) ;
#147057=CARTESIAN_POINT('',(2.4,-0.4,-34.29)) ;
#147058=CARTESIAN_POINT('Origin',(2.4,-0.3,-33.99)) ;
#147059=CARTESIAN_POINT('Origin',(-0.899999999999999,-2.,-3.21)) ;
#147060=CARTESIAN_POINT('Origin',(-0.899999999999999,0.4,-3.21)) ;
#147061=CARTESIAN_POINT('Origin',(-0.899999999999999,-1.9,-3.21)) ;
#147062=CARTESIAN_POINT('Origin',(0.600000000000001,0.4,-3.41)) ;
#147063=CARTESIAN_POINT('Origin',(0.500000000000001,0.4,-3.41)) ;
#147064=CARTESIAN_POINT('Origin',(-0.899999999999999,0.4,-3.41)) ;
#147065=CARTESIAN_POINT('Origin',(0.500000000000001,0.4,-3.41)) ;
#147066=CARTESIAN_POINT('',(0.600000000000001,0.4,-3.41)) ;
#147067=CARTESIAN_POINT('Origin',(0.500000000000001,0.4,-3.41)) ;
#147068=CARTESIAN_POINT('Origin',(0.500000000000001,0.4,-3.41)) ;
#147069=CARTESIAN_POINT('Origin',(-0.899999999999999,-1.9,-3.21)) ;
#147070=CARTESIAN_POINT('Origin',(-0.899999999999999,-1.9,-3.21)) ;
#147071=CARTESIAN_POINT('Origin',(-0.899999999999999,-1.9,-3.21)) ;
#147072=CARTESIAN_POINT('Origin',(-0.899999999999999,0.4,-3.41)) ;
#147073=CARTESIAN_POINT('Origin',(-0.899999999999999,0.6,-3.41)) ;
#147074=CARTESIAN_POINT('Origin',(0.500000000000001,0.4,-3.81)) ;
#147075=CARTESIAN_POINT('Origin',(0.500000000000001,0.4,-4.21)) ;
#147076=CARTESIAN_POINT('',(0.600000000000001,0.4,-4.11)) ;
#147077=CARTESIAN_POINT('Ctrl Pts',(0.595612997216081,0.370705721320404,
-4.1807057213204)) ;
#147078=CARTESIAN_POINT('Ctrl Pts',(0.596180587760892,0.372558268494358,
-4.17885549883217)) ;
#147079=CARTESIAN_POINT('Ctrl Pts',(0.596672461925686,0.374355839771985,
-4.17691417986631)) ;
#147080=CARTESIAN_POINT('Ctrl Pts',(0.599015141889212,0.383869350930066,
-4.16576499365627)) ;
#147081=CARTESIAN_POINT('Ctrl Pts',(0.599609996542525,0.390224332900452,
-4.15497260265412)) ;
#147082=CARTESIAN_POINT('Ctrl Pts',(0.600050586298726,0.398117439141561,
-4.13233105320467)) ;
#147083=CARTESIAN_POINT('Ctrl Pts',(0.600000000000001,0.399999999999999,
-4.12120125063352)) ;
#147084=CARTESIAN_POINT('Ctrl Pts',(0.600000000000001,0.399999999999999,
-4.11)) ;
#147085=CARTESIAN_POINT('',(0.600000000000001,0.4,-3.81)) ;
#147086=CARTESIAN_POINT('Origin',(0.500000000000001,-4.56640444411541E-17,
-3.41)) ;
#147087=CARTESIAN_POINT('',(0.500000000000001,0.394987437106619,-3.51)) ;
#147088=CARTESIAN_POINT('Ctrl Pts',(0.500000000000001,0.394987437106619,
-3.51)) ;
#147089=CARTESIAN_POINT('Ctrl Pts',(0.505940567948953,0.3955844866499,-3.51)) ;
#147090=CARTESIAN_POINT('Ctrl Pts',(0.511931971019142,0.396132036079018,
-3.50946630032796)) ;
#147091=CARTESIAN_POINT('Ctrl Pts',(0.517829015308552,0.396618246075354,
-3.50839779577372)) ;
#147092=CARTESIAN_POINT('Ctrl Pts',(0.522982218721203,0.397043126556053,
-3.50746407015711)) ;
#147093=CARTESIAN_POINT('Ctrl Pts',(0.528062648970231,0.397421319341388,
-3.50612282679706)) ;
#147094=CARTESIAN_POINT('Ctrl Pts',(0.532978106724,0.397751505046071,-3.50440574387663)) ;
#147095=CARTESIAN_POINT('Ctrl Pts',(0.538583536338964,0.398128038182999,
-3.50244763784955)) ;
#147096=CARTESIAN_POINT('Ctrl Pts',(0.544059405914891,0.398447721828295,
-3.49997000831105)) ;
#147097=CARTESIAN_POINT('Ctrl Pts',(0.549268572255782,0.398712331108983,
-3.49702073194289)) ;
#147098=CARTESIAN_POINT('Ctrl Pts',(0.553856850427147,0.398945401221756,
-3.49442298414684)) ;
#147099=CARTESIAN_POINT('Ctrl Pts',(0.558237825069328,0.399135987683843,
-3.49146038497999)) ;
#147100=CARTESIAN_POINT('Ctrl Pts',(0.562333836086213,0.399290378266507,
-3.48819522286417)) ;
#147101=CARTESIAN_POINT('Ctrl Pts',(0.56699032895789,0.399465895042381,
-3.48448326895231)) ;
#147102=CARTESIAN_POINT('Ctrl Pts',(0.571349096493424,0.399597278936107,
-3.4803228064848)) ;
#147103=CARTESIAN_POINT('Ctrl Pts',(0.57529692005671,0.399694832180837,
-3.47580557597935)) ;
#147104=CARTESIAN_POINT('Ctrl Pts',(0.578744263667905,0.399780018245913,
-3.47186101121508)) ;
#147105=CARTESIAN_POINT('Ctrl Pts',(0.581878314560428,0.399839626289636,
-3.46764552184211)) ;
#147106=CARTESIAN_POINT('Ctrl Pts',(0.584648147334855,0.399882153365958,
-3.4632418177073)) ;
#147107=CARTESIAN_POINT('Ctrl Pts',(0.587839270208174,0.399931148788079,
-3.4581683125045)) ;
#147108=CARTESIAN_POINT('Ctrl Pts',(0.590595054415095,0.399958289583404,
-3.45276663624445)) ;
#147109=CARTESIAN_POINT('Ctrl Pts',(0.592838618943107,0.399974357003159,
-3.44716168500939)) ;
#147110=CARTESIAN_POINT('Ctrl Pts',(0.594777336851657,0.399988241245861,
-3.44231831224239)) ;
#147111=CARTESIAN_POINT('Ctrl Pts',(0.59633405150619,0.399993946552814,
-3.43732416622712)) ;
#147112=CARTESIAN_POINT('Ctrl Pts',(0.597488309822309,0.39999684570125,
-3.43227171856839)) ;
#147113=CARTESIAN_POINT('Ctrl Pts',(0.598804024094397,0.400000150378306,
-3.42651254196058)) ;
#147114=CARTESIAN_POINT('Ctrl Pts',(0.599612685195426,0.399999963509465,
-3.42060284389063)) ;
#147115=CARTESIAN_POINT('Ctrl Pts',(0.599890230999718,0.399999993975383,
-3.41468420226113)) ;
#147116=CARTESIAN_POINT('Ctrl Pts',(0.599963464549399,0.400000002014155,
-3.41312250278986)) ;
#147117=CARTESIAN_POINT('Ctrl Pts',(0.600000000000001,0.399999999999999,
-3.4115602215092)) ;
#147118=CARTESIAN_POINT('Ctrl Pts',(0.600000000000001,0.399999999999999,
-3.41)) ;
#147119=CARTESIAN_POINT('',(0.600000000000001,0.299999999999999,-3.41)) ;
#147120=CARTESIAN_POINT('Ctrl Pts',(0.500000000000001,0.394987437106619,
-3.51)) ;
#147121=CARTESIAN_POINT('Ctrl Pts',(0.500454935589683,0.395033159853733,
-3.51)) ;
#147122=CARTESIAN_POINT('Ctrl Pts',(0.500909898680391,0.395078570329052,
-3.50999689549113)) ;
#147123=CARTESIAN_POINT('Ctrl Pts',(0.502892456245154,0.395275075889088,
-3.50996983394194)) ;
#147124=CARTESIAN_POINT('Ctrl Pts',(0.504418747482365,0.395422812032198,
-3.50991398542099)) ;
#147125=CARTESIAN_POINT('Ctrl Pts',(0.508462199543374,0.395804395682036,
-3.50967328105664)) ;
#147126=CARTESIAN_POINT('Ctrl Pts',(0.51097495334332,0.396031485023319,
-3.50942793914505)) ;
#147127=CARTESIAN_POINT('Ctrl Pts',(0.521160739721337,0.396903453186241,
-3.50804279449155)) ;
#147128=CARTESIAN_POINT('Ctrl Pts',(0.528708678528462,0.397444933153163,
-3.50610421770467)) ;
#147129=CARTESIAN_POINT('Ctrl Pts',(0.545943206358151,0.398105551684111,
-3.49946463945111)) ;
#147130=CARTESIAN_POINT('Ctrl Pts',(0.555229535466881,0.397987646678422,
-3.49403535883592)) ;
#147131=CARTESIAN_POINT('Ctrl Pts',(0.571394604995817,0.395490482808027,
-3.4807755133638)) ;
#147132=CARTESIAN_POINT('Ctrl Pts',(0.578055313702888,0.393198948698317,
-3.47324074563169)) ;
#147133=CARTESIAN_POINT('Ctrl Pts',(0.588559132202554,0.385442756729274,
-3.45739223398396)) ;
#147134=CARTESIAN_POINT('Ctrl Pts',(0.592167355639999,0.380240075126842,
-3.44954826560675)) ;
#147135=CARTESIAN_POINT('Ctrl Pts',(0.597496615531132,0.365892753466902,
-3.43392552179521)) ;
#147136=CARTESIAN_POINT('Ctrl Pts',(0.598734255154207,0.35666056430058,
-3.42677274172686)) ;
#147137=CARTESIAN_POINT('Ctrl Pts',(0.600012754681691,0.335223914398476,
-3.41558230586558)) ;
#147138=CARTESIAN_POINT('Ctrl Pts',(0.59999390055981,0.322655037091807,
-3.41166151936557)) ;
#147139=CARTESIAN_POINT('Ctrl Pts',(0.600000296204999,0.306106913582338,
-3.41013962634704)) ;
#147140=CARTESIAN_POINT('Ctrl Pts',(0.600000000000001,0.303050992413427,
-3.41)) ;
#147141=CARTESIAN_POINT('Ctrl Pts',(0.600000000000001,0.299999999999999,
-3.41)) ;
#147142=CARTESIAN_POINT('',(0.600000000000001,-2.3980000991444E-17,-3.41)) ;
#147143=CARTESIAN_POINT('Origin',(0.500000000000001,-1.9,-3.41)) ;
#147144=CARTESIAN_POINT('Origin',(0.600000000000001,-1.9,-3.21)) ;
#147145=CARTESIAN_POINT('Origin',(0.500000000000001,-1.9,-3.21)) ;
#147146=CARTESIAN_POINT('Origin',(-0.899999999999999,-1.9,-2.435)) ;
#147147=CARTESIAN_POINT('Origin',(-0.899999999999999,-1.9,-2.535)) ;
#147148=CARTESIAN_POINT('Origin',(-0.899999999999999,0.6,-3.31)) ;
#147149=CARTESIAN_POINT('Origin',(-0.899999999999999,0.6,-4.21)) ;
#147150=CARTESIAN_POINT('Origin',(0.600000000000001,0.4,-4.21)) ;
#147151=CARTESIAN_POINT('Origin',(0.500000000000001,0.4,-4.21)) ;
#147152=CARTESIAN_POINT('Origin',(-0.899999999999999,0.4,-4.21)) ;
#147153=CARTESIAN_POINT('Origin',(0.500000000000001,0.4,-4.21)) ;
#147154=CARTESIAN_POINT('Origin',(0.500000000000001,-1.9,-3.21)) ;
#147155=CARTESIAN_POINT('Origin',(0.500000000000001,-2.1,-3.21)) ;
#147156=CARTESIAN_POINT('Origin',(-0.899999999999999,-1.9,-2.535)) ;
#147157=CARTESIAN_POINT('Origin',(-1.1,-1.9,-2.535)) ;
#147158=CARTESIAN_POINT('Origin',(-0.899999999999999,-2.1,-2.535)) ;
#147159=CARTESIAN_POINT('Origin',(-0.899999999999999,0.4,-4.21)) ;
#147160=CARTESIAN_POINT('Origin',(-0.899999999999999,0.4,-4.41)) ;
#147161=CARTESIAN_POINT('Origin',(0.500000000000001,-2.1,-3.81)) ;
#147162=CARTESIAN_POINT('Origin',(0.500000000000001,-2.1,-2.535)) ;
#147163=CARTESIAN_POINT('Origin',(0.600000000000001,-2.1,-2.535)) ;
#147164=CARTESIAN_POINT('Origin',(0.500000000000001,-2.1,-2.535)) ;
#147165=CARTESIAN_POINT('Origin',(-1.1,-4.42727195005761E-17,-2.535)) ;
#147166=CARTESIAN_POINT('',(-1.1,1.15,-2.435)) ;
#147167=CARTESIAN_POINT('',(-1.1,1.25,-2.435)) ;
#147168=CARTESIAN_POINT('Origin',(-1.1,1.15,-2.535)) ;
#147169=CARTESIAN_POINT('Origin',(-0.899999999999999,0.5,-4.41)) ;
#147170=CARTESIAN_POINT('Origin',(-0.899999999999999,-1.9,-4.41)) ;
#147171=CARTESIAN_POINT('Origin',(0.600000000000001,-1.9,-4.41)) ;
#147172=CARTESIAN_POINT('Origin',(0.500000000000001,-1.9,-4.41)) ;
#147173=CARTESIAN_POINT('Origin',(-0.899999999999999,-1.9,-4.41)) ;
#147174=CARTESIAN_POINT('Origin',(0.500000000000001,-1.9,-4.41)) ;
#147175=CARTESIAN_POINT('Origin',(0.500000000000001,-2.1,-4.41)) ;
#147176=CARTESIAN_POINT('Origin',(0.500000000000001,-2.1,-2.535)) ;
#147177=CARTESIAN_POINT('Origin',(0.500000000000001,-2.1,-2.535)) ;
#147178=CARTESIAN_POINT('Origin',(-1.1,-2.9,-2.335)) ;
#147179=CARTESIAN_POINT('Origin',(-1.1,-2.9,-2.335)) ;
#147180=CARTESIAN_POINT('Origin',(-1.1,-2.9,-2.335)) ;
#147181=CARTESIAN_POINT('Origin',(-1.1,1.25,-2.335)) ;
#147182=CARTESIAN_POINT('Origin',(-1.1,1.15,-2.335)) ;
#147183=CARTESIAN_POINT('Origin',(-1.1,1.15,-2.535)) ;
#147184=CARTESIAN_POINT('',(-1.1,1.25,-2.535)) ;
#147185=CARTESIAN_POINT('Origin',(-1.1,1.15,-2.535)) ;
#147186=CARTESIAN_POINT('Origin',(-1.1,1.15,-2.535)) ;
#147187=CARTESIAN_POINT('Origin',(-0.899999999999999,-1.9,-4.41)) ;
#147188=CARTESIAN_POINT('Origin',(-0.899999999999999,-1.9,-4.41)) ;
#147189=CARTESIAN_POINT('Origin',(0.500000000000001,-2.1,-3.81)) ;
#147190=CARTESIAN_POINT('Origin',(0.500000000000001,-2.1,-5.085)) ;
#147191=CARTESIAN_POINT('Origin',(0.500000000000001,1.36481920536411E-16,
-2.535)) ;
#147192=CARTESIAN_POINT('Origin',(0.500000000000001,-2.9,-2.535)) ;
#147193=CARTESIAN_POINT('Origin',(-0.999999999999999,-2.9,-2.335)) ;
#147194=CARTESIAN_POINT('Origin',(0.500000000000001,-2.9,-2.335)) ;
#147195=CARTESIAN_POINT('Origin',(-1.1,1.15,-2.535)) ;
#147196=CARTESIAN_POINT('Origin',(-1.1,1.35,-2.535)) ;
#147197=CARTESIAN_POINT('Origin',(-1.1,1.15,-3.81)) ;
#147198=CARTESIAN_POINT('',(-1.1,1.25,-5.085)) ;
#147199=CARTESIAN_POINT('',(-1.1,1.25,-5.185)) ;
#147200=CARTESIAN_POINT('Origin',(-1.1,1.15,-5.085)) ;
#147201=CARTESIAN_POINT('Origin',(-0.899999999999999,-1.9,-4.31)) ;
#147202=CARTESIAN_POINT('Origin',(-0.899999999999999,-1.9,-5.085)) ;
#147203=CARTESIAN_POINT('Origin',(-0.999999999999999,-2.1,-5.085)) ;
#147204=CARTESIAN_POINT('Origin',(0.500000000000001,-2.1,-5.085)) ;
#147205=CARTESIAN_POINT('Origin',(-0.899999999999999,-2.1,-5.085)) ;
#147206=CARTESIAN_POINT('Origin',(0.500000000000001,-2.1,-5.085)) ;
#147207=CARTESIAN_POINT('Origin',(0.500000000000001,-2.1,-5.085)) ;
#147208=CARTESIAN_POINT('Origin',(0.500000000000001,-2.9,-2.535)) ;
#147209=CARTESIAN_POINT('Origin',(0.700000000000002,-2.9,-2.535)) ;
#147210=CARTESIAN_POINT('Origin',(-1.1,1.35,-5.185)) ;
#147211=CARTESIAN_POINT('Origin',(-1.1,1.35,-5.085)) ;
#147212=CARTESIAN_POINT('Origin',(-1.1,1.15,-5.085)) ;
#147213=CARTESIAN_POINT('',(-1.1,1.15,-5.185)) ;
#147214=CARTESIAN_POINT('Origin',(-1.1,1.15,-5.085)) ;
#147215=CARTESIAN_POINT('Origin',(-1.1,1.15,-5.085)) ;
#147216=CARTESIAN_POINT('Origin',(-0.899999999999999,-1.9,-5.085)) ;
#147217=CARTESIAN_POINT('Origin',(-1.1,-1.9,-5.085)) ;
#147218=CARTESIAN_POINT('Origin',(0.500000000000001,-5.86744705109801E-17,
-5.085)) ;
#147219=CARTESIAN_POINT('Origin',(0.500000000000001,-2.9,-5.085)) ;
#147220=CARTESIAN_POINT('Origin',(0.700000000000002,-2.9,-3.81)) ;
#147221=CARTESIAN_POINT('Origin',(0.700000000000002,-2.9,-5.085)) ;
#147222=CARTESIAN_POINT('Origin',(-1.1,1.15,-5.085)) ;
#147223=CARTESIAN_POINT('Origin',(-1.1,1.15,-5.285)) ;
#147224=CARTESIAN_POINT('Origin',(-1.1,-2.39429110547967E-16,-5.085)) ;
#147225=CARTESIAN_POINT('',(-1.1,1.25,-5.185)) ;
#147226=CARTESIAN_POINT('Origin',(0.500000000000001,-2.9,-5.085)) ;
#147227=CARTESIAN_POINT('Origin',(0.500000000000001,-2.9,-5.285)) ;
#147228=CARTESIAN_POINT('Origin',(-1.1,1.25,-5.285)) ;
#147229=CARTESIAN_POINT('Origin',(-1.1,-2.9,-5.285)) ;
#147230=CARTESIAN_POINT('Origin',(-1.1,-2.9,-5.285)) ;
#147231=CARTESIAN_POINT('Origin',(-1.1,-2.9,-5.285)) ;
#147232=CARTESIAN_POINT('Origin',(-1.1,-2.9,-5.285)) ;
#147233=CARTESIAN_POINT('Origin',(1.5,1.9,-3.21)) ;
#147234=CARTESIAN_POINT('Origin',(1.5,1.9,-5.36)) ;
#147235=CARTESIAN_POINT('Origin',(1.5,1.9,-4.41)) ;
#147236=CARTESIAN_POINT('Origin',(1.5,2.1,-4.41)) ;
#147237=CARTESIAN_POINT('Origin',(1.5,2.1,-4.21)) ;
#147238=CARTESIAN_POINT('Origin',(1.5,1.9,-5.36)) ;
#147239=CARTESIAN_POINT('Origin',(1.5,1.9,-5.36)) ;
#147240=CARTESIAN_POINT('Origin',(1.5,2.1,-4.21)) ;
#147241=CARTESIAN_POINT('Origin',(1.5,2.4,-4.21)) ;
#147242=CARTESIAN_POINT('Origin',(1.5,2.1,-5.36)) ;
#147243=CARTESIAN_POINT('Origin',(1.5,-2.15,-5.36)) ;
#147244=CARTESIAN_POINT('Origin',(1.5,2.4,-4.41)) ;
#147245=CARTESIAN_POINT('Origin',(1.5,2.6,-4.41)) ;
#147246=CARTESIAN_POINT('Origin',(1.5,-2.15,-5.36)) ;
#147247=CARTESIAN_POINT('Origin',(1.5,-2.15,-5.36)) ;
#147248=CARTESIAN_POINT('Origin',(1.5,2.6,-3.21)) ;
#147249=CARTESIAN_POINT('Origin',(1.5,2.6,-4.51857864376269)) ;
#147250=CARTESIAN_POINT('Origin',(1.5,-2.15,-3.21)) ;
#147251=CARTESIAN_POINT('Origin',(1.5,-2.15,-4.71311959340942)) ;
#147252=CARTESIAN_POINT('Origin',(1.5,2.6,-4.51857864376269)) ;
#147253=CARTESIAN_POINT('Origin',(1.5,2.6,-4.51857864376269)) ;
#147254=CARTESIAN_POINT('Origin',(1.5,-2.15,-4.71311959340942)) ;
#147255=CARTESIAN_POINT('Origin',(1.5,-2.15,-4.71311959340942)) ;
#147256=CARTESIAN_POINT('Origin',(1.5,1.69571067811865,-3.61428932188135)) ;
#147257=CARTESIAN_POINT('Origin',(1.5,3.15,-5.06857864376269)) ;
#147258=CARTESIAN_POINT('Origin',(1.5,-3.65625,-3.81)) ;
#147259=CARTESIAN_POINT('Origin',(1.5,-2.15,-2.90688040659058)) ;
#147260=CARTESIAN_POINT('Origin',(1.5,3.15,-5.06857864376269)) ;
#147261=CARTESIAN_POINT('Origin',(1.5,3.15,-5.06857864376269)) ;
#147262=CARTESIAN_POINT('Origin',(1.5,-2.15,-2.90688040659058)) ;
#147263=CARTESIAN_POINT('Origin',(1.5,-2.15,-2.90688040659058)) ;
#147264=CARTESIAN_POINT('Origin',(1.5,3.15,-3.21)) ;
#147265=CARTESIAN_POINT('Origin',(1.5,-2.15,-3.21)) ;
#147266=CARTESIAN_POINT('Origin',(1.5,-2.15,-2.26)) ;
#147267=CARTESIAN_POINT('Origin',(1.5,-2.15,-2.26)) ;
#147268=CARTESIAN_POINT('Origin',(1.5,-2.15,-2.26)) ;
#147269=CARTESIAN_POINT('Origin',(1.5,2.29571067811866,-3.40571067811866)) ;
#147270=CARTESIAN_POINT('Origin',(1.5,2.6,-3.10142135623731)) ;
#147271=CARTESIAN_POINT('Origin',(1.5,2.1,-2.26)) ;
#147272=CARTESIAN_POINT('Origin',(1.5,1.9,-2.26)) ;
#147273=CARTESIAN_POINT('Origin',(1.5,2.6,-3.10142135623731)) ;
#147274=CARTESIAN_POINT('Origin',(1.5,2.6,-3.10142135623731)) ;
#147275=CARTESIAN_POINT('Origin',(1.5,1.9,-2.26)) ;
#147276=CARTESIAN_POINT('Origin',(1.5,1.9,-2.26)) ;
#147277=CARTESIAN_POINT('Origin',(1.5,2.6,-3.21)) ;
#147278=CARTESIAN_POINT('Origin',(1.5,2.6,-3.21)) ;
#147279=CARTESIAN_POINT('Origin',(1.5,1.9,-3.21)) ;
#147280=CARTESIAN_POINT('Origin',(1.5,1.9,-3.21)) ;
#147281=CARTESIAN_POINT('Origin',(1.5,2.4,-3.21)) ;
#147282=CARTESIAN_POINT('Origin',(1.5,2.4,-3.41)) ;
#147283=CARTESIAN_POINT('Origin',(1.5,2.1,-3.21)) ;
#147284=CARTESIAN_POINT('Origin',(1.5,2.1,-3.41)) ;
#147285=CARTESIAN_POINT('Origin',(1.5,2.1,-3.41)) ;
#147286=CARTESIAN_POINT('Origin',(7.9,2.1,-34.89)) ;
#147287=CARTESIAN_POINT('Origin',(7.9,2.4,-34.89)) ;
#147288=CARTESIAN_POINT('Origin',(7.9,2.1,-34.89)) ;
#147289=CARTESIAN_POINT('Origin',(7.9,2.4,-34.89)) ;
#147290=CARTESIAN_POINT('Origin',(7.9,2.4,-34.89)) ;
#147291=CARTESIAN_POINT('Origin',(7.9,2.1,-34.89)) ;
#147292=CARTESIAN_POINT('Origin',(7.9,2.1,-34.89)) ;
#147293=CARTESIAN_POINT('Origin',(7.9,2.4,-34.89)) ;
#147294=CARTESIAN_POINT('Origin',(7.9,2.4,-34.9985786437627)) ;
#147295=CARTESIAN_POINT('Origin',(7.9,2.1,-34.89)) ;
#147296=CARTESIAN_POINT('Origin',(7.9,2.1,-35.84)) ;
#147297=CARTESIAN_POINT('Origin',(7.9,2.6,-34.9985786437627)) ;
#147298=CARTESIAN_POINT('Origin',(7.9,2.45857864376269,-35.14)) ;
#147299=CARTESIAN_POINT('Origin',(7.9,1.9,-35.84)) ;
#147300=CARTESIAN_POINT('Origin',(7.9,1.9,-36.04)) ;
#147301=CARTESIAN_POINT('Origin',(7.9,2.45857864376269,-35.14)) ;
#147302=CARTESIAN_POINT('Origin',(7.9,1.9,-36.04)) ;
#147303=CARTESIAN_POINT('Origin',(7.9,-2.15,-36.04)) ;
#147304=CARTESIAN_POINT('Origin',(7.9,-2.15,-35.84)) ;
#147305=CARTESIAN_POINT('Origin',(7.9,-2.35,-35.84)) ;
#147306=CARTESIAN_POINT('Origin',(7.9,3.35,-35.5485786437627)) ;
#147307=CARTESIAN_POINT('Origin',(7.9,3.35,-33.0314213562373)) ;
#147308=CARTESIAN_POINT('Origin',(7.9,-2.35,-35.1931195934094)) ;
#147309=CARTESIAN_POINT('Origin',(7.9,-2.35,-35.1931195934094)) ;
#147310=CARTESIAN_POINT('Origin',(7.9,3.15,-33.0314213562373)) ;
#147311=CARTESIAN_POINT('Origin',(7.9,3.00857864376269,-32.89)) ;
#147312=CARTESIAN_POINT('Origin',(7.9,-2.15,-35.1931195934094)) ;
#147313=CARTESIAN_POINT('Origin',(7.9,-2.32153024911032,-35.0902732340176)) ;
#147314=CARTESIAN_POINT('Origin',(7.9,3.00857864376269,-32.89)) ;
#147315=CARTESIAN_POINT('Origin',(7.9,2.45857864376269,-33.44)) ;
#147316=CARTESIAN_POINT('Origin',(7.9,-3.65625,-34.29)) ;
#147317=CARTESIAN_POINT('Origin',(7.9,-2.32153024911033,-33.4897267659824)) ;
#147318=CARTESIAN_POINT('Origin',(7.9,2.6,-33.5814213562373)) ;
#147319=CARTESIAN_POINT('Origin',(7.9,2.4,-33.5814213562373)) ;
#147320=CARTESIAN_POINT('Origin',(7.9,-2.15,-33.3868804065906)) ;
#147321=CARTESIAN_POINT('Origin',(7.9,-2.35,-33.3868804065906)) ;
#147322=CARTESIAN_POINT('Origin',(7.9,2.4,-33.5814213562373)) ;
#147323=CARTESIAN_POINT('Origin',(7.9,2.4,-33.69)) ;
#147324=CARTESIAN_POINT('Origin',(7.9,-2.35,-32.74)) ;
#147325=CARTESIAN_POINT('Origin',(7.9,-2.35,-32.74)) ;
#147326=CARTESIAN_POINT('Origin',(7.9,2.4,-33.69)) ;
#147327=CARTESIAN_POINT('Origin',(7.9,2.4,-33.69)) ;
#147328=CARTESIAN_POINT('Origin',(7.9,-2.15,-32.74)) ;
#147329=CARTESIAN_POINT('Origin',(7.9,-2.15,-32.54)) ;
#147330=CARTESIAN_POINT('Origin',(7.9,2.4,-33.69)) ;
#147331=CARTESIAN_POINT('Origin',(7.9,2.1,-33.69)) ;
#147332=CARTESIAN_POINT('Origin',(7.9,1.9,-32.54)) ;
#147333=CARTESIAN_POINT('Origin',(7.9,1.9,-32.54)) ;
#147334=CARTESIAN_POINT('Origin',(7.9,2.1,-33.69)) ;
#147335=CARTESIAN_POINT('Origin',(7.9,2.1,-33.69)) ;
#147336=CARTESIAN_POINT('Origin',(7.9,1.9,-32.74)) ;
#147337=CARTESIAN_POINT('Origin',(7.9,2.1,-32.74)) ;
#147338=CARTESIAN_POINT('Origin',(7.9,2.1,-32.74)) ;
#147339=CARTESIAN_POINT('Origin',(7.9,2.1,-31.08)) ;
#147340=CARTESIAN_POINT('Origin',(7.9,2.4,-31.08)) ;
#147341=CARTESIAN_POINT('Origin',(7.9,2.1,-31.08)) ;
#147342=CARTESIAN_POINT('Origin',(7.9,2.4,-31.08)) ;
#147343=CARTESIAN_POINT('Origin',(7.9,2.4,-31.08)) ;
#147344=CARTESIAN_POINT('Origin',(7.9,2.1,-31.08)) ;
#147345=CARTESIAN_POINT('Origin',(7.9,2.1,-31.08)) ;
#147346=CARTESIAN_POINT('Origin',(7.9,2.4,-31.08)) ;
#147347=CARTESIAN_POINT('Origin',(7.9,2.4,-31.1885786437627)) ;
#147348=CARTESIAN_POINT('Origin',(7.9,2.1,-31.08)) ;
#147349=CARTESIAN_POINT('Origin',(7.9,2.1,-32.03)) ;
#147350=CARTESIAN_POINT('Origin',(7.9,2.6,-31.1885786437627)) ;
#147351=CARTESIAN_POINT('Origin',(7.9,2.45857864376269,-31.33)) ;
#147352=CARTESIAN_POINT('Origin',(7.9,1.9,-32.03)) ;
#147353=CARTESIAN_POINT('Origin',(7.9,1.9,-32.23)) ;
#147354=CARTESIAN_POINT('Origin',(7.9,2.45857864376269,-31.33)) ;
#147355=CARTESIAN_POINT('Origin',(7.9,1.9,-32.23)) ;
#147356=CARTESIAN_POINT('Origin',(7.9,-2.15,-32.23)) ;
#147357=CARTESIAN_POINT('Origin',(7.9,-2.15,-32.03)) ;
#147358=CARTESIAN_POINT('Origin',(7.9,-2.35,-32.03)) ;
#147359=CARTESIAN_POINT('Origin',(7.9,3.35,-31.7385786437627)) ;
#147360=CARTESIAN_POINT('Origin',(7.9,3.35,-29.2214213562373)) ;
#147361=CARTESIAN_POINT('Origin',(7.9,-2.35,-31.3831195934094)) ;
#147362=CARTESIAN_POINT('Origin',(7.9,-2.35,-31.3831195934094)) ;
#147363=CARTESIAN_POINT('Origin',(7.9,3.15,-29.2214213562373)) ;
#147364=CARTESIAN_POINT('Origin',(7.9,3.00857864376269,-29.08)) ;
#147365=CARTESIAN_POINT('Origin',(7.9,-2.15,-31.3831195934094)) ;
#147366=CARTESIAN_POINT('Origin',(7.9,-2.32153024911032,-31.2802732340176)) ;
#147367=CARTESIAN_POINT('Origin',(7.9,3.00857864376269,-29.08)) ;
#147368=CARTESIAN_POINT('Origin',(7.9,2.45857864376269,-29.63)) ;
#147369=CARTESIAN_POINT('Origin',(7.9,-3.65625,-30.48)) ;
#147370=CARTESIAN_POINT('Origin',(7.9,-2.32153024911032,-29.6797267659824)) ;
#147371=CARTESIAN_POINT('Origin',(7.9,2.6,-29.7714213562373)) ;
#147372=CARTESIAN_POINT('Origin',(7.9,2.4,-29.7714213562373)) ;
#147373=CARTESIAN_POINT('Origin',(7.9,-2.15,-29.5768804065906)) ;
#147374=CARTESIAN_POINT('Origin',(7.9,-2.35,-29.5768804065906)) ;
#147375=CARTESIAN_POINT('Origin',(7.9,2.4,-29.7714213562373)) ;
#147376=CARTESIAN_POINT('Origin',(7.9,2.4,-29.88)) ;
#147377=CARTESIAN_POINT('Origin',(7.9,-2.35,-28.93)) ;
#147378=CARTESIAN_POINT('Origin',(7.9,-2.35,-28.93)) ;
#147379=CARTESIAN_POINT('Origin',(7.9,2.4,-29.88)) ;
#147380=CARTESIAN_POINT('Origin',(7.9,2.4,-29.88)) ;
#147381=CARTESIAN_POINT('Origin',(7.9,-2.15,-28.93)) ;
#147382=CARTESIAN_POINT('Origin',(7.9,-2.15,-28.73)) ;
#147383=CARTESIAN_POINT('Origin',(7.9,2.4,-29.88)) ;
#147384=CARTESIAN_POINT('Origin',(7.9,2.1,-29.88)) ;
#147385=CARTESIAN_POINT('Origin',(7.9,1.9,-28.73)) ;
#147386=CARTESIAN_POINT('Origin',(7.9,1.9,-28.73)) ;
#147387=CARTESIAN_POINT('Origin',(7.9,2.1,-29.88)) ;
#147388=CARTESIAN_POINT('Origin',(7.9,2.1,-29.88)) ;
#147389=CARTESIAN_POINT('Origin',(7.9,1.9,-28.93)) ;
#147390=CARTESIAN_POINT('Origin',(7.9,2.1,-28.93)) ;
#147391=CARTESIAN_POINT('Origin',(7.9,2.1,-28.93)) ;
#147392=CARTESIAN_POINT('Origin',(7.9,2.1,-27.27)) ;
#147393=CARTESIAN_POINT('Origin',(7.9,2.4,-27.27)) ;
#147394=CARTESIAN_POINT('Origin',(7.9,2.1,-27.27)) ;
#147395=CARTESIAN_POINT('Origin',(7.9,2.4,-27.27)) ;
#147396=CARTESIAN_POINT('Origin',(7.9,2.4,-27.27)) ;
#147397=CARTESIAN_POINT('Origin',(7.9,2.1,-27.27)) ;
#147398=CARTESIAN_POINT('Origin',(7.9,2.1,-27.27)) ;
#147399=CARTESIAN_POINT('Origin',(7.9,2.4,-27.27)) ;
#147400=CARTESIAN_POINT('Origin',(7.9,2.4,-27.3785786437627)) ;
#147401=CARTESIAN_POINT('Origin',(7.9,2.1,-27.27)) ;
#147402=CARTESIAN_POINT('Origin',(7.9,2.1,-28.22)) ;
#147403=CARTESIAN_POINT('Origin',(7.9,2.6,-27.3785786437627)) ;
#147404=CARTESIAN_POINT('Origin',(7.9,2.45857864376269,-27.52)) ;
#147405=CARTESIAN_POINT('Origin',(7.9,1.9,-28.22)) ;
#147406=CARTESIAN_POINT('Origin',(7.9,1.9,-28.42)) ;
#147407=CARTESIAN_POINT('Origin',(7.9,2.45857864376269,-27.52)) ;
#147408=CARTESIAN_POINT('Origin',(7.9,1.9,-28.42)) ;
#147409=CARTESIAN_POINT('Origin',(7.9,-2.15,-28.42)) ;
#147410=CARTESIAN_POINT('Origin',(7.9,-2.15,-28.22)) ;
#147411=CARTESIAN_POINT('Origin',(7.9,-2.35,-28.22)) ;
#147412=CARTESIAN_POINT('Origin',(7.9,3.35,-27.9285786437627)) ;
#147413=CARTESIAN_POINT('Origin',(7.9,3.35,-25.4114213562373)) ;
#147414=CARTESIAN_POINT('Origin',(7.9,-2.35,-27.5731195934094)) ;
#147415=CARTESIAN_POINT('Origin',(7.9,-2.35,-27.5731195934094)) ;
#147416=CARTESIAN_POINT('Origin',(7.9,3.15,-25.4114213562373)) ;
#147417=CARTESIAN_POINT('Origin',(7.9,3.00857864376269,-25.27)) ;
#147418=CARTESIAN_POINT('Origin',(7.9,-2.15,-27.5731195934094)) ;
#147419=CARTESIAN_POINT('Origin',(7.9,-2.32153024911032,-27.4702732340176)) ;
#147420=CARTESIAN_POINT('Origin',(7.9,3.00857864376269,-25.27)) ;
#147421=CARTESIAN_POINT('Origin',(7.9,2.45857864376269,-25.82)) ;
#147422=CARTESIAN_POINT('Origin',(7.9,-3.65625,-26.67)) ;
#147423=CARTESIAN_POINT('Origin',(7.9,-2.32153024911032,-25.8697267659824)) ;
#147424=CARTESIAN_POINT('Origin',(7.9,2.6,-25.9614213562373)) ;
#147425=CARTESIAN_POINT('Origin',(7.9,2.4,-25.9614213562373)) ;
#147426=CARTESIAN_POINT('Origin',(7.9,-2.15,-25.7668804065906)) ;
#147427=CARTESIAN_POINT('Origin',(7.9,-2.35,-25.7668804065906)) ;
#147428=CARTESIAN_POINT('Origin',(7.9,2.4,-25.9614213562373)) ;
#147429=CARTESIAN_POINT('Origin',(7.9,2.4,-26.07)) ;
#147430=CARTESIAN_POINT('Origin',(7.9,-2.35,-25.12)) ;
#147431=CARTESIAN_POINT('Origin',(7.9,-2.35,-25.12)) ;
#147432=CARTESIAN_POINT('Origin',(7.9,2.4,-26.07)) ;
#147433=CARTESIAN_POINT('Origin',(7.9,2.4,-26.07)) ;
#147434=CARTESIAN_POINT('Origin',(7.9,-2.15,-25.12)) ;
#147435=CARTESIAN_POINT('Origin',(7.9,-2.15,-24.92)) ;
#147436=CARTESIAN_POINT('Origin',(7.9,2.4,-26.07)) ;
#147437=CARTESIAN_POINT('Origin',(7.9,2.1,-26.07)) ;
#147438=CARTESIAN_POINT('Origin',(7.9,1.9,-24.92)) ;
#147439=CARTESIAN_POINT('Origin',(7.9,1.9,-24.92)) ;
#147440=CARTESIAN_POINT('Origin',(7.9,2.1,-26.07)) ;
#147441=CARTESIAN_POINT('Origin',(7.9,2.1,-26.07)) ;
#147442=CARTESIAN_POINT('Origin',(7.9,1.9,-25.12)) ;
#147443=CARTESIAN_POINT('Origin',(7.9,2.1,-25.12)) ;
#147444=CARTESIAN_POINT('Origin',(7.9,2.1,-25.12)) ;
#147445=CARTESIAN_POINT('Origin',(7.9,2.1,-23.46)) ;
#147446=CARTESIAN_POINT('Origin',(7.9,2.4,-23.46)) ;
#147447=CARTESIAN_POINT('Origin',(7.9,2.1,-23.46)) ;
#147448=CARTESIAN_POINT('Origin',(7.9,2.4,-23.46)) ;
#147449=CARTESIAN_POINT('Origin',(7.9,2.4,-23.46)) ;
#147450=CARTESIAN_POINT('Origin',(7.9,2.1,-23.46)) ;
#147451=CARTESIAN_POINT('Origin',(7.9,2.1,-23.46)) ;
#147452=CARTESIAN_POINT('Origin',(7.9,2.4,-23.46)) ;
#147453=CARTESIAN_POINT('Origin',(7.9,2.4,-23.5685786437627)) ;
#147454=CARTESIAN_POINT('Origin',(7.9,2.1,-23.46)) ;
#147455=CARTESIAN_POINT('Origin',(7.9,2.1,-24.41)) ;
#147456=CARTESIAN_POINT('Origin',(7.9,2.6,-23.5685786437627)) ;
#147457=CARTESIAN_POINT('Origin',(7.9,2.45857864376269,-23.71)) ;
#147458=CARTESIAN_POINT('Origin',(7.9,1.9,-24.41)) ;
#147459=CARTESIAN_POINT('Origin',(7.9,1.9,-24.61)) ;
#147460=CARTESIAN_POINT('Origin',(7.9,2.45857864376269,-23.71)) ;
#147461=CARTESIAN_POINT('Origin',(7.9,1.9,-24.61)) ;
#147462=CARTESIAN_POINT('Origin',(7.9,-2.15,-24.61)) ;
#147463=CARTESIAN_POINT('Origin',(7.9,-2.15,-24.41)) ;
#147464=CARTESIAN_POINT('Origin',(7.9,-2.35,-24.41)) ;
#147465=CARTESIAN_POINT('Origin',(7.9,3.35,-24.1185786437627)) ;
#147466=CARTESIAN_POINT('Origin',(7.9,3.35,-21.6014213562373)) ;
#147467=CARTESIAN_POINT('Origin',(7.9,-2.35,-23.7631195934094)) ;
#147468=CARTESIAN_POINT('Origin',(7.9,-2.35,-23.7631195934094)) ;
#147469=CARTESIAN_POINT('Origin',(7.9,3.15,-21.6014213562373)) ;
#147470=CARTESIAN_POINT('Origin',(7.9,3.00857864376269,-21.46)) ;
#147471=CARTESIAN_POINT('Origin',(7.9,-2.15,-23.7631195934094)) ;
#147472=CARTESIAN_POINT('Origin',(7.9,-2.32153024911032,-23.6602732340176)) ;
#147473=CARTESIAN_POINT('Origin',(7.9,3.00857864376269,-21.46)) ;
#147474=CARTESIAN_POINT('Origin',(7.9,2.45857864376269,-22.01)) ;
#147475=CARTESIAN_POINT('Origin',(7.9,-3.65625,-22.86)) ;
#147476=CARTESIAN_POINT('Origin',(7.9,-2.32153024911032,-22.0597267659824)) ;
#147477=CARTESIAN_POINT('Origin',(7.9,2.6,-22.1514213562373)) ;
#147478=CARTESIAN_POINT('Origin',(7.9,2.4,-22.1514213562373)) ;
#147479=CARTESIAN_POINT('Origin',(7.9,-2.15,-21.9568804065906)) ;
#147480=CARTESIAN_POINT('Origin',(7.9,-2.35,-21.9568804065906)) ;
#147481=CARTESIAN_POINT('Origin',(7.9,2.4,-22.1514213562373)) ;
#147482=CARTESIAN_POINT('Origin',(7.9,2.4,-22.26)) ;
#147483=CARTESIAN_POINT('Origin',(7.9,-2.35,-21.31)) ;
#147484=CARTESIAN_POINT('Origin',(7.9,-2.35,-21.31)) ;
#147485=CARTESIAN_POINT('Origin',(7.9,2.4,-22.26)) ;
#147486=CARTESIAN_POINT('Origin',(7.9,2.4,-22.26)) ;
#147487=CARTESIAN_POINT('Origin',(7.9,-2.15,-21.31)) ;
#147488=CARTESIAN_POINT('Origin',(7.9,-2.15,-21.11)) ;
#147489=CARTESIAN_POINT('Origin',(7.9,2.4,-22.26)) ;
#147490=CARTESIAN_POINT('Origin',(7.9,2.1,-22.26)) ;
#147491=CARTESIAN_POINT('Origin',(7.9,1.9,-21.11)) ;
#147492=CARTESIAN_POINT('Origin',(7.9,1.9,-21.11)) ;
#147493=CARTESIAN_POINT('Origin',(7.9,2.1,-22.26)) ;
#147494=CARTESIAN_POINT('Origin',(7.9,2.1,-22.26)) ;
#147495=CARTESIAN_POINT('Origin',(7.9,1.9,-21.31)) ;
#147496=CARTESIAN_POINT('Origin',(7.9,2.1,-21.31)) ;
#147497=CARTESIAN_POINT('Origin',(7.9,2.1,-21.31)) ;
#147498=CARTESIAN_POINT('Origin',(7.9,2.1,-19.65)) ;
#147499=CARTESIAN_POINT('Origin',(7.9,2.4,-19.65)) ;
#147500=CARTESIAN_POINT('Origin',(7.9,2.1,-19.65)) ;
#147501=CARTESIAN_POINT('Origin',(7.9,2.4,-19.65)) ;
#147502=CARTESIAN_POINT('Origin',(7.9,2.4,-19.65)) ;
#147503=CARTESIAN_POINT('Origin',(7.9,2.1,-19.65)) ;
#147504=CARTESIAN_POINT('Origin',(7.9,2.1,-19.65)) ;
#147505=CARTESIAN_POINT('Origin',(7.9,2.4,-19.65)) ;
#147506=CARTESIAN_POINT('Origin',(7.9,2.4,-19.7585786437627)) ;
#147507=CARTESIAN_POINT('Origin',(7.9,2.1,-19.65)) ;
#147508=CARTESIAN_POINT('Origin',(7.9,2.1,-20.6)) ;
#147509=CARTESIAN_POINT('Origin',(7.9,2.6,-19.7585786437627)) ;
#147510=CARTESIAN_POINT('Origin',(7.9,2.45857864376269,-19.9)) ;
#147511=CARTESIAN_POINT('Origin',(7.9,1.9,-20.6)) ;
#147512=CARTESIAN_POINT('Origin',(7.9,1.9,-20.8)) ;
#147513=CARTESIAN_POINT('Origin',(7.9,2.45857864376269,-19.9)) ;
#147514=CARTESIAN_POINT('Origin',(7.9,1.9,-20.8)) ;
#147515=CARTESIAN_POINT('Origin',(7.9,-2.15,-20.8)) ;
#147516=CARTESIAN_POINT('Origin',(7.9,-2.15,-20.6)) ;
#147517=CARTESIAN_POINT('Origin',(7.9,-2.35,-20.6)) ;
#147518=CARTESIAN_POINT('Origin',(7.9,3.35,-20.3085786437627)) ;
#147519=CARTESIAN_POINT('Origin',(7.9,3.35,-17.7914213562373)) ;
#147520=CARTESIAN_POINT('Origin',(7.9,-2.35,-19.9531195934094)) ;
#147521=CARTESIAN_POINT('Origin',(7.9,-2.35,-19.9531195934094)) ;
#147522=CARTESIAN_POINT('Origin',(7.9,3.15,-17.7914213562373)) ;
#147523=CARTESIAN_POINT('Origin',(7.9,3.00857864376269,-17.65)) ;
#147524=CARTESIAN_POINT('Origin',(7.9,-2.15,-19.9531195934094)) ;
#147525=CARTESIAN_POINT('Origin',(7.9,-2.32153024911032,-19.8502732340176)) ;
#147526=CARTESIAN_POINT('Origin',(7.9,3.00857864376269,-17.65)) ;
#147527=CARTESIAN_POINT('Origin',(7.9,2.45857864376269,-18.2)) ;
#147528=CARTESIAN_POINT('Origin',(7.9,-3.65625,-19.05)) ;
#147529=CARTESIAN_POINT('Origin',(7.9,-2.32153024911032,-18.2497267659824)) ;
#147530=CARTESIAN_POINT('Origin',(7.9,2.6,-18.3414213562373)) ;
#147531=CARTESIAN_POINT('Origin',(7.9,2.4,-18.3414213562373)) ;
#147532=CARTESIAN_POINT('Origin',(7.9,-2.15,-18.1468804065906)) ;
#147533=CARTESIAN_POINT('Origin',(7.9,-2.35,-18.1468804065906)) ;
#147534=CARTESIAN_POINT('Origin',(7.9,2.4,-18.3414213562373)) ;
#147535=CARTESIAN_POINT('Origin',(7.9,2.4,-18.45)) ;
#147536=CARTESIAN_POINT('Origin',(7.9,-2.35,-17.5)) ;
#147537=CARTESIAN_POINT('Origin',(7.9,-2.35,-17.5)) ;
#147538=CARTESIAN_POINT('Origin',(7.9,2.4,-18.45)) ;
#147539=CARTESIAN_POINT('Origin',(7.9,2.4,-18.45)) ;
#147540=CARTESIAN_POINT('Origin',(7.9,-2.15,-17.5)) ;
#147541=CARTESIAN_POINT('Origin',(7.9,-2.15,-17.3)) ;
#147542=CARTESIAN_POINT('Origin',(7.9,2.4,-18.45)) ;
#147543=CARTESIAN_POINT('Origin',(7.9,2.1,-18.45)) ;
#147544=CARTESIAN_POINT('Origin',(7.9,1.9,-17.3)) ;
#147545=CARTESIAN_POINT('Origin',(7.9,1.9,-17.3)) ;
#147546=CARTESIAN_POINT('Origin',(7.9,2.1,-18.45)) ;
#147547=CARTESIAN_POINT('Origin',(7.9,2.1,-18.45)) ;
#147548=CARTESIAN_POINT('Origin',(7.9,1.9,-17.5)) ;
#147549=CARTESIAN_POINT('Origin',(7.9,2.1,-17.5)) ;
#147550=CARTESIAN_POINT('Origin',(7.9,2.1,-17.5)) ;
#147551=CARTESIAN_POINT('Origin',(7.9,2.1,-15.84)) ;
#147552=CARTESIAN_POINT('Origin',(7.9,2.4,-15.84)) ;
#147553=CARTESIAN_POINT('Origin',(7.9,2.1,-15.84)) ;
#147554=CARTESIAN_POINT('Origin',(7.9,2.4,-15.84)) ;
#147555=CARTESIAN_POINT('Origin',(7.9,2.4,-15.84)) ;
#147556=CARTESIAN_POINT('Origin',(7.9,2.1,-15.84)) ;
#147557=CARTESIAN_POINT('Origin',(7.9,2.1,-15.84)) ;
#147558=CARTESIAN_POINT('Origin',(7.9,2.4,-15.84)) ;
#147559=CARTESIAN_POINT('Origin',(7.9,2.4,-15.9485786437627)) ;
#147560=CARTESIAN_POINT('Origin',(7.9,2.1,-15.84)) ;
#147561=CARTESIAN_POINT('Origin',(7.9,2.1,-16.79)) ;
#147562=CARTESIAN_POINT('Origin',(7.9,2.6,-15.9485786437627)) ;
#147563=CARTESIAN_POINT('Origin',(7.9,2.45857864376269,-16.09)) ;
#147564=CARTESIAN_POINT('Origin',(7.9,1.9,-16.79)) ;
#147565=CARTESIAN_POINT('Origin',(7.9,1.9,-16.99)) ;
#147566=CARTESIAN_POINT('Origin',(7.9,2.45857864376269,-16.09)) ;
#147567=CARTESIAN_POINT('Origin',(7.9,1.9,-16.99)) ;
#147568=CARTESIAN_POINT('Origin',(7.9,-2.15,-16.99)) ;
#147569=CARTESIAN_POINT('Origin',(7.9,-2.15,-16.79)) ;
#147570=CARTESIAN_POINT('Origin',(7.9,-2.35,-16.79)) ;
#147571=CARTESIAN_POINT('Origin',(7.9,3.35,-16.4985786437627)) ;
#147572=CARTESIAN_POINT('Origin',(7.9,3.35,-13.9814213562373)) ;
#147573=CARTESIAN_POINT('Origin',(7.9,-2.35,-16.1431195934094)) ;
#147574=CARTESIAN_POINT('Origin',(7.9,-2.35,-16.1431195934094)) ;
#147575=CARTESIAN_POINT('Origin',(7.9,3.15,-13.9814213562373)) ;
#147576=CARTESIAN_POINT('Origin',(7.9,3.00857864376269,-13.84)) ;
#147577=CARTESIAN_POINT('Origin',(7.9,-2.15,-16.1431195934094)) ;
#147578=CARTESIAN_POINT('Origin',(7.9,-2.32153024911032,-16.0402732340176)) ;
#147579=CARTESIAN_POINT('Origin',(7.9,3.00857864376269,-13.84)) ;
#147580=CARTESIAN_POINT('Origin',(7.9,2.45857864376269,-14.39)) ;
#147581=CARTESIAN_POINT('Origin',(7.9,-3.65625,-15.24)) ;
#147582=CARTESIAN_POINT('Origin',(7.9,-2.32153024911032,-14.4397267659824)) ;
#147583=CARTESIAN_POINT('Origin',(7.9,2.6,-14.5314213562373)) ;
#147584=CARTESIAN_POINT('Origin',(7.9,2.4,-14.5314213562373)) ;
#147585=CARTESIAN_POINT('Origin',(7.9,-2.15,-14.3368804065906)) ;
#147586=CARTESIAN_POINT('Origin',(7.9,-2.35,-14.3368804065906)) ;
#147587=CARTESIAN_POINT('Origin',(7.9,2.4,-14.5314213562373)) ;
#147588=CARTESIAN_POINT('Origin',(7.9,2.4,-14.64)) ;
#147589=CARTESIAN_POINT('Origin',(7.9,-2.35,-13.69)) ;
#147590=CARTESIAN_POINT('Origin',(7.9,-2.35,-13.69)) ;
#147591=CARTESIAN_POINT('Origin',(7.9,2.4,-14.64)) ;
#147592=CARTESIAN_POINT('Origin',(7.9,2.4,-14.64)) ;
#147593=CARTESIAN_POINT('Origin',(7.9,-2.15,-13.69)) ;
#147594=CARTESIAN_POINT('Origin',(7.9,-2.15,-13.49)) ;
#147595=CARTESIAN_POINT('Origin',(7.9,2.4,-14.64)) ;
#147596=CARTESIAN_POINT('Origin',(7.9,2.1,-14.64)) ;
#147597=CARTESIAN_POINT('Origin',(7.9,1.9,-13.49)) ;
#147598=CARTESIAN_POINT('Origin',(7.9,1.9,-13.49)) ;
#147599=CARTESIAN_POINT('Origin',(7.9,2.1,-14.64)) ;
#147600=CARTESIAN_POINT('Origin',(7.9,2.1,-14.64)) ;
#147601=CARTESIAN_POINT('Origin',(7.9,1.9,-13.69)) ;
#147602=CARTESIAN_POINT('Origin',(7.9,2.1,-13.69)) ;
#147603=CARTESIAN_POINT('Origin',(7.9,2.1,-13.69)) ;
#147604=CARTESIAN_POINT('Origin',(7.9,2.1,-12.03)) ;
#147605=CARTESIAN_POINT('Origin',(7.9,2.4,-12.03)) ;
#147606=CARTESIAN_POINT('Origin',(7.9,2.1,-12.03)) ;
#147607=CARTESIAN_POINT('Origin',(7.9,2.4,-12.03)) ;
#147608=CARTESIAN_POINT('Origin',(7.9,2.4,-12.03)) ;
#147609=CARTESIAN_POINT('Origin',(7.9,2.1,-12.03)) ;
#147610=CARTESIAN_POINT('Origin',(7.9,2.1,-12.03)) ;
#147611=CARTESIAN_POINT('Origin',(7.9,2.4,-12.03)) ;
#147612=CARTESIAN_POINT('Origin',(7.9,2.4,-12.1385786437627)) ;
#147613=CARTESIAN_POINT('Origin',(7.9,2.1,-12.03)) ;
#147614=CARTESIAN_POINT('Origin',(7.9,2.1,-12.98)) ;
#147615=CARTESIAN_POINT('Origin',(7.9,2.6,-12.1385786437627)) ;
#147616=CARTESIAN_POINT('Origin',(7.9,2.45857864376269,-12.28)) ;
#147617=CARTESIAN_POINT('Origin',(7.9,1.9,-12.98)) ;
#147618=CARTESIAN_POINT('Origin',(7.9,1.9,-13.18)) ;
#147619=CARTESIAN_POINT('Origin',(7.9,2.45857864376269,-12.28)) ;
#147620=CARTESIAN_POINT('Origin',(7.9,1.9,-13.18)) ;
#147621=CARTESIAN_POINT('Origin',(7.9,-2.15,-13.18)) ;
#147622=CARTESIAN_POINT('Origin',(7.9,-2.15,-12.98)) ;
#147623=CARTESIAN_POINT('Origin',(7.9,-2.35,-12.98)) ;
#147624=CARTESIAN_POINT('Origin',(7.9,3.35,-12.6885786437627)) ;
#147625=CARTESIAN_POINT('Origin',(7.9,3.35,-10.1714213562373)) ;
#147626=CARTESIAN_POINT('Origin',(7.9,-2.35,-12.3331195934094)) ;
#147627=CARTESIAN_POINT('Origin',(7.9,-2.35,-12.3331195934094)) ;
#147628=CARTESIAN_POINT('Origin',(7.9,3.15,-10.1714213562373)) ;
#147629=CARTESIAN_POINT('Origin',(7.9,3.00857864376269,-10.03)) ;
#147630=CARTESIAN_POINT('Origin',(7.9,-2.15,-12.3331195934094)) ;
#147631=CARTESIAN_POINT('Origin',(7.9,-2.32153024911032,-12.2302732340176)) ;
#147632=CARTESIAN_POINT('Origin',(7.9,3.00857864376269,-10.03)) ;
#147633=CARTESIAN_POINT('Origin',(7.9,2.45857864376269,-10.58)) ;
#147634=CARTESIAN_POINT('Origin',(7.9,-3.65625,-11.43)) ;
#147635=CARTESIAN_POINT('Origin',(7.9,-2.32153024911032,-10.6297267659824)) ;
#147636=CARTESIAN_POINT('Origin',(7.9,2.6,-10.7214213562373)) ;
#147637=CARTESIAN_POINT('Origin',(7.9,2.4,-10.7214213562373)) ;
#147638=CARTESIAN_POINT('Origin',(7.9,-2.15,-10.5268804065906)) ;
#147639=CARTESIAN_POINT('Origin',(7.9,-2.35,-10.5268804065906)) ;
#147640=CARTESIAN_POINT('Origin',(7.9,2.4,-10.7214213562373)) ;
#147641=CARTESIAN_POINT('Origin',(7.9,2.4,-10.83)) ;
#147642=CARTESIAN_POINT('Origin',(7.9,-2.35,-9.88)) ;
#147643=CARTESIAN_POINT('Origin',(7.9,-2.35,-9.88)) ;
#147644=CARTESIAN_POINT('Origin',(7.9,2.4,-10.83)) ;
#147645=CARTESIAN_POINT('Origin',(7.9,2.4,-10.83)) ;
#147646=CARTESIAN_POINT('Origin',(7.9,-2.15,-9.88)) ;
#147647=CARTESIAN_POINT('Origin',(7.9,-2.15,-9.68)) ;
#147648=CARTESIAN_POINT('Origin',(7.9,2.4,-10.83)) ;
#147649=CARTESIAN_POINT('Origin',(7.9,2.1,-10.83)) ;
#147650=CARTESIAN_POINT('Origin',(7.9,1.9,-9.68)) ;
#147651=CARTESIAN_POINT('Origin',(7.9,1.9,-9.68)) ;
#147652=CARTESIAN_POINT('Origin',(7.9,2.1,-10.83)) ;
#147653=CARTESIAN_POINT('Origin',(7.9,2.1,-10.83)) ;
#147654=CARTESIAN_POINT('Origin',(7.9,1.9,-9.88)) ;
#147655=CARTESIAN_POINT('Origin',(7.9,2.1,-9.88)) ;
#147656=CARTESIAN_POINT('Origin',(7.9,2.1,-9.88)) ;
#147657=CARTESIAN_POINT('Origin',(7.9,2.1,-8.22)) ;
#147658=CARTESIAN_POINT('Origin',(7.9,2.4,-8.22)) ;
#147659=CARTESIAN_POINT('Origin',(7.9,2.1,-8.22)) ;
#147660=CARTESIAN_POINT('Origin',(7.9,2.4,-8.22)) ;
#147661=CARTESIAN_POINT('Origin',(7.9,2.4,-8.22)) ;
#147662=CARTESIAN_POINT('Origin',(7.9,2.1,-8.22)) ;
#147663=CARTESIAN_POINT('Origin',(7.9,2.1,-8.22)) ;
#147664=CARTESIAN_POINT('Origin',(7.9,2.4,-8.22)) ;
#147665=CARTESIAN_POINT('Origin',(7.9,2.4,-8.32857864376269)) ;
#147666=CARTESIAN_POINT('Origin',(7.9,2.1,-8.22)) ;
#147667=CARTESIAN_POINT('Origin',(7.9,2.1,-9.17)) ;
#147668=CARTESIAN_POINT('Origin',(7.9,2.6,-8.32857864376269)) ;
#147669=CARTESIAN_POINT('Origin',(7.9,2.45857864376269,-8.47)) ;
#147670=CARTESIAN_POINT('Origin',(7.9,1.9,-9.17)) ;
#147671=CARTESIAN_POINT('Origin',(7.9,1.9,-9.37)) ;
#147672=CARTESIAN_POINT('Origin',(7.9,2.45857864376269,-8.47)) ;
#147673=CARTESIAN_POINT('Origin',(7.9,1.9,-9.37)) ;
#147674=CARTESIAN_POINT('Origin',(7.9,-2.15,-9.37)) ;
#147675=CARTESIAN_POINT('Origin',(7.9,-2.15,-9.17)) ;
#147676=CARTESIAN_POINT('Origin',(7.9,-2.35,-9.17)) ;
#147677=CARTESIAN_POINT('Origin',(7.9,3.35,-8.87857864376269)) ;
#147678=CARTESIAN_POINT('Origin',(7.9,3.35,-6.36142135623731)) ;
#147679=CARTESIAN_POINT('Origin',(7.9,-2.35,-8.52311959340942)) ;
#147680=CARTESIAN_POINT('Origin',(7.9,-2.35,-8.52311959340942)) ;
#147681=CARTESIAN_POINT('Origin',(7.9,3.15,-6.36142135623731)) ;
#147682=CARTESIAN_POINT('Origin',(7.9,3.00857864376269,-6.22)) ;
#147683=CARTESIAN_POINT('Origin',(7.9,-2.15,-8.52311959340942)) ;
#147684=CARTESIAN_POINT('Origin',(7.9,-2.32153024911032,-8.4202732340176)) ;
#147685=CARTESIAN_POINT('Origin',(7.9,3.00857864376269,-6.22)) ;
#147686=CARTESIAN_POINT('Origin',(7.9,2.45857864376269,-6.77)) ;
#147687=CARTESIAN_POINT('Origin',(7.9,-3.65625,-7.62)) ;
#147688=CARTESIAN_POINT('Origin',(7.9,-2.32153024911032,-6.8197267659824)) ;
#147689=CARTESIAN_POINT('Origin',(7.9,2.6,-6.91142135623731)) ;
#147690=CARTESIAN_POINT('Origin',(7.9,2.4,-6.91142135623731)) ;
#147691=CARTESIAN_POINT('Origin',(7.9,-2.15,-6.71688040659058)) ;
#147692=CARTESIAN_POINT('Origin',(7.9,-2.35,-6.71688040659058)) ;
#147693=CARTESIAN_POINT('Origin',(7.9,2.4,-6.91142135623731)) ;
#147694=CARTESIAN_POINT('Origin',(7.9,2.4,-7.02)) ;
#147695=CARTESIAN_POINT('Origin',(7.9,-2.35,-6.07)) ;
#147696=CARTESIAN_POINT('Origin',(7.9,-2.35,-6.07)) ;
#147697=CARTESIAN_POINT('Origin',(7.9,2.4,-7.02)) ;
#147698=CARTESIAN_POINT('Origin',(7.9,2.4,-7.02)) ;
#147699=CARTESIAN_POINT('Origin',(7.9,-2.15,-6.07)) ;
#147700=CARTESIAN_POINT('Origin',(7.9,-2.15,-5.87)) ;
#147701=CARTESIAN_POINT('Origin',(7.9,2.4,-7.02)) ;
#147702=CARTESIAN_POINT('Origin',(7.9,2.1,-7.02)) ;
#147703=CARTESIAN_POINT('Origin',(7.9,1.9,-5.87)) ;
#147704=CARTESIAN_POINT('Origin',(7.9,1.9,-5.87)) ;
#147705=CARTESIAN_POINT('Origin',(7.9,2.1,-7.02)) ;
#147706=CARTESIAN_POINT('Origin',(7.9,2.1,-7.02)) ;
#147707=CARTESIAN_POINT('Origin',(7.9,1.9,-6.07)) ;
#147708=CARTESIAN_POINT('Origin',(7.9,2.1,-6.07)) ;
#147709=CARTESIAN_POINT('Origin',(7.9,2.1,-6.07)) ;
#147710=CARTESIAN_POINT('Origin',(7.9,2.1,-4.41)) ;
#147711=CARTESIAN_POINT('Origin',(7.9,2.4,-4.41)) ;
#147712=CARTESIAN_POINT('Origin',(7.9,2.1,-4.41)) ;
#147713=CARTESIAN_POINT('Origin',(7.9,2.4,-4.41)) ;
#147714=CARTESIAN_POINT('Origin',(7.9,2.4,-4.41)) ;
#147715=CARTESIAN_POINT('Origin',(7.9,2.1,-4.41)) ;
#147716=CARTESIAN_POINT('Origin',(7.9,2.1,-4.41)) ;
#147717=CARTESIAN_POINT('Origin',(7.9,2.4,-4.41)) ;
#147718=CARTESIAN_POINT('Origin',(7.9,2.4,-4.51857864376269)) ;
#147719=CARTESIAN_POINT('Origin',(7.9,2.1,-4.41)) ;
#147720=CARTESIAN_POINT('Origin',(7.9,2.1,-5.36)) ;
#147721=CARTESIAN_POINT('Origin',(7.9,2.6,-4.51857864376269)) ;
#147722=CARTESIAN_POINT('Origin',(7.9,2.45857864376269,-4.66)) ;
#147723=CARTESIAN_POINT('Origin',(7.9,1.9,-5.36)) ;
#147724=CARTESIAN_POINT('Origin',(7.9,1.9,-5.56)) ;
#147725=CARTESIAN_POINT('Origin',(7.9,2.45857864376269,-4.66)) ;
#147726=CARTESIAN_POINT('Origin',(7.9,1.9,-5.56)) ;
#147727=CARTESIAN_POINT('Origin',(7.9,-2.15,-5.56)) ;
#147728=CARTESIAN_POINT('Origin',(7.9,-2.15,-5.36)) ;
#147729=CARTESIAN_POINT('Origin',(7.9,-2.35,-5.36)) ;
#147730=CARTESIAN_POINT('Origin',(7.9,3.35,-5.06857864376269)) ;
#147731=CARTESIAN_POINT('Origin',(7.9,3.35,-2.55142135623731)) ;
#147732=CARTESIAN_POINT('Origin',(7.9,-2.35,-4.71311959340942)) ;
#147733=CARTESIAN_POINT('Origin',(7.9,-2.35,-4.71311959340942)) ;
#147734=CARTESIAN_POINT('Origin',(7.9,3.15,-2.55142135623731)) ;
#147735=CARTESIAN_POINT('Origin',(7.9,3.00857864376269,-2.41)) ;
#147736=CARTESIAN_POINT('Origin',(7.9,-2.15,-4.71311959340942)) ;
#147737=CARTESIAN_POINT('Origin',(7.9,-2.32153024911032,-4.6102732340176)) ;
#147738=CARTESIAN_POINT('Origin',(7.9,3.00857864376269,-2.41)) ;
#147739=CARTESIAN_POINT('Origin',(7.9,2.45857864376269,-2.96)) ;
#147740=CARTESIAN_POINT('Origin',(7.9,-3.65625,-3.81)) ;
#147741=CARTESIAN_POINT('Origin',(7.9,-2.32153024911032,-3.0097267659824)) ;
#147742=CARTESIAN_POINT('Origin',(7.9,2.6,-3.10142135623731)) ;
#147743=CARTESIAN_POINT('Origin',(7.9,2.4,-3.10142135623731)) ;
#147744=CARTESIAN_POINT('Origin',(7.9,-2.15,-2.90688040659058)) ;
#147745=CARTESIAN_POINT('Origin',(7.9,-2.35,-2.90688040659058)) ;
#147746=CARTESIAN_POINT('Origin',(7.9,2.4,-3.10142135623731)) ;
#147747=CARTESIAN_POINT('Origin',(7.9,2.4,-3.21)) ;
#147748=CARTESIAN_POINT('Origin',(7.9,-2.35,-2.26)) ;
#147749=CARTESIAN_POINT('Origin',(7.9,-2.35,-2.26)) ;
#147750=CARTESIAN_POINT('Origin',(7.9,2.4,-3.21)) ;
#147751=CARTESIAN_POINT('Origin',(7.9,2.4,-3.21)) ;
#147752=CARTESIAN_POINT('Origin',(7.9,-2.15,-2.26)) ;
#147753=CARTESIAN_POINT('Origin',(7.9,-2.15,-2.06)) ;
#147754=CARTESIAN_POINT('Origin',(7.9,2.4,-3.21)) ;
#147755=CARTESIAN_POINT('Origin',(7.9,2.1,-3.21)) ;
#147756=CARTESIAN_POINT('Origin',(7.9,1.9,-2.06)) ;
#147757=CARTESIAN_POINT('Origin',(7.9,1.9,-2.06)) ;
#147758=CARTESIAN_POINT('Origin',(7.9,2.1,-3.21)) ;
#147759=CARTESIAN_POINT('Origin',(7.9,2.1,-3.21)) ;
#147760=CARTESIAN_POINT('Origin',(7.9,1.9,-2.26)) ;
#147761=CARTESIAN_POINT('Origin',(7.9,2.1,-2.26)) ;
#147762=CARTESIAN_POINT('Origin',(7.9,2.1,-2.26)) ;
#147763=CARTESIAN_POINT('Origin',(-0.899999999999999,-2.,-7.02)) ;
#147764=CARTESIAN_POINT('Origin',(-0.899999999999999,0.4,-7.02)) ;
#147765=CARTESIAN_POINT('Origin',(-0.899999999999999,-1.9,-7.02)) ;
#147766=CARTESIAN_POINT('Origin',(0.600000000000001,0.4,-7.22)) ;
#147767=CARTESIAN_POINT('Origin',(0.500000000000001,0.4,-7.22)) ;
#147768=CARTESIAN_POINT('Origin',(-0.899999999999999,0.4,-7.22)) ;
#147769=CARTESIAN_POINT('Origin',(0.500000000000001,0.4,-7.22)) ;
#147770=CARTESIAN_POINT('',(0.600000000000001,0.4,-7.22)) ;
#147771=CARTESIAN_POINT('Origin',(0.500000000000001,0.4,-7.22)) ;
#147772=CARTESIAN_POINT('Origin',(0.500000000000001,0.4,-7.22)) ;
#147773=CARTESIAN_POINT('Origin',(-0.899999999999999,-1.9,-7.02)) ;
#147774=CARTESIAN_POINT('Origin',(-0.899999999999999,-1.9,-7.02)) ;
#147775=CARTESIAN_POINT('Origin',(-0.899999999999999,-1.9,-7.02)) ;
#147776=CARTESIAN_POINT('Origin',(-0.899999999999999,0.4,-7.22)) ;
#147777=CARTESIAN_POINT('Origin',(-0.899999999999999,0.6,-7.22)) ;
#147778=CARTESIAN_POINT('Origin',(0.500000000000001,0.4,-7.62)) ;
#147779=CARTESIAN_POINT('Origin',(0.500000000000001,0.4,-8.02)) ;
#147780=CARTESIAN_POINT('',(0.600000000000001,0.4,-7.92)) ;
#147781=CARTESIAN_POINT('Ctrl Pts',(0.595612997216081,0.370705721320404,
-7.9907057213204)) ;
#147782=CARTESIAN_POINT('Ctrl Pts',(0.596180587760891,0.372558268494353,
-7.98885549883217)) ;
#147783=CARTESIAN_POINT('Ctrl Pts',(0.596672461925684,0.374355839771976,
-7.98691417986632)) ;
#147784=CARTESIAN_POINT('Ctrl Pts',(0.599015141889213,0.383869350930064,
-7.97576499365627)) ;
#147785=CARTESIAN_POINT('Ctrl Pts',(0.599609996542524,0.390224332900447,
-7.96497260265412)) ;
#147786=CARTESIAN_POINT('Ctrl Pts',(0.600050586298725,0.398117439141558,
-7.94233105320469)) ;
#147787=CARTESIAN_POINT('Ctrl Pts',(0.600000000000001,0.399999999999999,
-7.93120125063353)) ;
#147788=CARTESIAN_POINT('Ctrl Pts',(0.600000000000001,0.399999999999999,
-7.92)) ;
#147789=CARTESIAN_POINT('',(0.600000000000001,0.4,-7.62)) ;
#147790=CARTESIAN_POINT('Origin',(0.500000000000001,-4.5664044441154E-17,
-7.22)) ;
#147791=CARTESIAN_POINT('',(0.500000000000001,0.394987437106619,-7.32)) ;
#147792=CARTESIAN_POINT('Ctrl Pts',(0.500000000000001,0.394987437106619,
-7.32)) ;
#147793=CARTESIAN_POINT('Ctrl Pts',(0.505940567948952,0.3955844866499,-7.32)) ;
#147794=CARTESIAN_POINT('Ctrl Pts',(0.51193197101914,0.396132036079018,
-7.31946630032796)) ;
#147795=CARTESIAN_POINT('Ctrl Pts',(0.517829015308548,0.396618246075354,
-7.31839779577372)) ;
#147796=CARTESIAN_POINT('Ctrl Pts',(0.522982218721201,0.397043126556053,
-7.31746407015711)) ;
#147797=CARTESIAN_POINT('Ctrl Pts',(0.52806264897023,0.397421319341388,
-7.31612282679706)) ;
#147798=CARTESIAN_POINT('Ctrl Pts',(0.532978106724,0.397751505046071,-7.31440574387663)) ;
#147799=CARTESIAN_POINT('Ctrl Pts',(0.538583536338966,0.398128038182999,
-7.31244763784955)) ;
#147800=CARTESIAN_POINT('Ctrl Pts',(0.544059405914893,0.398447721828296,
-7.30997000831105)) ;
#147801=CARTESIAN_POINT('Ctrl Pts',(0.549268572255785,0.398712331108984,
-7.30702073194289)) ;
#147802=CARTESIAN_POINT('Ctrl Pts',(0.553856850427149,0.398945401221756,
-7.30442298414684)) ;
#147803=CARTESIAN_POINT('Ctrl Pts',(0.558237825069329,0.399135987683843,
-7.30146038497999)) ;
#147804=CARTESIAN_POINT('Ctrl Pts',(0.562333836086214,0.399290378266507,
-7.29819522286417)) ;
#147805=CARTESIAN_POINT('Ctrl Pts',(0.566990328957901,0.399465895042381,
-7.2944832689523)) ;
#147806=CARTESIAN_POINT('Ctrl Pts',(0.571349096493437,0.399597278936107,
-7.29032280648479)) ;
#147807=CARTESIAN_POINT('Ctrl Pts',(0.57529692005673,0.399694832180838,
-7.28580557597932)) ;
#147808=CARTESIAN_POINT('Ctrl Pts',(0.578744263667919,0.399780018245914,
-7.28186101121506)) ;
#147809=CARTESIAN_POINT('Ctrl Pts',(0.581878314560434,0.399839626289636,
-7.2776455218421)) ;
#147810=CARTESIAN_POINT('Ctrl Pts',(0.584648147334856,0.399882153365958,
-7.27324181770729)) ;
#147811=CARTESIAN_POINT('Ctrl Pts',(0.587839270208173,0.399931148788079,
-7.2681683125045)) ;
#147812=CARTESIAN_POINT('Ctrl Pts',(0.590595054415089,0.399958289583404,
-7.26276663624446)) ;
#147813=CARTESIAN_POINT('Ctrl Pts',(0.5928386189431,0.399974357003159,-7.2571616850094)) ;
#147814=CARTESIAN_POINT('Ctrl Pts',(0.594777336851653,0.399988241245861,
-7.2523183122424)) ;
#147815=CARTESIAN_POINT('Ctrl Pts',(0.596334051506188,0.399993946552814,
-7.24732416622713)) ;
#147816=CARTESIAN_POINT('Ctrl Pts',(0.597488309822308,0.39999684570125,
-7.24227171856839)) ;
#147817=CARTESIAN_POINT('Ctrl Pts',(0.598804024094406,0.400000150378306,
-7.23651254196053)) ;
#147818=CARTESIAN_POINT('Ctrl Pts',(0.599612685195437,0.399999963509465,
-7.23060284389055)) ;
#147819=CARTESIAN_POINT('Ctrl Pts',(0.599890230999724,0.399999993975383,
-7.224684202261)) ;
#147820=CARTESIAN_POINT('Ctrl Pts',(0.599963464549401,0.400000002014155,
-7.22312250278977)) ;
#147821=CARTESIAN_POINT('Ctrl Pts',(0.600000000000001,0.399999999999999,
-7.22156022150916)) ;
#147822=CARTESIAN_POINT('Ctrl Pts',(0.600000000000001,0.399999999999999,
-7.22)) ;
#147823=CARTESIAN_POINT('',(0.600000000000001,0.299999999999999,-7.22)) ;
#147824=CARTESIAN_POINT('Ctrl Pts',(0.500000000000001,0.394987437106619,
-7.32)) ;
#147825=CARTESIAN_POINT('Ctrl Pts',(0.500454935589846,0.395033159853749,
-7.32)) ;
#147826=CARTESIAN_POINT('Ctrl Pts',(0.500909898680472,0.39507857032906,
-7.31999689549112)) ;
#147827=CARTESIAN_POINT('Ctrl Pts',(0.502892456245169,0.39527507588909,
-7.31996983394194)) ;
#147828=CARTESIAN_POINT('Ctrl Pts',(0.504418747482366,0.395422812032198,
-7.31991398542099)) ;
#147829=CARTESIAN_POINT('Ctrl Pts',(0.508462199543345,0.395804395682033,
-7.31967328105664)) ;
#147830=CARTESIAN_POINT('Ctrl Pts',(0.510974953343295,0.396031485023317,
-7.31942793914506)) ;
#147831=CARTESIAN_POINT('Ctrl Pts',(0.521160739721272,0.396903453186235,
-7.31804279449156)) ;
#147832=CARTESIAN_POINT('Ctrl Pts',(0.528708678528402,0.397444933153161,
-7.31610421770469)) ;
#147833=CARTESIAN_POINT('Ctrl Pts',(0.545943206358073,0.398105551684108,
-7.30946463945115)) ;
#147834=CARTESIAN_POINT('Ctrl Pts',(0.555229535466813,0.397987646678431,
-7.30403535883597)) ;
#147835=CARTESIAN_POINT('Ctrl Pts',(0.571394604995744,0.395490482808038,
-7.29077551336386)) ;
#147836=CARTESIAN_POINT('Ctrl Pts',(0.578055313702842,0.39319894869835,
-7.28324074563176)) ;
#147837=CARTESIAN_POINT('Ctrl Pts',(0.588559132202514,0.385442756729305,
-7.26739223398403)) ;
#147838=CARTESIAN_POINT('Ctrl Pts',(0.592167355639978,0.380240075126892,
-7.2595482656068)) ;
#147839=CARTESIAN_POINT('Ctrl Pts',(0.597496615531108,0.365892753466966,
-7.24392552179528)) ;
#147840=CARTESIAN_POINT('Ctrl Pts',(0.598734255154202,0.356660564300668,
-7.23677274172691)) ;
#147841=CARTESIAN_POINT('Ctrl Pts',(0.600012754681688,0.335223914398549,
-7.22558230586562)) ;
#147842=CARTESIAN_POINT('Ctrl Pts',(0.59999390055981,0.322655037091896,
-7.22166151936558)) ;
#147843=CARTESIAN_POINT('Ctrl Pts',(0.600000296204999,0.30610691358235,
-7.22013962634704)) ;
#147844=CARTESIAN_POINT('Ctrl Pts',(0.600000000000001,0.303050992413436,
-7.22)) ;
#147845=CARTESIAN_POINT('Ctrl Pts',(0.600000000000001,0.299999999999999,
-7.22)) ;
#147846=CARTESIAN_POINT('',(0.600000000000001,-2.39800009914439E-17,-7.22)) ;
#147847=CARTESIAN_POINT('Origin',(0.500000000000001,-1.9,-7.22)) ;
#147848=CARTESIAN_POINT('Origin',(0.600000000000001,-1.9,-7.02)) ;
#147849=CARTESIAN_POINT('Origin',(0.500000000000001,-1.9,-7.02)) ;
#147850=CARTESIAN_POINT('Origin',(-0.899999999999999,-1.9,-6.245)) ;
#147851=CARTESIAN_POINT('Origin',(-0.899999999999999,-1.9,-6.345)) ;
#147852=CARTESIAN_POINT('Origin',(-0.899999999999999,0.6,-7.12)) ;
#147853=CARTESIAN_POINT('Origin',(-0.899999999999999,0.6,-8.02)) ;
#147854=CARTESIAN_POINT('Origin',(0.600000000000001,0.4,-8.02)) ;
#147855=CARTESIAN_POINT('Origin',(0.500000000000001,0.4,-8.02)) ;
#147856=CARTESIAN_POINT('Origin',(-0.899999999999999,0.4,-8.02)) ;
#147857=CARTESIAN_POINT('Origin',(0.500000000000001,0.4,-8.02)) ;
#147858=CARTESIAN_POINT('Origin',(0.500000000000001,-1.9,-7.02)) ;
#147859=CARTESIAN_POINT('Origin',(0.500000000000001,-2.1,-7.02)) ;
#147860=CARTESIAN_POINT('Origin',(-0.899999999999999,-1.9,-6.345)) ;
#147861=CARTESIAN_POINT('Origin',(-1.1,-1.9,-6.345)) ;
#147862=CARTESIAN_POINT('Origin',(-0.899999999999999,-2.1,-6.345)) ;
#147863=CARTESIAN_POINT('Origin',(-0.899999999999999,0.4,-8.02)) ;
#147864=CARTESIAN_POINT('Origin',(-0.899999999999999,0.4,-8.22)) ;
#147865=CARTESIAN_POINT('Origin',(0.500000000000001,-2.1,-7.62)) ;
#147866=CARTESIAN_POINT('Origin',(0.500000000000001,-2.1,-6.345)) ;
#147867=CARTESIAN_POINT('Origin',(0.600000000000001,-2.1,-6.345)) ;
#147868=CARTESIAN_POINT('Origin',(0.500000000000001,-2.1,-6.345)) ;
#147869=CARTESIAN_POINT('Origin',(-1.1,-4.42727195005761E-17,-6.345)) ;
#147870=CARTESIAN_POINT('',(-1.1,1.15,-6.245)) ;
#147871=CARTESIAN_POINT('',(-1.1,1.25,-6.245)) ;
#147872=CARTESIAN_POINT('Origin',(-1.1,1.15,-6.345)) ;
#147873=CARTESIAN_POINT('Origin',(-0.899999999999999,0.5,-8.22)) ;
#147874=CARTESIAN_POINT('Origin',(-0.899999999999999,-1.9,-8.22)) ;
#147875=CARTESIAN_POINT('Origin',(0.600000000000001,-1.9,-8.22)) ;
#147876=CARTESIAN_POINT('Origin',(0.500000000000001,-1.9,-8.22)) ;
#147877=CARTESIAN_POINT('Origin',(-0.899999999999999,-1.9,-8.22)) ;
#147878=CARTESIAN_POINT('Origin',(0.500000000000001,-1.9,-8.22)) ;
#147879=CARTESIAN_POINT('Origin',(0.500000000000001,-2.1,-8.22)) ;
#147880=CARTESIAN_POINT('Origin',(0.500000000000001,-2.1,-6.345)) ;
#147881=CARTESIAN_POINT('Origin',(0.500000000000001,-2.1,-6.345)) ;
#147882=CARTESIAN_POINT('Origin',(-1.1,-2.9,-6.145)) ;
#147883=CARTESIAN_POINT('Origin',(-1.1,-2.9,-6.145)) ;
#147884=CARTESIAN_POINT('Origin',(-1.1,-2.9,-6.145)) ;
#147885=CARTESIAN_POINT('Origin',(-1.1,1.25,-6.145)) ;
#147886=CARTESIAN_POINT('Origin',(-1.1,1.15,-6.145)) ;
#147887=CARTESIAN_POINT('Origin',(-1.1,1.15,-6.345)) ;
#147888=CARTESIAN_POINT('',(-1.1,1.25,-6.345)) ;
#147889=CARTESIAN_POINT('Origin',(-1.1,1.15,-6.345)) ;
#147890=CARTESIAN_POINT('Origin',(-1.1,1.15,-6.345)) ;
#147891=CARTESIAN_POINT('Origin',(-0.899999999999999,-1.9,-8.22)) ;
#147892=CARTESIAN_POINT('Origin',(-0.899999999999999,-1.9,-8.22)) ;
#147893=CARTESIAN_POINT('Origin',(0.500000000000001,-2.1,-7.62)) ;
#147894=CARTESIAN_POINT('Origin',(0.500000000000001,-2.1,-8.895)) ;
#147895=CARTESIAN_POINT('Origin',(0.500000000000001,1.36481920536411E-16,
-6.345)) ;
#147896=CARTESIAN_POINT('Origin',(0.500000000000001,-2.9,-6.345)) ;
#147897=CARTESIAN_POINT('Origin',(-0.999999999999999,-2.9,-6.145)) ;
#147898=CARTESIAN_POINT('Origin',(0.500000000000001,-2.9,-6.145)) ;
#147899=CARTESIAN_POINT('Origin',(-1.1,1.15,-6.345)) ;
#147900=CARTESIAN_POINT('Origin',(-1.1,1.35,-6.345)) ;
#147901=CARTESIAN_POINT('Origin',(-1.1,1.15,-7.62)) ;
#147902=CARTESIAN_POINT('',(-1.1,1.25,-8.895)) ;
#147903=CARTESIAN_POINT('',(-1.1,1.25,-8.995)) ;
#147904=CARTESIAN_POINT('Origin',(-1.1,1.15,-8.895)) ;
#147905=CARTESIAN_POINT('Origin',(-0.899999999999999,-1.9,-8.12)) ;
#147906=CARTESIAN_POINT('Origin',(-0.899999999999999,-1.9,-8.895)) ;
#147907=CARTESIAN_POINT('Origin',(-0.999999999999999,-2.1,-8.895)) ;
#147908=CARTESIAN_POINT('Origin',(0.500000000000001,-2.1,-8.895)) ;
#147909=CARTESIAN_POINT('Origin',(-0.899999999999999,-2.1,-8.895)) ;
#147910=CARTESIAN_POINT('Origin',(0.500000000000001,-2.1,-8.895)) ;
#147911=CARTESIAN_POINT('Origin',(0.500000000000001,-2.1,-8.895)) ;
#147912=CARTESIAN_POINT('Origin',(0.500000000000001,-2.9,-6.345)) ;
#147913=CARTESIAN_POINT('Origin',(0.700000000000002,-2.9,-6.345)) ;
#147914=CARTESIAN_POINT('Origin',(-1.1,1.35,-8.995)) ;
#147915=CARTESIAN_POINT('Origin',(-1.1,1.35,-8.895)) ;
#147916=CARTESIAN_POINT('Origin',(-1.1,1.15,-8.895)) ;
#147917=CARTESIAN_POINT('',(-1.1,1.15,-8.995)) ;
#147918=CARTESIAN_POINT('Origin',(-1.1,1.15,-8.895)) ;
#147919=CARTESIAN_POINT('Origin',(-1.1,1.15,-8.895)) ;
#147920=CARTESIAN_POINT('Origin',(-0.899999999999999,-1.9,-8.895)) ;
#147921=CARTESIAN_POINT('Origin',(-1.1,-1.9,-8.895)) ;
#147922=CARTESIAN_POINT('Origin',(0.500000000000001,-5.86744705109802E-17,
-8.895)) ;
#147923=CARTESIAN_POINT('Origin',(0.500000000000001,-2.9,-8.895)) ;
#147924=CARTESIAN_POINT('Origin',(0.700000000000002,-2.9,-7.62)) ;
#147925=CARTESIAN_POINT('Origin',(0.700000000000002,-2.9,-8.895)) ;
#147926=CARTESIAN_POINT('Origin',(-1.1,1.15,-8.895)) ;
#147927=CARTESIAN_POINT('Origin',(-1.1,1.15,-9.095)) ;
#147928=CARTESIAN_POINT('Origin',(-1.1,-2.39429110547967E-16,-8.895)) ;
#147929=CARTESIAN_POINT('',(-1.1,1.25,-8.995)) ;
#147930=CARTESIAN_POINT('Origin',(0.500000000000001,-2.9,-8.895)) ;
#147931=CARTESIAN_POINT('Origin',(0.500000000000001,-2.9,-9.095)) ;
#147932=CARTESIAN_POINT('Origin',(-1.1,1.25,-9.095)) ;
#147933=CARTESIAN_POINT('Origin',(-1.1,-2.9,-9.095)) ;
#147934=CARTESIAN_POINT('Origin',(-1.1,-2.9,-9.095)) ;
#147935=CARTESIAN_POINT('Origin',(-1.1,-2.9,-9.095)) ;
#147936=CARTESIAN_POINT('Origin',(-1.1,-2.9,-9.095)) ;
#147937=CARTESIAN_POINT('Origin',(1.5,1.9,-7.02)) ;
#147938=CARTESIAN_POINT('Origin',(1.5,1.9,-9.17)) ;
#147939=CARTESIAN_POINT('Origin',(1.5,1.9,-8.22)) ;
#147940=CARTESIAN_POINT('Origin',(1.5,2.1,-8.22)) ;
#147941=CARTESIAN_POINT('Origin',(1.5,2.1,-8.02)) ;
#147942=CARTESIAN_POINT('Origin',(1.5,1.9,-9.17)) ;
#147943=CARTESIAN_POINT('Origin',(1.5,1.9,-9.17)) ;
#147944=CARTESIAN_POINT('Origin',(1.5,2.1,-8.02)) ;
#147945=CARTESIAN_POINT('Origin',(1.5,2.4,-8.02)) ;
#147946=CARTESIAN_POINT('Origin',(1.5,2.1,-9.17)) ;
#147947=CARTESIAN_POINT('Origin',(1.5,-2.15,-9.17)) ;
#147948=CARTESIAN_POINT('Origin',(1.5,2.4,-8.22)) ;
#147949=CARTESIAN_POINT('Origin',(1.5,2.6,-8.22)) ;
#147950=CARTESIAN_POINT('Origin',(1.5,-2.15,-9.17)) ;
#147951=CARTESIAN_POINT('Origin',(1.5,-2.15,-9.17)) ;
#147952=CARTESIAN_POINT('Origin',(1.5,2.6,-7.02)) ;
#147953=CARTESIAN_POINT('Origin',(1.5,2.6,-8.32857864376269)) ;
#147954=CARTESIAN_POINT('Origin',(1.5,-2.15,-7.02)) ;
#147955=CARTESIAN_POINT('Origin',(1.5,-2.15,-8.52311959340942)) ;
#147956=CARTESIAN_POINT('Origin',(1.5,2.6,-8.32857864376269)) ;
#147957=CARTESIAN_POINT('Origin',(1.5,2.6,-8.32857864376269)) ;
#147958=CARTESIAN_POINT('Origin',(1.5,-2.15,-8.52311959340942)) ;
#147959=CARTESIAN_POINT('Origin',(1.5,-2.15,-8.52311959340942)) ;
#147960=CARTESIAN_POINT('Origin',(1.5,1.69571067811865,-7.42428932188135)) ;
#147961=CARTESIAN_POINT('Origin',(1.5,3.15,-8.87857864376269)) ;
#147962=CARTESIAN_POINT('Origin',(1.5,-3.65625,-7.62)) ;
#147963=CARTESIAN_POINT('Origin',(1.5,-2.15,-6.71688040659058)) ;
#147964=CARTESIAN_POINT('Origin',(1.5,3.15,-8.87857864376269)) ;
#147965=CARTESIAN_POINT('Origin',(1.5,3.15,-8.87857864376269)) ;
#147966=CARTESIAN_POINT('Origin',(1.5,-2.15,-6.71688040659058)) ;
#147967=CARTESIAN_POINT('Origin',(1.5,-2.15,-6.71688040659058)) ;
#147968=CARTESIAN_POINT('Origin',(1.5,3.15,-7.02)) ;
#147969=CARTESIAN_POINT('Origin',(1.5,-2.15,-7.02)) ;
#147970=CARTESIAN_POINT('Origin',(1.5,-2.15,-6.07)) ;
#147971=CARTESIAN_POINT('Origin',(1.5,-2.15,-6.07)) ;
#147972=CARTESIAN_POINT('Origin',(1.5,-2.15,-6.07)) ;
#147973=CARTESIAN_POINT('Origin',(1.5,2.29571067811866,-7.21571067811866)) ;
#147974=CARTESIAN_POINT('Origin',(1.5,2.6,-6.91142135623731)) ;
#147975=CARTESIAN_POINT('Origin',(1.5,2.1,-6.07)) ;
#147976=CARTESIAN_POINT('Origin',(1.5,1.9,-6.07)) ;
#147977=CARTESIAN_POINT('Origin',(1.5,2.6,-6.91142135623731)) ;
#147978=CARTESIAN_POINT('Origin',(1.5,2.6,-6.91142135623731)) ;
#147979=CARTESIAN_POINT('Origin',(1.5,1.9,-6.07)) ;
#147980=CARTESIAN_POINT('Origin',(1.5,1.9,-6.07)) ;
#147981=CARTESIAN_POINT('Origin',(1.5,2.6,-7.02)) ;
#147982=CARTESIAN_POINT('Origin',(1.5,2.6,-7.02)) ;
#147983=CARTESIAN_POINT('Origin',(1.5,1.9,-7.02)) ;
#147984=CARTESIAN_POINT('Origin',(1.5,1.9,-7.02)) ;
#147985=CARTESIAN_POINT('Origin',(1.5,2.4,-7.02)) ;
#147986=CARTESIAN_POINT('Origin',(1.5,2.4,-7.22)) ;
#147987=CARTESIAN_POINT('Origin',(1.5,2.1,-7.02)) ;
#147988=CARTESIAN_POINT('Origin',(1.5,2.1,-7.22)) ;
#147989=CARTESIAN_POINT('Origin',(1.5,2.1,-7.22)) ;
#147990=CARTESIAN_POINT('Origin',(-0.899999999999999,-2.,-10.83)) ;
#147991=CARTESIAN_POINT('Origin',(-0.899999999999999,0.4,-10.83)) ;
#147992=CARTESIAN_POINT('Origin',(-0.899999999999999,-1.9,-10.83)) ;
#147993=CARTESIAN_POINT('Origin',(0.600000000000001,0.4,-11.03)) ;
#147994=CARTESIAN_POINT('Origin',(0.500000000000001,0.4,-11.03)) ;
#147995=CARTESIAN_POINT('Origin',(-0.899999999999999,0.4,-11.03)) ;
#147996=CARTESIAN_POINT('Origin',(0.500000000000001,0.4,-11.03)) ;
#147997=CARTESIAN_POINT('',(0.600000000000001,0.4,-11.03)) ;
#147998=CARTESIAN_POINT('Origin',(0.500000000000001,0.4,-11.03)) ;
#147999=CARTESIAN_POINT('Origin',(0.500000000000001,0.4,-11.03)) ;
#148000=CARTESIAN_POINT('Origin',(-0.899999999999999,-1.9,-10.83)) ;
#148001=CARTESIAN_POINT('Origin',(-0.899999999999999,-1.9,-10.83)) ;
#148002=CARTESIAN_POINT('Origin',(-0.899999999999999,-1.9,-10.83)) ;
#148003=CARTESIAN_POINT('Origin',(-0.899999999999999,0.4,-11.03)) ;
#148004=CARTESIAN_POINT('Origin',(-0.899999999999999,0.6,-11.03)) ;
#148005=CARTESIAN_POINT('Origin',(0.500000000000001,0.4,-11.43)) ;
#148006=CARTESIAN_POINT('Origin',(0.500000000000001,0.4,-11.83)) ;
#148007=CARTESIAN_POINT('',(0.600000000000001,0.4,-11.73)) ;
#148008=CARTESIAN_POINT('Ctrl Pts',(0.595612997216082,0.370705721320405,
-11.8007057213204)) ;
#148009=CARTESIAN_POINT('Ctrl Pts',(0.596180587760892,0.372558268494355,
-11.7988554988322)) ;
#148010=CARTESIAN_POINT('Ctrl Pts',(0.596672461925685,0.374355839771978,
-11.7969141798663)) ;
#148011=CARTESIAN_POINT('Ctrl Pts',(0.599015141889211,0.383869350930053,
-11.7857649936563)) ;
#148012=CARTESIAN_POINT('Ctrl Pts',(0.599609996542523,0.390224332900442,
-11.7749726026541)) ;
#148013=CARTESIAN_POINT('Ctrl Pts',(0.600050586298725,0.398117439141559,
-11.7523310532047)) ;
#148014=CARTESIAN_POINT('Ctrl Pts',(0.600000000000001,0.399999999999999,
-11.7412012506335)) ;
#148015=CARTESIAN_POINT('Ctrl Pts',(0.600000000000001,0.399999999999999,
-11.73)) ;
#148016=CARTESIAN_POINT('',(0.600000000000001,0.4,-11.43)) ;
#148017=CARTESIAN_POINT('Origin',(0.500000000000001,-4.56640444411542E-17,
-11.03)) ;
#148018=CARTESIAN_POINT('',(0.500000000000001,0.394987437106619,-11.13)) ;
#148019=CARTESIAN_POINT('Ctrl Pts',(0.500000000000001,0.394987437106619,
-11.13)) ;
#148020=CARTESIAN_POINT('Ctrl Pts',(0.505940567948954,0.395584486649901,
-11.13)) ;
#148021=CARTESIAN_POINT('Ctrl Pts',(0.511931971019137,0.396132036079018,
-11.129466300328)) ;
#148022=CARTESIAN_POINT('Ctrl Pts',(0.51782901530855,0.396618246075355,
-11.1283977957737)) ;
#148023=CARTESIAN_POINT('Ctrl Pts',(0.522982218721202,0.397043126556054,
-11.1274640701571)) ;
#148024=CARTESIAN_POINT('Ctrl Pts',(0.528062648970239,0.397421319341388,
-11.1261228267971)) ;
#148025=CARTESIAN_POINT('Ctrl Pts',(0.532978106724003,0.397751505046071,
-11.1244057438766)) ;
#148026=CARTESIAN_POINT('Ctrl Pts',(0.538583536338951,0.398128038182998,
-11.1224476378496)) ;
#148027=CARTESIAN_POINT('Ctrl Pts',(0.544059405914855,0.398447721828294,
-11.1199700083111)) ;
#148028=CARTESIAN_POINT('Ctrl Pts',(0.549268572255748,0.398712331108982,
-11.1170207319429)) ;
#148029=CARTESIAN_POINT('Ctrl Pts',(0.553856850427136,0.398945401221755,
-11.1144229841468)) ;
#148030=CARTESIAN_POINT('Ctrl Pts',(0.558237825069313,0.399135987683842,
-11.11146038498)) ;
#148031=CARTESIAN_POINT('Ctrl Pts',(0.562333836086205,0.399290378266507,
-11.1081952228642)) ;
#148032=CARTESIAN_POINT('Ctrl Pts',(0.566990328957881,0.399465895042381,
-11.1044832689523)) ;
#148033=CARTESIAN_POINT('Ctrl Pts',(0.571349096493411,0.399597278936107,
-11.1003228064848)) ;
#148034=CARTESIAN_POINT('Ctrl Pts',(0.575296920056702,0.399694832180837,
-11.0958055759794)) ;
#148035=CARTESIAN_POINT('Ctrl Pts',(0.578744263667896,0.399780018245913,
-11.0918610112151)) ;
#148036=CARTESIAN_POINT('Ctrl Pts',(0.581878314560452,0.399839626289636,
-11.0876455218421)) ;
#148037=CARTESIAN_POINT('Ctrl Pts',(0.584648147334861,0.399882153365958,
-11.0832418177073)) ;
#148038=CARTESIAN_POINT('Ctrl Pts',(0.587839270208171,0.399931148788079,
-11.0781683125045)) ;
#148039=CARTESIAN_POINT('Ctrl Pts',(0.590595054415094,0.399958289583404,
-11.0727666362445)) ;
#148040=CARTESIAN_POINT('Ctrl Pts',(0.59283861894311,0.399974357003159,
-11.0671616850094)) ;
#148041=CARTESIAN_POINT('Ctrl Pts',(0.594777336851653,0.399988241245861,
-11.0623183122424)) ;
#148042=CARTESIAN_POINT('Ctrl Pts',(0.596334051506183,0.399993946552814,
-11.0573241662271)) ;
#148043=CARTESIAN_POINT('Ctrl Pts',(0.597488309822303,0.39999684570125,
-11.0522717185684)) ;
#148044=CARTESIAN_POINT('Ctrl Pts',(0.598804024094406,0.400000150378306,
-11.0465125419605)) ;
#148045=CARTESIAN_POINT('Ctrl Pts',(0.599612685195435,0.399999963509465,
-11.0406028438906)) ;
#148046=CARTESIAN_POINT('Ctrl Pts',(0.599890230999722,0.399999993975383,
-11.034684202261)) ;
#148047=CARTESIAN_POINT('Ctrl Pts',(0.5999634645494,0.400000002014155,-11.0331225027898)) ;
#148048=CARTESIAN_POINT('Ctrl Pts',(0.600000000000001,0.399999999999999,
-11.0315602215092)) ;
#148049=CARTESIAN_POINT('Ctrl Pts',(0.600000000000001,0.399999999999999,
-11.03)) ;
#148050=CARTESIAN_POINT('',(0.600000000000001,0.299999999999999,-11.03)) ;
#148051=CARTESIAN_POINT('Ctrl Pts',(0.500000000000001,0.394987437106619,
-11.13)) ;
#148052=CARTESIAN_POINT('Ctrl Pts',(0.50045493559049,0.395033159853814,
-11.13)) ;
#148053=CARTESIAN_POINT('Ctrl Pts',(0.500909898680794,0.395078570329092,
-11.1299968954911)) ;
#148054=CARTESIAN_POINT('Ctrl Pts',(0.502892456245032,0.395275075889076,
-11.1299698339419)) ;
#148055=CARTESIAN_POINT('Ctrl Pts',(0.504418747482277,0.395422812032189,
-11.129913985421)) ;
#148056=CARTESIAN_POINT('Ctrl Pts',(0.508462199543281,0.395804395682027,
-11.1296732810566)) ;
#148057=CARTESIAN_POINT('Ctrl Pts',(0.510974953343229,0.396031485023311,
-11.1294279391451)) ;
#148058=CARTESIAN_POINT('Ctrl Pts',(0.521160739721084,0.396903453186219,
-11.1280427944916)) ;
#148059=CARTESIAN_POINT('Ctrl Pts',(0.528708678528227,0.397444933153154,
-11.1261042177048)) ;
#148060=CARTESIAN_POINT('Ctrl Pts',(0.545943206357832,0.398105551684098,
-11.1194646394512)) ;
#148061=CARTESIAN_POINT('Ctrl Pts',(0.555229535466621,0.397987646678464,
-11.1140353588361)) ;
#148062=CARTESIAN_POINT('Ctrl Pts',(0.571394604995555,0.395490482808064,
-11.100775513364)) ;
#148063=CARTESIAN_POINT('Ctrl Pts',(0.57805531370272,0.393198948698444,
-11.093240745632)) ;
#148064=CARTESIAN_POINT('Ctrl Pts',(0.588559132202387,0.385442756729392,
-11.0773922339842)) ;
#148065=CARTESIAN_POINT('Ctrl Pts',(0.592167355639922,0.380240075127053,
-11.069548265607)) ;
#148066=CARTESIAN_POINT('Ctrl Pts',(0.597496615531038,0.36589275346714,
-11.0539255217955)) ;
#148067=CARTESIAN_POINT('Ctrl Pts',(0.598734255154188,0.356660564300906,
-11.046772741727)) ;
#148068=CARTESIAN_POINT('Ctrl Pts',(0.60001275468167,0.335223914398785,
-11.0355823058657)) ;
#148069=CARTESIAN_POINT('Ctrl Pts',(0.59999390055981,0.322655037092193,
-11.0316615193656)) ;
#148070=CARTESIAN_POINT('Ctrl Pts',(0.600000296204999,0.30610691358234,
-11.030139626347)) ;
#148071=CARTESIAN_POINT('Ctrl Pts',(0.600000000000001,0.303050992413441,
-11.03)) ;
#148072=CARTESIAN_POINT('Ctrl Pts',(0.600000000000001,0.299999999999999,
-11.03)) ;
#148073=CARTESIAN_POINT('',(0.600000000000001,-2.39800009914441E-17,-11.03)) ;
#148074=CARTESIAN_POINT('Origin',(0.500000000000001,-1.9,-11.03)) ;
#148075=CARTESIAN_POINT('Origin',(0.600000000000001,-1.9,-10.83)) ;
#148076=CARTESIAN_POINT('Origin',(0.500000000000001,-1.9,-10.83)) ;
#148077=CARTESIAN_POINT('Origin',(-0.899999999999999,-1.9,-10.055)) ;
#148078=CARTESIAN_POINT('Origin',(-0.899999999999999,-1.9,-10.155)) ;
#148079=CARTESIAN_POINT('Origin',(-0.899999999999999,0.6,-10.93)) ;
#148080=CARTESIAN_POINT('Origin',(-0.899999999999999,0.6,-11.83)) ;
#148081=CARTESIAN_POINT('Origin',(0.600000000000001,0.4,-11.83)) ;
#148082=CARTESIAN_POINT('Origin',(0.500000000000001,0.4,-11.83)) ;
#148083=CARTESIAN_POINT('Origin',(-0.899999999999999,0.4,-11.83)) ;
#148084=CARTESIAN_POINT('Origin',(0.500000000000001,0.4,-11.83)) ;
#148085=CARTESIAN_POINT('Origin',(0.500000000000001,-1.9,-10.83)) ;
#148086=CARTESIAN_POINT('Origin',(0.500000000000001,-2.1,-10.83)) ;
#148087=CARTESIAN_POINT('Origin',(-0.899999999999999,-1.9,-10.155)) ;
#148088=CARTESIAN_POINT('Origin',(-1.1,-1.9,-10.155)) ;
#148089=CARTESIAN_POINT('Origin',(-0.899999999999999,-2.1,-10.155)) ;
#148090=CARTESIAN_POINT('Origin',(-0.899999999999999,0.4,-11.83)) ;
#148091=CARTESIAN_POINT('Origin',(-0.899999999999999,0.4,-12.03)) ;
#148092=CARTESIAN_POINT('Origin',(0.500000000000001,-2.1,-11.43)) ;
#148093=CARTESIAN_POINT('Origin',(0.500000000000001,-2.1,-10.155)) ;
#148094=CARTESIAN_POINT('Origin',(0.600000000000001,-2.1,-10.155)) ;
#148095=CARTESIAN_POINT('Origin',(0.500000000000001,-2.1,-10.155)) ;
#148096=CARTESIAN_POINT('Origin',(-1.1,-4.4272719500576E-17,-10.155)) ;
#148097=CARTESIAN_POINT('',(-1.1,1.15,-10.055)) ;
#148098=CARTESIAN_POINT('',(-1.1,1.25,-10.055)) ;
#148099=CARTESIAN_POINT('Origin',(-1.1,1.15,-10.155)) ;
#148100=CARTESIAN_POINT('Origin',(-0.899999999999999,0.5,-12.03)) ;
#148101=CARTESIAN_POINT('Origin',(-0.899999999999999,-1.9,-12.03)) ;
#148102=CARTESIAN_POINT('Origin',(0.600000000000001,-1.9,-12.03)) ;
#148103=CARTESIAN_POINT('Origin',(0.500000000000001,-1.9,-12.03)) ;
#148104=CARTESIAN_POINT('Origin',(-0.899999999999999,-1.9,-12.03)) ;
#148105=CARTESIAN_POINT('Origin',(0.500000000000001,-1.9,-12.03)) ;
#148106=CARTESIAN_POINT('Origin',(0.500000000000001,-2.1,-12.03)) ;
#148107=CARTESIAN_POINT('Origin',(0.500000000000001,-2.1,-10.155)) ;
#148108=CARTESIAN_POINT('Origin',(0.500000000000001,-2.1,-10.155)) ;
#148109=CARTESIAN_POINT('Origin',(-1.1,-2.9,-9.955)) ;
#148110=CARTESIAN_POINT('Origin',(-1.1,-2.9,-9.955)) ;
#148111=CARTESIAN_POINT('Origin',(-1.1,-2.9,-9.955)) ;
#148112=CARTESIAN_POINT('Origin',(-1.1,1.25,-9.955)) ;
#148113=CARTESIAN_POINT('Origin',(-1.1,1.15,-9.955)) ;
#148114=CARTESIAN_POINT('Origin',(-1.1,1.15,-10.155)) ;
#148115=CARTESIAN_POINT('',(-1.1,1.25,-10.155)) ;
#148116=CARTESIAN_POINT('Origin',(-1.1,1.15,-10.155)) ;
#148117=CARTESIAN_POINT('Origin',(-1.1,1.15,-10.155)) ;
#148118=CARTESIAN_POINT('Origin',(-0.899999999999999,-1.9,-12.03)) ;
#148119=CARTESIAN_POINT('Origin',(-0.899999999999999,-1.9,-12.03)) ;
#148120=CARTESIAN_POINT('Origin',(0.500000000000001,-2.1,-11.43)) ;
#148121=CARTESIAN_POINT('Origin',(0.500000000000001,-2.1,-12.705)) ;
#148122=CARTESIAN_POINT('Origin',(0.500000000000001,1.36481920536411E-16,
-10.155)) ;
#148123=CARTESIAN_POINT('Origin',(0.500000000000001,-2.9,-10.155)) ;
#148124=CARTESIAN_POINT('Origin',(-0.999999999999999,-2.9,-9.955)) ;
#148125=CARTESIAN_POINT('Origin',(0.500000000000001,-2.9,-9.955)) ;
#148126=CARTESIAN_POINT('Origin',(-1.1,1.15,-10.155)) ;
#148127=CARTESIAN_POINT('Origin',(-1.1,1.35,-10.155)) ;
#148128=CARTESIAN_POINT('Origin',(-1.1,1.15,-11.43)) ;
#148129=CARTESIAN_POINT('',(-1.1,1.25,-12.705)) ;
#148130=CARTESIAN_POINT('',(-1.1,1.25,-12.805)) ;
#148131=CARTESIAN_POINT('Origin',(-1.1,1.15,-12.705)) ;
#148132=CARTESIAN_POINT('Origin',(-0.899999999999999,-1.9,-11.93)) ;
#148133=CARTESIAN_POINT('Origin',(-0.899999999999999,-1.9,-12.705)) ;
#148134=CARTESIAN_POINT('Origin',(-0.999999999999999,-2.1,-12.705)) ;
#148135=CARTESIAN_POINT('Origin',(0.500000000000001,-2.1,-12.705)) ;
#148136=CARTESIAN_POINT('Origin',(-0.899999999999999,-2.1,-12.705)) ;
#148137=CARTESIAN_POINT('Origin',(0.500000000000001,-2.1,-12.705)) ;
#148138=CARTESIAN_POINT('Origin',(0.500000000000001,-2.1,-12.705)) ;
#148139=CARTESIAN_POINT('Origin',(0.500000000000001,-2.9,-10.155)) ;
#148140=CARTESIAN_POINT('Origin',(0.700000000000002,-2.9,-10.155)) ;
#148141=CARTESIAN_POINT('Origin',(-1.1,1.35,-12.805)) ;
#148142=CARTESIAN_POINT('Origin',(-1.1,1.35,-12.705)) ;
#148143=CARTESIAN_POINT('Origin',(-1.1,1.15,-12.705)) ;
#148144=CARTESIAN_POINT('',(-1.1,1.15,-12.805)) ;
#148145=CARTESIAN_POINT('Origin',(-1.1,1.15,-12.705)) ;
#148146=CARTESIAN_POINT('Origin',(-1.1,1.15,-12.705)) ;
#148147=CARTESIAN_POINT('Origin',(-0.899999999999999,-1.9,-12.705)) ;
#148148=CARTESIAN_POINT('Origin',(-1.1,-1.9,-12.705)) ;
#148149=CARTESIAN_POINT('Origin',(0.500000000000001,-5.86744705109802E-17,
-12.705)) ;
#148150=CARTESIAN_POINT('Origin',(0.500000000000001,-2.9,-12.705)) ;
#148151=CARTESIAN_POINT('Origin',(0.700000000000002,-2.9,-11.43)) ;
#148152=CARTESIAN_POINT('Origin',(0.700000000000002,-2.9,-12.705)) ;
#148153=CARTESIAN_POINT('Origin',(-1.1,1.15,-12.705)) ;
#148154=CARTESIAN_POINT('Origin',(-1.1,1.15,-12.905)) ;
#148155=CARTESIAN_POINT('Origin',(-1.1,-2.39429110547967E-16,-12.705)) ;
#148156=CARTESIAN_POINT('',(-1.1,1.25,-12.805)) ;
#148157=CARTESIAN_POINT('Origin',(0.500000000000001,-2.9,-12.705)) ;
#148158=CARTESIAN_POINT('Origin',(0.500000000000001,-2.9,-12.905)) ;
#148159=CARTESIAN_POINT('Origin',(-1.1,1.25,-12.905)) ;
#148160=CARTESIAN_POINT('Origin',(-1.1,-2.9,-12.905)) ;
#148161=CARTESIAN_POINT('Origin',(-1.1,-2.9,-12.905)) ;
#148162=CARTESIAN_POINT('Origin',(-1.1,-2.9,-12.905)) ;
#148163=CARTESIAN_POINT('Origin',(-1.1,-2.9,-12.905)) ;
#148164=CARTESIAN_POINT('Origin',(1.5,1.9,-10.83)) ;
#148165=CARTESIAN_POINT('Origin',(1.5,1.9,-12.98)) ;
#148166=CARTESIAN_POINT('Origin',(1.5,1.9,-12.03)) ;
#148167=CARTESIAN_POINT('Origin',(1.5,2.1,-12.03)) ;
#148168=CARTESIAN_POINT('Origin',(1.5,2.1,-11.83)) ;
#148169=CARTESIAN_POINT('Origin',(1.5,1.9,-12.98)) ;
#148170=CARTESIAN_POINT('Origin',(1.5,1.9,-12.98)) ;
#148171=CARTESIAN_POINT('Origin',(1.5,2.1,-11.83)) ;
#148172=CARTESIAN_POINT('Origin',(1.5,2.4,-11.83)) ;
#148173=CARTESIAN_POINT('Origin',(1.5,2.1,-12.98)) ;
#148174=CARTESIAN_POINT('Origin',(1.5,-2.15,-12.98)) ;
#148175=CARTESIAN_POINT('Origin',(1.5,2.4,-12.03)) ;
#148176=CARTESIAN_POINT('Origin',(1.5,2.6,-12.03)) ;
#148177=CARTESIAN_POINT('Origin',(1.5,-2.15,-12.98)) ;
#148178=CARTESIAN_POINT('Origin',(1.5,-2.15,-12.98)) ;
#148179=CARTESIAN_POINT('Origin',(1.5,2.6,-10.83)) ;
#148180=CARTESIAN_POINT('Origin',(1.5,2.6,-12.1385786437627)) ;
#148181=CARTESIAN_POINT('Origin',(1.5,-2.15,-10.83)) ;
#148182=CARTESIAN_POINT('Origin',(1.5,-2.15,-12.3331195934094)) ;
#148183=CARTESIAN_POINT('Origin',(1.5,2.6,-12.1385786437627)) ;
#148184=CARTESIAN_POINT('Origin',(1.5,2.6,-12.1385786437627)) ;
#148185=CARTESIAN_POINT('Origin',(1.5,-2.15,-12.3331195934094)) ;
#148186=CARTESIAN_POINT('Origin',(1.5,-2.15,-12.3331195934094)) ;
#148187=CARTESIAN_POINT('Origin',(1.5,1.69571067811865,-11.2342893218813)) ;
#148188=CARTESIAN_POINT('Origin',(1.5,3.15,-12.6885786437627)) ;
#148189=CARTESIAN_POINT('Origin',(1.5,-3.65625,-11.43)) ;
#148190=CARTESIAN_POINT('Origin',(1.5,-2.15,-10.5268804065906)) ;
#148191=CARTESIAN_POINT('Origin',(1.5,3.15,-12.6885786437627)) ;
#148192=CARTESIAN_POINT('Origin',(1.5,3.15,-12.6885786437627)) ;
#148193=CARTESIAN_POINT('Origin',(1.5,-2.15,-10.5268804065906)) ;
#148194=CARTESIAN_POINT('Origin',(1.5,-2.15,-10.5268804065906)) ;
#148195=CARTESIAN_POINT('Origin',(1.5,3.15,-10.83)) ;
#148196=CARTESIAN_POINT('Origin',(1.5,-2.15,-10.83)) ;
#148197=CARTESIAN_POINT('Origin',(1.5,-2.15,-9.88)) ;
#148198=CARTESIAN_POINT('Origin',(1.5,-2.15,-9.88)) ;
#148199=CARTESIAN_POINT('Origin',(1.5,-2.15,-9.88)) ;
#148200=CARTESIAN_POINT('Origin',(1.5,2.29571067811866,-11.0257106781187)) ;
#148201=CARTESIAN_POINT('Origin',(1.5,2.6,-10.7214213562373)) ;
#148202=CARTESIAN_POINT('Origin',(1.5,2.1,-9.88)) ;
#148203=CARTESIAN_POINT('Origin',(1.5,1.9,-9.88)) ;
#148204=CARTESIAN_POINT('Origin',(1.5,2.6,-10.7214213562373)) ;
#148205=CARTESIAN_POINT('Origin',(1.5,2.6,-10.7214213562373)) ;
#148206=CARTESIAN_POINT('Origin',(1.5,1.9,-9.88)) ;
#148207=CARTESIAN_POINT('Origin',(1.5,1.9,-9.88)) ;
#148208=CARTESIAN_POINT('Origin',(1.5,2.6,-10.83)) ;
#148209=CARTESIAN_POINT('Origin',(1.5,2.6,-10.83)) ;
#148210=CARTESIAN_POINT('Origin',(1.5,1.9,-10.83)) ;
#148211=CARTESIAN_POINT('Origin',(1.5,1.9,-10.83)) ;
#148212=CARTESIAN_POINT('Origin',(1.5,2.4,-10.83)) ;
#148213=CARTESIAN_POINT('Origin',(1.5,2.4,-11.03)) ;
#148214=CARTESIAN_POINT('Origin',(1.5,2.1,-10.83)) ;
#148215=CARTESIAN_POINT('Origin',(1.5,2.1,-11.03)) ;
#148216=CARTESIAN_POINT('Origin',(1.5,2.1,-11.03)) ;
#148217=CARTESIAN_POINT('Origin',(-0.899999999999999,-2.,-14.64)) ;
#148218=CARTESIAN_POINT('Origin',(-0.899999999999999,0.4,-14.64)) ;
#148219=CARTESIAN_POINT('Origin',(-0.899999999999999,-1.9,-14.64)) ;
#148220=CARTESIAN_POINT('Origin',(0.600000000000001,0.4,-14.84)) ;
#148221=CARTESIAN_POINT('Origin',(0.500000000000001,0.4,-14.84)) ;
#148222=CARTESIAN_POINT('Origin',(-0.899999999999999,0.4,-14.84)) ;
#148223=CARTESIAN_POINT('Origin',(0.500000000000001,0.4,-14.84)) ;
#148224=CARTESIAN_POINT('',(0.600000000000001,0.4,-14.84)) ;
#148225=CARTESIAN_POINT('Origin',(0.500000000000001,0.4,-14.84)) ;
#148226=CARTESIAN_POINT('Origin',(0.500000000000001,0.4,-14.84)) ;
#148227=CARTESIAN_POINT('Origin',(-0.899999999999999,-1.9,-14.64)) ;
#148228=CARTESIAN_POINT('Origin',(-0.899999999999999,-1.9,-14.64)) ;
#148229=CARTESIAN_POINT('Origin',(-0.899999999999999,-1.9,-14.64)) ;
#148230=CARTESIAN_POINT('Origin',(-0.899999999999999,0.4,-14.84)) ;
#148231=CARTESIAN_POINT('Origin',(-0.899999999999999,0.6,-14.84)) ;
#148232=CARTESIAN_POINT('Origin',(0.500000000000001,0.4,-15.24)) ;
#148233=CARTESIAN_POINT('Origin',(0.500000000000001,0.4,-15.64)) ;
#148234=CARTESIAN_POINT('',(0.600000000000001,0.4,-15.54)) ;
#148235=CARTESIAN_POINT('Ctrl Pts',(0.595612997216082,0.370705721320405,
-15.6107057213204)) ;
#148236=CARTESIAN_POINT('Ctrl Pts',(0.596180587760893,0.372558268494361,
-15.6088554988322)) ;
#148237=CARTESIAN_POINT('Ctrl Pts',(0.596672461925687,0.374355839771988,
-15.6069141798663)) ;
#148238=CARTESIAN_POINT('Ctrl Pts',(0.599015141889213,0.383869350930072,
-15.5957649936563)) ;
#148239=CARTESIAN_POINT('Ctrl Pts',(0.599609996542525,0.390224332900456,
-15.5849726026541)) ;
#148240=CARTESIAN_POINT('Ctrl Pts',(0.600050586298725,0.398117439141561,
-15.5623310532047)) ;
#148241=CARTESIAN_POINT('Ctrl Pts',(0.600000000000001,0.4,-15.5512012506335)) ;
#148242=CARTESIAN_POINT('Ctrl Pts',(0.600000000000001,0.399999999999999,
-15.54)) ;
#148243=CARTESIAN_POINT('',(0.600000000000001,0.4,-15.24)) ;
#148244=CARTESIAN_POINT('Origin',(0.500000000000001,-4.56640444411542E-17,
-14.84)) ;
#148245=CARTESIAN_POINT('',(0.500000000000001,0.394987437106619,-14.94)) ;
#148246=CARTESIAN_POINT('Ctrl Pts',(0.500000000000001,0.394987437106619,
-14.94)) ;
#148247=CARTESIAN_POINT('Ctrl Pts',(0.505940567948958,0.395584486649901,
-14.94)) ;
#148248=CARTESIAN_POINT('Ctrl Pts',(0.511931971019147,0.396132036079019,
-14.939466300328)) ;
#148249=CARTESIAN_POINT('Ctrl Pts',(0.517829015308562,0.396618246075356,
-14.9383977957737)) ;
#148250=CARTESIAN_POINT('Ctrl Pts',(0.522982218721209,0.397043126556054,
-14.9374640701571)) ;
#148251=CARTESIAN_POINT('Ctrl Pts',(0.528062648970245,0.397421319341388,
-14.9361228267971)) ;
#148252=CARTESIAN_POINT('Ctrl Pts',(0.532978106724004,0.397751505046071,
-14.9344057438766)) ;
#148253=CARTESIAN_POINT('Ctrl Pts',(0.538583536338963,0.398128038182999,
-14.9324476378495)) ;
#148254=CARTESIAN_POINT('Ctrl Pts',(0.544059405914874,0.398447721828296,
-14.9299700083111)) ;
#148255=CARTESIAN_POINT('Ctrl Pts',(0.549268572255776,0.398712331108984,
-14.9270207319429)) ;
#148256=CARTESIAN_POINT('Ctrl Pts',(0.553856850427151,0.398945401221756,
-14.9244229841468)) ;
#148257=CARTESIAN_POINT('Ctrl Pts',(0.558237825069319,0.399135987683843,
-14.92146038498)) ;
#148258=CARTESIAN_POINT('Ctrl Pts',(0.562333836086205,0.399290378266507,
-14.9181952228642)) ;
#148259=CARTESIAN_POINT('Ctrl Pts',(0.56699032895788,0.399465895042381,
-14.9144832689523)) ;
#148260=CARTESIAN_POINT('Ctrl Pts',(0.571349096493406,0.399597278936107,
-14.9103228064848)) ;
#148261=CARTESIAN_POINT('Ctrl Pts',(0.575296920056693,0.399694832180837,
-14.9058055759794)) ;
#148262=CARTESIAN_POINT('Ctrl Pts',(0.578744263667893,0.399780018245913,
-14.9018610112151)) ;
#148263=CARTESIAN_POINT('Ctrl Pts',(0.581878314560404,0.399839626289636,
-14.8976455218421)) ;
#148264=CARTESIAN_POINT('Ctrl Pts',(0.584648147334845,0.399882153365958,
-14.8932418177073)) ;
#148265=CARTESIAN_POINT('Ctrl Pts',(0.587839270208164,0.399931148788079,
-14.8881683125045)) ;
#148266=CARTESIAN_POINT('Ctrl Pts',(0.590595054415084,0.399958289583404,
-14.8827666362445)) ;
#148267=CARTESIAN_POINT('Ctrl Pts',(0.592838618943089,0.399974357003159,
-14.8771616850094)) ;
#148268=CARTESIAN_POINT('Ctrl Pts',(0.594777336851653,0.399988241245861,
-14.8723183122424)) ;
#148269=CARTESIAN_POINT('Ctrl Pts',(0.596334051506184,0.399993946552814,
-14.8673241662272)) ;
#148270=CARTESIAN_POINT('Ctrl Pts',(0.597488309822312,0.39999684570125,
-14.8622717185684)) ;
#148271=CARTESIAN_POINT('Ctrl Pts',(0.598804024094403,0.400000150378306,
-14.8565125419605)) ;
#148272=CARTESIAN_POINT('Ctrl Pts',(0.599612685195422,0.399999963509465,
-14.8506028438907)) ;
#148273=CARTESIAN_POINT('Ctrl Pts',(0.599890230999715,0.399999993975383,
-14.8446842022612)) ;
#148274=CARTESIAN_POINT('Ctrl Pts',(0.599963464549397,0.400000002014155,
-14.8431225027899)) ;
#148275=CARTESIAN_POINT('Ctrl Pts',(0.600000000000001,0.399999999999999,
-14.8415602215092)) ;
#148276=CARTESIAN_POINT('Ctrl Pts',(0.600000000000001,0.399999999999999,
-14.84)) ;
#148277=CARTESIAN_POINT('',(0.600000000000001,0.299999999999999,-14.84)) ;
#148278=CARTESIAN_POINT('Ctrl Pts',(0.500000000000001,0.394987437106619,
-14.94)) ;
#148279=CARTESIAN_POINT('Ctrl Pts',(0.500454935590171,0.395033159853782,
-14.94)) ;
#148280=CARTESIAN_POINT('Ctrl Pts',(0.500909898680634,0.395078570329076,
-14.9399968954911)) ;
#148281=CARTESIAN_POINT('Ctrl Pts',(0.502892456245054,0.395275075889078,
-14.9399698339419)) ;
#148282=CARTESIAN_POINT('Ctrl Pts',(0.504418747482298,0.395422812032191,
-14.939913985421)) ;
#148283=CARTESIAN_POINT('Ctrl Pts',(0.508462199543321,0.395804395682031,
-14.9396732810566)) ;
#148284=CARTESIAN_POINT('Ctrl Pts',(0.510974953343265,0.396031485023314,
-14.9394279391451)) ;
#148285=CARTESIAN_POINT('Ctrl Pts',(0.521160739721169,0.396903453186227,
-14.9380427944916)) ;
#148286=CARTESIAN_POINT('Ctrl Pts',(0.528708678528302,0.397444933153157,
-14.9361042177047)) ;
#148287=CARTESIAN_POINT('Ctrl Pts',(0.54594320635793,0.398105551684103,
-14.9294646394512)) ;
#148288=CARTESIAN_POINT('Ctrl Pts',(0.555229535466698,0.397987646678449,
-14.9240353588361)) ;
#148289=CARTESIAN_POINT('Ctrl Pts',(0.571394604995641,0.395490482808055,
-14.9107755133639)) ;
#148290=CARTESIAN_POINT('Ctrl Pts',(0.578055313702769,0.393198948698403,
-14.9032407456319)) ;
#148291=CARTESIAN_POINT('Ctrl Pts',(0.58855913220244,0.385442756729361,
-14.8873922339841)) ;
#148292=CARTESIAN_POINT('Ctrl Pts',(0.592167355639942,0.380240075126989,
-14.8795482656069)) ;
#148293=CARTESIAN_POINT('Ctrl Pts',(0.59749661553107,0.365892753467073,
-14.8639255217954)) ;
#148294=CARTESIAN_POINT('Ctrl Pts',(0.598734255154193,0.356660564300806,
-14.856772741727)) ;
#148295=CARTESIAN_POINT('Ctrl Pts',(0.600012754681677,0.335223914398739,
-14.8455823058657)) ;
#148296=CARTESIAN_POINT('Ctrl Pts',(0.59999390055981,0.322655037092125,
-14.8416615193656)) ;
#148297=CARTESIAN_POINT('Ctrl Pts',(0.600000296204999,0.306106913582367,
-14.840139626347)) ;
#148298=CARTESIAN_POINT('Ctrl Pts',(0.600000000000001,0.303050992413449,
-14.84)) ;
#148299=CARTESIAN_POINT('Ctrl Pts',(0.600000000000001,0.299999999999999,
-14.84)) ;
#148300=CARTESIAN_POINT('',(0.600000000000001,-2.39800009914441E-17,-14.84)) ;
#148301=CARTESIAN_POINT('Origin',(0.500000000000001,-1.9,-14.84)) ;
#148302=CARTESIAN_POINT('Origin',(0.600000000000001,-1.9,-14.64)) ;
#148303=CARTESIAN_POINT('Origin',(0.500000000000001,-1.9,-14.64)) ;
#148304=CARTESIAN_POINT('Origin',(-0.899999999999999,-1.9,-13.865)) ;
#148305=CARTESIAN_POINT('Origin',(-0.899999999999999,-1.9,-13.965)) ;
#148306=CARTESIAN_POINT('Origin',(-0.899999999999999,0.6,-14.74)) ;
#148307=CARTESIAN_POINT('Origin',(-0.899999999999999,0.6,-15.64)) ;
#148308=CARTESIAN_POINT('Origin',(0.600000000000001,0.4,-15.64)) ;
#148309=CARTESIAN_POINT('Origin',(0.500000000000001,0.4,-15.64)) ;
#148310=CARTESIAN_POINT('Origin',(-0.899999999999999,0.4,-15.64)) ;
#148311=CARTESIAN_POINT('Origin',(0.500000000000001,0.4,-15.64)) ;
#148312=CARTESIAN_POINT('Origin',(0.500000000000001,-1.9,-14.64)) ;
#148313=CARTESIAN_POINT('Origin',(0.500000000000001,-2.1,-14.64)) ;
#148314=CARTESIAN_POINT('Origin',(-0.899999999999999,-1.9,-13.965)) ;
#148315=CARTESIAN_POINT('Origin',(-1.1,-1.9,-13.965)) ;
#148316=CARTESIAN_POINT('Origin',(-0.899999999999999,-2.1,-13.965)) ;
#148317=CARTESIAN_POINT('Origin',(-0.899999999999999,0.4,-15.64)) ;
#148318=CARTESIAN_POINT('Origin',(-0.899999999999999,0.4,-15.84)) ;
#148319=CARTESIAN_POINT('Origin',(0.500000000000001,-2.1,-15.24)) ;
#148320=CARTESIAN_POINT('Origin',(0.500000000000001,-2.1,-13.965)) ;
#148321=CARTESIAN_POINT('Origin',(0.600000000000001,-2.1,-13.965)) ;
#148322=CARTESIAN_POINT('Origin',(0.500000000000001,-2.1,-13.965)) ;
#148323=CARTESIAN_POINT('Origin',(-1.1,-4.4272719500576E-17,-13.965)) ;
#148324=CARTESIAN_POINT('',(-1.1,1.15,-13.865)) ;
#148325=CARTESIAN_POINT('',(-1.1,1.25,-13.865)) ;
#148326=CARTESIAN_POINT('Origin',(-1.1,1.15,-13.965)) ;
#148327=CARTESIAN_POINT('Origin',(-0.899999999999999,0.5,-15.84)) ;
#148328=CARTESIAN_POINT('Origin',(-0.899999999999999,-1.9,-15.84)) ;
#148329=CARTESIAN_POINT('Origin',(0.600000000000001,-1.9,-15.84)) ;
#148330=CARTESIAN_POINT('Origin',(0.500000000000001,-1.9,-15.84)) ;
#148331=CARTESIAN_POINT('Origin',(-0.899999999999999,-1.9,-15.84)) ;
#148332=CARTESIAN_POINT('Origin',(0.500000000000001,-1.9,-15.84)) ;
#148333=CARTESIAN_POINT('Origin',(0.500000000000001,-2.1,-15.84)) ;
#148334=CARTESIAN_POINT('Origin',(0.500000000000001,-2.1,-13.965)) ;
#148335=CARTESIAN_POINT('Origin',(0.500000000000001,-2.1,-13.965)) ;
#148336=CARTESIAN_POINT('Origin',(-1.1,-2.9,-13.765)) ;
#148337=CARTESIAN_POINT('Origin',(-1.1,-2.9,-13.765)) ;
#148338=CARTESIAN_POINT('Origin',(-1.1,-2.9,-13.765)) ;
#148339=CARTESIAN_POINT('Origin',(-1.1,1.25,-13.765)) ;
#148340=CARTESIAN_POINT('Origin',(-1.1,1.15,-13.765)) ;
#148341=CARTESIAN_POINT('Origin',(-1.1,1.15,-13.965)) ;
#148342=CARTESIAN_POINT('',(-1.1,1.25,-13.965)) ;
#148343=CARTESIAN_POINT('Origin',(-1.1,1.15,-13.965)) ;
#148344=CARTESIAN_POINT('Origin',(-1.1,1.15,-13.965)) ;
#148345=CARTESIAN_POINT('Origin',(-0.899999999999999,-1.9,-15.84)) ;
#148346=CARTESIAN_POINT('Origin',(-0.899999999999999,-1.9,-15.84)) ;
#148347=CARTESIAN_POINT('Origin',(0.500000000000001,-2.1,-15.24)) ;
#148348=CARTESIAN_POINT('Origin',(0.500000000000001,-2.1,-16.515)) ;
#148349=CARTESIAN_POINT('Origin',(0.500000000000001,1.36481920536411E-16,
-13.965)) ;
#148350=CARTESIAN_POINT('Origin',(0.500000000000001,-2.9,-13.965)) ;
#148351=CARTESIAN_POINT('Origin',(-0.999999999999999,-2.9,-13.765)) ;
#148352=CARTESIAN_POINT('Origin',(0.500000000000001,-2.9,-13.765)) ;
#148353=CARTESIAN_POINT('Origin',(-1.1,1.15,-13.965)) ;
#148354=CARTESIAN_POINT('Origin',(-1.1,1.35,-13.965)) ;
#148355=CARTESIAN_POINT('Origin',(-1.1,1.15,-15.24)) ;
#148356=CARTESIAN_POINT('',(-1.1,1.25,-16.515)) ;
#148357=CARTESIAN_POINT('',(-1.1,1.25,-16.615)) ;
#148358=CARTESIAN_POINT('Origin',(-1.1,1.15,-16.515)) ;
#148359=CARTESIAN_POINT('Origin',(-0.899999999999999,-1.9,-15.74)) ;
#148360=CARTESIAN_POINT('Origin',(-0.899999999999999,-1.9,-16.515)) ;
#148361=CARTESIAN_POINT('Origin',(-0.999999999999999,-2.1,-16.515)) ;
#148362=CARTESIAN_POINT('Origin',(0.500000000000001,-2.1,-16.515)) ;
#148363=CARTESIAN_POINT('Origin',(-0.899999999999999,-2.1,-16.515)) ;
#148364=CARTESIAN_POINT('Origin',(0.500000000000001,-2.1,-16.515)) ;
#148365=CARTESIAN_POINT('Origin',(0.500000000000001,-2.1,-16.515)) ;
#148366=CARTESIAN_POINT('Origin',(0.500000000000001,-2.9,-13.965)) ;
#148367=CARTESIAN_POINT('Origin',(0.700000000000002,-2.9,-13.965)) ;
#148368=CARTESIAN_POINT('Origin',(-1.1,1.35,-16.615)) ;
#148369=CARTESIAN_POINT('Origin',(-1.1,1.35,-16.515)) ;
#148370=CARTESIAN_POINT('Origin',(-1.1,1.15,-16.515)) ;
#148371=CARTESIAN_POINT('',(-1.1,1.15,-16.615)) ;
#148372=CARTESIAN_POINT('Origin',(-1.1,1.15,-16.515)) ;
#148373=CARTESIAN_POINT('Origin',(-1.1,1.15,-16.515)) ;
#148374=CARTESIAN_POINT('Origin',(-0.899999999999999,-1.9,-16.515)) ;
#148375=CARTESIAN_POINT('Origin',(-1.1,-1.9,-16.515)) ;
#148376=CARTESIAN_POINT('Origin',(0.500000000000001,-5.86744705109802E-17,
-16.515)) ;
#148377=CARTESIAN_POINT('Origin',(0.500000000000001,-2.9,-16.515)) ;
#148378=CARTESIAN_POINT('Origin',(0.700000000000002,-2.9,-15.24)) ;
#148379=CARTESIAN_POINT('Origin',(0.700000000000002,-2.9,-16.515)) ;
#148380=CARTESIAN_POINT('Origin',(-1.1,1.15,-16.515)) ;
#148381=CARTESIAN_POINT('Origin',(-1.1,1.15,-16.715)) ;
#148382=CARTESIAN_POINT('Origin',(-1.1,-2.39429110547967E-16,-16.515)) ;
#148383=CARTESIAN_POINT('',(-1.1,1.25,-16.615)) ;
#148384=CARTESIAN_POINT('Origin',(0.500000000000001,-2.9,-16.515)) ;
#148385=CARTESIAN_POINT('Origin',(0.500000000000001,-2.9,-16.715)) ;
#148386=CARTESIAN_POINT('Origin',(-1.1,1.25,-16.715)) ;
#148387=CARTESIAN_POINT('Origin',(-1.1,-2.9,-16.715)) ;
#148388=CARTESIAN_POINT('Origin',(-1.1,-2.9,-16.715)) ;
#148389=CARTESIAN_POINT('Origin',(-1.1,-2.9,-16.715)) ;
#148390=CARTESIAN_POINT('Origin',(-1.1,-2.9,-16.715)) ;
#148391=CARTESIAN_POINT('Origin',(1.5,1.9,-14.64)) ;
#148392=CARTESIAN_POINT('Origin',(1.5,1.9,-16.79)) ;
#148393=CARTESIAN_POINT('Origin',(1.5,1.9,-15.84)) ;
#148394=CARTESIAN_POINT('Origin',(1.5,2.1,-15.84)) ;
#148395=CARTESIAN_POINT('Origin',(1.5,2.1,-15.64)) ;
#148396=CARTESIAN_POINT('Origin',(1.5,1.9,-16.79)) ;
#148397=CARTESIAN_POINT('Origin',(1.5,1.9,-16.79)) ;
#148398=CARTESIAN_POINT('Origin',(1.5,2.1,-15.64)) ;
#148399=CARTESIAN_POINT('Origin',(1.5,2.4,-15.64)) ;
#148400=CARTESIAN_POINT('Origin',(1.5,2.1,-16.79)) ;
#148401=CARTESIAN_POINT('Origin',(1.5,-2.15,-16.79)) ;
#148402=CARTESIAN_POINT('Origin',(1.5,2.4,-15.84)) ;
#148403=CARTESIAN_POINT('Origin',(1.5,2.6,-15.84)) ;
#148404=CARTESIAN_POINT('Origin',(1.5,-2.15,-16.79)) ;
#148405=CARTESIAN_POINT('Origin',(1.5,-2.15,-16.79)) ;
#148406=CARTESIAN_POINT('Origin',(1.5,2.6,-14.64)) ;
#148407=CARTESIAN_POINT('Origin',(1.5,2.6,-15.9485786437627)) ;
#148408=CARTESIAN_POINT('Origin',(1.5,-2.15,-14.64)) ;
#148409=CARTESIAN_POINT('Origin',(1.5,-2.15,-16.1431195934094)) ;
#148410=CARTESIAN_POINT('Origin',(1.5,2.6,-15.9485786437627)) ;
#148411=CARTESIAN_POINT('Origin',(1.5,2.6,-15.9485786437627)) ;
#148412=CARTESIAN_POINT('Origin',(1.5,-2.15,-16.1431195934094)) ;
#148413=CARTESIAN_POINT('Origin',(1.5,-2.15,-16.1431195934094)) ;
#148414=CARTESIAN_POINT('Origin',(1.5,1.69571067811865,-15.0442893218814)) ;
#148415=CARTESIAN_POINT('Origin',(1.5,3.15,-16.4985786437627)) ;
#148416=CARTESIAN_POINT('Origin',(1.5,-3.65625,-15.24)) ;
#148417=CARTESIAN_POINT('Origin',(1.5,-2.15,-14.3368804065906)) ;
#148418=CARTESIAN_POINT('Origin',(1.5,3.15,-16.4985786437627)) ;
#148419=CARTESIAN_POINT('Origin',(1.5,3.15,-16.4985786437627)) ;
#148420=CARTESIAN_POINT('Origin',(1.5,-2.15,-14.3368804065906)) ;
#148421=CARTESIAN_POINT('Origin',(1.5,-2.15,-14.3368804065906)) ;
#148422=CARTESIAN_POINT('Origin',(1.5,3.15,-14.64)) ;
#148423=CARTESIAN_POINT('Origin',(1.5,-2.15,-14.64)) ;
#148424=CARTESIAN_POINT('Origin',(1.5,-2.15,-13.69)) ;
#148425=CARTESIAN_POINT('Origin',(1.5,-2.15,-13.69)) ;
#148426=CARTESIAN_POINT('Origin',(1.5,-2.15,-13.69)) ;
#148427=CARTESIAN_POINT('Origin',(1.5,2.29571067811866,-14.8357106781187)) ;
#148428=CARTESIAN_POINT('Origin',(1.5,2.6,-14.5314213562373)) ;
#148429=CARTESIAN_POINT('Origin',(1.5,2.1,-13.69)) ;
#148430=CARTESIAN_POINT('Origin',(1.5,1.9,-13.69)) ;
#148431=CARTESIAN_POINT('Origin',(1.5,2.6,-14.5314213562373)) ;
#148432=CARTESIAN_POINT('Origin',(1.5,2.6,-14.5314213562373)) ;
#148433=CARTESIAN_POINT('Origin',(1.5,1.9,-13.69)) ;
#148434=CARTESIAN_POINT('Origin',(1.5,1.9,-13.69)) ;
#148435=CARTESIAN_POINT('Origin',(1.5,2.6,-14.64)) ;
#148436=CARTESIAN_POINT('Origin',(1.5,2.6,-14.64)) ;
#148437=CARTESIAN_POINT('Origin',(1.5,1.9,-14.64)) ;
#148438=CARTESIAN_POINT('Origin',(1.5,1.9,-14.64)) ;
#148439=CARTESIAN_POINT('Origin',(1.5,2.4,-14.64)) ;
#148440=CARTESIAN_POINT('Origin',(1.5,2.4,-14.84)) ;
#148441=CARTESIAN_POINT('Origin',(1.5,2.1,-14.64)) ;
#148442=CARTESIAN_POINT('Origin',(1.5,2.1,-14.84)) ;
#148443=CARTESIAN_POINT('Origin',(1.5,2.1,-14.84)) ;
#148444=CARTESIAN_POINT('Origin',(-0.899999999999999,-2.,-18.45)) ;
#148445=CARTESIAN_POINT('Origin',(-0.899999999999999,0.4,-18.45)) ;
#148446=CARTESIAN_POINT('Origin',(-0.899999999999999,-1.9,-18.45)) ;
#148447=CARTESIAN_POINT('Origin',(0.600000000000001,0.4,-18.65)) ;
#148448=CARTESIAN_POINT('Origin',(0.500000000000001,0.4,-18.65)) ;
#148449=CARTESIAN_POINT('Origin',(-0.899999999999999,0.4,-18.65)) ;
#148450=CARTESIAN_POINT('Origin',(0.500000000000001,0.4,-18.65)) ;
#148451=CARTESIAN_POINT('',(0.600000000000001,0.4,-18.65)) ;
#148452=CARTESIAN_POINT('Origin',(0.500000000000001,0.4,-18.65)) ;
#148453=CARTESIAN_POINT('Origin',(0.500000000000001,0.4,-18.65)) ;
#148454=CARTESIAN_POINT('Origin',(-0.899999999999999,-1.9,-18.45)) ;
#148455=CARTESIAN_POINT('Origin',(-0.899999999999999,-1.9,-18.45)) ;
#148456=CARTESIAN_POINT('Origin',(-0.899999999999999,-1.9,-18.45)) ;
#148457=CARTESIAN_POINT('Origin',(-0.899999999999999,0.4,-18.65)) ;
#148458=CARTESIAN_POINT('Origin',(-0.899999999999999,0.6,-18.65)) ;
#148459=CARTESIAN_POINT('Origin',(0.500000000000001,0.4,-19.05)) ;
#148460=CARTESIAN_POINT('Origin',(0.500000000000001,0.4,-19.45)) ;
#148461=CARTESIAN_POINT('',(0.600000000000001,0.4,-19.35)) ;
#148462=CARTESIAN_POINT('Ctrl Pts',(0.595612997216082,0.370705721320406,
-19.4207057213204)) ;
#148463=CARTESIAN_POINT('Ctrl Pts',(0.596180587760892,0.372558268494356,
-19.4188554988322)) ;
#148464=CARTESIAN_POINT('Ctrl Pts',(0.596672461925685,0.374355839771979,
-19.4169141798663)) ;
#148465=CARTESIAN_POINT('Ctrl Pts',(0.599015141889215,0.38386935093007,
-19.4057649936563)) ;
#148466=CARTESIAN_POINT('Ctrl Pts',(0.599609996542524,0.390224332900451,
-19.3949726026541)) ;
#148467=CARTESIAN_POINT('Ctrl Pts',(0.600050586298725,0.398117439141558,
-19.3723310532047)) ;
#148468=CARTESIAN_POINT('Ctrl Pts',(0.600000000000001,0.399999999999999,
-19.3612012506335)) ;
#148469=CARTESIAN_POINT('Ctrl Pts',(0.600000000000001,0.399999999999999,
-19.35)) ;
#148470=CARTESIAN_POINT('',(0.600000000000001,0.4,-19.05)) ;
#148471=CARTESIAN_POINT('Origin',(0.500000000000001,-4.56640444411542E-17,
-18.65)) ;
#148472=CARTESIAN_POINT('',(0.500000000000001,0.394987437106619,-18.75)) ;
#148473=CARTESIAN_POINT('Ctrl Pts',(0.500000000000001,0.394987437106619,
-18.75)) ;
#148474=CARTESIAN_POINT('Ctrl Pts',(0.505940567948962,0.395584486649901,
-18.75)) ;
#148475=CARTESIAN_POINT('Ctrl Pts',(0.511931971019156,0.39613203607902,
-18.749466300328)) ;
#148476=CARTESIAN_POINT('Ctrl Pts',(0.517829015308575,0.396618246075357,
-18.7483977957737)) ;
#148477=CARTESIAN_POINT('Ctrl Pts',(0.522982218721217,0.397043126556055,
-18.7474640701571)) ;
#148478=CARTESIAN_POINT('Ctrl Pts',(0.528062648970247,0.397421319341388,
-18.7461228267971)) ;
#148479=CARTESIAN_POINT('Ctrl Pts',(0.532978106724002,0.39775150504607,
-18.7444057438766)) ;
#148480=CARTESIAN_POINT('Ctrl Pts',(0.538583536338963,0.398128038182999,
-18.7424476378495)) ;
#148481=CARTESIAN_POINT('Ctrl Pts',(0.544059405914878,0.398447721828296,
-18.7399700083111)) ;
#148482=CARTESIAN_POINT('Ctrl Pts',(0.549268572255783,0.398712331108984,
-18.7370207319429)) ;
#148483=CARTESIAN_POINT('Ctrl Pts',(0.553856850427154,0.398945401221756,
-18.7344229841468)) ;
#148484=CARTESIAN_POINT('Ctrl Pts',(0.558237825069319,0.399135987683843,
-18.73146038498)) ;
#148485=CARTESIAN_POINT('Ctrl Pts',(0.5623338360862,0.399290378266507,-18.7281952228642)) ;
#148486=CARTESIAN_POINT('Ctrl Pts',(0.566990328957884,0.399465895042381,
-18.7244832689523)) ;
#148487=CARTESIAN_POINT('Ctrl Pts',(0.571349096493418,0.399597278936107,
-18.7203228064848)) ;
#148488=CARTESIAN_POINT('Ctrl Pts',(0.575296920056713,0.399694832180838,
-18.7158055759793)) ;
#148489=CARTESIAN_POINT('Ctrl Pts',(0.5787442636679,0.399780018245914,-18.7118610112151)) ;
#148490=CARTESIAN_POINT('Ctrl Pts',(0.581878314560451,0.399839626289636,
-18.7076455218421)) ;
#148491=CARTESIAN_POINT('Ctrl Pts',(0.584648147334859,0.399882153365958,
-18.7032418177073)) ;
#148492=CARTESIAN_POINT('Ctrl Pts',(0.587839270208173,0.399931148788079,
-18.6981683125045)) ;
#148493=CARTESIAN_POINT('Ctrl Pts',(0.590595054415093,0.399958289583404,
-18.6927666362444)) ;
#148494=CARTESIAN_POINT('Ctrl Pts',(0.59283861894311,0.399974357003159,
-18.6871616850094)) ;
#148495=CARTESIAN_POINT('Ctrl Pts',(0.594777336851653,0.399988241245861,
-18.6823183122424)) ;
#148496=CARTESIAN_POINT('Ctrl Pts',(0.596334051506184,0.399993946552814,
-18.6773241662271)) ;
#148497=CARTESIAN_POINT('Ctrl Pts',(0.597488309822305,0.39999684570125,
-18.6722717185684)) ;
#148498=CARTESIAN_POINT('Ctrl Pts',(0.598804024094405,0.400000150378306,
-18.6665125419605)) ;
#148499=CARTESIAN_POINT('Ctrl Pts',(0.599612685195428,0.399999963509465,
-18.6606028438907)) ;
#148500=CARTESIAN_POINT('Ctrl Pts',(0.59989023099972,0.399999993975383,
-18.6546842022611)) ;
#148501=CARTESIAN_POINT('Ctrl Pts',(0.5999634645494,0.400000002014155,-18.6531225027898)) ;
#148502=CARTESIAN_POINT('Ctrl Pts',(0.600000000000001,0.399999999999999,
-18.6515602215092)) ;
#148503=CARTESIAN_POINT('Ctrl Pts',(0.600000000000001,0.399999999999999,
-18.65)) ;
#148504=CARTESIAN_POINT('',(0.600000000000001,0.299999999999999,-18.65)) ;
#148505=CARTESIAN_POINT('Ctrl Pts',(0.500000000000001,0.394987437106619,
-18.75)) ;
#148506=CARTESIAN_POINT('Ctrl Pts',(0.500454935590171,0.395033159853782,
-18.75)) ;
#148507=CARTESIAN_POINT('Ctrl Pts',(0.500909898680634,0.395078570329076,
-18.7499968954911)) ;
#148508=CARTESIAN_POINT('Ctrl Pts',(0.502892456245054,0.395275075889078,
-18.7499698339419)) ;
#148509=CARTESIAN_POINT('Ctrl Pts',(0.504418747482298,0.395422812032191,
-18.749913985421)) ;
#148510=CARTESIAN_POINT('Ctrl Pts',(0.508462199543321,0.395804395682031,
-18.7496732810566)) ;
#148511=CARTESIAN_POINT('Ctrl Pts',(0.510974953343265,0.396031485023314,
-18.7494279391451)) ;
#148512=CARTESIAN_POINT('Ctrl Pts',(0.521160739721169,0.396903453186227,
-18.7480427944916)) ;
#148513=CARTESIAN_POINT('Ctrl Pts',(0.528708678528302,0.397444933153157,
-18.7461042177047)) ;
#148514=CARTESIAN_POINT('Ctrl Pts',(0.54594320635793,0.398105551684103,
-18.7394646394512)) ;
#148515=CARTESIAN_POINT('Ctrl Pts',(0.555229535466698,0.397987646678449,
-18.7340353588361)) ;
#148516=CARTESIAN_POINT('Ctrl Pts',(0.571394604995641,0.395490482808055,
-18.7207755133639)) ;
#148517=CARTESIAN_POINT('Ctrl Pts',(0.578055313702769,0.393198948698403,
-18.7132407456319)) ;
#148518=CARTESIAN_POINT('Ctrl Pts',(0.58855913220244,0.385442756729361,
-18.6973922339841)) ;
#148519=CARTESIAN_POINT('Ctrl Pts',(0.592167355639942,0.380240075126989,
-18.6895482656069)) ;
#148520=CARTESIAN_POINT('Ctrl Pts',(0.59749661553107,0.365892753467073,
-18.6739255217954)) ;
#148521=CARTESIAN_POINT('Ctrl Pts',(0.598734255154193,0.356660564300806,
-18.666772741727)) ;
#148522=CARTESIAN_POINT('Ctrl Pts',(0.600012754681677,0.335223914398739,
-18.6555823058657)) ;
#148523=CARTESIAN_POINT('Ctrl Pts',(0.59999390055981,0.322655037092125,
-18.6516615193656)) ;
#148524=CARTESIAN_POINT('Ctrl Pts',(0.600000296204999,0.306106913582367,
-18.650139626347)) ;
#148525=CARTESIAN_POINT('Ctrl Pts',(0.600000000000001,0.303050992413449,
-18.65)) ;
#148526=CARTESIAN_POINT('Ctrl Pts',(0.600000000000001,0.299999999999999,
-18.65)) ;
#148527=CARTESIAN_POINT('',(0.600000000000001,-2.39800009914441E-17,-18.65)) ;
#148528=CARTESIAN_POINT('Origin',(0.500000000000001,-1.9,-18.65)) ;
#148529=CARTESIAN_POINT('Origin',(0.600000000000001,-1.9,-18.45)) ;
#148530=CARTESIAN_POINT('Origin',(0.500000000000001,-1.9,-18.45)) ;
#148531=CARTESIAN_POINT('Origin',(-0.899999999999999,-1.9,-17.675)) ;
#148532=CARTESIAN_POINT('Origin',(-0.899999999999999,-1.9,-17.775)) ;
#148533=CARTESIAN_POINT('Origin',(-0.899999999999999,0.6,-18.55)) ;
#148534=CARTESIAN_POINT('Origin',(-0.899999999999999,0.6,-19.45)) ;
#148535=CARTESIAN_POINT('Origin',(0.600000000000001,0.4,-19.45)) ;
#148536=CARTESIAN_POINT('Origin',(0.500000000000001,0.4,-19.45)) ;
#148537=CARTESIAN_POINT('Origin',(-0.899999999999999,0.4,-19.45)) ;
#148538=CARTESIAN_POINT('Origin',(0.500000000000001,0.4,-19.45)) ;
#148539=CARTESIAN_POINT('Origin',(0.500000000000001,-1.9,-18.45)) ;
#148540=CARTESIAN_POINT('Origin',(0.500000000000001,-2.1,-18.45)) ;
#148541=CARTESIAN_POINT('Origin',(-0.899999999999999,-1.9,-17.775)) ;
#148542=CARTESIAN_POINT('Origin',(-1.1,-1.9,-17.775)) ;
#148543=CARTESIAN_POINT('Origin',(-0.899999999999999,-2.1,-17.775)) ;
#148544=CARTESIAN_POINT('Origin',(-0.899999999999999,0.4,-19.45)) ;
#148545=CARTESIAN_POINT('Origin',(-0.899999999999999,0.4,-19.65)) ;
#148546=CARTESIAN_POINT('Origin',(0.500000000000001,-2.1,-19.05)) ;
#148547=CARTESIAN_POINT('Origin',(0.500000000000001,-2.1,-17.775)) ;
#148548=CARTESIAN_POINT('Origin',(0.600000000000001,-2.1,-17.775)) ;
#148549=CARTESIAN_POINT('Origin',(0.500000000000001,-2.1,-17.775)) ;
#148550=CARTESIAN_POINT('Origin',(-1.1,-4.42727195005762E-17,-17.775)) ;
#148551=CARTESIAN_POINT('',(-1.1,1.15,-17.675)) ;
#148552=CARTESIAN_POINT('',(-1.1,1.25,-17.675)) ;
#148553=CARTESIAN_POINT('Origin',(-1.1,1.15,-17.775)) ;
#148554=CARTESIAN_POINT('Origin',(-0.899999999999999,0.5,-19.65)) ;
#148555=CARTESIAN_POINT('Origin',(-0.899999999999999,-1.9,-19.65)) ;
#148556=CARTESIAN_POINT('Origin',(0.600000000000001,-1.9,-19.65)) ;
#148557=CARTESIAN_POINT('Origin',(0.500000000000001,-1.9,-19.65)) ;
#148558=CARTESIAN_POINT('Origin',(-0.899999999999999,-1.9,-19.65)) ;
#148559=CARTESIAN_POINT('Origin',(0.500000000000001,-1.9,-19.65)) ;
#148560=CARTESIAN_POINT('Origin',(0.500000000000001,-2.1,-19.65)) ;
#148561=CARTESIAN_POINT('Origin',(0.500000000000001,-2.1,-17.775)) ;
#148562=CARTESIAN_POINT('Origin',(0.500000000000001,-2.1,-17.775)) ;
#148563=CARTESIAN_POINT('Origin',(-1.1,-2.9,-17.575)) ;
#148564=CARTESIAN_POINT('Origin',(-1.1,-2.9,-17.575)) ;
#148565=CARTESIAN_POINT('Origin',(-1.1,-2.9,-17.575)) ;
#148566=CARTESIAN_POINT('Origin',(-1.1,1.25,-17.575)) ;
#148567=CARTESIAN_POINT('Origin',(-1.1,1.15,-17.575)) ;
#148568=CARTESIAN_POINT('Origin',(-1.1,1.15,-17.775)) ;
#148569=CARTESIAN_POINT('',(-1.1,1.25,-17.775)) ;
#148570=CARTESIAN_POINT('Origin',(-1.1,1.15,-17.775)) ;
#148571=CARTESIAN_POINT('Origin',(-1.1,1.15,-17.775)) ;
#148572=CARTESIAN_POINT('Origin',(-0.899999999999999,-1.9,-19.65)) ;
#148573=CARTESIAN_POINT('Origin',(-0.899999999999999,-1.9,-19.65)) ;
#148574=CARTESIAN_POINT('Origin',(0.500000000000001,-2.1,-19.05)) ;
#148575=CARTESIAN_POINT('Origin',(0.500000000000001,-2.1,-20.325)) ;
#148576=CARTESIAN_POINT('Origin',(0.500000000000001,1.36481920536411E-16,
-17.775)) ;
#148577=CARTESIAN_POINT('Origin',(0.500000000000001,-2.9,-17.775)) ;
#148578=CARTESIAN_POINT('Origin',(-0.999999999999999,-2.9,-17.575)) ;
#148579=CARTESIAN_POINT('Origin',(0.500000000000001,-2.9,-17.575)) ;
#148580=CARTESIAN_POINT('Origin',(-1.1,1.15,-17.775)) ;
#148581=CARTESIAN_POINT('Origin',(-1.1,1.35,-17.775)) ;
#148582=CARTESIAN_POINT('Origin',(-1.1,1.15,-19.05)) ;
#148583=CARTESIAN_POINT('',(-1.1,1.25,-20.325)) ;
#148584=CARTESIAN_POINT('',(-1.1,1.25,-20.425)) ;
#148585=CARTESIAN_POINT('Origin',(-1.1,1.15,-20.325)) ;
#148586=CARTESIAN_POINT('Origin',(-0.899999999999999,-1.9,-19.55)) ;
#148587=CARTESIAN_POINT('Origin',(-0.899999999999999,-1.9,-20.325)) ;
#148588=CARTESIAN_POINT('Origin',(-0.999999999999999,-2.1,-20.325)) ;
#148589=CARTESIAN_POINT('Origin',(0.500000000000001,-2.1,-20.325)) ;
#148590=CARTESIAN_POINT('Origin',(-0.899999999999999,-2.1,-20.325)) ;
#148591=CARTESIAN_POINT('Origin',(0.500000000000001,-2.1,-20.325)) ;
#148592=CARTESIAN_POINT('Origin',(0.500000000000001,-2.1,-20.325)) ;
#148593=CARTESIAN_POINT('Origin',(0.500000000000001,-2.9,-17.775)) ;
#148594=CARTESIAN_POINT('Origin',(0.700000000000002,-2.9,-17.775)) ;
#148595=CARTESIAN_POINT('Origin',(-1.1,1.35,-20.425)) ;
#148596=CARTESIAN_POINT('Origin',(-1.1,1.35,-20.325)) ;
#148597=CARTESIAN_POINT('Origin',(-1.1,1.15,-20.325)) ;
#148598=CARTESIAN_POINT('',(-1.1,1.15,-20.425)) ;
#148599=CARTESIAN_POINT('Origin',(-1.1,1.15,-20.325)) ;
#148600=CARTESIAN_POINT('Origin',(-1.1,1.15,-20.325)) ;
#148601=CARTESIAN_POINT('Origin',(-0.899999999999999,-1.9,-20.325)) ;
#148602=CARTESIAN_POINT('Origin',(-1.1,-1.9,-20.325)) ;
#148603=CARTESIAN_POINT('Origin',(0.500000000000001,-5.86744705109802E-17,
-20.325)) ;
#148604=CARTESIAN_POINT('Origin',(0.500000000000001,-2.9,-20.325)) ;
#148605=CARTESIAN_POINT('Origin',(0.700000000000002,-2.9,-19.05)) ;
#148606=CARTESIAN_POINT('Origin',(0.700000000000002,-2.9,-20.325)) ;
#148607=CARTESIAN_POINT('Origin',(-1.1,1.15,-20.325)) ;
#148608=CARTESIAN_POINT('Origin',(-1.1,1.15,-20.525)) ;
#148609=CARTESIAN_POINT('Origin',(-1.1,-2.39429110547967E-16,-20.325)) ;
#148610=CARTESIAN_POINT('',(-1.1,1.25,-20.425)) ;
#148611=CARTESIAN_POINT('Origin',(0.500000000000001,-2.9,-20.325)) ;
#148612=CARTESIAN_POINT('Origin',(0.500000000000001,-2.9,-20.525)) ;
#148613=CARTESIAN_POINT('Origin',(-1.1,1.25,-20.525)) ;
#148614=CARTESIAN_POINT('Origin',(-1.1,-2.9,-20.525)) ;
#148615=CARTESIAN_POINT('Origin',(-1.1,-2.9,-20.525)) ;
#148616=CARTESIAN_POINT('Origin',(-1.1,-2.9,-20.525)) ;
#148617=CARTESIAN_POINT('Origin',(-1.1,-2.9,-20.525)) ;
#148618=CARTESIAN_POINT('Origin',(1.5,1.9,-18.45)) ;
#148619=CARTESIAN_POINT('Origin',(1.5,1.9,-20.6)) ;
#148620=CARTESIAN_POINT('Origin',(1.5,1.9,-19.65)) ;
#148621=CARTESIAN_POINT('Origin',(1.5,2.1,-19.65)) ;
#148622=CARTESIAN_POINT('Origin',(1.5,2.1,-19.45)) ;
#148623=CARTESIAN_POINT('Origin',(1.5,1.9,-20.6)) ;
#148624=CARTESIAN_POINT('Origin',(1.5,1.9,-20.6)) ;
#148625=CARTESIAN_POINT('Origin',(1.5,2.1,-19.45)) ;
#148626=CARTESIAN_POINT('Origin',(1.5,2.4,-19.45)) ;
#148627=CARTESIAN_POINT('Origin',(1.5,2.1,-20.6)) ;
#148628=CARTESIAN_POINT('Origin',(1.5,-2.15,-20.6)) ;
#148629=CARTESIAN_POINT('Origin',(1.5,2.4,-19.65)) ;
#148630=CARTESIAN_POINT('Origin',(1.5,2.6,-19.65)) ;
#148631=CARTESIAN_POINT('Origin',(1.5,-2.15,-20.6)) ;
#148632=CARTESIAN_POINT('Origin',(1.5,-2.15,-20.6)) ;
#148633=CARTESIAN_POINT('Origin',(1.5,2.6,-18.45)) ;
#148634=CARTESIAN_POINT('Origin',(1.5,2.6,-19.7585786437627)) ;
#148635=CARTESIAN_POINT('Origin',(1.5,-2.15,-18.45)) ;
#148636=CARTESIAN_POINT('Origin',(1.5,-2.15,-19.9531195934094)) ;
#148637=CARTESIAN_POINT('Origin',(1.5,2.6,-19.7585786437627)) ;
#148638=CARTESIAN_POINT('Origin',(1.5,2.6,-19.7585786437627)) ;
#148639=CARTESIAN_POINT('Origin',(1.5,-2.15,-19.9531195934094)) ;
#148640=CARTESIAN_POINT('Origin',(1.5,-2.15,-19.9531195934094)) ;
#148641=CARTESIAN_POINT('Origin',(1.5,1.69571067811865,-18.8542893218813)) ;
#148642=CARTESIAN_POINT('Origin',(1.5,3.15,-20.3085786437627)) ;
#148643=CARTESIAN_POINT('Origin',(1.5,-3.65625,-19.05)) ;
#148644=CARTESIAN_POINT('Origin',(1.5,-2.15,-18.1468804065906)) ;
#148645=CARTESIAN_POINT('Origin',(1.5,3.15,-20.3085786437627)) ;
#148646=CARTESIAN_POINT('Origin',(1.5,3.15,-20.3085786437627)) ;
#148647=CARTESIAN_POINT('Origin',(1.5,-2.15,-18.1468804065906)) ;
#148648=CARTESIAN_POINT('Origin',(1.5,-2.15,-18.1468804065906)) ;
#148649=CARTESIAN_POINT('Origin',(1.5,3.15,-18.45)) ;
#148650=CARTESIAN_POINT('Origin',(1.5,-2.15,-18.45)) ;
#148651=CARTESIAN_POINT('Origin',(1.5,-2.15,-17.5)) ;
#148652=CARTESIAN_POINT('Origin',(1.5,-2.15,-17.5)) ;
#148653=CARTESIAN_POINT('Origin',(1.5,-2.15,-17.5)) ;
#148654=CARTESIAN_POINT('Origin',(1.5,2.29571067811866,-18.6457106781187)) ;
#148655=CARTESIAN_POINT('Origin',(1.5,2.6,-18.3414213562373)) ;
#148656=CARTESIAN_POINT('Origin',(1.5,2.1,-17.5)) ;
#148657=CARTESIAN_POINT('Origin',(1.5,1.9,-17.5)) ;
#148658=CARTESIAN_POINT('Origin',(1.5,2.6,-18.3414213562373)) ;
#148659=CARTESIAN_POINT('Origin',(1.5,2.6,-18.3414213562373)) ;
#148660=CARTESIAN_POINT('Origin',(1.5,1.9,-17.5)) ;
#148661=CARTESIAN_POINT('Origin',(1.5,1.9,-17.5)) ;
#148662=CARTESIAN_POINT('Origin',(1.5,2.6,-18.45)) ;
#148663=CARTESIAN_POINT('Origin',(1.5,2.6,-18.45)) ;
#148664=CARTESIAN_POINT('Origin',(1.5,1.9,-18.45)) ;
#148665=CARTESIAN_POINT('Origin',(1.5,1.9,-18.45)) ;
#148666=CARTESIAN_POINT('Origin',(1.5,2.4,-18.45)) ;
#148667=CARTESIAN_POINT('Origin',(1.5,2.4,-18.65)) ;
#148668=CARTESIAN_POINT('Origin',(1.5,2.1,-18.45)) ;
#148669=CARTESIAN_POINT('Origin',(1.5,2.1,-18.65)) ;
#148670=CARTESIAN_POINT('Origin',(1.5,2.1,-18.65)) ;
#148671=CARTESIAN_POINT('Origin',(-0.899999999999999,-2.,-22.26)) ;
#148672=CARTESIAN_POINT('Origin',(-0.899999999999999,0.4,-22.26)) ;
#148673=CARTESIAN_POINT('Origin',(-0.899999999999999,-1.9,-22.26)) ;
#148674=CARTESIAN_POINT('Origin',(0.600000000000001,0.4,-22.46)) ;
#148675=CARTESIAN_POINT('Origin',(0.500000000000001,0.4,-22.46)) ;
#148676=CARTESIAN_POINT('Origin',(-0.899999999999999,0.4,-22.46)) ;
#148677=CARTESIAN_POINT('Origin',(0.500000000000001,0.4,-22.46)) ;
#148678=CARTESIAN_POINT('',(0.600000000000001,0.4,-22.46)) ;
#148679=CARTESIAN_POINT('Origin',(0.500000000000001,0.4,-22.46)) ;
#148680=CARTESIAN_POINT('Origin',(0.500000000000001,0.4,-22.46)) ;
#148681=CARTESIAN_POINT('Origin',(-0.899999999999999,-1.9,-22.26)) ;
#148682=CARTESIAN_POINT('Origin',(-0.899999999999999,-1.9,-22.26)) ;
#148683=CARTESIAN_POINT('Origin',(-0.899999999999999,-1.9,-22.26)) ;
#148684=CARTESIAN_POINT('Origin',(-0.899999999999999,0.4,-22.46)) ;
#148685=CARTESIAN_POINT('Origin',(-0.899999999999999,0.6,-22.46)) ;
#148686=CARTESIAN_POINT('Origin',(0.500000000000001,0.4,-22.86)) ;
#148687=CARTESIAN_POINT('Origin',(0.500000000000001,0.4,-23.26)) ;
#148688=CARTESIAN_POINT('',(0.600000000000001,0.4,-23.16)) ;
#148689=CARTESIAN_POINT('Ctrl Pts',(0.595612997216081,0.370705721320404,
-23.2307057213204)) ;
#148690=CARTESIAN_POINT('Ctrl Pts',(0.596180587760893,0.372558268494359,
-23.2288554988322)) ;
#148691=CARTESIAN_POINT('Ctrl Pts',(0.596672461925686,0.374355839771986,
-23.2269141798663)) ;
#148692=CARTESIAN_POINT('Ctrl Pts',(0.599015141889206,0.38386935093004,
-23.2157649936563)) ;
#148693=CARTESIAN_POINT('Ctrl Pts',(0.599609996542524,0.390224332900438,
-23.2049726026542)) ;
#148694=CARTESIAN_POINT('Ctrl Pts',(0.600050586298726,0.398117439141562,
-23.1823310532047)) ;
#148695=CARTESIAN_POINT('Ctrl Pts',(0.600000000000001,0.4,-23.1712012506335)) ;
#148696=CARTESIAN_POINT('Ctrl Pts',(0.600000000000001,0.399999999999999,
-23.16)) ;
#148697=CARTESIAN_POINT('',(0.600000000000001,0.4,-22.86)) ;
#148698=CARTESIAN_POINT('Origin',(0.500000000000001,-4.56640444411542E-17,
-22.46)) ;
#148699=CARTESIAN_POINT('',(0.500000000000001,0.394987437106619,-22.56)) ;
#148700=CARTESIAN_POINT('Ctrl Pts',(0.500000000000001,0.394987437106619,
-22.56)) ;
#148701=CARTESIAN_POINT('Ctrl Pts',(0.50594056794894,0.395584486649899,
-22.56)) ;
#148702=CARTESIAN_POINT('Ctrl Pts',(0.511931971019111,0.396132036079016,
-22.559466300328)) ;
#148703=CARTESIAN_POINT('Ctrl Pts',(0.517829015308511,0.396618246075352,
-22.5583977957737)) ;
#148704=CARTESIAN_POINT('Ctrl Pts',(0.522982218721178,0.397043126556052,
-22.5574640701571)) ;
#148705=CARTESIAN_POINT('Ctrl Pts',(0.528062648970232,0.397421319341387,
-22.5561228267971)) ;
#148706=CARTESIAN_POINT('Ctrl Pts',(0.532978106724004,0.397751505046071,
-22.5544057438766)) ;
#148707=CARTESIAN_POINT('Ctrl Pts',(0.538583536338997,0.398128038183002,
-22.5524476378495)) ;
#148708=CARTESIAN_POINT('Ctrl Pts',(0.544059405914977,0.3984477218283,-22.549970008311)) ;
#148709=CARTESIAN_POINT('Ctrl Pts',(0.549268572255885,0.398712331108989,
-22.5470207319428)) ;
#148710=CARTESIAN_POINT('Ctrl Pts',(0.553856850427199,0.398945401221759,
-22.5444229841468)) ;
#148711=CARTESIAN_POINT('Ctrl Pts',(0.558237825069336,0.399135987683844,
-22.54146038498)) ;
#148712=CARTESIAN_POINT('Ctrl Pts',(0.562333836086193,0.399290378266507,
-22.5381952228642)) ;
#148713=CARTESIAN_POINT('Ctrl Pts',(0.56699032895789,0.399465895042382,
-22.5344832689523)) ;
#148714=CARTESIAN_POINT('Ctrl Pts',(0.571349096493477,0.399597278936108,
-22.5303228064847)) ;
#148715=CARTESIAN_POINT('Ctrl Pts',(0.575296920056774,0.399694832180838,
-22.5258055759793)) ;
#148716=CARTESIAN_POINT('Ctrl Pts',(0.578744263667953,0.399780018245914,
-22.521861011215)) ;
#148717=CARTESIAN_POINT('Ctrl Pts',(0.581878314560456,0.399839626289636,
-22.5176455218421)) ;
#148718=CARTESIAN_POINT('Ctrl Pts',(0.584648147334871,0.399882153365958,
-22.5132418177073)) ;
#148719=CARTESIAN_POINT('Ctrl Pts',(0.587839270208222,0.39993114878808,
-22.5081683125044)) ;
#148720=CARTESIAN_POINT('Ctrl Pts',(0.590595054415142,0.399958289583405,
-22.5027666362444)) ;
#148721=CARTESIAN_POINT('Ctrl Pts',(0.592838618943166,0.39997435700316,
-22.4971616850092)) ;
#148722=CARTESIAN_POINT('Ctrl Pts',(0.594777336851685,0.399988241245861,
-22.4923183122423)) ;
#148723=CARTESIAN_POINT('Ctrl Pts',(0.596334051506206,0.399993946552814,
-22.4873241662271)) ;
#148724=CARTESIAN_POINT('Ctrl Pts',(0.59748830982231,0.39999684570125,-22.4822717185684)) ;
#148725=CARTESIAN_POINT('Ctrl Pts',(0.598804024094403,0.400000150378306,
-22.4765125419605)) ;
#148726=CARTESIAN_POINT('Ctrl Pts',(0.599612685195435,0.399999963509465,
-22.4706028438905)) ;
#148727=CARTESIAN_POINT('Ctrl Pts',(0.599890230999722,0.399999993975383,
-22.4646842022611)) ;
#148728=CARTESIAN_POINT('Ctrl Pts',(0.5999634645494,0.400000002014155,-22.4631225027898)) ;
#148729=CARTESIAN_POINT('Ctrl Pts',(0.600000000000001,0.399999999999999,
-22.4615602215092)) ;
#148730=CARTESIAN_POINT('Ctrl Pts',(0.600000000000001,0.399999999999999,
-22.46)) ;
#148731=CARTESIAN_POINT('',(0.600000000000001,0.299999999999999,-22.46)) ;
#148732=CARTESIAN_POINT('Ctrl Pts',(0.500000000000001,0.394987437106619,
-22.56)) ;
#148733=CARTESIAN_POINT('Ctrl Pts',(0.50045493558952,0.395033159853717,
-22.56)) ;
#148734=CARTESIAN_POINT('Ctrl Pts',(0.50090989868031,0.395078570329044,
-22.5599968954911)) ;
#148735=CARTESIAN_POINT('Ctrl Pts',(0.502892456245184,0.395275075889091,
-22.5599698339419)) ;
#148736=CARTESIAN_POINT('Ctrl Pts',(0.504418747482384,0.395422812032199,
-22.559913985421)) ;
#148737=CARTESIAN_POINT('Ctrl Pts',(0.508462199543371,0.395804395682036,
-22.5596732810566)) ;
#148738=CARTESIAN_POINT('Ctrl Pts',(0.510974953343326,0.396031485023319,
-22.5594279391451)) ;
#148739=CARTESIAN_POINT('Ctrl Pts',(0.521160739721382,0.396903453186245,
-22.5580427944915)) ;
#148740=CARTESIAN_POINT('Ctrl Pts',(0.528708678528517,0.397444933153166,
-22.5561042177046)) ;
#148741=CARTESIAN_POINT('Ctrl Pts',(0.545943206358243,0.398105551684114,
-22.5494646394511)) ;
#148742=CARTESIAN_POINT('Ctrl Pts',(0.555229535466965,0.397987646678414,
-22.5440353588359)) ;
#148743=CARTESIAN_POINT('Ctrl Pts',(0.57139460499589,0.395490482808011,
-22.5307755133637)) ;
#148744=CARTESIAN_POINT('Ctrl Pts',(0.578055313702948,0.393198948698283,
-22.5232407456316)) ;
#148745=CARTESIAN_POINT('Ctrl Pts',(0.588559132202604,0.385442756729229,
-22.5073922339839)) ;
#148746=CARTESIAN_POINT('Ctrl Pts',(0.592167355640029,0.380240075126779,
-22.4995482656067)) ;
#148747=CARTESIAN_POINT('Ctrl Pts',(0.597496615531157,0.365892753466814,
-22.4839255217951)) ;
#148748=CARTESIAN_POINT('Ctrl Pts',(0.598734255154217,0.35666056430046,
-22.4767727417268)) ;
#148749=CARTESIAN_POINT('Ctrl Pts',(0.600012754681695,0.335223914398355,
-22.4655823058655)) ;
#148750=CARTESIAN_POINT('Ctrl Pts',(0.59999390055981,0.322655037091671,
-22.4616615193655)) ;
#148751=CARTESIAN_POINT('Ctrl Pts',(0.600000296204999,0.306106913582289,
-22.460139626347)) ;
#148752=CARTESIAN_POINT('Ctrl Pts',(0.600000000000001,0.303050992413402,
-22.46)) ;
#148753=CARTESIAN_POINT('Ctrl Pts',(0.600000000000001,0.299999999999999,
-22.46)) ;
#148754=CARTESIAN_POINT('',(0.600000000000001,-2.39800009914441E-17,-22.46)) ;
#148755=CARTESIAN_POINT('Origin',(0.500000000000001,-1.9,-22.46)) ;
#148756=CARTESIAN_POINT('Origin',(0.600000000000001,-1.9,-22.26)) ;
#148757=CARTESIAN_POINT('Origin',(0.500000000000001,-1.9,-22.26)) ;
#148758=CARTESIAN_POINT('Origin',(-0.899999999999999,-1.9,-21.485)) ;
#148759=CARTESIAN_POINT('Origin',(-0.899999999999999,-1.9,-21.585)) ;
#148760=CARTESIAN_POINT('Origin',(-0.899999999999999,0.6,-22.36)) ;
#148761=CARTESIAN_POINT('Origin',(-0.899999999999999,0.6,-23.26)) ;
#148762=CARTESIAN_POINT('Origin',(0.600000000000001,0.4,-23.26)) ;
#148763=CARTESIAN_POINT('Origin',(0.500000000000001,0.4,-23.26)) ;
#148764=CARTESIAN_POINT('Origin',(-0.899999999999999,0.4,-23.26)) ;
#148765=CARTESIAN_POINT('Origin',(0.500000000000001,0.4,-23.26)) ;
#148766=CARTESIAN_POINT('Origin',(0.500000000000001,-1.9,-22.26)) ;
#148767=CARTESIAN_POINT('Origin',(0.500000000000001,-2.1,-22.26)) ;
#148768=CARTESIAN_POINT('Origin',(-0.899999999999999,-1.9,-21.585)) ;
#148769=CARTESIAN_POINT('Origin',(-1.1,-1.9,-21.585)) ;
#148770=CARTESIAN_POINT('Origin',(-0.899999999999999,-2.1,-21.585)) ;
#148771=CARTESIAN_POINT('Origin',(-0.899999999999999,0.4,-23.26)) ;
#148772=CARTESIAN_POINT('Origin',(-0.899999999999999,0.4,-23.46)) ;
#148773=CARTESIAN_POINT('Origin',(0.500000000000001,-2.1,-22.86)) ;
#148774=CARTESIAN_POINT('Origin',(0.500000000000001,-2.1,-21.585)) ;
#148775=CARTESIAN_POINT('Origin',(0.600000000000001,-2.1,-21.585)) ;
#148776=CARTESIAN_POINT('Origin',(0.500000000000001,-2.1,-21.585)) ;
#148777=CARTESIAN_POINT('Origin',(-1.1,-4.42727195005762E-17,-21.585)) ;
#148778=CARTESIAN_POINT('',(-1.1,1.15,-21.485)) ;
#148779=CARTESIAN_POINT('',(-1.1,1.25,-21.485)) ;
#148780=CARTESIAN_POINT('Origin',(-1.1,1.15,-21.585)) ;
#148781=CARTESIAN_POINT('Origin',(-0.899999999999999,0.5,-23.46)) ;
#148782=CARTESIAN_POINT('Origin',(-0.899999999999999,-1.9,-23.46)) ;
#148783=CARTESIAN_POINT('Origin',(0.600000000000001,-1.9,-23.46)) ;
#148784=CARTESIAN_POINT('Origin',(0.500000000000001,-1.9,-23.46)) ;
#148785=CARTESIAN_POINT('Origin',(-0.899999999999999,-1.9,-23.46)) ;
#148786=CARTESIAN_POINT('Origin',(0.500000000000001,-1.9,-23.46)) ;
#148787=CARTESIAN_POINT('Origin',(0.500000000000001,-2.1,-23.46)) ;
#148788=CARTESIAN_POINT('Origin',(0.500000000000001,-2.1,-21.585)) ;
#148789=CARTESIAN_POINT('Origin',(0.500000000000001,-2.1,-21.585)) ;
#148790=CARTESIAN_POINT('Origin',(-1.1,-2.9,-21.385)) ;
#148791=CARTESIAN_POINT('Origin',(-1.1,-2.9,-21.385)) ;
#148792=CARTESIAN_POINT('Origin',(-1.1,-2.9,-21.385)) ;
#148793=CARTESIAN_POINT('Origin',(-1.1,1.25,-21.385)) ;
#148794=CARTESIAN_POINT('Origin',(-1.1,1.15,-21.385)) ;
#148795=CARTESIAN_POINT('Origin',(-1.1,1.15,-21.585)) ;
#148796=CARTESIAN_POINT('',(-1.1,1.25,-21.585)) ;
#148797=CARTESIAN_POINT('Origin',(-1.1,1.15,-21.585)) ;
#148798=CARTESIAN_POINT('Origin',(-1.1,1.15,-21.585)) ;
#148799=CARTESIAN_POINT('Origin',(-0.899999999999999,-1.9,-23.46)) ;
#148800=CARTESIAN_POINT('Origin',(-0.899999999999999,-1.9,-23.46)) ;
#148801=CARTESIAN_POINT('Origin',(0.500000000000001,-2.1,-22.86)) ;
#148802=CARTESIAN_POINT('Origin',(0.500000000000001,-2.1,-24.135)) ;
#148803=CARTESIAN_POINT('Origin',(0.500000000000001,1.36481920536411E-16,
-21.585)) ;
#148804=CARTESIAN_POINT('Origin',(0.500000000000001,-2.9,-21.585)) ;
#148805=CARTESIAN_POINT('Origin',(-0.999999999999999,-2.9,-21.385)) ;
#148806=CARTESIAN_POINT('Origin',(0.500000000000001,-2.9,-21.385)) ;
#148807=CARTESIAN_POINT('Origin',(-1.1,1.15,-21.585)) ;
#148808=CARTESIAN_POINT('Origin',(-1.1,1.35,-21.585)) ;
#148809=CARTESIAN_POINT('Origin',(-1.1,1.15,-22.86)) ;
#148810=CARTESIAN_POINT('',(-1.1,1.25,-24.135)) ;
#148811=CARTESIAN_POINT('',(-1.1,1.25,-24.235)) ;
#148812=CARTESIAN_POINT('Origin',(-1.1,1.15,-24.135)) ;
#148813=CARTESIAN_POINT('Origin',(-0.899999999999999,-1.9,-23.36)) ;
#148814=CARTESIAN_POINT('Origin',(-0.899999999999999,-1.9,-24.135)) ;
#148815=CARTESIAN_POINT('Origin',(-0.999999999999999,-2.1,-24.135)) ;
#148816=CARTESIAN_POINT('Origin',(0.500000000000001,-2.1,-24.135)) ;
#148817=CARTESIAN_POINT('Origin',(-0.899999999999999,-2.1,-24.135)) ;
#148818=CARTESIAN_POINT('Origin',(0.500000000000001,-2.1,-24.135)) ;
#148819=CARTESIAN_POINT('Origin',(0.500000000000001,-2.1,-24.135)) ;
#148820=CARTESIAN_POINT('Origin',(0.500000000000001,-2.9,-21.585)) ;
#148821=CARTESIAN_POINT('Origin',(0.700000000000002,-2.9,-21.585)) ;
#148822=CARTESIAN_POINT('Origin',(-1.1,1.35,-24.235)) ;
#148823=CARTESIAN_POINT('Origin',(-1.1,1.35,-24.135)) ;
#148824=CARTESIAN_POINT('Origin',(-1.1,1.15,-24.135)) ;
#148825=CARTESIAN_POINT('',(-1.1,1.15,-24.235)) ;
#148826=CARTESIAN_POINT('Origin',(-1.1,1.15,-24.135)) ;
#148827=CARTESIAN_POINT('Origin',(-1.1,1.15,-24.135)) ;
#148828=CARTESIAN_POINT('Origin',(-0.899999999999999,-1.9,-24.135)) ;
#148829=CARTESIAN_POINT('Origin',(-1.1,-1.9,-24.135)) ;
#148830=CARTESIAN_POINT('Origin',(0.500000000000001,-5.86744705109802E-17,
-24.135)) ;
#148831=CARTESIAN_POINT('Origin',(0.500000000000001,-2.9,-24.135)) ;
#148832=CARTESIAN_POINT('Origin',(0.700000000000002,-2.9,-22.86)) ;
#148833=CARTESIAN_POINT('Origin',(0.700000000000002,-2.9,-24.135)) ;
#148834=CARTESIAN_POINT('Origin',(-1.1,1.15,-24.135)) ;
#148835=CARTESIAN_POINT('Origin',(-1.1,1.15,-24.335)) ;
#148836=CARTESIAN_POINT('Origin',(-1.1,-2.39429110547967E-16,-24.135)) ;
#148837=CARTESIAN_POINT('',(-1.1,1.25,-24.235)) ;
#148838=CARTESIAN_POINT('Origin',(0.500000000000001,-2.9,-24.135)) ;
#148839=CARTESIAN_POINT('Origin',(0.500000000000001,-2.9,-24.335)) ;
#148840=CARTESIAN_POINT('Origin',(-1.1,1.25,-24.335)) ;
#148841=CARTESIAN_POINT('Origin',(-1.1,-2.9,-24.335)) ;
#148842=CARTESIAN_POINT('Origin',(-1.1,-2.9,-24.335)) ;
#148843=CARTESIAN_POINT('Origin',(-1.1,-2.9,-24.335)) ;
#148844=CARTESIAN_POINT('Origin',(-1.1,-2.9,-24.335)) ;
#148845=CARTESIAN_POINT('Origin',(1.5,1.9,-22.26)) ;
#148846=CARTESIAN_POINT('Origin',(1.5,1.9,-24.41)) ;
#148847=CARTESIAN_POINT('Origin',(1.5,1.9,-23.46)) ;
#148848=CARTESIAN_POINT('Origin',(1.5,2.1,-23.46)) ;
#148849=CARTESIAN_POINT('Origin',(1.5,2.1,-23.26)) ;
#148850=CARTESIAN_POINT('Origin',(1.5,1.9,-24.41)) ;
#148851=CARTESIAN_POINT('Origin',(1.5,1.9,-24.41)) ;
#148852=CARTESIAN_POINT('Origin',(1.5,2.1,-23.26)) ;
#148853=CARTESIAN_POINT('Origin',(1.5,2.4,-23.26)) ;
#148854=CARTESIAN_POINT('Origin',(1.5,2.1,-24.41)) ;
#148855=CARTESIAN_POINT('Origin',(1.5,-2.15,-24.41)) ;
#148856=CARTESIAN_POINT('Origin',(1.5,2.4,-23.46)) ;
#148857=CARTESIAN_POINT('Origin',(1.5,2.6,-23.46)) ;
#148858=CARTESIAN_POINT('Origin',(1.5,-2.15,-24.41)) ;
#148859=CARTESIAN_POINT('Origin',(1.5,-2.15,-24.41)) ;
#148860=CARTESIAN_POINT('Origin',(1.5,2.6,-22.26)) ;
#148861=CARTESIAN_POINT('Origin',(1.5,2.6,-23.5685786437627)) ;
#148862=CARTESIAN_POINT('Origin',(1.5,-2.15,-22.26)) ;
#148863=CARTESIAN_POINT('Origin',(1.5,-2.15,-23.7631195934094)) ;
#148864=CARTESIAN_POINT('Origin',(1.5,2.6,-23.5685786437627)) ;
#148865=CARTESIAN_POINT('Origin',(1.5,2.6,-23.5685786437627)) ;
#148866=CARTESIAN_POINT('Origin',(1.5,-2.15,-23.7631195934094)) ;
#148867=CARTESIAN_POINT('Origin',(1.5,-2.15,-23.7631195934094)) ;
#148868=CARTESIAN_POINT('Origin',(1.5,1.69571067811865,-22.6642893218813)) ;
#148869=CARTESIAN_POINT('Origin',(1.5,3.15,-24.1185786437627)) ;
#148870=CARTESIAN_POINT('Origin',(1.5,-3.65625,-22.86)) ;
#148871=CARTESIAN_POINT('Origin',(1.5,-2.15,-21.9568804065906)) ;
#148872=CARTESIAN_POINT('Origin',(1.5,3.15,-24.1185786437627)) ;
#148873=CARTESIAN_POINT('Origin',(1.5,3.15,-24.1185786437627)) ;
#148874=CARTESIAN_POINT('Origin',(1.5,-2.15,-21.9568804065906)) ;
#148875=CARTESIAN_POINT('Origin',(1.5,-2.15,-21.9568804065906)) ;
#148876=CARTESIAN_POINT('Origin',(1.5,3.15,-22.26)) ;
#148877=CARTESIAN_POINT('Origin',(1.5,-2.15,-22.26)) ;
#148878=CARTESIAN_POINT('Origin',(1.5,-2.15,-21.31)) ;
#148879=CARTESIAN_POINT('Origin',(1.5,-2.15,-21.31)) ;
#148880=CARTESIAN_POINT('Origin',(1.5,-2.15,-21.31)) ;
#148881=CARTESIAN_POINT('Origin',(1.5,2.29571067811866,-22.4557106781187)) ;
#148882=CARTESIAN_POINT('Origin',(1.5,2.6,-22.1514213562373)) ;
#148883=CARTESIAN_POINT('Origin',(1.5,2.1,-21.31)) ;
#148884=CARTESIAN_POINT('Origin',(1.5,1.9,-21.31)) ;
#148885=CARTESIAN_POINT('Origin',(1.5,2.6,-22.1514213562373)) ;
#148886=CARTESIAN_POINT('Origin',(1.5,2.6,-22.1514213562373)) ;
#148887=CARTESIAN_POINT('Origin',(1.5,1.9,-21.31)) ;
#148888=CARTESIAN_POINT('Origin',(1.5,1.9,-21.31)) ;
#148889=CARTESIAN_POINT('Origin',(1.5,2.6,-22.26)) ;
#148890=CARTESIAN_POINT('Origin',(1.5,2.6,-22.26)) ;
#148891=CARTESIAN_POINT('Origin',(1.5,1.9,-22.26)) ;
#148892=CARTESIAN_POINT('Origin',(1.5,1.9,-22.26)) ;
#148893=CARTESIAN_POINT('Origin',(1.5,2.4,-22.26)) ;
#148894=CARTESIAN_POINT('Origin',(1.5,2.4,-22.46)) ;
#148895=CARTESIAN_POINT('Origin',(1.5,2.1,-22.26)) ;
#148896=CARTESIAN_POINT('Origin',(1.5,2.1,-22.46)) ;
#148897=CARTESIAN_POINT('Origin',(1.5,2.1,-22.46)) ;
#148898=CARTESIAN_POINT('Origin',(-0.899999999999999,-2.,-26.07)) ;
#148899=CARTESIAN_POINT('Origin',(-0.899999999999999,0.4,-26.07)) ;
#148900=CARTESIAN_POINT('Origin',(-0.899999999999999,-1.9,-26.07)) ;
#148901=CARTESIAN_POINT('Origin',(0.600000000000001,0.4,-26.27)) ;
#148902=CARTESIAN_POINT('Origin',(0.500000000000001,0.4,-26.27)) ;
#148903=CARTESIAN_POINT('Origin',(-0.899999999999999,0.4,-26.27)) ;
#148904=CARTESIAN_POINT('Origin',(0.500000000000001,0.4,-26.27)) ;
#148905=CARTESIAN_POINT('',(0.600000000000001,0.4,-26.27)) ;
#148906=CARTESIAN_POINT('Origin',(0.500000000000001,0.4,-26.27)) ;
#148907=CARTESIAN_POINT('Origin',(0.500000000000001,0.4,-26.27)) ;
#148908=CARTESIAN_POINT('Origin',(-0.899999999999999,-1.9,-26.07)) ;
#148909=CARTESIAN_POINT('Origin',(-0.899999999999999,-1.9,-26.07)) ;
#148910=CARTESIAN_POINT('Origin',(-0.899999999999999,-1.9,-26.07)) ;
#148911=CARTESIAN_POINT('Origin',(-0.899999999999999,0.4,-26.27)) ;
#148912=CARTESIAN_POINT('Origin',(-0.899999999999999,0.6,-26.27)) ;
#148913=CARTESIAN_POINT('Origin',(0.500000000000001,0.4,-26.67)) ;
#148914=CARTESIAN_POINT('Origin',(0.500000000000001,0.4,-27.07)) ;
#148915=CARTESIAN_POINT('',(0.600000000000001,0.4,-26.97)) ;
#148916=CARTESIAN_POINT('Ctrl Pts',(0.595612997216081,0.370705721320404,
-27.0407057213204)) ;
#148917=CARTESIAN_POINT('Ctrl Pts',(0.596180587760891,0.372558268494353,
-27.0388554988322)) ;
#148918=CARTESIAN_POINT('Ctrl Pts',(0.596672461925684,0.374355839771976,
-27.0369141798663)) ;
#148919=CARTESIAN_POINT('Ctrl Pts',(0.599015141889213,0.383869350930061,
-27.0257649936563)) ;
#148920=CARTESIAN_POINT('Ctrl Pts',(0.599609996542524,0.390224332900445,
-27.0149726026541)) ;
#148921=CARTESIAN_POINT('Ctrl Pts',(0.600050586298725,0.398117439141558,
-26.9923310532047)) ;
#148922=CARTESIAN_POINT('Ctrl Pts',(0.600000000000001,0.4,-26.9812012506335)) ;
#148923=CARTESIAN_POINT('Ctrl Pts',(0.600000000000001,0.399999999999999,
-26.97)) ;
#148924=CARTESIAN_POINT('',(0.600000000000001,0.4,-26.67)) ;
#148925=CARTESIAN_POINT('Origin',(0.500000000000001,-4.56640444411542E-17,
-26.27)) ;
#148926=CARTESIAN_POINT('',(0.500000000000001,0.394987437106619,-26.37)) ;
#148927=CARTESIAN_POINT('Ctrl Pts',(0.500000000000001,0.394987437106619,
-26.37)) ;
#148928=CARTESIAN_POINT('Ctrl Pts',(0.505940567948943,0.395584486649899,
-26.37)) ;
#148929=CARTESIAN_POINT('Ctrl Pts',(0.511931971019117,0.396132036079017,
-26.369466300328)) ;
#148930=CARTESIAN_POINT('Ctrl Pts',(0.517829015308519,0.396618246075352,
-26.3683977957737)) ;
#148931=CARTESIAN_POINT('Ctrl Pts',(0.522982218721183,0.397043126556052,
-26.3674640701571)) ;
#148932=CARTESIAN_POINT('Ctrl Pts',(0.528062648970233,0.397421319341387,
-26.3661228267971)) ;
#148933=CARTESIAN_POINT('Ctrl Pts',(0.532978106724005,0.397751505046071,
-26.3644057438766)) ;
#148934=CARTESIAN_POINT('Ctrl Pts',(0.538583536338987,0.398128038183001,
-26.3624476378495)) ;
#148935=CARTESIAN_POINT('Ctrl Pts',(0.544059405914956,0.398447721828298,
-26.359970008311)) ;
#148936=CARTESIAN_POINT('Ctrl Pts',(0.549268572255855,0.398712331108987,
-26.3570207319429)) ;
#148937=CARTESIAN_POINT('Ctrl Pts',(0.553856850427182,0.398945401221758,
-26.3544229841468)) ;
#148938=CARTESIAN_POINT('Ctrl Pts',(0.558237825069334,0.399135987683844,
-26.35146038498)) ;
#148939=CARTESIAN_POINT('Ctrl Pts',(0.562333836086203,0.399290378266507,
-26.3481952228642)) ;
#148940=CARTESIAN_POINT('Ctrl Pts',(0.566990328957878,0.399465895042381,
-26.3444832689523)) ;
#148941=CARTESIAN_POINT('Ctrl Pts',(0.571349096493401,0.399597278936106,
-26.3403228064848)) ;
#148942=CARTESIAN_POINT('Ctrl Pts',(0.575296920056684,0.399694832180836,
-26.3358055759794)) ;
#148943=CARTESIAN_POINT('Ctrl Pts',(0.57874426366789,0.399780018245913,
-26.3318610112151)) ;
#148944=CARTESIAN_POINT('Ctrl Pts',(0.581878314560405,0.399839626289636,
-26.3276455218421)) ;
#148945=CARTESIAN_POINT('Ctrl Pts',(0.584648147334854,0.399882153365959,
-26.3232418177073)) ;
#148946=CARTESIAN_POINT('Ctrl Pts',(0.587839270208225,0.39993114878808,
-26.3181683125044)) ;
#148947=CARTESIAN_POINT('Ctrl Pts',(0.590595054415145,0.399958289583405,
-26.3127666362444)) ;
#148948=CARTESIAN_POINT('Ctrl Pts',(0.592838618943168,0.39997435700316,
-26.3071616850092)) ;
#148949=CARTESIAN_POINT('Ctrl Pts',(0.594777336851685,0.399988241245861,
-26.3023183122423)) ;
#148950=CARTESIAN_POINT('Ctrl Pts',(0.596334051506207,0.399993946552814,
-26.2973241662271)) ;
#148951=CARTESIAN_POINT('Ctrl Pts',(0.597488309822313,0.39999684570125,
-26.2922717185684)) ;
#148952=CARTESIAN_POINT('Ctrl Pts',(0.598804024094449,0.400000150378306,
-26.2865125419603)) ;
#148953=CARTESIAN_POINT('Ctrl Pts',(0.599612685195482,0.399999963509465,
-26.2806028438903)) ;
#148954=CARTESIAN_POINT('Ctrl Pts',(0.599890230999748,0.399999993975383,
-26.2746842022605)) ;
#148955=CARTESIAN_POINT('Ctrl Pts',(0.59996346454941,0.400000002014155,
-26.2731225027894)) ;
#148956=CARTESIAN_POINT('Ctrl Pts',(0.600000000000001,0.399999999999999,
-26.271560221509)) ;
#148957=CARTESIAN_POINT('Ctrl Pts',(0.600000000000001,0.399999999999999,
-26.27)) ;
#148958=CARTESIAN_POINT('',(0.600000000000001,0.299999999999999,-26.27)) ;
#148959=CARTESIAN_POINT('Ctrl Pts',(0.500000000000001,0.394987437106619,
-26.37)) ;
#148960=CARTESIAN_POINT('Ctrl Pts',(0.500454935590171,0.395033159853782,
-26.37)) ;
#148961=CARTESIAN_POINT('Ctrl Pts',(0.500909898680634,0.395078570329076,
-26.3699968954911)) ;
#148962=CARTESIAN_POINT('Ctrl Pts',(0.502892456244958,0.395275075889069,
-26.3699698339419)) ;
#148963=CARTESIAN_POINT('Ctrl Pts',(0.50441874748225,0.395422812032187,
-26.369913985421)) ;
#148964=CARTESIAN_POINT('Ctrl Pts',(0.508462199543321,0.395804395682031,
-26.3696732810567)) ;
#148965=CARTESIAN_POINT('Ctrl Pts',(0.510974953343264,0.396031485023314,
-26.3694279391451)) ;
#148966=CARTESIAN_POINT('Ctrl Pts',(0.521160739721166,0.396903453186226,
-26.3680427944916)) ;
#148967=CARTESIAN_POINT('Ctrl Pts',(0.528708678528252,0.397444933153152,
-26.3661042177047)) ;
#148968=CARTESIAN_POINT('Ctrl Pts',(0.545943206357825,0.398105551684101,
-26.3594646394513)) ;
#148969=CARTESIAN_POINT('Ctrl Pts',(0.555229535466584,0.397987646678453,
-26.3540353588361)) ;
#148970=CARTESIAN_POINT('Ctrl Pts',(0.571394604995541,0.395490482808082,
-26.3407755133641)) ;
#148971=CARTESIAN_POINT('Ctrl Pts',(0.578055313702682,0.393198948698442,
-26.333240745632)) ;
#148972=CARTESIAN_POINT('Ctrl Pts',(0.588559132202378,0.385442756729426,
-26.3173922339843)) ;
#148973=CARTESIAN_POINT('Ctrl Pts',(0.592167355639896,0.380240075127069,
-26.309548265607)) ;
#148974=CARTESIAN_POINT('Ctrl Pts',(0.597496615531045,0.365892753467188,
-26.2939255217955)) ;
#148975=CARTESIAN_POINT('Ctrl Pts',(0.598734255154177,0.356660564300953,
-26.2867727417271)) ;
#148976=CARTESIAN_POINT('Ctrl Pts',(0.60001275468168,0.335223914398804,
-26.2755823058657)) ;
#148977=CARTESIAN_POINT('Ctrl Pts',(0.599993900559809,0.322655037092181,
-26.2716615193656)) ;
#148978=CARTESIAN_POINT('Ctrl Pts',(0.600000296204999,0.30610691358248,
-26.2701396263471)) ;
#148979=CARTESIAN_POINT('Ctrl Pts',(0.600000000000001,0.303050992413506,
-26.27)) ;
#148980=CARTESIAN_POINT('Ctrl Pts',(0.600000000000001,0.299999999999999,
-26.27)) ;
#148981=CARTESIAN_POINT('',(0.600000000000001,-2.39800009914441E-17,-26.27)) ;
#148982=CARTESIAN_POINT('Origin',(0.500000000000001,-1.9,-26.27)) ;
#148983=CARTESIAN_POINT('Origin',(0.600000000000001,-1.9,-26.07)) ;
#148984=CARTESIAN_POINT('Origin',(0.500000000000001,-1.9,-26.07)) ;
#148985=CARTESIAN_POINT('Origin',(-0.899999999999999,-1.9,-25.295)) ;
#148986=CARTESIAN_POINT('Origin',(-0.899999999999999,-1.9,-25.395)) ;
#148987=CARTESIAN_POINT('Origin',(-0.899999999999999,0.6,-26.17)) ;
#148988=CARTESIAN_POINT('Origin',(-0.899999999999999,0.6,-27.07)) ;
#148989=CARTESIAN_POINT('Origin',(0.600000000000001,0.4,-27.07)) ;
#148990=CARTESIAN_POINT('Origin',(0.500000000000001,0.4,-27.07)) ;
#148991=CARTESIAN_POINT('Origin',(-0.899999999999999,0.4,-27.07)) ;
#148992=CARTESIAN_POINT('Origin',(0.500000000000001,0.4,-27.07)) ;
#148993=CARTESIAN_POINT('Origin',(0.500000000000001,-1.9,-26.07)) ;
#148994=CARTESIAN_POINT('Origin',(0.500000000000001,-2.1,-26.07)) ;
#148995=CARTESIAN_POINT('Origin',(-0.899999999999999,-1.9,-25.395)) ;
#148996=CARTESIAN_POINT('Origin',(-1.1,-1.9,-25.395)) ;
#148997=CARTESIAN_POINT('Origin',(-0.899999999999999,-2.1,-25.395)) ;
#148998=CARTESIAN_POINT('Origin',(-0.899999999999999,0.4,-27.07)) ;
#148999=CARTESIAN_POINT('Origin',(-0.899999999999999,0.4,-27.27)) ;
#149000=CARTESIAN_POINT('Origin',(0.500000000000001,-2.1,-26.67)) ;
#149001=CARTESIAN_POINT('Origin',(0.500000000000001,-2.1,-25.395)) ;
#149002=CARTESIAN_POINT('Origin',(0.600000000000001,-2.1,-25.395)) ;
#149003=CARTESIAN_POINT('Origin',(0.500000000000001,-2.1,-25.395)) ;
#149004=CARTESIAN_POINT('Origin',(-1.1,-4.42727195005762E-17,-25.395)) ;
#149005=CARTESIAN_POINT('',(-1.1,1.15,-25.295)) ;
#149006=CARTESIAN_POINT('',(-1.1,1.25,-25.295)) ;
#149007=CARTESIAN_POINT('Origin',(-1.1,1.15,-25.395)) ;
#149008=CARTESIAN_POINT('Origin',(-0.899999999999999,0.5,-27.27)) ;
#149009=CARTESIAN_POINT('Origin',(-0.899999999999999,-1.9,-27.27)) ;
#149010=CARTESIAN_POINT('Origin',(0.600000000000001,-1.9,-27.27)) ;
#149011=CARTESIAN_POINT('Origin',(0.500000000000001,-1.9,-27.27)) ;
#149012=CARTESIAN_POINT('Origin',(-0.899999999999999,-1.9,-27.27)) ;
#149013=CARTESIAN_POINT('Origin',(0.500000000000001,-1.9,-27.27)) ;
#149014=CARTESIAN_POINT('Origin',(0.500000000000001,-2.1,-27.27)) ;
#149015=CARTESIAN_POINT('Origin',(0.500000000000001,-2.1,-25.395)) ;
#149016=CARTESIAN_POINT('Origin',(0.500000000000001,-2.1,-25.395)) ;
#149017=CARTESIAN_POINT('Origin',(-1.1,-2.9,-25.195)) ;
#149018=CARTESIAN_POINT('Origin',(-1.1,-2.9,-25.195)) ;
#149019=CARTESIAN_POINT('Origin',(-1.1,-2.9,-25.195)) ;
#149020=CARTESIAN_POINT('Origin',(-1.1,1.25,-25.195)) ;
#149021=CARTESIAN_POINT('Origin',(-1.1,1.15,-25.195)) ;
#149022=CARTESIAN_POINT('Origin',(-1.1,1.15,-25.395)) ;
#149023=CARTESIAN_POINT('',(-1.1,1.25,-25.395)) ;
#149024=CARTESIAN_POINT('Origin',(-1.1,1.15,-25.395)) ;
#149025=CARTESIAN_POINT('Origin',(-1.1,1.15,-25.395)) ;
#149026=CARTESIAN_POINT('Origin',(-0.899999999999999,-1.9,-27.27)) ;
#149027=CARTESIAN_POINT('Origin',(-0.899999999999999,-1.9,-27.27)) ;
#149028=CARTESIAN_POINT('Origin',(0.500000000000001,-2.1,-26.67)) ;
#149029=CARTESIAN_POINT('Origin',(0.500000000000001,-2.1,-27.945)) ;
#149030=CARTESIAN_POINT('Origin',(0.500000000000001,1.36481920536411E-16,
-25.395)) ;
#149031=CARTESIAN_POINT('Origin',(0.500000000000001,-2.9,-25.395)) ;
#149032=CARTESIAN_POINT('Origin',(-0.999999999999999,-2.9,-25.195)) ;
#149033=CARTESIAN_POINT('Origin',(0.500000000000001,-2.9,-25.195)) ;
#149034=CARTESIAN_POINT('Origin',(-1.1,1.15,-25.395)) ;
#149035=CARTESIAN_POINT('Origin',(-1.1,1.35,-25.395)) ;
#149036=CARTESIAN_POINT('Origin',(-1.1,1.15,-26.67)) ;
#149037=CARTESIAN_POINT('',(-1.1,1.25,-27.945)) ;
#149038=CARTESIAN_POINT('',(-1.1,1.25,-28.045)) ;
#149039=CARTESIAN_POINT('Origin',(-1.1,1.15,-27.945)) ;
#149040=CARTESIAN_POINT('Origin',(-0.899999999999999,-1.9,-27.17)) ;
#149041=CARTESIAN_POINT('Origin',(-0.899999999999999,-1.9,-27.945)) ;
#149042=CARTESIAN_POINT('Origin',(-0.999999999999999,-2.1,-27.945)) ;
#149043=CARTESIAN_POINT('Origin',(0.500000000000001,-2.1,-27.945)) ;
#149044=CARTESIAN_POINT('Origin',(-0.899999999999999,-2.1,-27.945)) ;
#149045=CARTESIAN_POINT('Origin',(0.500000000000001,-2.1,-27.945)) ;
#149046=CARTESIAN_POINT('Origin',(0.500000000000001,-2.1,-27.945)) ;
#149047=CARTESIAN_POINT('Origin',(0.500000000000001,-2.9,-25.395)) ;
#149048=CARTESIAN_POINT('Origin',(0.700000000000002,-2.9,-25.395)) ;
#149049=CARTESIAN_POINT('Origin',(-1.1,1.35,-28.045)) ;
#149050=CARTESIAN_POINT('Origin',(-1.1,1.35,-27.945)) ;
#149051=CARTESIAN_POINT('Origin',(-1.1,1.15,-27.945)) ;
#149052=CARTESIAN_POINT('',(-1.1,1.15,-28.045)) ;
#149053=CARTESIAN_POINT('Origin',(-1.1,1.15,-27.945)) ;
#149054=CARTESIAN_POINT('Origin',(-1.1,1.15,-27.945)) ;
#149055=CARTESIAN_POINT('Origin',(-0.899999999999999,-1.9,-27.945)) ;
#149056=CARTESIAN_POINT('Origin',(-1.1,-1.9,-27.945)) ;
#149057=CARTESIAN_POINT('Origin',(0.500000000000001,-5.86744705109802E-17,
-27.945)) ;
#149058=CARTESIAN_POINT('Origin',(0.500000000000001,-2.9,-27.945)) ;
#149059=CARTESIAN_POINT('Origin',(0.700000000000002,-2.9,-26.67)) ;
#149060=CARTESIAN_POINT('Origin',(0.700000000000002,-2.9,-27.945)) ;
#149061=CARTESIAN_POINT('Origin',(-1.1,1.15,-27.945)) ;
#149062=CARTESIAN_POINT('Origin',(-1.1,1.15,-28.145)) ;
#149063=CARTESIAN_POINT('Origin',(-1.1,-2.39429110547967E-16,-27.945)) ;
#149064=CARTESIAN_POINT('',(-1.1,1.25,-28.045)) ;
#149065=CARTESIAN_POINT('Origin',(0.500000000000001,-2.9,-27.945)) ;
#149066=CARTESIAN_POINT('Origin',(0.500000000000001,-2.9,-28.145)) ;
#149067=CARTESIAN_POINT('Origin',(-1.1,1.25,-28.145)) ;
#149068=CARTESIAN_POINT('Origin',(-1.1,-2.9,-28.145)) ;
#149069=CARTESIAN_POINT('Origin',(-1.1,-2.9,-28.145)) ;
#149070=CARTESIAN_POINT('Origin',(-1.1,-2.9,-28.145)) ;
#149071=CARTESIAN_POINT('Origin',(-1.1,-2.9,-28.145)) ;
#149072=CARTESIAN_POINT('Origin',(1.5,1.9,-26.07)) ;
#149073=CARTESIAN_POINT('Origin',(1.5,1.9,-28.22)) ;
#149074=CARTESIAN_POINT('Origin',(1.5,1.9,-27.27)) ;
#149075=CARTESIAN_POINT('Origin',(1.5,2.1,-27.27)) ;
#149076=CARTESIAN_POINT('Origin',(1.5,2.1,-27.07)) ;
#149077=CARTESIAN_POINT('Origin',(1.5,1.9,-28.22)) ;
#149078=CARTESIAN_POINT('Origin',(1.5,1.9,-28.22)) ;
#149079=CARTESIAN_POINT('Origin',(1.5,2.1,-27.07)) ;
#149080=CARTESIAN_POINT('Origin',(1.5,2.4,-27.07)) ;
#149081=CARTESIAN_POINT('Origin',(1.5,2.1,-28.22)) ;
#149082=CARTESIAN_POINT('Origin',(1.5,-2.15,-28.22)) ;
#149083=CARTESIAN_POINT('Origin',(1.5,2.4,-27.27)) ;
#149084=CARTESIAN_POINT('Origin',(1.5,2.6,-27.27)) ;
#149085=CARTESIAN_POINT('Origin',(1.5,-2.15,-28.22)) ;
#149086=CARTESIAN_POINT('Origin',(1.5,-2.15,-28.22)) ;
#149087=CARTESIAN_POINT('Origin',(1.5,2.6,-26.07)) ;
#149088=CARTESIAN_POINT('Origin',(1.5,2.6,-27.3785786437627)) ;
#149089=CARTESIAN_POINT('Origin',(1.5,-2.15,-26.07)) ;
#149090=CARTESIAN_POINT('Origin',(1.5,-2.15,-27.5731195934094)) ;
#149091=CARTESIAN_POINT('Origin',(1.5,2.6,-27.3785786437627)) ;
#149092=CARTESIAN_POINT('Origin',(1.5,2.6,-27.3785786437627)) ;
#149093=CARTESIAN_POINT('Origin',(1.5,-2.15,-27.5731195934094)) ;
#149094=CARTESIAN_POINT('Origin',(1.5,-2.15,-27.5731195934094)) ;
#149095=CARTESIAN_POINT('Origin',(1.5,1.69571067811865,-26.4742893218813)) ;
#149096=CARTESIAN_POINT('Origin',(1.5,3.15,-27.9285786437627)) ;
#149097=CARTESIAN_POINT('Origin',(1.5,-3.65625,-26.67)) ;
#149098=CARTESIAN_POINT('Origin',(1.5,-2.15,-25.7668804065906)) ;
#149099=CARTESIAN_POINT('Origin',(1.5,3.15,-27.9285786437627)) ;
#149100=CARTESIAN_POINT('Origin',(1.5,3.15,-27.9285786437627)) ;
#149101=CARTESIAN_POINT('Origin',(1.5,-2.15,-25.7668804065906)) ;
#149102=CARTESIAN_POINT('Origin',(1.5,-2.15,-25.7668804065906)) ;
#149103=CARTESIAN_POINT('Origin',(1.5,3.15,-26.07)) ;
#149104=CARTESIAN_POINT('Origin',(1.5,-2.15,-26.07)) ;
#149105=CARTESIAN_POINT('Origin',(1.5,-2.15,-25.12)) ;
#149106=CARTESIAN_POINT('Origin',(1.5,-2.15,-25.12)) ;
#149107=CARTESIAN_POINT('Origin',(1.5,-2.15,-25.12)) ;
#149108=CARTESIAN_POINT('Origin',(1.5,2.29571067811866,-26.2657106781187)) ;
#149109=CARTESIAN_POINT('Origin',(1.5,2.6,-25.9614213562373)) ;
#149110=CARTESIAN_POINT('Origin',(1.5,2.1,-25.12)) ;
#149111=CARTESIAN_POINT('Origin',(1.5,1.9,-25.12)) ;
#149112=CARTESIAN_POINT('Origin',(1.5,2.6,-25.9614213562373)) ;
#149113=CARTESIAN_POINT('Origin',(1.5,2.6,-25.9614213562373)) ;
#149114=CARTESIAN_POINT('Origin',(1.5,1.9,-25.12)) ;
#149115=CARTESIAN_POINT('Origin',(1.5,1.9,-25.12)) ;
#149116=CARTESIAN_POINT('Origin',(1.5,2.6,-26.07)) ;
#149117=CARTESIAN_POINT('Origin',(1.5,2.6,-26.07)) ;
#149118=CARTESIAN_POINT('Origin',(1.5,1.9,-26.07)) ;
#149119=CARTESIAN_POINT('Origin',(1.5,1.9,-26.07)) ;
#149120=CARTESIAN_POINT('Origin',(1.5,2.4,-26.07)) ;
#149121=CARTESIAN_POINT('Origin',(1.5,2.4,-26.27)) ;
#149122=CARTESIAN_POINT('Origin',(1.5,2.1,-26.07)) ;
#149123=CARTESIAN_POINT('Origin',(1.5,2.1,-26.27)) ;
#149124=CARTESIAN_POINT('Origin',(1.5,2.1,-26.27)) ;
#149125=CARTESIAN_POINT('Origin',(-0.899999999999999,-2.,-29.88)) ;
#149126=CARTESIAN_POINT('Origin',(-0.899999999999999,0.4,-29.88)) ;
#149127=CARTESIAN_POINT('Origin',(-0.899999999999999,-1.9,-29.88)) ;
#149128=CARTESIAN_POINT('Origin',(0.600000000000001,0.4,-30.08)) ;
#149129=CARTESIAN_POINT('Origin',(0.500000000000001,0.4,-30.08)) ;
#149130=CARTESIAN_POINT('Origin',(-0.899999999999999,0.4,-30.08)) ;
#149131=CARTESIAN_POINT('Origin',(0.500000000000001,0.4,-30.08)) ;
#149132=CARTESIAN_POINT('',(0.600000000000001,0.4,-30.08)) ;
#149133=CARTESIAN_POINT('Origin',(0.500000000000001,0.4,-30.08)) ;
#149134=CARTESIAN_POINT('Origin',(0.500000000000001,0.4,-30.08)) ;
#149135=CARTESIAN_POINT('Origin',(-0.899999999999999,-1.9,-29.88)) ;
#149136=CARTESIAN_POINT('Origin',(-0.899999999999999,-1.9,-29.88)) ;
#149137=CARTESIAN_POINT('Origin',(-0.899999999999999,-1.9,-29.88)) ;
#149138=CARTESIAN_POINT('Origin',(-0.899999999999999,0.4,-30.08)) ;
#149139=CARTESIAN_POINT('Origin',(-0.899999999999999,0.6,-30.08)) ;
#149140=CARTESIAN_POINT('Origin',(0.500000000000001,0.4,-30.48)) ;
#149141=CARTESIAN_POINT('Origin',(0.500000000000001,0.4,-30.88)) ;
#149142=CARTESIAN_POINT('',(0.600000000000001,0.4,-30.78)) ;
#149143=CARTESIAN_POINT('Ctrl Pts',(0.595612997216081,0.370705721320405,
-30.8507057213204)) ;
#149144=CARTESIAN_POINT('Ctrl Pts',(0.596180587760891,0.372558268494354,
-30.8488554988322)) ;
#149145=CARTESIAN_POINT('Ctrl Pts',(0.596672461925684,0.374355839771976,
-30.8469141798663)) ;
#149146=CARTESIAN_POINT('Ctrl Pts',(0.599015141889203,0.383869350930023,
-30.8357649936563)) ;
#149147=CARTESIAN_POINT('Ctrl Pts',(0.599609996542522,0.390224332900425,
-30.8249726026542)) ;
#149148=CARTESIAN_POINT('Ctrl Pts',(0.600050586298725,0.398117439141557,
-30.8023310532047)) ;
#149149=CARTESIAN_POINT('Ctrl Pts',(0.600000000000001,0.399999999999999,
-30.7912012506335)) ;
#149150=CARTESIAN_POINT('Ctrl Pts',(0.600000000000001,0.399999999999999,
-30.78)) ;
#149151=CARTESIAN_POINT('',(0.600000000000001,0.4,-30.48)) ;
#149152=CARTESIAN_POINT('Origin',(0.500000000000001,-4.56640444411542E-17,
-30.08)) ;
#149153=CARTESIAN_POINT('',(0.500000000000001,0.394987437106619,-30.18)) ;
#149154=CARTESIAN_POINT('Ctrl Pts',(0.500000000000001,0.394987437106619,
-30.18)) ;
#149155=CARTESIAN_POINT('Ctrl Pts',(0.505940567948935,0.395584486649899,
-30.18)) ;
#149156=CARTESIAN_POINT('Ctrl Pts',(0.511931971019101,0.396132036079015,
-30.179466300328)) ;
#149157=CARTESIAN_POINT('Ctrl Pts',(0.517829015308496,0.39661824607535,
-30.1783977957737)) ;
#149158=CARTESIAN_POINT('Ctrl Pts',(0.522982218721168,0.397043126556051,
-30.1774640701571)) ;
#149159=CARTESIAN_POINT('Ctrl Pts',(0.528062648970226,0.397421319341387,
-30.1761228267971)) ;
#149160=CARTESIAN_POINT('Ctrl Pts',(0.532978106724004,0.397751505046071,
-30.1744057438766)) ;
#149161=CARTESIAN_POINT('Ctrl Pts',(0.538583536338982,0.398128038183001,
-30.1724476378495)) ;
#149162=CARTESIAN_POINT('Ctrl Pts',(0.544059405914951,0.398447721828298,
-30.169970008311)) ;
#149163=CARTESIAN_POINT('Ctrl Pts',(0.549268572255847,0.398712331108986,
-30.1670207319429)) ;
#149164=CARTESIAN_POINT('Ctrl Pts',(0.553856850427178,0.398945401221757,
-30.1644229841468)) ;
#149165=CARTESIAN_POINT('Ctrl Pts',(0.558237825069329,0.399135987683843,
-30.16146038498)) ;
#149166=CARTESIAN_POINT('Ctrl Pts',(0.562333836086197,0.399290378266506,
-30.1581952228642)) ;
#149167=CARTESIAN_POINT('Ctrl Pts',(0.566990328957886,0.399465895042381,
-30.1544832689523)) ;
#149168=CARTESIAN_POINT('Ctrl Pts',(0.57134909649342,0.399597278936108,
-30.1503228064848)) ;
#149169=CARTESIAN_POINT('Ctrl Pts',(0.575296920056715,0.399694832180838,
-30.1458055759793)) ;
#149170=CARTESIAN_POINT('Ctrl Pts',(0.5787442636679,0.399780018245914,-30.1418610112151)) ;
#149171=CARTESIAN_POINT('Ctrl Pts',(0.581878314560451,0.399839626289636,
-30.1376455218421)) ;
#149172=CARTESIAN_POINT('Ctrl Pts',(0.584648147334861,0.399882153365958,
-30.1332418177073)) ;
#149173=CARTESIAN_POINT('Ctrl Pts',(0.587839270208171,0.399931148788079,
-30.1281683125045)) ;
#149174=CARTESIAN_POINT('Ctrl Pts',(0.590595054415091,0.399958289583404,
-30.1227666362445)) ;
#149175=CARTESIAN_POINT('Ctrl Pts',(0.592838618943106,0.399974357003159,
-30.1171616850094)) ;
#149176=CARTESIAN_POINT('Ctrl Pts',(0.594777336851655,0.399988241245861,
-30.1123183122424)) ;
#149177=CARTESIAN_POINT('Ctrl Pts',(0.596334051506183,0.399993946552814,
-30.1073241662271)) ;
#149178=CARTESIAN_POINT('Ctrl Pts',(0.597488309822302,0.39999684570125,
-30.1022717185684)) ;
#149179=CARTESIAN_POINT('Ctrl Pts',(0.598804024094428,0.400000150378306,
-30.0965125419604)) ;
#149180=CARTESIAN_POINT('Ctrl Pts',(0.599612685195468,0.399999963509465,
-30.0906028438904)) ;
#149181=CARTESIAN_POINT('Ctrl Pts',(0.599890230999741,0.399999993975383,
-30.0846842022606)) ;
#149182=CARTESIAN_POINT('Ctrl Pts',(0.599963464549407,0.400000002014155,
-30.0831225027895)) ;
#149183=CARTESIAN_POINT('Ctrl Pts',(0.600000000000001,0.399999999999999,
-30.081560221509)) ;
#149184=CARTESIAN_POINT('Ctrl Pts',(0.600000000000001,0.399999999999999,
-30.08)) ;
#149185=CARTESIAN_POINT('',(0.600000000000001,0.299999999999999,-30.08)) ;
#149186=CARTESIAN_POINT('Ctrl Pts',(0.500000000000001,0.394987437106619,
-30.18)) ;
#149187=CARTESIAN_POINT('Ctrl Pts',(0.500454935590171,0.395033159853782,
-30.18)) ;
#149188=CARTESIAN_POINT('Ctrl Pts',(0.500909898680634,0.395078570329076,
-30.1799968954911)) ;
#149189=CARTESIAN_POINT('Ctrl Pts',(0.502892456244958,0.395275075889069,
-30.1799698339419)) ;
#149190=CARTESIAN_POINT('Ctrl Pts',(0.50441874748225,0.395422812032187,
-30.179913985421)) ;
#149191=CARTESIAN_POINT('Ctrl Pts',(0.508462199543321,0.395804395682031,
-30.1796732810567)) ;
#149192=CARTESIAN_POINT('Ctrl Pts',(0.510974953343264,0.396031485023314,
-30.1794279391451)) ;
#149193=CARTESIAN_POINT('Ctrl Pts',(0.521160739721166,0.396903453186226,
-30.1780427944916)) ;
#149194=CARTESIAN_POINT('Ctrl Pts',(0.528708678528252,0.397444933153152,
-30.1761042177047)) ;
#149195=CARTESIAN_POINT('Ctrl Pts',(0.545943206357825,0.398105551684101,
-30.1694646394513)) ;
#149196=CARTESIAN_POINT('Ctrl Pts',(0.555229535466584,0.397987646678453,
-30.1640353588361)) ;
#149197=CARTESIAN_POINT('Ctrl Pts',(0.571394604995541,0.395490482808082,
-30.150775513364)) ;
#149198=CARTESIAN_POINT('Ctrl Pts',(0.578055313702682,0.393198948698442,
-30.143240745632)) ;
#149199=CARTESIAN_POINT('Ctrl Pts',(0.588559132202378,0.385442756729426,
-30.1273922339842)) ;
#149200=CARTESIAN_POINT('Ctrl Pts',(0.592167355639896,0.380240075127069,
-30.119548265607)) ;
#149201=CARTESIAN_POINT('Ctrl Pts',(0.597496615531045,0.365892753467188,
-30.1039255217955)) ;
#149202=CARTESIAN_POINT('Ctrl Pts',(0.598734255154177,0.356660564300953,
-30.0967727417271)) ;
#149203=CARTESIAN_POINT('Ctrl Pts',(0.60001275468168,0.335223914398804,
-30.0855823058657)) ;
#149204=CARTESIAN_POINT('Ctrl Pts',(0.599993900559809,0.322655037092181,
-30.0816615193656)) ;
#149205=CARTESIAN_POINT('Ctrl Pts',(0.600000296204999,0.30610691358248,
-30.0801396263471)) ;
#149206=CARTESIAN_POINT('Ctrl Pts',(0.600000000000001,0.303050992413506,
-30.08)) ;
#149207=CARTESIAN_POINT('Ctrl Pts',(0.600000000000001,0.299999999999999,
-30.08)) ;
#149208=CARTESIAN_POINT('',(0.600000000000001,-2.39800009914441E-17,-30.08)) ;
#149209=CARTESIAN_POINT('Origin',(0.500000000000001,-1.9,-30.08)) ;
#149210=CARTESIAN_POINT('Origin',(0.600000000000001,-1.9,-29.88)) ;
#149211=CARTESIAN_POINT('Origin',(0.500000000000001,-1.9,-29.88)) ;
#149212=CARTESIAN_POINT('Origin',(-0.899999999999999,-1.9,-29.105)) ;
#149213=CARTESIAN_POINT('Origin',(-0.899999999999999,-1.9,-29.205)) ;
#149214=CARTESIAN_POINT('Origin',(-0.899999999999999,0.6,-29.98)) ;
#149215=CARTESIAN_POINT('Origin',(-0.899999999999999,0.6,-30.88)) ;
#149216=CARTESIAN_POINT('Origin',(0.600000000000001,0.4,-30.88)) ;
#149217=CARTESIAN_POINT('Origin',(0.500000000000001,0.4,-30.88)) ;
#149218=CARTESIAN_POINT('Origin',(-0.899999999999999,0.4,-30.88)) ;
#149219=CARTESIAN_POINT('Origin',(0.500000000000001,0.4,-30.88)) ;
#149220=CARTESIAN_POINT('Origin',(0.500000000000001,-1.9,-29.88)) ;
#149221=CARTESIAN_POINT('Origin',(0.500000000000001,-2.1,-29.88)) ;
#149222=CARTESIAN_POINT('Origin',(-0.899999999999999,-1.9,-29.205)) ;
#149223=CARTESIAN_POINT('Origin',(-1.1,-1.9,-29.205)) ;
#149224=CARTESIAN_POINT('Origin',(-0.899999999999999,-2.1,-29.205)) ;
#149225=CARTESIAN_POINT('Origin',(-0.899999999999999,0.4,-30.88)) ;
#149226=CARTESIAN_POINT('Origin',(-0.899999999999999,0.4,-31.08)) ;
#149227=CARTESIAN_POINT('Origin',(0.500000000000001,-2.1,-30.48)) ;
#149228=CARTESIAN_POINT('Origin',(0.500000000000001,-2.1,-29.205)) ;
#149229=CARTESIAN_POINT('Origin',(0.600000000000001,-2.1,-29.205)) ;
#149230=CARTESIAN_POINT('Origin',(0.500000000000001,-2.1,-29.205)) ;
#149231=CARTESIAN_POINT('Origin',(-1.1,-4.42727195005762E-17,-29.205)) ;
#149232=CARTESIAN_POINT('',(-1.1,1.15,-29.105)) ;
#149233=CARTESIAN_POINT('',(-1.1,1.25,-29.105)) ;
#149234=CARTESIAN_POINT('Origin',(-1.1,1.15,-29.205)) ;
#149235=CARTESIAN_POINT('Origin',(-0.899999999999999,0.5,-31.08)) ;
#149236=CARTESIAN_POINT('Origin',(-0.899999999999999,-1.9,-31.08)) ;
#149237=CARTESIAN_POINT('Origin',(0.600000000000001,-1.9,-31.08)) ;
#149238=CARTESIAN_POINT('Origin',(0.500000000000001,-1.9,-31.08)) ;
#149239=CARTESIAN_POINT('Origin',(-0.899999999999999,-1.9,-31.08)) ;
#149240=CARTESIAN_POINT('Origin',(0.500000000000001,-1.9,-31.08)) ;
#149241=CARTESIAN_POINT('Origin',(0.500000000000001,-2.1,-31.08)) ;
#149242=CARTESIAN_POINT('Origin',(0.500000000000001,-2.1,-29.205)) ;
#149243=CARTESIAN_POINT('Origin',(0.500000000000001,-2.1,-29.205)) ;
#149244=CARTESIAN_POINT('Origin',(-1.1,-2.9,-29.005)) ;
#149245=CARTESIAN_POINT('Origin',(-1.1,-2.9,-29.005)) ;
#149246=CARTESIAN_POINT('Origin',(-1.1,-2.9,-29.005)) ;
#149247=CARTESIAN_POINT('Origin',(-1.1,1.25,-29.005)) ;
#149248=CARTESIAN_POINT('Origin',(-1.1,1.15,-29.005)) ;
#149249=CARTESIAN_POINT('Origin',(-1.1,1.15,-29.205)) ;
#149250=CARTESIAN_POINT('',(-1.1,1.25,-29.205)) ;
#149251=CARTESIAN_POINT('Origin',(-1.1,1.15,-29.205)) ;
#149252=CARTESIAN_POINT('Origin',(-1.1,1.15,-29.205)) ;
#149253=CARTESIAN_POINT('Origin',(-0.899999999999999,-1.9,-31.08)) ;
#149254=CARTESIAN_POINT('Origin',(-0.899999999999999,-1.9,-31.08)) ;
#149255=CARTESIAN_POINT('Origin',(0.500000000000001,-2.1,-30.48)) ;
#149256=CARTESIAN_POINT('Origin',(0.500000000000001,-2.1,-31.755)) ;
#149257=CARTESIAN_POINT('Origin',(0.500000000000001,1.36481920536411E-16,
-29.205)) ;
#149258=CARTESIAN_POINT('Origin',(0.500000000000001,-2.9,-29.205)) ;
#149259=CARTESIAN_POINT('Origin',(-0.999999999999999,-2.9,-29.005)) ;
#149260=CARTESIAN_POINT('Origin',(0.500000000000001,-2.9,-29.005)) ;
#149261=CARTESIAN_POINT('Origin',(-1.1,1.15,-29.205)) ;
#149262=CARTESIAN_POINT('Origin',(-1.1,1.35,-29.205)) ;
#149263=CARTESIAN_POINT('Origin',(-1.1,1.15,-30.48)) ;
#149264=CARTESIAN_POINT('',(-1.1,1.25,-31.755)) ;
#149265=CARTESIAN_POINT('',(-1.1,1.25,-31.855)) ;
#149266=CARTESIAN_POINT('Origin',(-1.1,1.15,-31.755)) ;
#149267=CARTESIAN_POINT('Origin',(-0.899999999999999,-1.9,-30.98)) ;
#149268=CARTESIAN_POINT('Origin',(-0.899999999999999,-1.9,-31.755)) ;
#149269=CARTESIAN_POINT('Origin',(-0.999999999999999,-2.1,-31.755)) ;
#149270=CARTESIAN_POINT('Origin',(0.500000000000001,-2.1,-31.755)) ;
#149271=CARTESIAN_POINT('Origin',(-0.899999999999999,-2.1,-31.755)) ;
#149272=CARTESIAN_POINT('Origin',(0.500000000000001,-2.1,-31.755)) ;
#149273=CARTESIAN_POINT('Origin',(0.500000000000001,-2.1,-31.755)) ;
#149274=CARTESIAN_POINT('Origin',(0.500000000000001,-2.9,-29.205)) ;
#149275=CARTESIAN_POINT('Origin',(0.700000000000002,-2.9,-29.205)) ;
#149276=CARTESIAN_POINT('Origin',(-1.1,1.35,-31.855)) ;
#149277=CARTESIAN_POINT('Origin',(-1.1,1.35,-31.755)) ;
#149278=CARTESIAN_POINT('Origin',(-1.1,1.15,-31.755)) ;
#149279=CARTESIAN_POINT('',(-1.1,1.15,-31.855)) ;
#149280=CARTESIAN_POINT('Origin',(-1.1,1.15,-31.755)) ;
#149281=CARTESIAN_POINT('Origin',(-1.1,1.15,-31.755)) ;
#149282=CARTESIAN_POINT('Origin',(-0.899999999999999,-1.9,-31.755)) ;
#149283=CARTESIAN_POINT('Origin',(-1.1,-1.9,-31.755)) ;
#149284=CARTESIAN_POINT('Origin',(0.500000000000001,-5.867447051098E-17,
-31.755)) ;
#149285=CARTESIAN_POINT('Origin',(0.500000000000001,-2.9,-31.755)) ;
#149286=CARTESIAN_POINT('Origin',(0.700000000000002,-2.9,-30.48)) ;
#149287=CARTESIAN_POINT('Origin',(0.700000000000002,-2.9,-31.755)) ;
#149288=CARTESIAN_POINT('Origin',(-1.1,1.15,-31.755)) ;
#149289=CARTESIAN_POINT('Origin',(-1.1,1.15,-31.955)) ;
#149290=CARTESIAN_POINT('Origin',(-1.1,-2.39429110547967E-16,-31.755)) ;
#149291=CARTESIAN_POINT('',(-1.1,1.25,-31.855)) ;
#149292=CARTESIAN_POINT('Origin',(0.500000000000001,-2.9,-31.755)) ;
#149293=CARTESIAN_POINT('Origin',(0.500000000000001,-2.9,-31.955)) ;
#149294=CARTESIAN_POINT('Origin',(-1.1,1.25,-31.955)) ;
#149295=CARTESIAN_POINT('Origin',(-1.1,-2.9,-31.955)) ;
#149296=CARTESIAN_POINT('Origin',(-1.1,-2.9,-31.955)) ;
#149297=CARTESIAN_POINT('Origin',(-1.1,-2.9,-31.955)) ;
#149298=CARTESIAN_POINT('Origin',(-1.1,-2.9,-31.955)) ;
#149299=CARTESIAN_POINT('Origin',(1.5,1.9,-29.88)) ;
#149300=CARTESIAN_POINT('Origin',(1.5,1.9,-32.03)) ;
#149301=CARTESIAN_POINT('Origin',(1.5,1.9,-31.08)) ;
#149302=CARTESIAN_POINT('Origin',(1.5,2.1,-31.08)) ;
#149303=CARTESIAN_POINT('Origin',(1.5,2.1,-30.88)) ;
#149304=CARTESIAN_POINT('Origin',(1.5,1.9,-32.03)) ;
#149305=CARTESIAN_POINT('Origin',(1.5,1.9,-32.03)) ;
#149306=CARTESIAN_POINT('Origin',(1.5,2.1,-30.88)) ;
#149307=CARTESIAN_POINT('Origin',(1.5,2.4,-30.88)) ;
#149308=CARTESIAN_POINT('Origin',(1.5,2.1,-32.03)) ;
#149309=CARTESIAN_POINT('Origin',(1.5,-2.15,-32.03)) ;
#149310=CARTESIAN_POINT('Origin',(1.5,2.4,-31.08)) ;
#149311=CARTESIAN_POINT('Origin',(1.5,2.6,-31.08)) ;
#149312=CARTESIAN_POINT('Origin',(1.5,-2.15,-32.03)) ;
#149313=CARTESIAN_POINT('Origin',(1.5,-2.15,-32.03)) ;
#149314=CARTESIAN_POINT('Origin',(1.5,2.6,-29.88)) ;
#149315=CARTESIAN_POINT('Origin',(1.5,2.6,-31.1885786437627)) ;
#149316=CARTESIAN_POINT('Origin',(1.5,-2.15,-29.88)) ;
#149317=CARTESIAN_POINT('Origin',(1.5,-2.15,-31.3831195934094)) ;
#149318=CARTESIAN_POINT('Origin',(1.5,2.6,-31.1885786437627)) ;
#149319=CARTESIAN_POINT('Origin',(1.5,2.6,-31.1885786437627)) ;
#149320=CARTESIAN_POINT('Origin',(1.5,-2.15,-31.3831195934094)) ;
#149321=CARTESIAN_POINT('Origin',(1.5,-2.15,-31.3831195934094)) ;
#149322=CARTESIAN_POINT('Origin',(1.5,1.69571067811865,-30.2842893218813)) ;
#149323=CARTESIAN_POINT('Origin',(1.5,3.15,-31.7385786437627)) ;
#149324=CARTESIAN_POINT('Origin',(1.5,-3.65625,-30.48)) ;
#149325=CARTESIAN_POINT('Origin',(1.5,-2.15,-29.5768804065906)) ;
#149326=CARTESIAN_POINT('Origin',(1.5,3.15,-31.7385786437627)) ;
#149327=CARTESIAN_POINT('Origin',(1.5,3.15,-31.7385786437627)) ;
#149328=CARTESIAN_POINT('Origin',(1.5,-2.15,-29.5768804065906)) ;
#149329=CARTESIAN_POINT('Origin',(1.5,-2.15,-29.5768804065906)) ;
#149330=CARTESIAN_POINT('Origin',(1.5,3.15,-29.88)) ;
#149331=CARTESIAN_POINT('Origin',(1.5,-2.15,-29.88)) ;
#149332=CARTESIAN_POINT('Origin',(1.5,-2.15,-28.93)) ;
#149333=CARTESIAN_POINT('Origin',(1.5,-2.15,-28.93)) ;
#149334=CARTESIAN_POINT('Origin',(1.5,-2.15,-28.93)) ;
#149335=CARTESIAN_POINT('Origin',(1.5,2.29571067811866,-30.0757106781187)) ;
#149336=CARTESIAN_POINT('Origin',(1.5,2.6,-29.7714213562373)) ;
#149337=CARTESIAN_POINT('Origin',(1.5,2.1,-28.93)) ;
#149338=CARTESIAN_POINT('Origin',(1.5,1.9,-28.93)) ;
#149339=CARTESIAN_POINT('Origin',(1.5,2.6,-29.7714213562373)) ;
#149340=CARTESIAN_POINT('Origin',(1.5,2.6,-29.7714213562373)) ;
#149341=CARTESIAN_POINT('Origin',(1.5,1.9,-28.93)) ;
#149342=CARTESIAN_POINT('Origin',(1.5,1.9,-28.93)) ;
#149343=CARTESIAN_POINT('Origin',(1.5,2.6,-29.88)) ;
#149344=CARTESIAN_POINT('Origin',(1.5,2.6,-29.88)) ;
#149345=CARTESIAN_POINT('Origin',(1.5,1.9,-29.88)) ;
#149346=CARTESIAN_POINT('Origin',(1.5,1.9,-29.88)) ;
#149347=CARTESIAN_POINT('Origin',(1.5,2.4,-29.88)) ;
#149348=CARTESIAN_POINT('Origin',(1.5,2.4,-30.08)) ;
#149349=CARTESIAN_POINT('Origin',(1.5,2.1,-29.88)) ;
#149350=CARTESIAN_POINT('Origin',(1.5,2.1,-30.08)) ;
#149351=CARTESIAN_POINT('Origin',(1.5,2.1,-30.08)) ;
#149352=CARTESIAN_POINT('Origin',(-0.899999999999999,-2.,-33.69)) ;
#149353=CARTESIAN_POINT('Origin',(-0.899999999999999,0.4,-33.69)) ;
#149354=CARTESIAN_POINT('Origin',(-0.899999999999999,-1.9,-33.69)) ;
#149355=CARTESIAN_POINT('Origin',(0.600000000000001,0.4,-33.89)) ;
#149356=CARTESIAN_POINT('Origin',(0.500000000000001,0.4,-33.89)) ;
#149357=CARTESIAN_POINT('Origin',(-0.899999999999999,0.4,-33.89)) ;
#149358=CARTESIAN_POINT('Origin',(0.500000000000001,0.4,-33.89)) ;
#149359=CARTESIAN_POINT('',(0.600000000000001,0.4,-33.89)) ;
#149360=CARTESIAN_POINT('Origin',(0.500000000000001,0.4,-33.89)) ;
#149361=CARTESIAN_POINT('Origin',(0.500000000000001,0.4,-33.89)) ;
#149362=CARTESIAN_POINT('Origin',(-0.899999999999999,-1.9,-33.69)) ;
#149363=CARTESIAN_POINT('Origin',(-0.899999999999999,-1.9,-33.69)) ;
#149364=CARTESIAN_POINT('Origin',(-0.899999999999999,-1.9,-33.69)) ;
#149365=CARTESIAN_POINT('Origin',(-0.899999999999999,0.4,-33.89)) ;
#149366=CARTESIAN_POINT('Origin',(-0.899999999999999,0.6,-33.89)) ;
#149367=CARTESIAN_POINT('Origin',(0.500000000000001,0.4,-34.29)) ;
#149368=CARTESIAN_POINT('Origin',(0.500000000000001,0.4,-34.69)) ;
#149369=CARTESIAN_POINT('',(0.600000000000001,0.4,-34.59)) ;
#149370=CARTESIAN_POINT('Ctrl Pts',(0.595612997216083,0.370705721320409,
-34.6607057213204)) ;
#149371=CARTESIAN_POINT('Ctrl Pts',(0.596180587760894,0.372558268494363,
-34.6588554988322)) ;
#149372=CARTESIAN_POINT('Ctrl Pts',(0.596672461925687,0.374355839771987,
-34.6569141798663)) ;
#149373=CARTESIAN_POINT('Ctrl Pts',(0.599015141889206,0.383869350930039,
-34.6457649936563)) ;
#149374=CARTESIAN_POINT('Ctrl Pts',(0.599609996542524,0.390224332900438,
-34.6349726026542)) ;
#149375=CARTESIAN_POINT('Ctrl Pts',(0.600050586298726,0.39811743914156,
-34.6123310532047)) ;
#149376=CARTESIAN_POINT('Ctrl Pts',(0.600000000000001,0.4,-34.6012012506335)) ;
#149377=CARTESIAN_POINT('Ctrl Pts',(0.600000000000001,0.399999999999999,
-34.59)) ;
#149378=CARTESIAN_POINT('',(0.600000000000001,0.4,-34.29)) ;
#149379=CARTESIAN_POINT('Origin',(0.500000000000001,-4.56640444411538E-17,
-33.89)) ;
#149380=CARTESIAN_POINT('',(0.500000000000001,0.394987437106619,-33.99)) ;
#149381=CARTESIAN_POINT('Ctrl Pts',(0.500000000000001,0.394987437106619,
-33.99)) ;
#149382=CARTESIAN_POINT('Ctrl Pts',(0.505940567948938,0.395584486649899,
-33.99)) ;
#149383=CARTESIAN_POINT('Ctrl Pts',(0.511931971019108,0.396132036079016,
-33.989466300328)) ;
#149384=CARTESIAN_POINT('Ctrl Pts',(0.517829015308506,0.396618246075351,
-33.9883977957737)) ;
#149385=CARTESIAN_POINT('Ctrl Pts',(0.522982218721175,0.397043126556051,
-33.9874640701571)) ;
#149386=CARTESIAN_POINT('Ctrl Pts',(0.52806264897023,0.397421319341387,
-33.9861228267971)) ;
#149387=CARTESIAN_POINT('Ctrl Pts',(0.532978106724009,0.397751505046071,
-33.9844057438766)) ;
#149388=CARTESIAN_POINT('Ctrl Pts',(0.538583536338943,0.398128038182998,
-33.9824476378496)) ;
#149389=CARTESIAN_POINT('Ctrl Pts',(0.544059405914837,0.398447721828293,
-33.9799700083111)) ;
#149390=CARTESIAN_POINT('Ctrl Pts',(0.549268572255721,0.39871233110898,
-33.9770207319429)) ;
#149391=CARTESIAN_POINT('Ctrl Pts',(0.553856850427124,0.398945401221754,
-33.9744229841469)) ;
#149392=CARTESIAN_POINT('Ctrl Pts',(0.55823782506931,0.399135987683842,
-33.97146038498)) ;
#149393=CARTESIAN_POINT('Ctrl Pts',(0.56233383608621,0.399290378266507,
-33.9681952228642)) ;
#149394=CARTESIAN_POINT('Ctrl Pts',(0.566990328957886,0.399465895042381,
-33.9644832689523)) ;
#149395=CARTESIAN_POINT('Ctrl Pts',(0.571349096493416,0.399597278936107,
-33.9603228064848)) ;
#149396=CARTESIAN_POINT('Ctrl Pts',(0.575296920056707,0.399694832180838,
-33.9558055759793)) ;
#149397=CARTESIAN_POINT('Ctrl Pts',(0.578744263667898,0.399780018245914,
-33.9518610112151)) ;
#149398=CARTESIAN_POINT('Ctrl Pts',(0.581878314560451,0.399839626289636,
-33.9476455218421)) ;
#149399=CARTESIAN_POINT('Ctrl Pts',(0.584648147334857,0.399882153365958,
-33.9432418177073)) ;
#149400=CARTESIAN_POINT('Ctrl Pts',(0.587839270208177,0.399931148788079,
-33.9381683125045)) ;
#149401=CARTESIAN_POINT('Ctrl Pts',(0.590595054415139,0.399958289583405,
-33.9327666362444)) ;
#149402=CARTESIAN_POINT('Ctrl Pts',(0.592838618943155,0.39997435700316,
-33.9271616850093)) ;
#149403=CARTESIAN_POINT('Ctrl Pts',(0.594777336851684,0.399988241245861,
-33.9223183122423)) ;
#149404=CARTESIAN_POINT('Ctrl Pts',(0.596334051506209,0.399993946552814,
-33.917324166227)) ;
#149405=CARTESIAN_POINT('Ctrl Pts',(0.597488309822315,0.39999684570125,
-33.9122717185684)) ;
#149406=CARTESIAN_POINT('Ctrl Pts',(0.598804024094335,0.400000150378306,
-33.9065125419608)) ;
#149407=CARTESIAN_POINT('Ctrl Pts',(0.599612685195353,0.399999963509465,
-33.9006028438911)) ;
#149408=CARTESIAN_POINT('Ctrl Pts',(0.599890230999679,0.399999993975383,
-33.894684202262)) ;
#149409=CARTESIAN_POINT('Ctrl Pts',(0.599963464549386,0.400000002014155,
-33.8931225027904)) ;
#149410=CARTESIAN_POINT('Ctrl Pts',(0.600000000000001,0.399999999999999,
-33.8915602215095)) ;
#149411=CARTESIAN_POINT('Ctrl Pts',(0.600000000000001,0.399999999999999,
-33.89)) ;
#149412=CARTESIAN_POINT('',(0.600000000000001,0.299999999999999,-33.89)) ;
#149413=CARTESIAN_POINT('Ctrl Pts',(0.500000000000001,0.394987437106619,
-33.99)) ;
#149414=CARTESIAN_POINT('Ctrl Pts',(0.500454935590171,0.395033159853782,
-33.99)) ;
#149415=CARTESIAN_POINT('Ctrl Pts',(0.500909898680634,0.395078570329076,
-33.9899968954911)) ;
#149416=CARTESIAN_POINT('Ctrl Pts',(0.502892456244958,0.395275075889069,
-33.9899698339419)) ;
#149417=CARTESIAN_POINT('Ctrl Pts',(0.50441874748225,0.395422812032187,
-33.989913985421)) ;
#149418=CARTESIAN_POINT('Ctrl Pts',(0.508462199543321,0.395804395682031,
-33.9896732810567)) ;
#149419=CARTESIAN_POINT('Ctrl Pts',(0.510974953343264,0.396031485023314,
-33.9894279391451)) ;
#149420=CARTESIAN_POINT('Ctrl Pts',(0.521160739721166,0.396903453186226,
-33.9880427944916)) ;
#149421=CARTESIAN_POINT('Ctrl Pts',(0.528708678528252,0.397444933153152,
-33.9861042177047)) ;
#149422=CARTESIAN_POINT('Ctrl Pts',(0.545943206357825,0.398105551684101,
-33.9794646394513)) ;
#149423=CARTESIAN_POINT('Ctrl Pts',(0.555229535466584,0.397987646678453,
-33.9740353588361)) ;
#149424=CARTESIAN_POINT('Ctrl Pts',(0.571394604995541,0.395490482808082,
-33.960775513364)) ;
#149425=CARTESIAN_POINT('Ctrl Pts',(0.578055313702682,0.393198948698442,
-33.953240745632)) ;
#149426=CARTESIAN_POINT('Ctrl Pts',(0.588559132202378,0.385442756729426,
-33.9373922339843)) ;
#149427=CARTESIAN_POINT('Ctrl Pts',(0.592167355639896,0.380240075127069,
-33.929548265607)) ;
#149428=CARTESIAN_POINT('Ctrl Pts',(0.597496615531045,0.365892753467188,
-33.9139255217955)) ;
#149429=CARTESIAN_POINT('Ctrl Pts',(0.598734255154177,0.356660564300953,
-33.9067727417271)) ;
#149430=CARTESIAN_POINT('Ctrl Pts',(0.60001275468168,0.335223914398804,
-33.8955823058657)) ;
#149431=CARTESIAN_POINT('Ctrl Pts',(0.599993900559809,0.322655037092181,
-33.8916615193656)) ;
#149432=CARTESIAN_POINT('Ctrl Pts',(0.600000296204999,0.30610691358248,
-33.8901396263471)) ;
#149433=CARTESIAN_POINT('Ctrl Pts',(0.600000000000001,0.303050992413506,
-33.89)) ;
#149434=CARTESIAN_POINT('Ctrl Pts',(0.600000000000001,0.299999999999999,
-33.89)) ;
#149435=CARTESIAN_POINT('',(0.600000000000001,-2.39800009914436E-17,-33.89)) ;
#149436=CARTESIAN_POINT('Origin',(0.500000000000001,-1.9,-33.89)) ;
#149437=CARTESIAN_POINT('Origin',(0.600000000000001,-1.9,-33.69)) ;
#149438=CARTESIAN_POINT('Origin',(0.500000000000001,-1.9,-33.69)) ;
#149439=CARTESIAN_POINT('Origin',(-0.899999999999999,-1.9,-32.915)) ;
#149440=CARTESIAN_POINT('Origin',(-0.899999999999999,-1.9,-33.015)) ;
#149441=CARTESIAN_POINT('Origin',(-0.899999999999999,0.6,-33.79)) ;
#149442=CARTESIAN_POINT('Origin',(-0.899999999999999,0.6,-34.69)) ;
#149443=CARTESIAN_POINT('Origin',(0.600000000000001,0.4,-34.69)) ;
#149444=CARTESIAN_POINT('Origin',(0.500000000000001,0.4,-34.69)) ;
#149445=CARTESIAN_POINT('Origin',(-0.899999999999999,0.4,-34.69)) ;
#149446=CARTESIAN_POINT('Origin',(0.500000000000001,0.4,-34.69)) ;
#149447=CARTESIAN_POINT('Origin',(0.500000000000001,-1.9,-33.69)) ;
#149448=CARTESIAN_POINT('Origin',(0.500000000000001,-2.1,-33.69)) ;
#149449=CARTESIAN_POINT('Origin',(-0.899999999999999,-1.9,-33.015)) ;
#149450=CARTESIAN_POINT('Origin',(-1.1,-1.9,-33.015)) ;
#149451=CARTESIAN_POINT('Origin',(-0.899999999999999,-2.1,-33.015)) ;
#149452=CARTESIAN_POINT('Origin',(-0.899999999999999,0.4,-34.69)) ;
#149453=CARTESIAN_POINT('Origin',(-0.899999999999999,0.4,-34.89)) ;
#149454=CARTESIAN_POINT('Origin',(0.500000000000001,-2.1,-34.29)) ;
#149455=CARTESIAN_POINT('Origin',(0.500000000000001,-2.1,-33.015)) ;
#149456=CARTESIAN_POINT('Origin',(0.600000000000001,-2.1,-33.015)) ;
#149457=CARTESIAN_POINT('Origin',(0.500000000000001,-2.1,-33.015)) ;
#149458=CARTESIAN_POINT('Origin',(-1.1,-4.42727195005762E-17,-33.015)) ;
#149459=CARTESIAN_POINT('',(-1.1,1.15,-32.915)) ;
#149460=CARTESIAN_POINT('',(-1.1,1.25,-32.915)) ;
#149461=CARTESIAN_POINT('Origin',(-1.1,1.15,-33.015)) ;
#149462=CARTESIAN_POINT('Origin',(-0.899999999999999,0.5,-34.89)) ;
#149463=CARTESIAN_POINT('Origin',(-0.899999999999999,-1.9,-34.89)) ;
#149464=CARTESIAN_POINT('Origin',(0.600000000000001,-1.9,-34.89)) ;
#149465=CARTESIAN_POINT('Origin',(0.500000000000001,-1.9,-34.89)) ;
#149466=CARTESIAN_POINT('Origin',(-0.899999999999999,-1.9,-34.89)) ;
#149467=CARTESIAN_POINT('Origin',(0.500000000000001,-1.9,-34.89)) ;
#149468=CARTESIAN_POINT('Origin',(0.500000000000001,-2.1,-34.89)) ;
#149469=CARTESIAN_POINT('Origin',(0.500000000000001,-2.1,-33.015)) ;
#149470=CARTESIAN_POINT('Origin',(0.500000000000001,-2.1,-33.015)) ;
#149471=CARTESIAN_POINT('Origin',(-1.1,-2.9,-32.815)) ;
#149472=CARTESIAN_POINT('Origin',(-1.1,-2.9,-32.815)) ;
#149473=CARTESIAN_POINT('Origin',(-1.1,-2.9,-32.815)) ;
#149474=CARTESIAN_POINT('Origin',(-1.1,1.25,-32.815)) ;
#149475=CARTESIAN_POINT('Origin',(-1.1,1.15,-32.815)) ;
#149476=CARTESIAN_POINT('Origin',(-1.1,1.15,-33.015)) ;
#149477=CARTESIAN_POINT('',(-1.1,1.25,-33.015)) ;
#149478=CARTESIAN_POINT('Origin',(-1.1,1.15,-33.015)) ;
#149479=CARTESIAN_POINT('Origin',(-1.1,1.15,-33.015)) ;
#149480=CARTESIAN_POINT('Origin',(-0.899999999999999,-1.9,-34.89)) ;
#149481=CARTESIAN_POINT('Origin',(-0.899999999999999,-1.9,-34.89)) ;
#149482=CARTESIAN_POINT('Origin',(0.500000000000001,-2.1,-34.29)) ;
#149483=CARTESIAN_POINT('Origin',(0.500000000000001,-2.1,-35.565)) ;
#149484=CARTESIAN_POINT('Origin',(0.500000000000001,1.36481920536411E-16,
-33.015)) ;
#149485=CARTESIAN_POINT('Origin',(0.500000000000001,-2.9,-33.015)) ;
#149486=CARTESIAN_POINT('Origin',(-0.999999999999999,-2.9,-32.815)) ;
#149487=CARTESIAN_POINT('Origin',(0.500000000000001,-2.9,-32.815)) ;
#149488=CARTESIAN_POINT('Origin',(-1.1,1.15,-33.015)) ;
#149489=CARTESIAN_POINT('Origin',(-1.1,1.35,-33.015)) ;
#149490=CARTESIAN_POINT('Origin',(-1.1,1.15,-34.29)) ;
#149491=CARTESIAN_POINT('',(-1.1,1.25,-35.565)) ;
#149492=CARTESIAN_POINT('',(-1.1,1.25,-35.665)) ;
#149493=CARTESIAN_POINT('Origin',(-1.1,1.15,-35.565)) ;
#149494=CARTESIAN_POINT('Origin',(-0.899999999999999,-1.9,-34.79)) ;
#149495=CARTESIAN_POINT('Origin',(-0.899999999999999,-1.9,-35.565)) ;
#149496=CARTESIAN_POINT('Origin',(-0.999999999999999,-2.1,-35.565)) ;
#149497=CARTESIAN_POINT('Origin',(0.500000000000001,-2.1,-35.565)) ;
#149498=CARTESIAN_POINT('Origin',(-0.899999999999999,-2.1,-35.565)) ;
#149499=CARTESIAN_POINT('Origin',(0.500000000000001,-2.1,-35.565)) ;
#149500=CARTESIAN_POINT('Origin',(0.500000000000001,-2.1,-35.565)) ;
#149501=CARTESIAN_POINT('Origin',(0.500000000000001,-2.9,-33.015)) ;
#149502=CARTESIAN_POINT('Origin',(0.700000000000002,-2.9,-33.015)) ;
#149503=CARTESIAN_POINT('Origin',(-1.1,1.35,-35.665)) ;
#149504=CARTESIAN_POINT('Origin',(-1.1,1.35,-35.565)) ;
#149505=CARTESIAN_POINT('Origin',(-1.1,1.15,-35.565)) ;
#149506=CARTESIAN_POINT('',(-1.1,1.15,-35.665)) ;
#149507=CARTESIAN_POINT('Origin',(-1.1,1.15,-35.565)) ;
#149508=CARTESIAN_POINT('Origin',(-1.1,1.15,-35.565)) ;
#149509=CARTESIAN_POINT('Origin',(-0.899999999999999,-1.9,-35.565)) ;
#149510=CARTESIAN_POINT('Origin',(-1.1,-1.9,-35.565)) ;
#149511=CARTESIAN_POINT('Origin',(0.500000000000001,-5.867447051098E-17,
-35.565)) ;
#149512=CARTESIAN_POINT('Origin',(0.500000000000001,-2.9,-35.565)) ;
#149513=CARTESIAN_POINT('Origin',(0.700000000000002,-2.9,-34.29)) ;
#149514=CARTESIAN_POINT('Origin',(0.700000000000002,-2.9,-35.565)) ;
#149515=CARTESIAN_POINT('Origin',(-1.1,1.15,-35.565)) ;
#149516=CARTESIAN_POINT('Origin',(-1.1,1.15,-35.765)) ;
#149517=CARTESIAN_POINT('Origin',(-1.1,-2.39429110547967E-16,-35.565)) ;
#149518=CARTESIAN_POINT('',(-1.1,1.25,-35.665)) ;
#149519=CARTESIAN_POINT('Origin',(0.500000000000001,-2.9,-35.565)) ;
#149520=CARTESIAN_POINT('Origin',(0.500000000000001,-2.9,-35.765)) ;
#149521=CARTESIAN_POINT('Origin',(-1.1,1.25,-35.765)) ;
#149522=CARTESIAN_POINT('Origin',(-1.1,-2.9,-35.765)) ;
#149523=CARTESIAN_POINT('Origin',(-1.1,-2.9,-35.765)) ;
#149524=CARTESIAN_POINT('Origin',(-1.1,-2.9,-35.765)) ;
#149525=CARTESIAN_POINT('Origin',(-1.1,-2.9,-35.765)) ;
#149526=CARTESIAN_POINT('Origin',(1.5,1.9,-33.69)) ;
#149527=CARTESIAN_POINT('Origin',(1.5,1.9,-35.84)) ;
#149528=CARTESIAN_POINT('Origin',(1.5,1.9,-34.89)) ;
#149529=CARTESIAN_POINT('Origin',(1.5,2.1,-34.89)) ;
#149530=CARTESIAN_POINT('Origin',(1.5,2.1,-34.69)) ;
#149531=CARTESIAN_POINT('Origin',(1.5,1.9,-35.84)) ;
#149532=CARTESIAN_POINT('Origin',(1.5,1.9,-35.84)) ;
#149533=CARTESIAN_POINT('Origin',(1.5,2.1,-34.69)) ;
#149534=CARTESIAN_POINT('Origin',(1.5,2.4,-34.69)) ;
#149535=CARTESIAN_POINT('Origin',(1.5,2.1,-35.84)) ;
#149536=CARTESIAN_POINT('Origin',(1.5,-2.15,-35.84)) ;
#149537=CARTESIAN_POINT('Origin',(1.5,2.4,-34.89)) ;
#149538=CARTESIAN_POINT('Origin',(1.5,2.6,-34.89)) ;
#149539=CARTESIAN_POINT('Origin',(1.5,-2.15,-35.84)) ;
#149540=CARTESIAN_POINT('Origin',(1.5,-2.15,-35.84)) ;
#149541=CARTESIAN_POINT('Origin',(1.5,2.6,-33.69)) ;
#149542=CARTESIAN_POINT('Origin',(1.5,2.6,-34.9985786437627)) ;
#149543=CARTESIAN_POINT('Origin',(1.5,-2.15,-33.69)) ;
#149544=CARTESIAN_POINT('Origin',(1.5,-2.15,-35.1931195934094)) ;
#149545=CARTESIAN_POINT('Origin',(1.5,2.6,-34.9985786437627)) ;
#149546=CARTESIAN_POINT('Origin',(1.5,2.6,-34.9985786437627)) ;
#149547=CARTESIAN_POINT('Origin',(1.5,-2.15,-35.1931195934094)) ;
#149548=CARTESIAN_POINT('Origin',(1.5,-2.15,-35.1931195934094)) ;
#149549=CARTESIAN_POINT('Origin',(1.5,1.69571067811865,-34.0942893218813)) ;
#149550=CARTESIAN_POINT('Origin',(1.5,3.15,-35.5485786437627)) ;
#149551=CARTESIAN_POINT('Origin',(1.5,-3.65625,-34.29)) ;
#149552=CARTESIAN_POINT('Origin',(1.5,-2.15,-33.3868804065906)) ;
#149553=CARTESIAN_POINT('Origin',(1.5,3.15,-35.5485786437627)) ;
#149554=CARTESIAN_POINT('Origin',(1.5,3.15,-35.5485786437627)) ;
#149555=CARTESIAN_POINT('Origin',(1.5,-2.15,-33.3868804065906)) ;
#149556=CARTESIAN_POINT('Origin',(1.5,-2.15,-33.3868804065906)) ;
#149557=CARTESIAN_POINT('Origin',(1.5,3.15,-33.69)) ;
#149558=CARTESIAN_POINT('Origin',(1.5,-2.15,-33.69)) ;
#149559=CARTESIAN_POINT('Origin',(1.5,-2.15,-32.74)) ;
#149560=CARTESIAN_POINT('Origin',(1.5,-2.15,-32.74)) ;
#149561=CARTESIAN_POINT('Origin',(1.5,-2.15,-32.74)) ;
#149562=CARTESIAN_POINT('Origin',(1.5,2.29571067811866,-33.8857106781187)) ;
#149563=CARTESIAN_POINT('Origin',(1.5,2.6,-33.5814213562373)) ;
#149564=CARTESIAN_POINT('Origin',(1.5,2.1,-32.74)) ;
#149565=CARTESIAN_POINT('Origin',(1.5,1.9,-32.74)) ;
#149566=CARTESIAN_POINT('Origin',(1.5,2.6,-33.5814213562373)) ;
#149567=CARTESIAN_POINT('Origin',(1.5,2.6,-33.5814213562373)) ;
#149568=CARTESIAN_POINT('Origin',(1.5,1.9,-32.74)) ;
#149569=CARTESIAN_POINT('Origin',(1.5,1.9,-32.74)) ;
#149570=CARTESIAN_POINT('Origin',(1.5,2.6,-33.69)) ;
#149571=CARTESIAN_POINT('Origin',(1.5,2.6,-33.69)) ;
#149572=CARTESIAN_POINT('Origin',(1.5,1.9,-33.69)) ;
#149573=CARTESIAN_POINT('Origin',(1.5,1.9,-33.69)) ;
#149574=CARTESIAN_POINT('Origin',(1.5,2.4,-33.69)) ;
#149575=CARTESIAN_POINT('Origin',(1.5,2.4,-33.89)) ;
#149576=CARTESIAN_POINT('Origin',(1.5,2.1,-33.69)) ;
#149577=CARTESIAN_POINT('Origin',(1.5,2.1,-33.89)) ;
#149578=CARTESIAN_POINT('Origin',(1.5,2.1,-33.89)) ;
#149579=CARTESIAN_POINT('Origin',(-0.4,-0.600000000000001,-3.41)) ;
#149580=CARTESIAN_POINT('',(-0.4,-0.600000000000001,-3.51)) ;
#149581=CARTESIAN_POINT('',(-0.4,-0.600000000000001,-4.11)) ;
#149582=CARTESIAN_POINT('',(-0.4,-0.600000000000001,-3.41)) ;
#149583=CARTESIAN_POINT('',(-0.4,-6.05857864376269,-4.11)) ;
#149584=CARTESIAN_POINT('',(-0.4,-0.600000000000001,-4.11)) ;
#149585=CARTESIAN_POINT('',(-0.4,-6.05857864376269,-3.51)) ;
#149586=CARTESIAN_POINT('',(-0.4,-6.05857864376269,-3.41)) ;
#149587=CARTESIAN_POINT('',(-0.4,-0.600000000000001,-3.51)) ;
#149588=CARTESIAN_POINT('Origin',(-0.4,-6.1,-3.41)) ;
#149589=CARTESIAN_POINT('',(-0.129289321881346,-6.37071067811866,-3.86857864376269)) ;
#149590=CARTESIAN_POINT('',(-0.129289321881346,-6.37071067811866,-3.75142135623731)) ;
#149591=CARTESIAN_POINT('',(-0.129289321881346,-6.37071067811866,-3.41)) ;
#149592=CARTESIAN_POINT('',(-0.370710678118655,-6.12928932188134,-3.51)) ;
#149593=CARTESIAN_POINT('',(-0.423570226039552,-6.07642977396045,-3.4571404520791)) ;
#149594=CARTESIAN_POINT('',(-0.370710678118655,-6.12928932188134,-4.11)) ;
#149595=CARTESIAN_POINT('',(-0.370710678118655,-6.12928932188134,-3.41)) ;
#149596=CARTESIAN_POINT('',(-0.156903559372885,-6.34309644062712,-3.89619288125423)) ;
#149597=CARTESIAN_POINT('Origin',(-0.1,-6.4,-3.41)) ;
#149598=CARTESIAN_POINT('',(0.0585786437626908,-6.4,-3.86857864376269)) ;
#149599=CARTESIAN_POINT('',(0.0585786437626908,-6.4,-3.75142135623731)) ;
#149600=CARTESIAN_POINT('',(0.0585786437626908,-6.4,-3.41)) ;
#149601=CARTESIAN_POINT('',(-0.0585786437626908,-6.4,-3.75142135623731)) ;
#149602=CARTESIAN_POINT('',(-0.1,-6.4,-3.75142135623731)) ;
#149603=CARTESIAN_POINT('',(-0.0585786437626908,-6.4,-3.86857864376269)) ;
#149604=CARTESIAN_POINT('',(-0.0585786437626908,-6.4,-3.41)) ;
#149605=CARTESIAN_POINT('',(-0.1,-6.4,-3.86857864376269)) ;
#149606=CARTESIAN_POINT('Origin',(0.1,-6.4,-3.41)) ;
#149607=CARTESIAN_POINT('',(0.370710678118655,-6.12928932188134,-4.11)) ;
#149608=CARTESIAN_POINT('',(0.370710678118655,-6.12928932188134,-3.51)) ;
#149609=CARTESIAN_POINT('',(0.370710678118655,-6.12928932188134,-3.41)) ;
#149610=CARTESIAN_POINT('',(0.129289321881346,-6.37071067811866,-3.75142135623731)) ;
#149611=CARTESIAN_POINT('',(0.223570226039552,-6.27642977396045,-3.6571404520791)) ;
#149612=CARTESIAN_POINT('',(0.129289321881346,-6.37071067811866,-3.86857864376269)) ;
#149613=CARTESIAN_POINT('',(0.129289321881346,-6.37071067811866,-3.41)) ;
#149614=CARTESIAN_POINT('',(-0.0430964406271149,-6.54309644062712,-3.69619288125423)) ;
#149615=CARTESIAN_POINT('Origin',(0.4,-6.1,-3.41)) ;
#149616=CARTESIAN_POINT('',(0.4,-6.05857864376269,-3.51)) ;
#149617=CARTESIAN_POINT('',(0.4,-6.05857864376269,-4.11)) ;
#149618=CARTESIAN_POINT('',(0.4,-6.05857864376269,-3.41)) ;
#149619=CARTESIAN_POINT('',(0.4,-0.6,-4.11)) ;
#149620=CARTESIAN_POINT('',(0.4,-6.1,-4.11)) ;
#149621=CARTESIAN_POINT('',(0.4,-0.6,-3.51)) ;
#149622=CARTESIAN_POINT('',(0.4,-0.6,-3.41)) ;
#149623=CARTESIAN_POINT('',(0.4,-6.05857864376269,-3.51)) ;
#149624=CARTESIAN_POINT('Origin',(0.6,-0.600000000000001,-3.41)) ;
#149625=CARTESIAN_POINT('',(0.3,-6.05857864376269,-3.41)) ;
#149626=CARTESIAN_POINT('',(0.3,-0.6,-3.41)) ;
#149627=CARTESIAN_POINT('',(0.3,-0.6,-3.41)) ;
#149628=CARTESIAN_POINT('Origin',(0.6,-0.6,-3.41)) ;
#149629=CARTESIAN_POINT('',(-0.3,-0.600000000000001,-3.41)) ;
#149630=CARTESIAN_POINT('Origin',(0.6,-0.600000000000001,-3.41)) ;
#149631=CARTESIAN_POINT('',(-0.299999999999999,-6.05857864376269,-3.41)) ;
#149632=CARTESIAN_POINT('',(-0.3,-0.600000000000001,-3.41)) ;
#149633=CARTESIAN_POINT('',(0.4,-6.05857864376269,-3.41)) ;
#149634=CARTESIAN_POINT('Origin',(0.6,-0.600000000000001,-4.21)) ;
#149635=CARTESIAN_POINT('',(-0.300000000000001,-6.05857864376269,-4.21)) ;
#149636=CARTESIAN_POINT('',(-0.3,-0.600000000000001,-4.21)) ;
#149637=CARTESIAN_POINT('',(-0.3,-0.600000000000001,-4.21)) ;
#149638=CARTESIAN_POINT('Origin',(0.6,-0.600000000000001,-4.21)) ;
#149639=CARTESIAN_POINT('',(0.3,-0.6,-4.21)) ;
#149640=CARTESIAN_POINT('Origin',(0.6,-0.6,-4.21)) ;
#149641=CARTESIAN_POINT('',(0.3,-6.05857864376269,-4.21)) ;
#149642=CARTESIAN_POINT('',(0.3,-0.600000000000001,-4.21)) ;
#149643=CARTESIAN_POINT('',(0.6,-6.05857864376269,-4.21)) ;
#149644=CARTESIAN_POINT('Origin',(0.6,-0.600000000000001,-3.41)) ;
#149645=CARTESIAN_POINT('Origin',(0.6,-0.600000000000001,-4.11)) ;
#149646=CARTESIAN_POINT('Origin',(0.6,-0.600000000000001,-3.51)) ;
#149647=CARTESIAN_POINT('Origin',(0.6,-0.6,-3.41)) ;
#149648=CARTESIAN_POINT('Origin',(0.6,-0.6,-4.11)) ;
#149649=CARTESIAN_POINT('Origin',(0.6,-0.6,-3.51)) ;
#149650=CARTESIAN_POINT('Origin',(7.,0.1,-3.41)) ;
#149651=CARTESIAN_POINT('',(6.72928932188135,0.370710678118655,-4.11)) ;
#149652=CARTESIAN_POINT('',(6.72928932188135,0.370710678118655,-3.51)) ;
#149653=CARTESIAN_POINT('',(6.72928932188135,0.370710678118655,-3.41)) ;
#149654=CARTESIAN_POINT('',(6.97071067811866,0.129289321881346,-3.75142135623731)) ;
#149655=CARTESIAN_POINT('',(6.87642977396045,0.223570226039552,-3.6571404520791)) ;
#149656=CARTESIAN_POINT('',(6.97071067811866,0.129289321881346,-3.86857864376269)) ;
#149657=CARTESIAN_POINT('',(6.97071067811866,0.129289321881346,-3.41)) ;
#149658=CARTESIAN_POINT('',(7.14309644062712,-0.0430964406271146,-3.69619288125423)) ;
#149659=CARTESIAN_POINT('Origin',(6.7,0.400000000000001,-3.41)) ;
#149660=CARTESIAN_POINT('',(6.65857864376269,0.400000000000001,-3.51)) ;
#149661=CARTESIAN_POINT('',(6.65857864376269,0.400000000000001,-4.11)) ;
#149662=CARTESIAN_POINT('',(6.65857864376269,0.400000000000001,-3.41)) ;
#149663=CARTESIAN_POINT('',(6.7,0.400000000000001,-4.11)) ;
#149664=CARTESIAN_POINT('',(6.65857864376269,0.400000000000001,-3.51)) ;
#149665=CARTESIAN_POINT('Origin',(0.6,-0.4,-3.41)) ;
#149666=CARTESIAN_POINT('',(6.65857864376269,-0.400000000000001,-4.11)) ;
#149667=CARTESIAN_POINT('',(0.6,-0.4,-4.11)) ;
#149668=CARTESIAN_POINT('',(6.65857864376269,-0.400000000000001,-3.51)) ;
#149669=CARTESIAN_POINT('',(6.65857864376269,-0.400000000000001,-3.41)) ;
#149670=CARTESIAN_POINT('',(2.4,-0.4,-3.51)) ;
#149671=CARTESIAN_POINT('Origin',(6.7,-0.400000000000001,-3.41)) ;
#149672=CARTESIAN_POINT('',(6.97071067811866,-0.129289321881346,-3.86857864376269)) ;
#149673=CARTESIAN_POINT('',(6.97071067811866,-0.129289321881346,-3.75142135623731)) ;
#149674=CARTESIAN_POINT('',(6.97071067811866,-0.129289321881346,-3.41)) ;
#149675=CARTESIAN_POINT('',(6.72928932188135,-0.370710678118655,-3.51)) ;
#149676=CARTESIAN_POINT('',(6.67642977396045,-0.423570226039552,-3.4571404520791)) ;
#149677=CARTESIAN_POINT('',(6.72928932188135,-0.370710678118655,-4.11)) ;
#149678=CARTESIAN_POINT('',(6.72928932188135,-0.370710678118655,-3.41)) ;
#149679=CARTESIAN_POINT('',(6.94309644062712,-0.156903559372885,-3.89619288125423)) ;
#149680=CARTESIAN_POINT('Origin',(7.,-0.1,-3.41)) ;
#149681=CARTESIAN_POINT('',(7.,-0.0585786437626909,-3.75142135623731)) ;
#149682=CARTESIAN_POINT('',(7.,-0.0585786437626909,-3.86857864376269)) ;
#149683=CARTESIAN_POINT('',(7.,-0.0585786437626909,-3.41)) ;
#149684=CARTESIAN_POINT('',(7.,0.0585786437626909,-3.86857864376269)) ;
#149685=CARTESIAN_POINT('',(7.,-0.1,-3.86857864376269)) ;
#149686=CARTESIAN_POINT('',(7.,0.0585786437626909,-3.75142135623731)) ;
#149687=CARTESIAN_POINT('',(7.,0.0585786437626909,-3.41)) ;
#149688=CARTESIAN_POINT('',(7.,-0.1,-3.75142135623731)) ;
#149689=CARTESIAN_POINT('Origin',(0.6,-0.600000000000001,-3.41)) ;
#149690=CARTESIAN_POINT('',(6.65857864376269,-0.300000000000001,-3.41)) ;
#149691=CARTESIAN_POINT('',(6.65857864376269,0.3,-3.41)) ;
#149692=CARTESIAN_POINT('',(6.65857864376269,-0.399999999999999,-3.41)) ;
#149693=CARTESIAN_POINT('',(2.4,0.3,-3.41)) ;
#149694=CARTESIAN_POINT('',(6.65857864376269,-0.300000000000001,-3.41)) ;
#149695=CARTESIAN_POINT('Origin',(0.6,-0.600000000000001,-4.21)) ;
#149696=CARTESIAN_POINT('',(6.65857864376269,0.300000000000001,-4.21)) ;
#149697=CARTESIAN_POINT('',(0.6,0.299999999999999,-4.21)) ;
#149698=CARTESIAN_POINT('',(6.65857864376269,-0.300000000000001,-4.21)) ;
#149699=CARTESIAN_POINT('',(6.65857864376269,-0.6,-4.21)) ;
#149700=CARTESIAN_POINT('',(0.6,-0.3,-4.21)) ;
#149701=CARTESIAN_POINT('Origin',(-0.4,-0.600000000000001,-7.22)) ;
#149702=CARTESIAN_POINT('',(-0.4,-0.600000000000001,-7.32)) ;
#149703=CARTESIAN_POINT('',(-0.4,-0.600000000000001,-7.92)) ;
#149704=CARTESIAN_POINT('',(-0.4,-0.600000000000001,-7.22)) ;
#149705=CARTESIAN_POINT('',(-0.4,-6.05857864376269,-7.92)) ;
#149706=CARTESIAN_POINT('',(-0.4,-0.600000000000001,-7.92)) ;
#149707=CARTESIAN_POINT('',(-0.4,-6.05857864376269,-7.32)) ;
#149708=CARTESIAN_POINT('',(-0.4,-6.05857864376269,-7.22)) ;
#149709=CARTESIAN_POINT('',(-0.4,-0.600000000000001,-7.32)) ;
#149710=CARTESIAN_POINT('Origin',(-0.4,-6.1,-7.22)) ;
#149711=CARTESIAN_POINT('',(-0.129289321881345,-6.37071067811866,-7.67857864376269)) ;
#149712=CARTESIAN_POINT('',(-0.129289321881346,-6.37071067811866,-7.56142135623731)) ;
#149713=CARTESIAN_POINT('',(-0.129289321881346,-6.37071067811866,-7.22)) ;
#149714=CARTESIAN_POINT('',(-0.370710678118655,-6.12928932188134,-7.32)) ;
#149715=CARTESIAN_POINT('',(-0.423570226039552,-6.07642977396045,-7.2671404520791)) ;
#149716=CARTESIAN_POINT('',(-0.370710678118655,-6.12928932188134,-7.92)) ;
#149717=CARTESIAN_POINT('',(-0.370710678118655,-6.12928932188134,-7.22)) ;
#149718=CARTESIAN_POINT('',(-0.156903559372885,-6.34309644062712,-7.70619288125423)) ;
#149719=CARTESIAN_POINT('Origin',(-0.1,-6.4,-7.22)) ;
#149720=CARTESIAN_POINT('',(0.0585786437626908,-6.4,-7.67857864376269)) ;
#149721=CARTESIAN_POINT('',(0.0585786437626908,-6.4,-7.56142135623731)) ;
#149722=CARTESIAN_POINT('',(0.0585786437626908,-6.4,-7.22)) ;
#149723=CARTESIAN_POINT('',(-0.0585786437626908,-6.4,-7.56142135623731)) ;
#149724=CARTESIAN_POINT('',(-0.1,-6.4,-7.56142135623731)) ;
#149725=CARTESIAN_POINT('',(-0.0585786437626908,-6.4,-7.67857864376269)) ;
#149726=CARTESIAN_POINT('',(-0.0585786437626908,-6.4,-7.22)) ;
#149727=CARTESIAN_POINT('',(-0.1,-6.4,-7.67857864376269)) ;
#149728=CARTESIAN_POINT('Origin',(0.1,-6.4,-7.22)) ;
#149729=CARTESIAN_POINT('',(0.370710678118655,-6.12928932188134,-7.92)) ;
#149730=CARTESIAN_POINT('',(0.370710678118655,-6.12928932188134,-7.32)) ;
#149731=CARTESIAN_POINT('',(0.370710678118655,-6.12928932188134,-7.22)) ;
#149732=CARTESIAN_POINT('',(0.129289321881346,-6.37071067811866,-7.56142135623731)) ;
#149733=CARTESIAN_POINT('',(0.223570226039553,-6.27642977396045,-7.4671404520791)) ;
#149734=CARTESIAN_POINT('',(0.129289321881346,-6.37071067811866,-7.67857864376269)) ;
#149735=CARTESIAN_POINT('',(0.129289321881346,-6.37071067811866,-7.22)) ;
#149736=CARTESIAN_POINT('',(-0.0430964406271151,-6.54309644062712,-7.50619288125423)) ;
#149737=CARTESIAN_POINT('Origin',(0.4,-6.1,-7.22)) ;
#149738=CARTESIAN_POINT('',(0.4,-6.05857864376269,-7.32)) ;
#149739=CARTESIAN_POINT('',(0.4,-6.05857864376269,-7.92)) ;
#149740=CARTESIAN_POINT('',(0.4,-6.05857864376269,-7.22)) ;
#149741=CARTESIAN_POINT('',(0.4,-0.6,-7.92)) ;
#149742=CARTESIAN_POINT('',(0.4,-6.1,-7.92)) ;
#149743=CARTESIAN_POINT('',(0.4,-0.6,-7.32)) ;
#149744=CARTESIAN_POINT('',(0.4,-0.6,-7.22)) ;
#149745=CARTESIAN_POINT('',(0.4,-6.05857864376269,-7.32)) ;
#149746=CARTESIAN_POINT('Origin',(0.6,-0.600000000000001,-7.22)) ;
#149747=CARTESIAN_POINT('',(0.3,-6.05857864376269,-7.22)) ;
#149748=CARTESIAN_POINT('',(0.3,-0.6,-7.22)) ;
#149749=CARTESIAN_POINT('',(0.3,-0.6,-7.22)) ;
#149750=CARTESIAN_POINT('Origin',(0.6,-0.6,-7.22)) ;
#149751=CARTESIAN_POINT('',(-0.3,-0.600000000000001,-7.22)) ;
#149752=CARTESIAN_POINT('Origin',(0.6,-0.600000000000001,-7.22)) ;
#149753=CARTESIAN_POINT('',(-0.300000000000001,-6.05857864376269,-7.22)) ;
#149754=CARTESIAN_POINT('',(-0.3,-0.600000000000001,-7.22)) ;
#149755=CARTESIAN_POINT('',(0.4,-6.05857864376269,-7.22)) ;
#149756=CARTESIAN_POINT('Origin',(0.6,-0.600000000000001,-8.02)) ;
#149757=CARTESIAN_POINT('',(-0.299999999999999,-6.05857864376269,-8.02)) ;
#149758=CARTESIAN_POINT('',(-0.3,-0.600000000000001,-8.02)) ;
#149759=CARTESIAN_POINT('',(-0.3,-0.600000000000001,-8.02)) ;
#149760=CARTESIAN_POINT('Origin',(0.6,-0.600000000000001,-8.02)) ;
#149761=CARTESIAN_POINT('',(0.3,-0.6,-8.02)) ;
#149762=CARTESIAN_POINT('Origin',(0.6,-0.6,-8.02)) ;
#149763=CARTESIAN_POINT('',(0.3,-6.05857864376269,-8.02)) ;
#149764=CARTESIAN_POINT('',(0.3,-0.600000000000001,-8.02)) ;
#149765=CARTESIAN_POINT('',(0.6,-6.05857864376269,-8.02)) ;
#149766=CARTESIAN_POINT('Origin',(0.6,-0.600000000000001,-7.22)) ;
#149767=CARTESIAN_POINT('Origin',(0.6,-0.600000000000001,-7.92)) ;
#149768=CARTESIAN_POINT('Origin',(0.6,-0.600000000000001,-7.32)) ;
#149769=CARTESIAN_POINT('Origin',(0.6,-0.6,-7.22)) ;
#149770=CARTESIAN_POINT('Origin',(0.6,-0.6,-7.92)) ;
#149771=CARTESIAN_POINT('Origin',(0.6,-0.6,-7.32)) ;
#149772=CARTESIAN_POINT('Origin',(7.,0.1,-7.22)) ;
#149773=CARTESIAN_POINT('',(6.72928932188135,0.370710678118655,-7.92)) ;
#149774=CARTESIAN_POINT('',(6.72928932188135,0.370710678118655,-7.32)) ;
#149775=CARTESIAN_POINT('',(6.72928932188135,0.370710678118655,-7.22)) ;
#149776=CARTESIAN_POINT('',(6.97071067811866,0.129289321881346,-7.56142135623731)) ;
#149777=CARTESIAN_POINT('',(6.87642977396045,0.223570226039553,-7.4671404520791)) ;
#149778=CARTESIAN_POINT('',(6.97071067811866,0.129289321881346,-7.67857864376269)) ;
#149779=CARTESIAN_POINT('',(6.97071067811866,0.129289321881346,-7.22)) ;
#149780=CARTESIAN_POINT('',(7.14309644062712,-0.0430964406271152,-7.50619288125423)) ;
#149781=CARTESIAN_POINT('Origin',(6.7,0.400000000000001,-7.22)) ;
#149782=CARTESIAN_POINT('',(6.65857864376269,0.400000000000001,-7.32)) ;
#149783=CARTESIAN_POINT('',(6.65857864376269,0.400000000000001,-7.92)) ;
#149784=CARTESIAN_POINT('',(6.65857864376269,0.400000000000001,-7.22)) ;
#149785=CARTESIAN_POINT('',(6.7,0.400000000000001,-7.92)) ;
#149786=CARTESIAN_POINT('',(6.65857864376269,0.400000000000001,-7.32)) ;
#149787=CARTESIAN_POINT('Origin',(0.6,-0.4,-7.22)) ;
#149788=CARTESIAN_POINT('',(6.65857864376269,-0.400000000000001,-7.92)) ;
#149789=CARTESIAN_POINT('',(0.6,-0.4,-7.92)) ;
#149790=CARTESIAN_POINT('',(6.65857864376269,-0.400000000000001,-7.32)) ;
#149791=CARTESIAN_POINT('',(6.65857864376269,-0.400000000000001,-7.22)) ;
#149792=CARTESIAN_POINT('',(2.4,-0.4,-7.32)) ;
#149793=CARTESIAN_POINT('Origin',(6.7,-0.400000000000001,-7.22)) ;
#149794=CARTESIAN_POINT('',(6.97071067811866,-0.129289321881346,-7.67857864376269)) ;
#149795=CARTESIAN_POINT('',(6.97071067811866,-0.129289321881346,-7.56142135623731)) ;
#149796=CARTESIAN_POINT('',(6.97071067811866,-0.129289321881346,-7.22)) ;
#149797=CARTESIAN_POINT('',(6.72928932188135,-0.370710678118655,-7.32)) ;
#149798=CARTESIAN_POINT('',(6.67642977396045,-0.423570226039553,-7.2671404520791)) ;
#149799=CARTESIAN_POINT('',(6.72928932188135,-0.370710678118655,-7.92)) ;
#149800=CARTESIAN_POINT('',(6.72928932188135,-0.370710678118655,-7.22)) ;
#149801=CARTESIAN_POINT('',(6.94309644062712,-0.156903559372885,-7.70619288125423)) ;
#149802=CARTESIAN_POINT('Origin',(7.,-0.1,-7.22)) ;
#149803=CARTESIAN_POINT('',(7.,-0.0585786437626909,-7.56142135623731)) ;
#149804=CARTESIAN_POINT('',(7.,-0.0585786437626909,-7.67857864376269)) ;
#149805=CARTESIAN_POINT('',(7.,-0.0585786437626909,-7.22)) ;
#149806=CARTESIAN_POINT('',(7.,0.0585786437626909,-7.67857864376269)) ;
#149807=CARTESIAN_POINT('',(7.,-0.1,-7.67857864376269)) ;
#149808=CARTESIAN_POINT('',(7.,0.0585786437626909,-7.56142135623731)) ;
#149809=CARTESIAN_POINT('',(7.,0.0585786437626909,-7.22)) ;
#149810=CARTESIAN_POINT('',(7.,-0.1,-7.56142135623731)) ;
#149811=CARTESIAN_POINT('Origin',(0.6,-0.600000000000001,-7.22)) ;
#149812=CARTESIAN_POINT('',(6.65857864376269,-0.300000000000001,-7.22)) ;
#149813=CARTESIAN_POINT('',(6.65857864376269,0.300000000000002,-7.22)) ;
#149814=CARTESIAN_POINT('',(6.65857864376269,-0.399999999999999,-7.22)) ;
#149815=CARTESIAN_POINT('',(2.4,0.3,-7.22)) ;
#149816=CARTESIAN_POINT('',(6.65857864376269,-0.300000000000001,-7.22)) ;
#149817=CARTESIAN_POINT('Origin',(0.6,-0.600000000000001,-8.02)) ;
#149818=CARTESIAN_POINT('',(6.65857864376269,0.300000000000002,-8.02)) ;
#149819=CARTESIAN_POINT('',(0.6,0.299999999999999,-8.02)) ;
#149820=CARTESIAN_POINT('',(6.65857864376269,-0.300000000000001,-8.02)) ;
#149821=CARTESIAN_POINT('',(6.65857864376269,-0.6,-8.02)) ;
#149822=CARTESIAN_POINT('',(0.6,-0.3,-8.02)) ;
#149823=CARTESIAN_POINT('Origin',(-0.4,-0.600000000000001,-11.03)) ;
#149824=CARTESIAN_POINT('',(-0.4,-0.600000000000001,-11.13)) ;
#149825=CARTESIAN_POINT('',(-0.4,-0.600000000000001,-11.73)) ;
#149826=CARTESIAN_POINT('',(-0.4,-0.600000000000001,-11.03)) ;
#149827=CARTESIAN_POINT('',(-0.4,-6.05857864376269,-11.73)) ;
#149828=CARTESIAN_POINT('',(-0.4,-0.600000000000001,-11.73)) ;
#149829=CARTESIAN_POINT('',(-0.4,-6.05857864376269,-11.13)) ;
#149830=CARTESIAN_POINT('',(-0.4,-6.05857864376269,-11.03)) ;
#149831=CARTESIAN_POINT('',(-0.4,-0.600000000000001,-11.13)) ;
#149832=CARTESIAN_POINT('Origin',(-0.4,-6.1,-11.03)) ;
#149833=CARTESIAN_POINT('',(-0.129289321881346,-6.37071067811866,-11.4885786437627)) ;
#149834=CARTESIAN_POINT('',(-0.129289321881346,-6.37071067811866,-11.3714213562373)) ;
#149835=CARTESIAN_POINT('',(-0.129289321881346,-6.37071067811866,-11.03)) ;
#149836=CARTESIAN_POINT('',(-0.370710678118655,-6.12928932188134,-11.13)) ;
#149837=CARTESIAN_POINT('',(-0.423570226039552,-6.07642977396045,-11.0771404520791)) ;
#149838=CARTESIAN_POINT('',(-0.370710678118655,-6.12928932188134,-11.73)) ;
#149839=CARTESIAN_POINT('',(-0.370710678118655,-6.12928932188134,-11.03)) ;
#149840=CARTESIAN_POINT('',(-0.156903559372884,-6.34309644062712,-11.5161928812542)) ;
#149841=CARTESIAN_POINT('Origin',(-0.1,-6.4,-11.03)) ;
#149842=CARTESIAN_POINT('',(0.0585786437626908,-6.4,-11.4885786437627)) ;
#149843=CARTESIAN_POINT('',(0.0585786437626908,-6.4,-11.3714213562373)) ;
#149844=CARTESIAN_POINT('',(0.0585786437626908,-6.4,-11.03)) ;
#149845=CARTESIAN_POINT('',(-0.0585786437626908,-6.4,-11.3714213562373)) ;
#149846=CARTESIAN_POINT('',(-0.1,-6.4,-11.3714213562373)) ;
#149847=CARTESIAN_POINT('',(-0.0585786437626908,-6.4,-11.4885786437627)) ;
#149848=CARTESIAN_POINT('',(-0.0585786437626908,-6.4,-11.03)) ;
#149849=CARTESIAN_POINT('',(-0.1,-6.4,-11.4885786437627)) ;
#149850=CARTESIAN_POINT('Origin',(0.1,-6.4,-11.03)) ;
#149851=CARTESIAN_POINT('',(0.370710678118655,-6.12928932188134,-11.73)) ;
#149852=CARTESIAN_POINT('',(0.370710678118655,-6.12928932188134,-11.13)) ;
#149853=CARTESIAN_POINT('',(0.370710678118655,-6.12928932188134,-11.03)) ;
#149854=CARTESIAN_POINT('',(0.129289321881346,-6.37071067811866,-11.3714213562373)) ;
#149855=CARTESIAN_POINT('',(0.223570226039553,-6.27642977396045,-11.2771404520791)) ;
#149856=CARTESIAN_POINT('',(0.129289321881346,-6.37071067811866,-11.4885786437627)) ;
#149857=CARTESIAN_POINT('',(0.129289321881346,-6.37071067811866,-11.03)) ;
#149858=CARTESIAN_POINT('',(-0.0430964406271157,-6.54309644062712,-11.3161928812542)) ;
#149859=CARTESIAN_POINT('Origin',(0.4,-6.1,-11.03)) ;
#149860=CARTESIAN_POINT('',(0.4,-6.05857864376269,-11.13)) ;
#149861=CARTESIAN_POINT('',(0.4,-6.05857864376269,-11.73)) ;
#149862=CARTESIAN_POINT('',(0.4,-6.05857864376269,-11.03)) ;
#149863=CARTESIAN_POINT('',(0.4,-0.6,-11.73)) ;
#149864=CARTESIAN_POINT('',(0.4,-6.1,-11.73)) ;
#149865=CARTESIAN_POINT('',(0.4,-0.6,-11.13)) ;
#149866=CARTESIAN_POINT('',(0.4,-0.6,-11.03)) ;
#149867=CARTESIAN_POINT('',(0.4,-6.05857864376269,-11.13)) ;
#149868=CARTESIAN_POINT('Origin',(0.6,-0.600000000000001,-11.03)) ;
#149869=CARTESIAN_POINT('',(0.3,-6.05857864376269,-11.03)) ;
#149870=CARTESIAN_POINT('',(0.3,-0.6,-11.03)) ;
#149871=CARTESIAN_POINT('',(0.3,-0.6,-11.03)) ;
#149872=CARTESIAN_POINT('Origin',(0.6,-0.6,-11.03)) ;
#149873=CARTESIAN_POINT('',(-0.3,-0.600000000000001,-11.03)) ;
#149874=CARTESIAN_POINT('Origin',(0.6,-0.600000000000001,-11.03)) ;
#149875=CARTESIAN_POINT('',(-0.300000000000003,-6.05857864376269,-11.03)) ;
#149876=CARTESIAN_POINT('',(-0.3,-0.600000000000001,-11.03)) ;
#149877=CARTESIAN_POINT('',(0.4,-6.05857864376269,-11.03)) ;
#149878=CARTESIAN_POINT('Origin',(0.6,-0.600000000000001,-11.83)) ;
#149879=CARTESIAN_POINT('',(-0.299999999999999,-6.05857864376269,-11.83)) ;
#149880=CARTESIAN_POINT('',(-0.3,-0.600000000000001,-11.83)) ;
#149881=CARTESIAN_POINT('',(-0.3,-0.600000000000001,-11.83)) ;
#149882=CARTESIAN_POINT('Origin',(0.6,-0.600000000000001,-11.83)) ;
#149883=CARTESIAN_POINT('',(0.3,-0.6,-11.83)) ;
#149884=CARTESIAN_POINT('Origin',(0.6,-0.6,-11.83)) ;
#149885=CARTESIAN_POINT('',(0.3,-6.05857864376269,-11.83)) ;
#149886=CARTESIAN_POINT('',(0.3,-0.600000000000001,-11.83)) ;
#149887=CARTESIAN_POINT('',(0.6,-6.05857864376269,-11.83)) ;
#149888=CARTESIAN_POINT('Origin',(0.6,-0.600000000000001,-11.03)) ;
#149889=CARTESIAN_POINT('Origin',(0.6,-0.600000000000001,-11.73)) ;
#149890=CARTESIAN_POINT('Origin',(0.6,-0.600000000000001,-11.13)) ;
#149891=CARTESIAN_POINT('Origin',(0.6,-0.6,-11.03)) ;
#149892=CARTESIAN_POINT('Origin',(0.6,-0.6,-11.73)) ;
#149893=CARTESIAN_POINT('Origin',(0.6,-0.6,-11.13)) ;
#149894=CARTESIAN_POINT('Origin',(7.,0.1,-11.03)) ;
#149895=CARTESIAN_POINT('',(6.72928932188135,0.370710678118655,-11.73)) ;
#149896=CARTESIAN_POINT('',(6.72928932188135,0.370710678118655,-11.13)) ;
#149897=CARTESIAN_POINT('',(6.72928932188135,0.370710678118655,-11.03)) ;
#149898=CARTESIAN_POINT('',(6.97071067811866,0.129289321881346,-11.3714213562373)) ;
#149899=CARTESIAN_POINT('',(6.87642977396045,0.223570226039553,-11.2771404520791)) ;
#149900=CARTESIAN_POINT('',(6.97071067811866,0.129289321881346,-11.4885786437627)) ;
#149901=CARTESIAN_POINT('',(6.97071067811866,0.129289321881346,-11.03)) ;
#149902=CARTESIAN_POINT('',(7.14309644062712,-0.0430964406271147,-11.3161928812542)) ;
#149903=CARTESIAN_POINT('Origin',(6.7,0.400000000000001,-11.03)) ;
#149904=CARTESIAN_POINT('',(6.65857864376269,0.400000000000001,-11.13)) ;
#149905=CARTESIAN_POINT('',(6.65857864376269,0.400000000000001,-11.73)) ;
#149906=CARTESIAN_POINT('',(6.65857864376269,0.400000000000001,-11.03)) ;
#149907=CARTESIAN_POINT('',(6.7,0.400000000000001,-11.73)) ;
#149908=CARTESIAN_POINT('',(6.65857864376269,0.400000000000001,-11.13)) ;
#149909=CARTESIAN_POINT('Origin',(0.6,-0.4,-11.03)) ;
#149910=CARTESIAN_POINT('',(6.65857864376269,-0.400000000000001,-11.73)) ;
#149911=CARTESIAN_POINT('',(0.6,-0.4,-11.73)) ;
#149912=CARTESIAN_POINT('',(6.65857864376269,-0.400000000000001,-11.13)) ;
#149913=CARTESIAN_POINT('',(6.65857864376269,-0.400000000000001,-11.03)) ;
#149914=CARTESIAN_POINT('',(2.4,-0.4,-11.13)) ;
#149915=CARTESIAN_POINT('Origin',(6.7,-0.400000000000001,-11.03)) ;
#149916=CARTESIAN_POINT('',(6.97071067811866,-0.129289321881346,-11.4885786437627)) ;
#149917=CARTESIAN_POINT('',(6.97071067811866,-0.129289321881346,-11.3714213562373)) ;
#149918=CARTESIAN_POINT('',(6.97071067811866,-0.129289321881346,-11.03)) ;
#149919=CARTESIAN_POINT('',(6.72928932188135,-0.370710678118655,-11.13)) ;
#149920=CARTESIAN_POINT('',(6.67642977396045,-0.423570226039553,-11.0771404520791)) ;
#149921=CARTESIAN_POINT('',(6.72928932188135,-0.370710678118655,-11.73)) ;
#149922=CARTESIAN_POINT('',(6.72928932188135,-0.370710678118655,-11.03)) ;
#149923=CARTESIAN_POINT('',(6.94309644062712,-0.156903559372885,-11.5161928812542)) ;
#149924=CARTESIAN_POINT('Origin',(7.,-0.1,-11.03)) ;
#149925=CARTESIAN_POINT('',(7.,-0.0585786437626909,-11.3714213562373)) ;
#149926=CARTESIAN_POINT('',(7.,-0.0585786437626909,-11.4885786437627)) ;
#149927=CARTESIAN_POINT('',(7.,-0.0585786437626909,-11.03)) ;
#149928=CARTESIAN_POINT('',(7.,0.0585786437626909,-11.4885786437627)) ;
#149929=CARTESIAN_POINT('',(7.,-0.1,-11.4885786437627)) ;
#149930=CARTESIAN_POINT('',(7.,0.0585786437626909,-11.3714213562373)) ;
#149931=CARTESIAN_POINT('',(7.,0.0585786437626909,-11.03)) ;
#149932=CARTESIAN_POINT('',(7.,-0.1,-11.3714213562373)) ;
#149933=CARTESIAN_POINT('Origin',(0.6,-0.600000000000001,-11.03)) ;
#149934=CARTESIAN_POINT('',(6.65857864376269,-0.300000000000001,-11.03)) ;
#149935=CARTESIAN_POINT('',(6.65857864376269,0.300000000000002,-11.03)) ;
#149936=CARTESIAN_POINT('',(6.65857864376269,-0.399999999999999,-11.03)) ;
#149937=CARTESIAN_POINT('',(2.4,0.3,-11.03)) ;
#149938=CARTESIAN_POINT('',(6.65857864376269,-0.300000000000001,-11.03)) ;
#149939=CARTESIAN_POINT('Origin',(0.6,-0.600000000000001,-11.83)) ;
#149940=CARTESIAN_POINT('',(6.65857864376269,0.300000000000002,-11.83)) ;
#149941=CARTESIAN_POINT('',(0.6,0.299999999999999,-11.83)) ;
#149942=CARTESIAN_POINT('',(6.65857864376269,-0.300000000000001,-11.83)) ;
#149943=CARTESIAN_POINT('',(6.65857864376269,-0.6,-11.83)) ;
#149944=CARTESIAN_POINT('',(0.6,-0.3,-11.83)) ;
#149945=CARTESIAN_POINT('Origin',(-0.4,-0.600000000000001,-14.84)) ;
#149946=CARTESIAN_POINT('',(-0.4,-0.600000000000001,-14.94)) ;
#149947=CARTESIAN_POINT('',(-0.4,-0.600000000000001,-15.54)) ;
#149948=CARTESIAN_POINT('',(-0.4,-0.600000000000001,-14.84)) ;
#149949=CARTESIAN_POINT('',(-0.4,-6.05857864376269,-15.54)) ;
#149950=CARTESIAN_POINT('',(-0.4,-0.600000000000001,-15.54)) ;
#149951=CARTESIAN_POINT('',(-0.4,-6.05857864376269,-14.94)) ;
#149952=CARTESIAN_POINT('',(-0.4,-6.05857864376269,-14.84)) ;
#149953=CARTESIAN_POINT('',(-0.4,-0.600000000000001,-14.94)) ;
#149954=CARTESIAN_POINT('Origin',(-0.4,-6.1,-14.84)) ;
#149955=CARTESIAN_POINT('',(-0.129289321881346,-6.37071067811866,-15.2985786437627)) ;
#149956=CARTESIAN_POINT('',(-0.129289321881346,-6.37071067811866,-15.1814213562373)) ;
#149957=CARTESIAN_POINT('',(-0.129289321881346,-6.37071067811866,-14.84)) ;
#149958=CARTESIAN_POINT('',(-0.370710678118655,-6.12928932188134,-14.94)) ;
#149959=CARTESIAN_POINT('',(-0.423570226039552,-6.07642977396045,-14.8871404520791)) ;
#149960=CARTESIAN_POINT('',(-0.370710678118655,-6.12928932188134,-15.54)) ;
#149961=CARTESIAN_POINT('',(-0.370710678118655,-6.12928932188134,-14.84)) ;
#149962=CARTESIAN_POINT('',(-0.156903559372884,-6.34309644062712,-15.3261928812542)) ;
#149963=CARTESIAN_POINT('Origin',(-0.1,-6.4,-14.84)) ;
#149964=CARTESIAN_POINT('',(0.0585786437626908,-6.4,-15.2985786437627)) ;
#149965=CARTESIAN_POINT('',(0.0585786437626908,-6.4,-15.1814213562373)) ;
#149966=CARTESIAN_POINT('',(0.0585786437626908,-6.4,-14.84)) ;
#149967=CARTESIAN_POINT('',(-0.0585786437626908,-6.4,-15.1814213562373)) ;
#149968=CARTESIAN_POINT('',(-0.1,-6.4,-15.1814213562373)) ;
#149969=CARTESIAN_POINT('',(-0.0585786437626908,-6.4,-15.2985786437627)) ;
#149970=CARTESIAN_POINT('',(-0.0585786437626908,-6.4,-14.84)) ;
#149971=CARTESIAN_POINT('',(-0.1,-6.4,-15.2985786437627)) ;
#149972=CARTESIAN_POINT('Origin',(0.1,-6.4,-14.84)) ;
#149973=CARTESIAN_POINT('',(0.370710678118655,-6.12928932188134,-15.54)) ;
#149974=CARTESIAN_POINT('',(0.370710678118655,-6.12928932188134,-14.94)) ;
#149975=CARTESIAN_POINT('',(0.370710678118655,-6.12928932188134,-14.84)) ;
#149976=CARTESIAN_POINT('',(0.129289321881346,-6.37071067811866,-15.1814213562373)) ;
#149977=CARTESIAN_POINT('',(0.223570226039553,-6.27642977396045,-15.0871404520791)) ;
#149978=CARTESIAN_POINT('',(0.129289321881346,-6.37071067811866,-15.2985786437627)) ;
#149979=CARTESIAN_POINT('',(0.129289321881346,-6.37071067811866,-14.84)) ;
#149980=CARTESIAN_POINT('',(-0.0430964406271151,-6.54309644062712,-15.1261928812542)) ;
#149981=CARTESIAN_POINT('Origin',(0.4,-6.1,-14.84)) ;
#149982=CARTESIAN_POINT('',(0.4,-6.05857864376269,-14.94)) ;
#149983=CARTESIAN_POINT('',(0.4,-6.05857864376269,-15.54)) ;
#149984=CARTESIAN_POINT('',(0.4,-6.05857864376269,-14.84)) ;
#149985=CARTESIAN_POINT('',(0.4,-0.6,-15.54)) ;
#149986=CARTESIAN_POINT('',(0.4,-6.1,-15.54)) ;
#149987=CARTESIAN_POINT('',(0.4,-0.6,-14.94)) ;
#149988=CARTESIAN_POINT('',(0.4,-0.6,-14.84)) ;
#149989=CARTESIAN_POINT('',(0.4,-6.05857864376269,-14.94)) ;
#149990=CARTESIAN_POINT('Origin',(0.6,-0.600000000000001,-14.84)) ;
#149991=CARTESIAN_POINT('',(0.3,-6.05857864376269,-14.84)) ;
#149992=CARTESIAN_POINT('',(0.3,-0.6,-14.84)) ;
#149993=CARTESIAN_POINT('',(0.3,-0.6,-14.84)) ;
#149994=CARTESIAN_POINT('Origin',(0.6,-0.6,-14.84)) ;
#149995=CARTESIAN_POINT('',(-0.3,-0.600000000000001,-14.84)) ;
#149996=CARTESIAN_POINT('Origin',(0.6,-0.600000000000001,-14.84)) ;
#149997=CARTESIAN_POINT('',(-0.300000000000001,-6.05857864376269,-14.84)) ;
#149998=CARTESIAN_POINT('',(-0.3,-0.600000000000001,-14.84)) ;
#149999=CARTESIAN_POINT('',(0.4,-6.05857864376269,-14.84)) ;
#150000=CARTESIAN_POINT('Origin',(0.6,-0.600000000000001,-15.64)) ;
#150001=CARTESIAN_POINT('',(-0.299999999999999,-6.05857864376269,-15.64)) ;
#150002=CARTESIAN_POINT('',(-0.3,-0.600000000000001,-15.64)) ;
#150003=CARTESIAN_POINT('',(-0.3,-0.600000000000001,-15.64)) ;
#150004=CARTESIAN_POINT('Origin',(0.6,-0.600000000000001,-15.64)) ;
#150005=CARTESIAN_POINT('',(0.3,-0.6,-15.64)) ;
#150006=CARTESIAN_POINT('Origin',(0.6,-0.6,-15.64)) ;
#150007=CARTESIAN_POINT('',(0.3,-6.05857864376269,-15.64)) ;
#150008=CARTESIAN_POINT('',(0.3,-0.600000000000001,-15.64)) ;
#150009=CARTESIAN_POINT('',(0.6,-6.05857864376269,-15.64)) ;
#150010=CARTESIAN_POINT('Origin',(0.6,-0.600000000000001,-14.84)) ;
#150011=CARTESIAN_POINT('Origin',(0.6,-0.600000000000001,-15.54)) ;
#150012=CARTESIAN_POINT('Origin',(0.6,-0.600000000000001,-14.94)) ;
#150013=CARTESIAN_POINT('Origin',(0.6,-0.6,-14.84)) ;
#150014=CARTESIAN_POINT('Origin',(0.6,-0.6,-15.54)) ;
#150015=CARTESIAN_POINT('Origin',(0.6,-0.6,-14.94)) ;
#150016=CARTESIAN_POINT('Origin',(7.,0.1,-14.84)) ;
#150017=CARTESIAN_POINT('',(6.72928932188135,0.370710678118655,-15.54)) ;
#150018=CARTESIAN_POINT('',(6.72928932188135,0.370710678118655,-14.94)) ;
#150019=CARTESIAN_POINT('',(6.72928932188135,0.370710678118655,-14.84)) ;
#150020=CARTESIAN_POINT('',(6.97071067811866,0.129289321881346,-15.1814213562373)) ;
#150021=CARTESIAN_POINT('',(6.87642977396045,0.223570226039552,-15.0871404520791)) ;
#150022=CARTESIAN_POINT('',(6.97071067811866,0.129289321881346,-15.2985786437627)) ;
#150023=CARTESIAN_POINT('',(6.97071067811866,0.129289321881346,-14.84)) ;
#150024=CARTESIAN_POINT('',(7.14309644062712,-0.0430964406271147,-15.1261928812542)) ;
#150025=CARTESIAN_POINT('Origin',(6.7,0.400000000000001,-14.84)) ;
#150026=CARTESIAN_POINT('',(6.65857864376269,0.400000000000001,-14.94)) ;
#150027=CARTESIAN_POINT('',(6.65857864376269,0.400000000000001,-15.54)) ;
#150028=CARTESIAN_POINT('',(6.65857864376269,0.400000000000001,-14.84)) ;
#150029=CARTESIAN_POINT('',(6.7,0.400000000000001,-15.54)) ;
#150030=CARTESIAN_POINT('',(6.65857864376269,0.400000000000001,-14.94)) ;
#150031=CARTESIAN_POINT('Origin',(0.6,-0.4,-14.84)) ;
#150032=CARTESIAN_POINT('',(6.65857864376269,-0.400000000000001,-15.54)) ;
#150033=CARTESIAN_POINT('',(0.6,-0.4,-15.54)) ;
#150034=CARTESIAN_POINT('',(6.65857864376269,-0.400000000000001,-14.94)) ;
#150035=CARTESIAN_POINT('',(6.65857864376269,-0.400000000000001,-14.84)) ;
#150036=CARTESIAN_POINT('',(2.4,-0.4,-14.94)) ;
#150037=CARTESIAN_POINT('Origin',(6.7,-0.400000000000001,-14.84)) ;
#150038=CARTESIAN_POINT('',(6.97071067811866,-0.129289321881346,-15.2985786437627)) ;
#150039=CARTESIAN_POINT('',(6.97071067811866,-0.129289321881346,-15.1814213562373)) ;
#150040=CARTESIAN_POINT('',(6.97071067811866,-0.129289321881346,-14.84)) ;
#150041=CARTESIAN_POINT('',(6.72928932188135,-0.370710678118655,-14.94)) ;
#150042=CARTESIAN_POINT('',(6.67642977396045,-0.423570226039552,-14.8871404520791)) ;
#150043=CARTESIAN_POINT('',(6.72928932188135,-0.370710678118655,-15.54)) ;
#150044=CARTESIAN_POINT('',(6.72928932188135,-0.370710678118655,-14.84)) ;
#150045=CARTESIAN_POINT('',(6.94309644062712,-0.156903559372885,-15.3261928812542)) ;
#150046=CARTESIAN_POINT('Origin',(7.,-0.1,-14.84)) ;
#150047=CARTESIAN_POINT('',(7.,-0.0585786437626909,-15.1814213562373)) ;
#150048=CARTESIAN_POINT('',(7.,-0.0585786437626909,-15.2985786437627)) ;
#150049=CARTESIAN_POINT('',(7.,-0.0585786437626909,-14.84)) ;
#150050=CARTESIAN_POINT('',(7.,0.0585786437626909,-15.2985786437627)) ;
#150051=CARTESIAN_POINT('',(7.,-0.1,-15.2985786437627)) ;
#150052=CARTESIAN_POINT('',(7.,0.0585786437626909,-15.1814213562373)) ;
#150053=CARTESIAN_POINT('',(7.,0.0585786437626909,-14.84)) ;
#150054=CARTESIAN_POINT('',(7.,-0.1,-15.1814213562373)) ;
#150055=CARTESIAN_POINT('Origin',(0.6,-0.600000000000001,-14.84)) ;
#150056=CARTESIAN_POINT('',(6.65857864376269,-0.300000000000001,-14.84)) ;
#150057=CARTESIAN_POINT('',(6.65857864376269,0.3,-14.84)) ;
#150058=CARTESIAN_POINT('',(6.65857864376269,-0.399999999999999,-14.84)) ;
#150059=CARTESIAN_POINT('',(2.4,0.3,-14.84)) ;
#150060=CARTESIAN_POINT('',(6.65857864376269,-0.300000000000001,-14.84)) ;
#150061=CARTESIAN_POINT('Origin',(0.6,-0.600000000000001,-15.64)) ;
#150062=CARTESIAN_POINT('',(6.65857864376269,0.300000000000003,-15.64)) ;
#150063=CARTESIAN_POINT('',(0.6,0.299999999999999,-15.64)) ;
#150064=CARTESIAN_POINT('',(6.65857864376269,-0.300000000000001,-15.64)) ;
#150065=CARTESIAN_POINT('',(6.65857864376269,-0.6,-15.64)) ;
#150066=CARTESIAN_POINT('',(0.6,-0.3,-15.64)) ;
#150067=CARTESIAN_POINT('Origin',(-0.4,-0.600000000000001,-18.65)) ;
#150068=CARTESIAN_POINT('',(-0.4,-0.600000000000001,-18.75)) ;
#150069=CARTESIAN_POINT('',(-0.4,-0.600000000000001,-19.35)) ;
#150070=CARTESIAN_POINT('',(-0.4,-0.600000000000001,-18.65)) ;
#150071=CARTESIAN_POINT('',(-0.4,-6.05857864376269,-19.35)) ;
#150072=CARTESIAN_POINT('',(-0.4,-0.600000000000001,-19.35)) ;
#150073=CARTESIAN_POINT('',(-0.4,-6.05857864376269,-18.75)) ;
#150074=CARTESIAN_POINT('',(-0.4,-6.05857864376269,-18.65)) ;
#150075=CARTESIAN_POINT('',(-0.4,-0.600000000000001,-18.75)) ;
#150076=CARTESIAN_POINT('Origin',(-0.4,-6.1,-18.65)) ;
#150077=CARTESIAN_POINT('',(-0.129289321881345,-6.37071067811866,-19.1085786437627)) ;
#150078=CARTESIAN_POINT('',(-0.129289321881346,-6.37071067811866,-18.9914213562373)) ;
#150079=CARTESIAN_POINT('',(-0.129289321881346,-6.37071067811866,-18.65)) ;
#150080=CARTESIAN_POINT('',(-0.370710678118655,-6.12928932188134,-18.75)) ;
#150081=CARTESIAN_POINT('',(-0.423570226039551,-6.07642977396045,-18.6971404520791)) ;
#150082=CARTESIAN_POINT('',(-0.370710678118655,-6.12928932188134,-19.35)) ;
#150083=CARTESIAN_POINT('',(-0.370710678118655,-6.12928932188134,-18.65)) ;
#150084=CARTESIAN_POINT('',(-0.156903559372884,-6.34309644062712,-19.1361928812542)) ;
#150085=CARTESIAN_POINT('Origin',(-0.1,-6.4,-18.65)) ;
#150086=CARTESIAN_POINT('',(0.0585786437626908,-6.4,-19.1085786437627)) ;
#150087=CARTESIAN_POINT('',(0.0585786437626908,-6.4,-18.9914213562373)) ;
#150088=CARTESIAN_POINT('',(0.0585786437626908,-6.4,-18.65)) ;
#150089=CARTESIAN_POINT('',(-0.0585786437626908,-6.4,-18.9914213562373)) ;
#150090=CARTESIAN_POINT('',(-0.1,-6.4,-18.9914213562373)) ;
#150091=CARTESIAN_POINT('',(-0.0585786437626908,-6.4,-19.1085786437627)) ;
#150092=CARTESIAN_POINT('',(-0.0585786437626908,-6.4,-18.65)) ;
#150093=CARTESIAN_POINT('',(-0.1,-6.4,-19.1085786437627)) ;
#150094=CARTESIAN_POINT('Origin',(0.1,-6.4,-18.65)) ;
#150095=CARTESIAN_POINT('',(0.370710678118654,-6.12928932188135,-19.35)) ;
#150096=CARTESIAN_POINT('',(0.370710678118655,-6.12928932188134,-18.75)) ;
#150097=CARTESIAN_POINT('',(0.370710678118655,-6.12928932188134,-18.65)) ;
#150098=CARTESIAN_POINT('',(0.129289321881346,-6.37071067811866,-18.9914213562373)) ;
#150099=CARTESIAN_POINT('',(0.223570226039551,-6.27642977396045,-18.8971404520791)) ;
#150100=CARTESIAN_POINT('',(0.129289321881346,-6.37071067811866,-19.1085786437627)) ;
#150101=CARTESIAN_POINT('',(0.129289321881346,-6.37071067811866,-18.65)) ;
#150102=CARTESIAN_POINT('',(-0.0430964406271139,-6.54309644062711,-18.9361928812542)) ;
#150103=CARTESIAN_POINT('Origin',(0.4,-6.1,-18.65)) ;
#150104=CARTESIAN_POINT('',(0.4,-6.05857864376269,-18.75)) ;
#150105=CARTESIAN_POINT('',(0.4,-6.05857864376269,-19.35)) ;
#150106=CARTESIAN_POINT('',(0.4,-6.05857864376269,-18.65)) ;
#150107=CARTESIAN_POINT('',(0.4,-0.6,-19.35)) ;
#150108=CARTESIAN_POINT('',(0.4,-6.1,-19.35)) ;
#150109=CARTESIAN_POINT('',(0.4,-0.6,-18.75)) ;
#150110=CARTESIAN_POINT('',(0.4,-0.6,-18.65)) ;
#150111=CARTESIAN_POINT('',(0.4,-6.05857864376269,-18.75)) ;
#150112=CARTESIAN_POINT('Origin',(0.6,-0.600000000000001,-18.65)) ;
#150113=CARTESIAN_POINT('',(0.3,-6.05857864376269,-18.65)) ;
#150114=CARTESIAN_POINT('',(0.3,-0.6,-18.65)) ;
#150115=CARTESIAN_POINT('',(0.3,-0.6,-18.65)) ;
#150116=CARTESIAN_POINT('Origin',(0.6,-0.6,-18.65)) ;
#150117=CARTESIAN_POINT('',(-0.3,-0.600000000000001,-18.65)) ;
#150118=CARTESIAN_POINT('Origin',(0.6,-0.600000000000001,-18.65)) ;
#150119=CARTESIAN_POINT('',(-0.299999999999994,-6.0585786437627,-18.65)) ;
#150120=CARTESIAN_POINT('',(-0.3,-0.600000000000001,-18.65)) ;
#150121=CARTESIAN_POINT('',(0.4,-6.0585786437627,-18.65)) ;
#150122=CARTESIAN_POINT('Origin',(0.6,-0.600000000000001,-19.45)) ;
#150123=CARTESIAN_POINT('',(-0.299999999999994,-6.0585786437627,-19.45)) ;
#150124=CARTESIAN_POINT('',(-0.3,-0.600000000000001,-19.45)) ;
#150125=CARTESIAN_POINT('',(-0.3,-0.600000000000001,-19.45)) ;
#150126=CARTESIAN_POINT('Origin',(0.6,-0.600000000000001,-19.45)) ;
#150127=CARTESIAN_POINT('',(0.3,-0.6,-19.45)) ;
#150128=CARTESIAN_POINT('Origin',(0.6,-0.6,-19.45)) ;
#150129=CARTESIAN_POINT('',(0.3,-6.05857864376269,-19.45)) ;
#150130=CARTESIAN_POINT('',(0.3,-0.600000000000001,-19.45)) ;
#150131=CARTESIAN_POINT('',(0.6,-6.05857864376269,-19.45)) ;
#150132=CARTESIAN_POINT('Origin',(0.6,-0.600000000000001,-18.65)) ;
#150133=CARTESIAN_POINT('Origin',(0.6,-0.600000000000001,-19.35)) ;
#150134=CARTESIAN_POINT('Origin',(0.6,-0.600000000000001,-18.75)) ;
#150135=CARTESIAN_POINT('Origin',(0.6,-0.6,-18.65)) ;
#150136=CARTESIAN_POINT('Origin',(0.6,-0.6,-19.35)) ;
#150137=CARTESIAN_POINT('Origin',(0.6,-0.6,-18.75)) ;
#150138=CARTESIAN_POINT('Origin',(7.,0.1,-18.65)) ;
#150139=CARTESIAN_POINT('',(6.72928932188135,0.370710678118656,-19.35)) ;
#150140=CARTESIAN_POINT('',(6.72928932188135,0.370710678118655,-18.75)) ;
#150141=CARTESIAN_POINT('',(6.72928932188135,0.370710678118655,-18.65)) ;
#150142=CARTESIAN_POINT('',(6.97071067811866,0.129289321881346,-18.9914213562373)) ;
#150143=CARTESIAN_POINT('',(6.87642977396045,0.22357022603955,-18.8971404520791)) ;
#150144=CARTESIAN_POINT('',(6.97071067811866,0.129289321881346,-19.1085786437627)) ;
#150145=CARTESIAN_POINT('',(6.97071067811866,0.129289321881346,-18.65)) ;
#150146=CARTESIAN_POINT('',(7.14309644062712,-0.0430964406271155,-18.9361928812542)) ;
#150147=CARTESIAN_POINT('Origin',(6.7,0.400000000000001,-18.65)) ;
#150148=CARTESIAN_POINT('',(6.65857864376269,0.400000000000001,-18.75)) ;
#150149=CARTESIAN_POINT('',(6.65857864376269,0.400000000000001,-19.35)) ;
#150150=CARTESIAN_POINT('',(6.65857864376269,0.400000000000001,-18.65)) ;
#150151=CARTESIAN_POINT('',(6.7,0.400000000000001,-19.35)) ;
#150152=CARTESIAN_POINT('',(6.65857864376269,0.400000000000001,-18.75)) ;
#150153=CARTESIAN_POINT('Origin',(0.6,-0.4,-18.65)) ;
#150154=CARTESIAN_POINT('',(6.65857864376269,-0.400000000000001,-19.35)) ;
#150155=CARTESIAN_POINT('',(0.6,-0.4,-19.35)) ;
#150156=CARTESIAN_POINT('',(6.65857864376269,-0.400000000000001,-18.75)) ;
#150157=CARTESIAN_POINT('',(6.65857864376269,-0.400000000000001,-18.65)) ;
#150158=CARTESIAN_POINT('',(2.4,-0.4,-18.75)) ;
#150159=CARTESIAN_POINT('Origin',(6.7,-0.400000000000001,-18.65)) ;
#150160=CARTESIAN_POINT('',(6.97071067811866,-0.129289321881345,-19.1085786437627)) ;
#150161=CARTESIAN_POINT('',(6.97071067811866,-0.129289321881346,-18.9914213562373)) ;
#150162=CARTESIAN_POINT('',(6.97071067811866,-0.129289321881346,-18.65)) ;
#150163=CARTESIAN_POINT('',(6.72928932188135,-0.370710678118655,-18.75)) ;
#150164=CARTESIAN_POINT('',(6.67642977396045,-0.423570226039551,-18.6971404520791)) ;
#150165=CARTESIAN_POINT('',(6.72928932188135,-0.370710678118655,-19.35)) ;
#150166=CARTESIAN_POINT('',(6.72928932188135,-0.370710678118655,-18.65)) ;
#150167=CARTESIAN_POINT('',(6.94309644062712,-0.156903559372885,-19.1361928812542)) ;
#150168=CARTESIAN_POINT('Origin',(7.,-0.1,-18.65)) ;
#150169=CARTESIAN_POINT('',(7.,-0.0585786437626909,-18.9914213562373)) ;
#150170=CARTESIAN_POINT('',(7.,-0.0585786437626909,-19.1085786437627)) ;
#150171=CARTESIAN_POINT('',(7.,-0.0585786437626909,-18.65)) ;
#150172=CARTESIAN_POINT('',(7.,0.0585786437626909,-19.1085786437627)) ;
#150173=CARTESIAN_POINT('',(7.,-0.1,-19.1085786437627)) ;
#150174=CARTESIAN_POINT('',(7.,0.0585786437626909,-18.9914213562373)) ;
#150175=CARTESIAN_POINT('',(7.,0.0585786437626909,-18.65)) ;
#150176=CARTESIAN_POINT('',(7.,-0.1,-18.9914213562373)) ;
#150177=CARTESIAN_POINT('Origin',(0.6,-0.600000000000001,-18.65)) ;
#150178=CARTESIAN_POINT('',(6.65857864376269,-0.300000000000001,-18.65)) ;
#150179=CARTESIAN_POINT('',(6.6585786437627,0.299999999999992,-18.65)) ;
#150180=CARTESIAN_POINT('',(6.6585786437627,-0.399999999999999,-18.65)) ;
#150181=CARTESIAN_POINT('',(2.4,0.3,-18.65)) ;
#150182=CARTESIAN_POINT('',(6.65857864376269,-0.300000000000001,-18.65)) ;
#150183=CARTESIAN_POINT('Origin',(0.6,-0.600000000000001,-19.45)) ;
#150184=CARTESIAN_POINT('',(6.65857864376269,0.299999999999998,-19.45)) ;
#150185=CARTESIAN_POINT('',(0.6,0.299999999999999,-19.45)) ;
#150186=CARTESIAN_POINT('',(6.65857864376269,-0.300000000000001,-19.45)) ;
#150187=CARTESIAN_POINT('',(6.65857864376269,-0.6,-19.45)) ;
#150188=CARTESIAN_POINT('',(0.6,-0.3,-19.45)) ;
#150189=CARTESIAN_POINT('Origin',(-0.4,-0.600000000000001,-22.46)) ;
#150190=CARTESIAN_POINT('',(-0.4,-0.600000000000001,-22.56)) ;
#150191=CARTESIAN_POINT('',(-0.4,-0.600000000000001,-23.16)) ;
#150192=CARTESIAN_POINT('',(-0.4,-0.600000000000001,-22.46)) ;
#150193=CARTESIAN_POINT('',(-0.4,-6.05857864376269,-23.16)) ;
#150194=CARTESIAN_POINT('',(-0.4,-0.600000000000001,-23.16)) ;
#150195=CARTESIAN_POINT('',(-0.4,-6.05857864376269,-22.56)) ;
#150196=CARTESIAN_POINT('',(-0.4,-6.05857864376269,-22.46)) ;
#150197=CARTESIAN_POINT('',(-0.4,-0.600000000000001,-22.56)) ;
#150198=CARTESIAN_POINT('Origin',(-0.4,-6.1,-22.46)) ;
#150199=CARTESIAN_POINT('',(-0.129289321881345,-6.37071067811866,-22.9185786437627)) ;
#150200=CARTESIAN_POINT('',(-0.129289321881346,-6.37071067811866,-22.8014213562373)) ;
#150201=CARTESIAN_POINT('',(-0.129289321881346,-6.37071067811866,-22.46)) ;
#150202=CARTESIAN_POINT('',(-0.370710678118655,-6.12928932188134,-22.56)) ;
#150203=CARTESIAN_POINT('',(-0.423570226039551,-6.07642977396045,-22.5071404520791)) ;
#150204=CARTESIAN_POINT('',(-0.370710678118655,-6.12928932188134,-23.16)) ;
#150205=CARTESIAN_POINT('',(-0.370710678118655,-6.12928932188134,-22.46)) ;
#150206=CARTESIAN_POINT('',(-0.156903559372884,-6.34309644062712,-22.9461928812542)) ;
#150207=CARTESIAN_POINT('Origin',(-0.1,-6.4,-22.46)) ;
#150208=CARTESIAN_POINT('',(0.0585786437626908,-6.4,-22.9185786437627)) ;
#150209=CARTESIAN_POINT('',(0.0585786437626908,-6.4,-22.8014213562373)) ;
#150210=CARTESIAN_POINT('',(0.0585786437626908,-6.4,-22.46)) ;
#150211=CARTESIAN_POINT('',(-0.0585786437626908,-6.4,-22.8014213562373)) ;
#150212=CARTESIAN_POINT('',(-0.1,-6.4,-22.8014213562373)) ;
#150213=CARTESIAN_POINT('',(-0.0585786437626908,-6.4,-22.9185786437627)) ;
#150214=CARTESIAN_POINT('',(-0.0585786437626908,-6.4,-22.46)) ;
#150215=CARTESIAN_POINT('',(-0.1,-6.4,-22.9185786437627)) ;
#150216=CARTESIAN_POINT('Origin',(0.1,-6.4,-22.46)) ;
#150217=CARTESIAN_POINT('',(0.370710678118654,-6.12928932188135,-23.16)) ;
#150218=CARTESIAN_POINT('',(0.370710678118655,-6.12928932188134,-22.56)) ;
#150219=CARTESIAN_POINT('',(0.370710678118655,-6.12928932188134,-22.46)) ;
#150220=CARTESIAN_POINT('',(0.129289321881346,-6.37071067811866,-22.8014213562373)) ;
#150221=CARTESIAN_POINT('',(0.223570226039551,-6.27642977396045,-22.7071404520791)) ;
#150222=CARTESIAN_POINT('',(0.129289321881346,-6.37071067811866,-22.9185786437627)) ;
#150223=CARTESIAN_POINT('',(0.129289321881346,-6.37071067811866,-22.46)) ;
#150224=CARTESIAN_POINT('',(-0.0430964406271139,-6.54309644062711,-22.7461928812542)) ;
#150225=CARTESIAN_POINT('Origin',(0.4,-6.1,-22.46)) ;
#150226=CARTESIAN_POINT('',(0.4,-6.05857864376269,-22.56)) ;
#150227=CARTESIAN_POINT('',(0.4,-6.05857864376269,-23.16)) ;
#150228=CARTESIAN_POINT('',(0.4,-6.05857864376269,-22.46)) ;
#150229=CARTESIAN_POINT('',(0.4,-0.6,-23.16)) ;
#150230=CARTESIAN_POINT('',(0.4,-6.1,-23.16)) ;
#150231=CARTESIAN_POINT('',(0.4,-0.6,-22.56)) ;
#150232=CARTESIAN_POINT('',(0.4,-0.6,-22.46)) ;
#150233=CARTESIAN_POINT('',(0.4,-6.05857864376269,-22.56)) ;
#150234=CARTESIAN_POINT('Origin',(0.6,-0.600000000000001,-22.46)) ;
#150235=CARTESIAN_POINT('',(0.3,-6.05857864376269,-22.46)) ;
#150236=CARTESIAN_POINT('',(0.3,-0.6,-22.46)) ;
#150237=CARTESIAN_POINT('',(0.3,-0.6,-22.46)) ;
#150238=CARTESIAN_POINT('Origin',(0.6,-0.6,-22.46)) ;
#150239=CARTESIAN_POINT('',(-0.3,-0.600000000000001,-22.46)) ;
#150240=CARTESIAN_POINT('Origin',(0.6,-0.600000000000001,-22.46)) ;
#150241=CARTESIAN_POINT('',(-0.299999999999994,-6.0585786437627,-22.46)) ;
#150242=CARTESIAN_POINT('',(-0.3,-0.600000000000001,-22.46)) ;
#150243=CARTESIAN_POINT('',(0.4,-6.0585786437627,-22.46)) ;
#150244=CARTESIAN_POINT('Origin',(0.6,-0.600000000000001,-23.26)) ;
#150245=CARTESIAN_POINT('',(-0.299999999999994,-6.0585786437627,-23.26)) ;
#150246=CARTESIAN_POINT('',(-0.3,-0.600000000000001,-23.26)) ;
#150247=CARTESIAN_POINT('',(-0.3,-0.600000000000001,-23.26)) ;
#150248=CARTESIAN_POINT('Origin',(0.6,-0.600000000000001,-23.26)) ;
#150249=CARTESIAN_POINT('',(0.3,-0.6,-23.26)) ;
#150250=CARTESIAN_POINT('Origin',(0.6,-0.6,-23.26)) ;
#150251=CARTESIAN_POINT('',(0.3,-6.05857864376269,-23.26)) ;
#150252=CARTESIAN_POINT('',(0.3,-0.600000000000001,-23.26)) ;
#150253=CARTESIAN_POINT('',(0.6,-6.05857864376269,-23.26)) ;
#150254=CARTESIAN_POINT('Origin',(0.6,-0.600000000000001,-22.46)) ;
#150255=CARTESIAN_POINT('Origin',(0.6,-0.600000000000001,-23.16)) ;
#150256=CARTESIAN_POINT('Origin',(0.6,-0.600000000000001,-22.56)) ;
#150257=CARTESIAN_POINT('Origin',(0.6,-0.6,-22.46)) ;
#150258=CARTESIAN_POINT('Origin',(0.6,-0.6,-23.16)) ;
#150259=CARTESIAN_POINT('Origin',(0.6,-0.6,-22.56)) ;
#150260=CARTESIAN_POINT('Origin',(7.,0.1,-22.46)) ;
#150261=CARTESIAN_POINT('',(6.72928932188135,0.370710678118656,-23.16)) ;
#150262=CARTESIAN_POINT('',(6.72928932188135,0.370710678118655,-22.56)) ;
#150263=CARTESIAN_POINT('',(6.72928932188135,0.370710678118655,-22.46)) ;
#150264=CARTESIAN_POINT('',(6.97071067811866,0.129289321881346,-22.8014213562373)) ;
#150265=CARTESIAN_POINT('',(6.87642977396045,0.22357022603955,-22.7071404520791)) ;
#150266=CARTESIAN_POINT('',(6.97071067811866,0.129289321881346,-22.9185786437627)) ;
#150267=CARTESIAN_POINT('',(6.97071067811866,0.129289321881346,-22.46)) ;
#150268=CARTESIAN_POINT('',(7.14309644062712,-0.0430964406271155,-22.7461928812542)) ;
#150269=CARTESIAN_POINT('Origin',(6.7,0.400000000000001,-22.46)) ;
#150270=CARTESIAN_POINT('',(6.65857864376269,0.400000000000001,-22.56)) ;
#150271=CARTESIAN_POINT('',(6.65857864376269,0.400000000000001,-23.16)) ;
#150272=CARTESIAN_POINT('',(6.65857864376269,0.400000000000001,-22.46)) ;
#150273=CARTESIAN_POINT('',(6.7,0.400000000000001,-23.16)) ;
#150274=CARTESIAN_POINT('',(6.65857864376269,0.400000000000001,-22.56)) ;
#150275=CARTESIAN_POINT('Origin',(0.6,-0.4,-22.46)) ;
#150276=CARTESIAN_POINT('',(6.65857864376269,-0.400000000000001,-23.16)) ;
#150277=CARTESIAN_POINT('',(0.6,-0.4,-23.16)) ;
#150278=CARTESIAN_POINT('',(6.65857864376269,-0.400000000000001,-22.56)) ;
#150279=CARTESIAN_POINT('',(6.65857864376269,-0.400000000000001,-22.46)) ;
#150280=CARTESIAN_POINT('',(2.4,-0.4,-22.56)) ;
#150281=CARTESIAN_POINT('Origin',(6.7,-0.400000000000001,-22.46)) ;
#150282=CARTESIAN_POINT('',(6.97071067811866,-0.129289321881345,-22.9185786437627)) ;
#150283=CARTESIAN_POINT('',(6.97071067811866,-0.129289321881346,-22.8014213562373)) ;
#150284=CARTESIAN_POINT('',(6.97071067811866,-0.129289321881346,-22.46)) ;
#150285=CARTESIAN_POINT('',(6.72928932188135,-0.370710678118655,-22.56)) ;
#150286=CARTESIAN_POINT('',(6.67642977396045,-0.423570226039551,-22.5071404520791)) ;
#150287=CARTESIAN_POINT('',(6.72928932188135,-0.370710678118655,-23.16)) ;
#150288=CARTESIAN_POINT('',(6.72928932188135,-0.370710678118655,-22.46)) ;
#150289=CARTESIAN_POINT('',(6.94309644062712,-0.156903559372885,-22.9461928812542)) ;
#150290=CARTESIAN_POINT('Origin',(7.,-0.1,-22.46)) ;
#150291=CARTESIAN_POINT('',(7.,-0.0585786437626909,-22.8014213562373)) ;
#150292=CARTESIAN_POINT('',(7.,-0.0585786437626909,-22.9185786437627)) ;
#150293=CARTESIAN_POINT('',(7.,-0.0585786437626909,-22.46)) ;
#150294=CARTESIAN_POINT('',(7.,0.0585786437626909,-22.9185786437627)) ;
#150295=CARTESIAN_POINT('',(7.,-0.1,-22.9185786437627)) ;
#150296=CARTESIAN_POINT('',(7.,0.0585786437626909,-22.8014213562373)) ;
#150297=CARTESIAN_POINT('',(7.,0.0585786437626909,-22.46)) ;
#150298=CARTESIAN_POINT('',(7.,-0.1,-22.8014213562373)) ;
#150299=CARTESIAN_POINT('Origin',(0.6,-0.600000000000001,-22.46)) ;
#150300=CARTESIAN_POINT('',(6.65857864376269,-0.300000000000001,-22.46)) ;
#150301=CARTESIAN_POINT('',(6.6585786437627,0.299999999999994,-22.46)) ;
#150302=CARTESIAN_POINT('',(6.6585786437627,-0.399999999999999,-22.46)) ;
#150303=CARTESIAN_POINT('',(2.4,0.3,-22.46)) ;
#150304=CARTESIAN_POINT('',(6.65857864376269,-0.300000000000001,-22.46)) ;
#150305=CARTESIAN_POINT('Origin',(0.6,-0.600000000000001,-23.26)) ;
#150306=CARTESIAN_POINT('',(6.65857864376269,0.299999999999998,-23.26)) ;
#150307=CARTESIAN_POINT('',(0.6,0.299999999999999,-23.26)) ;
#150308=CARTESIAN_POINT('',(6.65857864376269,-0.300000000000001,-23.26)) ;
#150309=CARTESIAN_POINT('',(6.65857864376269,-0.6,-23.26)) ;
#150310=CARTESIAN_POINT('',(0.6,-0.3,-23.26)) ;
#150311=CARTESIAN_POINT('Origin',(-0.4,-0.600000000000001,-26.27)) ;
#150312=CARTESIAN_POINT('',(-0.4,-0.600000000000001,-26.37)) ;
#150313=CARTESIAN_POINT('',(-0.4,-0.600000000000001,-26.97)) ;
#150314=CARTESIAN_POINT('',(-0.4,-0.600000000000001,-26.27)) ;
#150315=CARTESIAN_POINT('',(-0.4,-6.05857864376269,-26.97)) ;
#150316=CARTESIAN_POINT('',(-0.4,-0.600000000000001,-26.97)) ;
#150317=CARTESIAN_POINT('',(-0.4,-6.05857864376269,-26.37)) ;
#150318=CARTESIAN_POINT('',(-0.4,-6.05857864376269,-26.27)) ;
#150319=CARTESIAN_POINT('',(-0.4,-0.600000000000001,-26.37)) ;
#150320=CARTESIAN_POINT('Origin',(-0.4,-6.1,-26.27)) ;
#150321=CARTESIAN_POINT('',(-0.129289321881345,-6.37071067811866,-26.7285786437627)) ;
#150322=CARTESIAN_POINT('',(-0.129289321881346,-6.37071067811866,-26.6114213562373)) ;
#150323=CARTESIAN_POINT('',(-0.129289321881346,-6.37071067811866,-26.27)) ;
#150324=CARTESIAN_POINT('',(-0.370710678118655,-6.12928932188134,-26.37)) ;
#150325=CARTESIAN_POINT('',(-0.423570226039551,-6.07642977396045,-26.3171404520791)) ;
#150326=CARTESIAN_POINT('',(-0.370710678118655,-6.12928932188134,-26.97)) ;
#150327=CARTESIAN_POINT('',(-0.370710678118655,-6.12928932188134,-26.27)) ;
#150328=CARTESIAN_POINT('',(-0.156903559372884,-6.34309644062712,-26.7561928812542)) ;
#150329=CARTESIAN_POINT('Origin',(-0.1,-6.4,-26.27)) ;
#150330=CARTESIAN_POINT('',(0.0585786437626908,-6.4,-26.7285786437627)) ;
#150331=CARTESIAN_POINT('',(0.0585786437626908,-6.4,-26.6114213562373)) ;
#150332=CARTESIAN_POINT('',(0.0585786437626908,-6.4,-26.27)) ;
#150333=CARTESIAN_POINT('',(-0.0585786437626908,-6.4,-26.6114213562373)) ;
#150334=CARTESIAN_POINT('',(-0.1,-6.4,-26.6114213562373)) ;
#150335=CARTESIAN_POINT('',(-0.0585786437626908,-6.4,-26.7285786437627)) ;
#150336=CARTESIAN_POINT('',(-0.0585786437626908,-6.4,-26.27)) ;
#150337=CARTESIAN_POINT('',(-0.1,-6.4,-26.7285786437627)) ;
#150338=CARTESIAN_POINT('Origin',(0.1,-6.4,-26.27)) ;
#150339=CARTESIAN_POINT('',(0.370710678118654,-6.12928932188135,-26.97)) ;
#150340=CARTESIAN_POINT('',(0.370710678118655,-6.12928932188134,-26.37)) ;
#150341=CARTESIAN_POINT('',(0.370710678118655,-6.12928932188134,-26.27)) ;
#150342=CARTESIAN_POINT('',(0.129289321881346,-6.37071067811866,-26.6114213562373)) ;
#150343=CARTESIAN_POINT('',(0.223570226039551,-6.27642977396045,-26.5171404520791)) ;
#150344=CARTESIAN_POINT('',(0.129289321881346,-6.37071067811866,-26.7285786437627)) ;
#150345=CARTESIAN_POINT('',(0.129289321881346,-6.37071067811866,-26.27)) ;
#150346=CARTESIAN_POINT('',(-0.0430964406271139,-6.54309644062711,-26.5561928812542)) ;
#150347=CARTESIAN_POINT('Origin',(0.4,-6.1,-26.27)) ;
#150348=CARTESIAN_POINT('',(0.4,-6.05857864376269,-26.37)) ;
#150349=CARTESIAN_POINT('',(0.4,-6.05857864376269,-26.97)) ;
#150350=CARTESIAN_POINT('',(0.4,-6.05857864376269,-26.27)) ;
#150351=CARTESIAN_POINT('',(0.4,-0.6,-26.97)) ;
#150352=CARTESIAN_POINT('',(0.4,-6.1,-26.97)) ;
#150353=CARTESIAN_POINT('',(0.4,-0.6,-26.37)) ;
#150354=CARTESIAN_POINT('',(0.4,-0.6,-26.27)) ;
#150355=CARTESIAN_POINT('',(0.4,-6.05857864376269,-26.37)) ;
#150356=CARTESIAN_POINT('Origin',(0.6,-0.600000000000001,-26.27)) ;
#150357=CARTESIAN_POINT('',(0.3,-6.05857864376269,-26.27)) ;
#150358=CARTESIAN_POINT('',(0.3,-0.6,-26.27)) ;
#150359=CARTESIAN_POINT('',(0.3,-0.6,-26.27)) ;
#150360=CARTESIAN_POINT('Origin',(0.6,-0.6,-26.27)) ;
#150361=CARTESIAN_POINT('',(-0.3,-0.600000000000001,-26.27)) ;
#150362=CARTESIAN_POINT('Origin',(0.6,-0.600000000000001,-26.27)) ;
#150363=CARTESIAN_POINT('',(-0.299999999999994,-6.0585786437627,-26.27)) ;
#150364=CARTESIAN_POINT('',(-0.3,-0.600000000000001,-26.27)) ;
#150365=CARTESIAN_POINT('',(0.4,-6.0585786437627,-26.27)) ;
#150366=CARTESIAN_POINT('Origin',(0.6,-0.600000000000001,-27.07)) ;
#150367=CARTESIAN_POINT('',(-0.299999999999994,-6.0585786437627,-27.07)) ;
#150368=CARTESIAN_POINT('',(-0.3,-0.600000000000001,-27.07)) ;
#150369=CARTESIAN_POINT('',(-0.3,-0.600000000000001,-27.07)) ;
#150370=CARTESIAN_POINT('Origin',(0.6,-0.600000000000001,-27.07)) ;
#150371=CARTESIAN_POINT('',(0.3,-0.6,-27.07)) ;
#150372=CARTESIAN_POINT('Origin',(0.6,-0.6,-27.07)) ;
#150373=CARTESIAN_POINT('',(0.3,-6.05857864376269,-27.07)) ;
#150374=CARTESIAN_POINT('',(0.3,-0.600000000000001,-27.07)) ;
#150375=CARTESIAN_POINT('',(0.6,-6.05857864376269,-27.07)) ;
#150376=CARTESIAN_POINT('Origin',(0.6,-0.600000000000001,-26.27)) ;
#150377=CARTESIAN_POINT('Origin',(0.6,-0.600000000000001,-26.97)) ;
#150378=CARTESIAN_POINT('Origin',(0.6,-0.600000000000001,-26.37)) ;
#150379=CARTESIAN_POINT('Origin',(0.6,-0.6,-26.27)) ;
#150380=CARTESIAN_POINT('Origin',(0.6,-0.6,-26.97)) ;
#150381=CARTESIAN_POINT('Origin',(0.6,-0.6,-26.37)) ;
#150382=CARTESIAN_POINT('Origin',(7.,0.1,-26.27)) ;
#150383=CARTESIAN_POINT('',(6.72928932188135,0.370710678118656,-26.97)) ;
#150384=CARTESIAN_POINT('',(6.72928932188135,0.370710678118655,-26.37)) ;
#150385=CARTESIAN_POINT('',(6.72928932188135,0.370710678118655,-26.27)) ;
#150386=CARTESIAN_POINT('',(6.97071067811866,0.129289321881346,-26.6114213562373)) ;
#150387=CARTESIAN_POINT('',(6.87642977396045,0.22357022603955,-26.5171404520791)) ;
#150388=CARTESIAN_POINT('',(6.97071067811866,0.129289321881346,-26.7285786437627)) ;
#150389=CARTESIAN_POINT('',(6.97071067811866,0.129289321881346,-26.27)) ;
#150390=CARTESIAN_POINT('',(7.14309644062712,-0.0430964406271155,-26.5561928812542)) ;
#150391=CARTESIAN_POINT('Origin',(6.7,0.400000000000001,-26.27)) ;
#150392=CARTESIAN_POINT('',(6.65857864376269,0.400000000000001,-26.37)) ;
#150393=CARTESIAN_POINT('',(6.65857864376269,0.400000000000001,-26.97)) ;
#150394=CARTESIAN_POINT('',(6.65857864376269,0.400000000000001,-26.27)) ;
#150395=CARTESIAN_POINT('',(6.7,0.400000000000001,-26.97)) ;
#150396=CARTESIAN_POINT('',(6.65857864376269,0.400000000000001,-26.37)) ;
#150397=CARTESIAN_POINT('Origin',(0.6,-0.4,-26.27)) ;
#150398=CARTESIAN_POINT('',(6.65857864376269,-0.400000000000001,-26.97)) ;
#150399=CARTESIAN_POINT('',(0.6,-0.4,-26.97)) ;
#150400=CARTESIAN_POINT('',(6.65857864376269,-0.400000000000001,-26.37)) ;
#150401=CARTESIAN_POINT('',(6.65857864376269,-0.400000000000001,-26.27)) ;
#150402=CARTESIAN_POINT('',(2.4,-0.4,-26.37)) ;
#150403=CARTESIAN_POINT('Origin',(6.7,-0.400000000000001,-26.27)) ;
#150404=CARTESIAN_POINT('',(6.97071067811866,-0.129289321881345,-26.7285786437627)) ;
#150405=CARTESIAN_POINT('',(6.97071067811866,-0.129289321881346,-26.6114213562373)) ;
#150406=CARTESIAN_POINT('',(6.97071067811866,-0.129289321881346,-26.27)) ;
#150407=CARTESIAN_POINT('',(6.72928932188135,-0.370710678118655,-26.37)) ;
#150408=CARTESIAN_POINT('',(6.67642977396045,-0.423570226039551,-26.3171404520791)) ;
#150409=CARTESIAN_POINT('',(6.72928932188135,-0.370710678118655,-26.97)) ;
#150410=CARTESIAN_POINT('',(6.72928932188135,-0.370710678118655,-26.27)) ;
#150411=CARTESIAN_POINT('',(6.94309644062712,-0.156903559372885,-26.7561928812542)) ;
#150412=CARTESIAN_POINT('Origin',(7.,-0.1,-26.27)) ;
#150413=CARTESIAN_POINT('',(7.,-0.0585786437626909,-26.6114213562373)) ;
#150414=CARTESIAN_POINT('',(7.,-0.0585786437626909,-26.7285786437627)) ;
#150415=CARTESIAN_POINT('',(7.,-0.0585786437626909,-26.27)) ;
#150416=CARTESIAN_POINT('',(7.,0.0585786437626909,-26.7285786437627)) ;
#150417=CARTESIAN_POINT('',(7.,-0.1,-26.7285786437627)) ;
#150418=CARTESIAN_POINT('',(7.,0.0585786437626909,-26.6114213562373)) ;
#150419=CARTESIAN_POINT('',(7.,0.0585786437626909,-26.27)) ;
#150420=CARTESIAN_POINT('',(7.,-0.1,-26.6114213562373)) ;
#150421=CARTESIAN_POINT('Origin',(0.6,-0.600000000000001,-26.27)) ;
#150422=CARTESIAN_POINT('',(6.65857864376269,-0.300000000000001,-26.27)) ;
#150423=CARTESIAN_POINT('',(6.6585786437627,0.299999999999994,-26.27)) ;
#150424=CARTESIAN_POINT('',(6.6585786437627,-0.399999999999999,-26.27)) ;
#150425=CARTESIAN_POINT('',(2.4,0.3,-26.27)) ;
#150426=CARTESIAN_POINT('',(6.65857864376269,-0.300000000000001,-26.27)) ;
#150427=CARTESIAN_POINT('Origin',(0.6,-0.600000000000001,-27.07)) ;
#150428=CARTESIAN_POINT('',(6.65857864376269,0.299999999999998,-27.07)) ;
#150429=CARTESIAN_POINT('',(0.6,0.299999999999999,-27.07)) ;
#150430=CARTESIAN_POINT('',(6.65857864376269,-0.300000000000001,-27.07)) ;
#150431=CARTESIAN_POINT('',(6.65857864376269,-0.6,-27.07)) ;
#150432=CARTESIAN_POINT('',(0.6,-0.3,-27.07)) ;
#150433=CARTESIAN_POINT('Origin',(-0.4,-0.600000000000001,-30.08)) ;
#150434=CARTESIAN_POINT('',(-0.4,-0.600000000000001,-30.18)) ;
#150435=CARTESIAN_POINT('',(-0.4,-0.600000000000001,-30.78)) ;
#150436=CARTESIAN_POINT('',(-0.4,-0.600000000000001,-30.08)) ;
#150437=CARTESIAN_POINT('',(-0.4,-6.05857864376269,-30.78)) ;
#150438=CARTESIAN_POINT('',(-0.4,-0.600000000000001,-30.78)) ;
#150439=CARTESIAN_POINT('',(-0.4,-6.05857864376269,-30.18)) ;
#150440=CARTESIAN_POINT('',(-0.4,-6.05857864376269,-30.08)) ;
#150441=CARTESIAN_POINT('',(-0.4,-0.600000000000001,-30.18)) ;
#150442=CARTESIAN_POINT('Origin',(-0.4,-6.1,-30.08)) ;
#150443=CARTESIAN_POINT('',(-0.129289321881345,-6.37071067811866,-30.5385786437627)) ;
#150444=CARTESIAN_POINT('',(-0.129289321881346,-6.37071067811866,-30.4214213562373)) ;
#150445=CARTESIAN_POINT('',(-0.129289321881346,-6.37071067811866,-30.08)) ;
#150446=CARTESIAN_POINT('',(-0.370710678118655,-6.12928932188134,-30.18)) ;
#150447=CARTESIAN_POINT('',(-0.423570226039551,-6.07642977396045,-30.1271404520791)) ;
#150448=CARTESIAN_POINT('',(-0.370710678118655,-6.12928932188134,-30.78)) ;
#150449=CARTESIAN_POINT('',(-0.370710678118655,-6.12928932188134,-30.08)) ;
#150450=CARTESIAN_POINT('',(-0.156903559372884,-6.34309644062712,-30.5661928812542)) ;
#150451=CARTESIAN_POINT('Origin',(-0.1,-6.4,-30.08)) ;
#150452=CARTESIAN_POINT('',(0.0585786437626908,-6.4,-30.5385786437627)) ;
#150453=CARTESIAN_POINT('',(0.0585786437626908,-6.4,-30.4214213562373)) ;
#150454=CARTESIAN_POINT('',(0.0585786437626908,-6.4,-30.08)) ;
#150455=CARTESIAN_POINT('',(-0.0585786437626908,-6.4,-30.4214213562373)) ;
#150456=CARTESIAN_POINT('',(-0.1,-6.4,-30.4214213562373)) ;
#150457=CARTESIAN_POINT('',(-0.0585786437626908,-6.4,-30.5385786437627)) ;
#150458=CARTESIAN_POINT('',(-0.0585786437626908,-6.4,-30.08)) ;
#150459=CARTESIAN_POINT('',(-0.1,-6.4,-30.5385786437627)) ;
#150460=CARTESIAN_POINT('Origin',(0.1,-6.4,-30.08)) ;
#150461=CARTESIAN_POINT('',(0.370710678118654,-6.12928932188135,-30.78)) ;
#150462=CARTESIAN_POINT('',(0.370710678118655,-6.12928932188134,-30.18)) ;
#150463=CARTESIAN_POINT('',(0.370710678118655,-6.12928932188134,-30.08)) ;
#150464=CARTESIAN_POINT('',(0.129289321881346,-6.37071067811866,-30.4214213562373)) ;
#150465=CARTESIAN_POINT('',(0.223570226039551,-6.27642977396045,-30.3271404520791)) ;
#150466=CARTESIAN_POINT('',(0.129289321881346,-6.37071067811866,-30.5385786437627)) ;
#150467=CARTESIAN_POINT('',(0.129289321881346,-6.37071067811866,-30.08)) ;
#150468=CARTESIAN_POINT('',(-0.0430964406271139,-6.54309644062711,-30.3661928812542)) ;
#150469=CARTESIAN_POINT('Origin',(0.4,-6.1,-30.08)) ;
#150470=CARTESIAN_POINT('',(0.4,-6.05857864376269,-30.18)) ;
#150471=CARTESIAN_POINT('',(0.4,-6.05857864376269,-30.78)) ;
#150472=CARTESIAN_POINT('',(0.4,-6.05857864376269,-30.08)) ;
#150473=CARTESIAN_POINT('',(0.4,-0.6,-30.78)) ;
#150474=CARTESIAN_POINT('',(0.4,-6.1,-30.78)) ;
#150475=CARTESIAN_POINT('',(0.4,-0.6,-30.18)) ;
#150476=CARTESIAN_POINT('',(0.4,-0.6,-30.08)) ;
#150477=CARTESIAN_POINT('',(0.4,-6.05857864376269,-30.18)) ;
#150478=CARTESIAN_POINT('Origin',(0.6,-0.600000000000001,-30.08)) ;
#150479=CARTESIAN_POINT('',(0.3,-6.05857864376269,-30.08)) ;
#150480=CARTESIAN_POINT('',(0.3,-0.6,-30.08)) ;
#150481=CARTESIAN_POINT('',(0.3,-0.6,-30.08)) ;
#150482=CARTESIAN_POINT('Origin',(0.6,-0.6,-30.08)) ;
#150483=CARTESIAN_POINT('',(-0.3,-0.600000000000001,-30.08)) ;
#150484=CARTESIAN_POINT('Origin',(0.6,-0.600000000000001,-30.08)) ;
#150485=CARTESIAN_POINT('',(-0.299999999999994,-6.0585786437627,-30.08)) ;
#150486=CARTESIAN_POINT('',(-0.3,-0.600000000000001,-30.08)) ;
#150487=CARTESIAN_POINT('',(0.4,-6.0585786437627,-30.08)) ;
#150488=CARTESIAN_POINT('Origin',(0.6,-0.600000000000001,-30.88)) ;
#150489=CARTESIAN_POINT('',(-0.299999999999994,-6.0585786437627,-30.88)) ;
#150490=CARTESIAN_POINT('',(-0.3,-0.600000000000001,-30.88)) ;
#150491=CARTESIAN_POINT('',(-0.3,-0.600000000000001,-30.88)) ;
#150492=CARTESIAN_POINT('Origin',(0.6,-0.600000000000001,-30.88)) ;
#150493=CARTESIAN_POINT('',(0.3,-0.6,-30.88)) ;
#150494=CARTESIAN_POINT('Origin',(0.6,-0.6,-30.88)) ;
#150495=CARTESIAN_POINT('',(0.3,-6.05857864376269,-30.88)) ;
#150496=CARTESIAN_POINT('',(0.3,-0.600000000000001,-30.88)) ;
#150497=CARTESIAN_POINT('',(0.6,-6.05857864376269,-30.88)) ;
#150498=CARTESIAN_POINT('Origin',(0.6,-0.600000000000001,-30.08)) ;
#150499=CARTESIAN_POINT('Origin',(0.6,-0.600000000000001,-30.78)) ;
#150500=CARTESIAN_POINT('Origin',(0.6,-0.600000000000001,-30.18)) ;
#150501=CARTESIAN_POINT('Origin',(0.6,-0.6,-30.08)) ;
#150502=CARTESIAN_POINT('Origin',(0.6,-0.6,-30.78)) ;
#150503=CARTESIAN_POINT('Origin',(0.6,-0.6,-30.18)) ;
#150504=CARTESIAN_POINT('Origin',(7.,0.1,-30.08)) ;
#150505=CARTESIAN_POINT('',(6.72928932188135,0.370710678118656,-30.78)) ;
#150506=CARTESIAN_POINT('',(6.72928932188135,0.370710678118655,-30.18)) ;
#150507=CARTESIAN_POINT('',(6.72928932188135,0.370710678118655,-30.08)) ;
#150508=CARTESIAN_POINT('',(6.97071067811866,0.129289321881346,-30.4214213562373)) ;
#150509=CARTESIAN_POINT('',(6.87642977396045,0.22357022603955,-30.3271404520791)) ;
#150510=CARTESIAN_POINT('',(6.97071067811866,0.129289321881346,-30.5385786437627)) ;
#150511=CARTESIAN_POINT('',(6.97071067811866,0.129289321881346,-30.08)) ;
#150512=CARTESIAN_POINT('',(7.14309644062712,-0.0430964406271155,-30.3661928812542)) ;
#150513=CARTESIAN_POINT('Origin',(6.7,0.400000000000001,-30.08)) ;
#150514=CARTESIAN_POINT('',(6.65857864376269,0.400000000000001,-30.18)) ;
#150515=CARTESIAN_POINT('',(6.65857864376269,0.400000000000001,-30.78)) ;
#150516=CARTESIAN_POINT('',(6.65857864376269,0.400000000000001,-30.08)) ;
#150517=CARTESIAN_POINT('',(6.7,0.400000000000001,-30.78)) ;
#150518=CARTESIAN_POINT('',(6.65857864376269,0.400000000000001,-30.18)) ;
#150519=CARTESIAN_POINT('Origin',(0.6,-0.4,-30.08)) ;
#150520=CARTESIAN_POINT('',(6.65857864376269,-0.400000000000001,-30.78)) ;
#150521=CARTESIAN_POINT('',(0.6,-0.4,-30.78)) ;
#150522=CARTESIAN_POINT('',(6.65857864376269,-0.400000000000001,-30.18)) ;
#150523=CARTESIAN_POINT('',(6.65857864376269,-0.400000000000001,-30.08)) ;
#150524=CARTESIAN_POINT('',(2.4,-0.4,-30.18)) ;
#150525=CARTESIAN_POINT('Origin',(6.7,-0.400000000000001,-30.08)) ;
#150526=CARTESIAN_POINT('',(6.97071067811866,-0.129289321881345,-30.5385786437627)) ;
#150527=CARTESIAN_POINT('',(6.97071067811866,-0.129289321881346,-30.4214213562373)) ;
#150528=CARTESIAN_POINT('',(6.97071067811866,-0.129289321881346,-30.08)) ;
#150529=CARTESIAN_POINT('',(6.72928932188135,-0.370710678118655,-30.18)) ;
#150530=CARTESIAN_POINT('',(6.67642977396045,-0.423570226039551,-30.1271404520791)) ;
#150531=CARTESIAN_POINT('',(6.72928932188135,-0.370710678118655,-30.78)) ;
#150532=CARTESIAN_POINT('',(6.72928932188135,-0.370710678118655,-30.08)) ;
#150533=CARTESIAN_POINT('',(6.94309644062712,-0.156903559372885,-30.5661928812542)) ;
#150534=CARTESIAN_POINT('Origin',(7.,-0.1,-30.08)) ;
#150535=CARTESIAN_POINT('',(7.,-0.0585786437626909,-30.4214213562373)) ;
#150536=CARTESIAN_POINT('',(7.,-0.0585786437626909,-30.5385786437627)) ;
#150537=CARTESIAN_POINT('',(7.,-0.0585786437626909,-30.08)) ;
#150538=CARTESIAN_POINT('',(7.,0.0585786437626909,-30.5385786437627)) ;
#150539=CARTESIAN_POINT('',(7.,-0.1,-30.5385786437627)) ;
#150540=CARTESIAN_POINT('',(7.,0.0585786437626909,-30.4214213562373)) ;
#150541=CARTESIAN_POINT('',(7.,0.0585786437626909,-30.08)) ;
#150542=CARTESIAN_POINT('',(7.,-0.1,-30.4214213562373)) ;
#150543=CARTESIAN_POINT('Origin',(0.6,-0.600000000000001,-30.08)) ;
#150544=CARTESIAN_POINT('',(6.65857864376269,-0.300000000000001,-30.08)) ;
#150545=CARTESIAN_POINT('',(6.6585786437627,0.299999999999994,-30.08)) ;
#150546=CARTESIAN_POINT('',(6.6585786437627,-0.399999999999999,-30.08)) ;
#150547=CARTESIAN_POINT('',(2.4,0.3,-30.08)) ;
#150548=CARTESIAN_POINT('',(6.65857864376269,-0.300000000000001,-30.08)) ;
#150549=CARTESIAN_POINT('Origin',(0.6,-0.600000000000001,-30.88)) ;
#150550=CARTESIAN_POINT('',(6.65857864376269,0.299999999999998,-30.88)) ;
#150551=CARTESIAN_POINT('',(0.6,0.299999999999999,-30.88)) ;
#150552=CARTESIAN_POINT('',(6.65857864376269,-0.300000000000001,-30.88)) ;
#150553=CARTESIAN_POINT('',(6.65857864376269,-0.6,-30.88)) ;
#150554=CARTESIAN_POINT('',(0.6,-0.3,-30.88)) ;
#150555=CARTESIAN_POINT('Origin',(-0.4,-0.600000000000001,-33.89)) ;
#150556=CARTESIAN_POINT('',(-0.4,-0.600000000000001,-33.99)) ;
#150557=CARTESIAN_POINT('',(-0.4,-0.600000000000001,-34.59)) ;
#150558=CARTESIAN_POINT('',(-0.4,-0.600000000000001,-33.89)) ;
#150559=CARTESIAN_POINT('',(-0.4,-6.05857864376269,-34.59)) ;
#150560=CARTESIAN_POINT('',(-0.4,-0.600000000000001,-34.59)) ;
#150561=CARTESIAN_POINT('',(-0.4,-6.05857864376269,-33.99)) ;
#150562=CARTESIAN_POINT('',(-0.4,-6.05857864376269,-33.89)) ;
#150563=CARTESIAN_POINT('',(-0.4,-0.600000000000001,-33.99)) ;
#150564=CARTESIAN_POINT('Origin',(-0.4,-6.1,-33.89)) ;
#150565=CARTESIAN_POINT('',(-0.129289321881345,-6.37071067811866,-34.3485786437627)) ;
#150566=CARTESIAN_POINT('',(-0.129289321881346,-6.37071067811866,-34.2314213562373)) ;
#150567=CARTESIAN_POINT('',(-0.129289321881346,-6.37071067811866,-33.89)) ;
#150568=CARTESIAN_POINT('',(-0.370710678118655,-6.12928932188134,-33.99)) ;
#150569=CARTESIAN_POINT('',(-0.423570226039552,-6.07642977396045,-33.9371404520791)) ;
#150570=CARTESIAN_POINT('',(-0.370710678118655,-6.12928932188134,-34.59)) ;
#150571=CARTESIAN_POINT('',(-0.370710678118655,-6.12928932188134,-33.89)) ;
#150572=CARTESIAN_POINT('',(-0.156903559372882,-6.34309644062712,-34.3761928812542)) ;
#150573=CARTESIAN_POINT('Origin',(-0.1,-6.4,-33.89)) ;
#150574=CARTESIAN_POINT('',(0.0585786437626908,-6.4,-34.3485786437627)) ;
#150575=CARTESIAN_POINT('',(0.0585786437626908,-6.4,-34.2314213562373)) ;
#150576=CARTESIAN_POINT('',(0.0585786437626908,-6.4,-33.89)) ;
#150577=CARTESIAN_POINT('',(-0.0585786437626908,-6.4,-34.2314213562373)) ;
#150578=CARTESIAN_POINT('',(-0.1,-6.4,-34.2314213562373)) ;
#150579=CARTESIAN_POINT('',(-0.0585786437626908,-6.4,-34.3485786437627)) ;
#150580=CARTESIAN_POINT('',(-0.0585786437626908,-6.4,-33.89)) ;
#150581=CARTESIAN_POINT('',(-0.1,-6.4,-34.3485786437627)) ;
#150582=CARTESIAN_POINT('Origin',(0.1,-6.4,-33.89)) ;
#150583=CARTESIAN_POINT('',(0.370710678118654,-6.12928932188135,-34.59)) ;
#150584=CARTESIAN_POINT('',(0.370710678118655,-6.12928932188134,-33.99)) ;
#150585=CARTESIAN_POINT('',(0.370710678118655,-6.12928932188134,-33.89)) ;
#150586=CARTESIAN_POINT('',(0.129289321881346,-6.37071067811866,-34.2314213562373)) ;
#150587=CARTESIAN_POINT('',(0.223570226039555,-6.27642977396044,-34.1371404520791)) ;
#150588=CARTESIAN_POINT('',(0.129289321881346,-6.37071067811866,-34.3485786437627)) ;
#150589=CARTESIAN_POINT('',(0.129289321881346,-6.37071067811866,-33.89)) ;
#150590=CARTESIAN_POINT('',(-0.0430964406271177,-6.54309644062712,-34.1761928812542)) ;
#150591=CARTESIAN_POINT('Origin',(0.4,-6.1,-33.89)) ;
#150592=CARTESIAN_POINT('',(0.4,-6.05857864376269,-33.99)) ;
#150593=CARTESIAN_POINT('',(0.4,-6.05857864376269,-34.59)) ;
#150594=CARTESIAN_POINT('',(0.4,-6.05857864376269,-33.89)) ;
#150595=CARTESIAN_POINT('',(0.4,-0.6,-34.59)) ;
#150596=CARTESIAN_POINT('',(0.4,-6.1,-34.59)) ;
#150597=CARTESIAN_POINT('',(0.4,-0.6,-33.99)) ;
#150598=CARTESIAN_POINT('',(0.4,-0.6,-33.89)) ;
#150599=CARTESIAN_POINT('',(0.4,-6.05857864376269,-33.99)) ;
#150600=CARTESIAN_POINT('Origin',(0.6,-0.600000000000001,-33.89)) ;
#150601=CARTESIAN_POINT('',(0.3,-6.05857864376269,-33.89)) ;
#150602=CARTESIAN_POINT('',(0.3,-0.6,-33.89)) ;
#150603=CARTESIAN_POINT('',(0.3,-0.6,-33.89)) ;
#150604=CARTESIAN_POINT('Origin',(0.6,-0.6,-33.89)) ;
#150605=CARTESIAN_POINT('',(-0.3,-0.600000000000001,-33.89)) ;
#150606=CARTESIAN_POINT('Origin',(0.6,-0.600000000000001,-33.89)) ;
#150607=CARTESIAN_POINT('',(-0.300000000000006,-6.05857864376268,-33.89)) ;
#150608=CARTESIAN_POINT('',(-0.3,-0.600000000000001,-33.89)) ;
#150609=CARTESIAN_POINT('',(0.4,-6.05857864376269,-33.89)) ;
#150610=CARTESIAN_POINT('Origin',(0.6,-0.600000000000001,-34.69)) ;
#150611=CARTESIAN_POINT('',(-0.299999999999998,-6.05857864376269,-34.69)) ;
#150612=CARTESIAN_POINT('',(-0.3,-0.600000000000001,-34.69)) ;
#150613=CARTESIAN_POINT('',(-0.3,-0.600000000000001,-34.69)) ;
#150614=CARTESIAN_POINT('Origin',(0.6,-0.600000000000001,-34.69)) ;
#150615=CARTESIAN_POINT('',(0.3,-0.6,-34.69)) ;
#150616=CARTESIAN_POINT('Origin',(0.6,-0.6,-34.69)) ;
#150617=CARTESIAN_POINT('',(0.3,-6.05857864376269,-34.69)) ;
#150618=CARTESIAN_POINT('',(0.3,-0.600000000000001,-34.69)) ;
#150619=CARTESIAN_POINT('',(0.6,-6.05857864376269,-34.69)) ;
#150620=CARTESIAN_POINT('Origin',(0.6,-0.600000000000001,-33.89)) ;
#150621=CARTESIAN_POINT('Origin',(0.6,-0.600000000000001,-34.59)) ;
#150622=CARTESIAN_POINT('Origin',(0.6,-0.600000000000001,-33.99)) ;
#150623=CARTESIAN_POINT('Origin',(0.6,-0.6,-33.89)) ;
#150624=CARTESIAN_POINT('Origin',(0.6,-0.6,-34.59)) ;
#150625=CARTESIAN_POINT('Origin',(0.6,-0.6,-33.99)) ;
#150626=CARTESIAN_POINT('Origin',(7.,0.1,-33.89)) ;
#150627=CARTESIAN_POINT('',(6.72928932188135,0.370710678118655,-34.59)) ;
#150628=CARTESIAN_POINT('',(6.72928932188135,0.370710678118655,-33.99)) ;
#150629=CARTESIAN_POINT('',(6.72928932188135,0.370710678118655,-33.89)) ;
#150630=CARTESIAN_POINT('',(6.97071067811866,0.129289321881346,-34.2314213562373)) ;
#150631=CARTESIAN_POINT('',(6.87642977396044,0.223570226039555,-34.1371404520791)) ;
#150632=CARTESIAN_POINT('',(6.97071067811866,0.129289321881346,-34.3485786437627)) ;
#150633=CARTESIAN_POINT('',(6.97071067811866,0.129289321881346,-33.89)) ;
#150634=CARTESIAN_POINT('',(7.14309644062712,-0.0430964406271179,-34.1761928812542)) ;
#150635=CARTESIAN_POINT('Origin',(6.7,0.400000000000001,-33.89)) ;
#150636=CARTESIAN_POINT('',(6.65857864376269,0.400000000000001,-33.99)) ;
#150637=CARTESIAN_POINT('',(6.65857864376269,0.400000000000001,-34.59)) ;
#150638=CARTESIAN_POINT('',(6.65857864376269,0.400000000000001,-33.89)) ;
#150639=CARTESIAN_POINT('',(6.7,0.400000000000001,-34.59)) ;
#150640=CARTESIAN_POINT('',(6.65857864376269,0.400000000000001,-33.99)) ;
#150641=CARTESIAN_POINT('Origin',(0.6,-0.4,-33.89)) ;
#150642=CARTESIAN_POINT('',(6.65857864376269,-0.400000000000001,-34.59)) ;
#150643=CARTESIAN_POINT('',(0.6,-0.4,-34.59)) ;
#150644=CARTESIAN_POINT('',(6.65857864376269,-0.400000000000001,-33.99)) ;
#150645=CARTESIAN_POINT('',(6.65857864376269,-0.400000000000001,-33.89)) ;
#150646=CARTESIAN_POINT('',(2.4,-0.4,-33.99)) ;
#150647=CARTESIAN_POINT('Origin',(6.7,-0.400000000000001,-33.89)) ;
#150648=CARTESIAN_POINT('',(6.97071067811866,-0.129289321881345,-34.3485786437627)) ;
#150649=CARTESIAN_POINT('',(6.97071067811866,-0.129289321881346,-34.2314213562373)) ;
#150650=CARTESIAN_POINT('',(6.97071067811866,-0.129289321881346,-33.89)) ;
#150651=CARTESIAN_POINT('',(6.72928932188135,-0.370710678118655,-33.99)) ;
#150652=CARTESIAN_POINT('',(6.67642977396045,-0.423570226039555,-33.9371404520791)) ;
#150653=CARTESIAN_POINT('',(6.72928932188135,-0.370710678118655,-34.59)) ;
#150654=CARTESIAN_POINT('',(6.72928932188135,-0.370710678118655,-33.89)) ;
#150655=CARTESIAN_POINT('',(6.94309644062712,-0.156903559372885,-34.3761928812542)) ;
#150656=CARTESIAN_POINT('Origin',(7.,-0.1,-33.89)) ;
#150657=CARTESIAN_POINT('',(7.,-0.0585786437626909,-34.2314213562373)) ;
#150658=CARTESIAN_POINT('',(7.,-0.0585786437626909,-34.3485786437627)) ;
#150659=CARTESIAN_POINT('',(7.,-0.0585786437626909,-33.89)) ;
#150660=CARTESIAN_POINT('',(7.,0.0585786437626909,-34.3485786437627)) ;
#150661=CARTESIAN_POINT('',(7.,-0.1,-34.3485786437627)) ;
#150662=CARTESIAN_POINT('',(7.,0.0585786437626909,-34.2314213562373)) ;
#150663=CARTESIAN_POINT('',(7.,0.0585786437626909,-33.89)) ;
#150664=CARTESIAN_POINT('',(7.,-0.1,-34.2314213562373)) ;
#150665=CARTESIAN_POINT('Origin',(0.6,-0.600000000000001,-33.89)) ;
#150666=CARTESIAN_POINT('',(6.65857864376269,-0.300000000000001,-33.89)) ;
#150667=CARTESIAN_POINT('',(6.65857864376269,0.300000000000007,-33.89)) ;
#150668=CARTESIAN_POINT('',(6.65857864376269,-0.399999999999999,-33.89)) ;
#150669=CARTESIAN_POINT('',(2.4,0.3,-33.89)) ;
#150670=CARTESIAN_POINT('',(6.65857864376269,-0.300000000000001,-33.89)) ;
#150671=CARTESIAN_POINT('Origin',(0.6,-0.600000000000001,-34.69)) ;
#150672=CARTESIAN_POINT('',(6.65857864376269,0.3,-34.69)) ;
#150673=CARTESIAN_POINT('',(0.6,0.299999999999999,-34.69)) ;
#150674=CARTESIAN_POINT('',(6.65857864376269,-0.300000000000001,-34.69)) ;
#150675=CARTESIAN_POINT('',(6.6585786437627,-0.6,-34.69)) ;
#150676=CARTESIAN_POINT('',(0.6,-0.3,-34.69)) ;
#150677=CARTESIAN_POINT('Origin',(0.4,-6.4,-34.39)) ;
#150678=CARTESIAN_POINT('',(-0.0585786437626895,-6.37071067811866,-34.4192893218813)) ;
#150679=CARTESIAN_POINT('',(-0.299999999999997,-6.12928932188135,-34.6607106781186)) ;
#150680=CARTESIAN_POINT('',(0.113807118745769,-6.54309644062712,-34.2469035593729)) ;
#150681=CARTESIAN_POINT('',(0.299999999999999,-6.12928932188134,-34.6607106781187)) ;
#150682=CARTESIAN_POINT('',(0.4,-6.12928932188135,-34.6607106781186)) ;
#150683=CARTESIAN_POINT('',(0.0585786437626844,-6.37071067811866,-34.4192893218813)) ;
#150684=CARTESIAN_POINT('',(0.152859547920894,-6.27642977396045,-34.5135702260395)) ;
#150685=CARTESIAN_POINT('',(0.4,-6.37071067811866,-34.4192893218813)) ;
#150686=CARTESIAN_POINT('Origin',(0.4,-6.1,-33.89)) ;
#150687=CARTESIAN_POINT('',(0.058578643762689,-6.37071067811866,-34.1607106781187)) ;
#150688=CARTESIAN_POINT('',(0.300000000000011,-6.12928932188133,-33.9192893218813)) ;
#150689=CARTESIAN_POINT('',(0.352859547920897,-6.07642977396045,-33.8664297739605)) ;
#150690=CARTESIAN_POINT('',(-0.300000000000007,-6.12928932188133,-33.9192893218813)) ;
#150691=CARTESIAN_POINT('',(0.4,-6.12928932188134,-33.9192893218814)) ;
#150692=CARTESIAN_POINT('',(-0.0585786437626846,-6.37071067811866,-34.1607106781187)) ;
#150693=CARTESIAN_POINT('',(-0.0861928812542284,-6.34309644062711,-34.1330964406271)) ;
#150694=CARTESIAN_POINT('',(0.4,-6.37071067811866,-34.1607106781187)) ;
#150695=CARTESIAN_POINT('Origin',(0.4,-6.4,-30.58)) ;
#150696=CARTESIAN_POINT('',(-0.0585786437626899,-6.37071067811865,-30.6092893218813)) ;
#150697=CARTESIAN_POINT('',(-0.299999999999994,-6.12928932188135,-30.8507106781187)) ;
#150698=CARTESIAN_POINT('',(0.11380711874577,-6.54309644062711,-30.4369035593729)) ;
#150699=CARTESIAN_POINT('',(0.299999999999999,-6.12928932188135,-30.8507106781187)) ;
#150700=CARTESIAN_POINT('',(0.4,-6.12928932188134,-30.8507106781187)) ;
#150701=CARTESIAN_POINT('',(0.058578643762692,-6.37071067811865,-30.6092893218813)) ;
#150702=CARTESIAN_POINT('',(0.152859547920897,-6.27642977396045,-30.7035702260396)) ;
#150703=CARTESIAN_POINT('',(0.4,-6.37071067811865,-30.6092893218813)) ;
#150704=CARTESIAN_POINT('Origin',(0.4,-6.1,-30.08)) ;
#150705=CARTESIAN_POINT('',(0.0585786437626916,-6.37071067811865,-30.3507106781187)) ;
#150706=CARTESIAN_POINT('',(0.299999999999992,-6.12928932188135,-30.1092893218814)) ;
#150707=CARTESIAN_POINT('',(0.352859547920897,-6.07642977396045,-30.0564297739604)) ;
#150708=CARTESIAN_POINT('',(-0.299999999999994,-6.12928932188135,-30.1092893218814)) ;
#150709=CARTESIAN_POINT('',(0.4,-6.12928932188135,-30.1092893218813)) ;
#150710=CARTESIAN_POINT('',(-0.0585786437626909,-6.37071067811865,-30.3507106781187)) ;
#150711=CARTESIAN_POINT('',(-0.0861928812542305,-6.34309644062712,-30.3230964406271)) ;
#150712=CARTESIAN_POINT('',(0.4,-6.37071067811865,-30.3507106781187)) ;
#150713=CARTESIAN_POINT('Origin',(0.4,-6.4,-26.77)) ;
#150714=CARTESIAN_POINT('',(-0.0585786437626899,-6.37071067811865,-26.7992893218813)) ;
#150715=CARTESIAN_POINT('',(-0.299999999999994,-6.12928932188135,-27.0407106781187)) ;
#150716=CARTESIAN_POINT('',(0.11380711874577,-6.54309644062711,-26.6269035593729)) ;
#150717=CARTESIAN_POINT('',(0.299999999999999,-6.12928932188135,-27.0407106781187)) ;
#150718=CARTESIAN_POINT('',(0.4,-6.12928932188134,-27.0407106781187)) ;
#150719=CARTESIAN_POINT('',(0.058578643762692,-6.37071067811865,-26.7992893218813)) ;
#150720=CARTESIAN_POINT('',(0.152859547920897,-6.27642977396045,-26.8935702260396)) ;
#150721=CARTESIAN_POINT('',(0.4,-6.37071067811865,-26.7992893218813)) ;
#150722=CARTESIAN_POINT('Origin',(0.4,-6.1,-26.27)) ;
#150723=CARTESIAN_POINT('',(0.0585786437626916,-6.37071067811865,-26.5407106781187)) ;
#150724=CARTESIAN_POINT('',(0.299999999999992,-6.12928932188135,-26.2992893218814)) ;
#150725=CARTESIAN_POINT('',(0.352859547920897,-6.07642977396045,-26.2464297739604)) ;
#150726=CARTESIAN_POINT('',(-0.299999999999994,-6.12928932188135,-26.2992893218814)) ;
#150727=CARTESIAN_POINT('',(0.4,-6.12928932188135,-26.2992893218813)) ;
#150728=CARTESIAN_POINT('',(-0.0585786437626909,-6.37071067811865,-26.5407106781187)) ;
#150729=CARTESIAN_POINT('',(-0.0861928812542305,-6.34309644062712,-26.5130964406271)) ;
#150730=CARTESIAN_POINT('',(0.4,-6.37071067811865,-26.5407106781187)) ;
#150731=CARTESIAN_POINT('Origin',(0.4,-6.4,-22.96)) ;
#150732=CARTESIAN_POINT('',(-0.0585786437626899,-6.37071067811865,-22.9892893218813)) ;
#150733=CARTESIAN_POINT('',(-0.299999999999994,-6.12928932188135,-23.2307106781187)) ;
#150734=CARTESIAN_POINT('',(0.11380711874577,-6.54309644062711,-22.8169035593729)) ;
#150735=CARTESIAN_POINT('',(0.299999999999999,-6.12928932188135,-23.2307106781187)) ;
#150736=CARTESIAN_POINT('',(0.4,-6.12928932188134,-23.2307106781187)) ;
#150737=CARTESIAN_POINT('',(0.058578643762692,-6.37071067811865,-22.9892893218813)) ;
#150738=CARTESIAN_POINT('',(0.152859547920897,-6.27642977396045,-23.0835702260395)) ;
#150739=CARTESIAN_POINT('',(0.4,-6.37071067811865,-22.9892893218813)) ;
#150740=CARTESIAN_POINT('Origin',(0.4,-6.1,-22.46)) ;
#150741=CARTESIAN_POINT('',(0.0585786437626916,-6.37071067811865,-22.7307106781187)) ;
#150742=CARTESIAN_POINT('',(0.299999999999992,-6.12928932188135,-22.4892893218814)) ;
#150743=CARTESIAN_POINT('',(0.352859547920897,-6.07642977396045,-22.4364297739604)) ;
#150744=CARTESIAN_POINT('',(-0.299999999999994,-6.12928932188135,-22.4892893218814)) ;
#150745=CARTESIAN_POINT('',(0.4,-6.12928932188135,-22.4892893218814)) ;
#150746=CARTESIAN_POINT('',(-0.0585786437626909,-6.37071067811865,-22.7307106781187)) ;
#150747=CARTESIAN_POINT('',(-0.0861928812542305,-6.34309644062712,-22.7030964406271)) ;
#150748=CARTESIAN_POINT('',(0.4,-6.37071067811865,-22.7307106781187)) ;
#150749=CARTESIAN_POINT('Origin',(0.4,-6.4,-19.15)) ;
#150750=CARTESIAN_POINT('',(-0.0585786437626899,-6.37071067811865,-19.1792893218813)) ;
#150751=CARTESIAN_POINT('',(-0.299999999999994,-6.12928932188135,-19.4207106781187)) ;
#150752=CARTESIAN_POINT('',(0.11380711874577,-6.54309644062711,-19.0069035593729)) ;
#150753=CARTESIAN_POINT('',(0.299999999999999,-6.12928932188135,-19.4207106781187)) ;
#150754=CARTESIAN_POINT('',(0.4,-6.12928932188134,-19.4207106781187)) ;
#150755=CARTESIAN_POINT('',(0.058578643762692,-6.37071067811865,-19.1792893218813)) ;
#150756=CARTESIAN_POINT('',(0.152859547920897,-6.27642977396045,-19.2735702260396)) ;
#150757=CARTESIAN_POINT('',(0.4,-6.37071067811865,-19.1792893218813)) ;
#150758=CARTESIAN_POINT('Origin',(0.4,-6.1,-18.65)) ;
#150759=CARTESIAN_POINT('',(0.0585786437626916,-6.37071067811865,-18.9207106781187)) ;
#150760=CARTESIAN_POINT('',(0.299999999999992,-6.12928932188135,-18.6792893218814)) ;
#150761=CARTESIAN_POINT('',(0.352859547920897,-6.07642977396045,-18.6264297739605)) ;
#150762=CARTESIAN_POINT('',(-0.299999999999994,-6.12928932188135,-18.6792893218814)) ;
#150763=CARTESIAN_POINT('',(0.4,-6.12928932188135,-18.6792893218813)) ;
#150764=CARTESIAN_POINT('',(-0.0585786437626909,-6.37071067811865,-18.9207106781187)) ;
#150765=CARTESIAN_POINT('',(-0.0861928812542305,-6.34309644062712,-18.8930964406271)) ;
#150766=CARTESIAN_POINT('',(0.4,-6.37071067811865,-18.9207106781187)) ;
#150767=CARTESIAN_POINT('Origin',(0.4,-6.4,-15.34)) ;
#150768=CARTESIAN_POINT('',(-0.0585786437626904,-6.37071067811866,-15.3692893218813)) ;
#150769=CARTESIAN_POINT('',(-0.299999999999999,-6.12928932188134,-15.6107106781187)) ;
#150770=CARTESIAN_POINT('',(0.11380711874577,-6.54309644062711,-15.1969035593729)) ;
#150771=CARTESIAN_POINT('',(0.3,-6.12928932188134,-15.6107106781187)) ;
#150772=CARTESIAN_POINT('',(0.4,-6.12928932188134,-15.6107106781187)) ;
#150773=CARTESIAN_POINT('',(0.0585786437626911,-6.37071067811866,-15.3692893218813)) ;
#150774=CARTESIAN_POINT('',(0.152859547920897,-6.27642977396045,-15.4635702260396)) ;
#150775=CARTESIAN_POINT('',(0.4,-6.37071067811866,-15.3692893218813)) ;
#150776=CARTESIAN_POINT('Origin',(0.4,-6.1,-14.84)) ;
#150777=CARTESIAN_POINT('',(0.0585786437626904,-6.37071067811866,-15.1107106781187)) ;
#150778=CARTESIAN_POINT('',(0.299999999999999,-6.12928932188135,-14.8692893218813)) ;
#150779=CARTESIAN_POINT('',(0.352859547920896,-6.07642977396045,-14.8164297739604)) ;
#150780=CARTESIAN_POINT('',(-0.300000000000001,-6.12928932188134,-14.8692893218813)) ;
#150781=CARTESIAN_POINT('',(0.4,-6.12928932188134,-14.8692893218813)) ;
#150782=CARTESIAN_POINT('',(-0.0585786437626914,-6.37071067811866,-15.1107106781187)) ;
#150783=CARTESIAN_POINT('',(-0.0861928812542312,-6.34309644062712,-15.0830964406271)) ;
#150784=CARTESIAN_POINT('',(0.4,-6.37071067811866,-15.1107106781187)) ;
#150785=CARTESIAN_POINT('Origin',(0.4,-6.4,-11.53)) ;
#150786=CARTESIAN_POINT('',(-0.0585786437626916,-6.37071067811866,-11.5592893218813)) ;
#150787=CARTESIAN_POINT('',(-0.3,-6.12928932188135,-11.8007106781187)) ;
#150788=CARTESIAN_POINT('',(0.113807118745769,-6.54309644062712,-11.3869035593729)) ;
#150789=CARTESIAN_POINT('',(0.299999999999998,-6.12928932188135,-11.8007106781187)) ;
#150790=CARTESIAN_POINT('',(0.4,-6.12928932188134,-11.8007106781187)) ;
#150791=CARTESIAN_POINT('',(0.0585786437626907,-6.37071067811866,-11.5592893218813)) ;
#150792=CARTESIAN_POINT('',(0.152859547920896,-6.27642977396045,-11.6535702260396)) ;
#150793=CARTESIAN_POINT('',(0.4,-6.37071067811866,-11.5592893218813)) ;
#150794=CARTESIAN_POINT('Origin',(0.4,-6.1,-11.03)) ;
#150795=CARTESIAN_POINT('',(0.0585786437626913,-6.37071067811866,-11.3007106781187)) ;
#150796=CARTESIAN_POINT('',(0.300000000000001,-6.12928932188134,-11.0592893218813)) ;
#150797=CARTESIAN_POINT('',(0.352859547920897,-6.07642977396045,-11.0064297739604)) ;
#150798=CARTESIAN_POINT('',(-0.300000000000003,-6.12928932188134,-11.0592893218813)) ;
#150799=CARTESIAN_POINT('',(0.4,-6.12928932188134,-11.0592893218813)) ;
#150800=CARTESIAN_POINT('',(-0.0585786437626915,-6.37071067811866,-11.3007106781187)) ;
#150801=CARTESIAN_POINT('',(-0.0861928812542312,-6.34309644062712,-11.2730964406271)) ;
#150802=CARTESIAN_POINT('',(0.4,-6.37071067811866,-11.3007106781187)) ;
#150803=CARTESIAN_POINT('Origin',(0.4,-6.4,-7.72)) ;
#150804=CARTESIAN_POINT('',(-0.0585786437626906,-6.37071067811866,-7.74928932188134)) ;
#150805=CARTESIAN_POINT('',(-0.299999999999999,-6.12928932188134,-7.99071067811865)) ;
#150806=CARTESIAN_POINT('',(0.113807118745769,-6.54309644062711,-7.57690355937288)) ;
#150807=CARTESIAN_POINT('',(0.3,-6.12928932188134,-7.99071067811865)) ;
#150808=CARTESIAN_POINT('',(0.4,-6.12928932188134,-7.99071067811866)) ;
#150809=CARTESIAN_POINT('',(0.0585786437626912,-6.37071067811866,-7.74928932188134)) ;
#150810=CARTESIAN_POINT('',(0.152859547920897,-6.27642977396045,-7.84357022603955)) ;
#150811=CARTESIAN_POINT('',(0.4,-6.37071067811866,-7.74928932188134)) ;
#150812=CARTESIAN_POINT('Origin',(0.4,-6.1,-7.22)) ;
#150813=CARTESIAN_POINT('',(0.0585786437626908,-6.37071067811866,-7.49071067811866)) ;
#150814=CARTESIAN_POINT('',(0.300000000000002,-6.12928932188134,-7.24928932188134)) ;
#150815=CARTESIAN_POINT('',(0.352859547920897,-6.07642977396045,-7.19642977396045)) ;
#150816=CARTESIAN_POINT('',(-0.300000000000001,-6.12928932188134,-7.24928932188134)) ;
#150817=CARTESIAN_POINT('',(0.4,-6.12928932188134,-7.24928932188134)) ;
#150818=CARTESIAN_POINT('',(-0.0585786437626907,-6.37071067811866,-7.49071067811866)) ;
#150819=CARTESIAN_POINT('',(-0.0861928812542307,-6.34309644062712,-7.46309644062712)) ;
#150820=CARTESIAN_POINT('',(0.4,-6.37071067811866,-7.49071067811866)) ;
#150821=CARTESIAN_POINT('Origin',(0.4,-6.4,-3.91)) ;
#150822=CARTESIAN_POINT('',(-0.0585786437626904,-6.37071067811866,-3.93928932188134)) ;
#150823=CARTESIAN_POINT('',(-0.300000000000001,-6.12928932188134,-4.18071067811866)) ;
#150824=CARTESIAN_POINT('',(0.11380711874577,-6.54309644062711,-3.76690355937288)) ;
#150825=CARTESIAN_POINT('',(0.300000000000001,-6.12928932188134,-4.18071067811866)) ;
#150826=CARTESIAN_POINT('',(0.4,-6.12928932188134,-4.18071067811865)) ;
#150827=CARTESIAN_POINT('',(0.0585786437626911,-6.37071067811866,-3.93928932188134)) ;
#150828=CARTESIAN_POINT('',(0.152859547920897,-6.27642977396045,-4.03357022603955)) ;
#150829=CARTESIAN_POINT('',(0.4,-6.37071067811866,-3.93928932188134)) ;
#150830=CARTESIAN_POINT('Origin',(0.4,-6.1,-3.41)) ;
#150831=CARTESIAN_POINT('',(0.0585786437626907,-6.37071067811866,-3.68071067811866)) ;
#150832=CARTESIAN_POINT('',(0.299999999999999,-6.12928932188135,-3.43928932188135)) ;
#150833=CARTESIAN_POINT('',(0.352859547920897,-6.07642977396045,-3.38642977396045)) ;
#150834=CARTESIAN_POINT('',(-0.299999999999999,-6.12928932188135,-3.43928932188135)) ;
#150835=CARTESIAN_POINT('',(0.4,-6.12928932188134,-3.43928932188135)) ;
#150836=CARTESIAN_POINT('',(-0.0585786437626909,-6.37071067811866,-3.68071067811866)) ;
#150837=CARTESIAN_POINT('',(-0.086192881254231,-6.34309644062712,-3.65309644062712)) ;
#150838=CARTESIAN_POINT('',(0.4,-6.37071067811866,-3.68071067811866)) ;
#150839=CARTESIAN_POINT('Origin',(6.7,-0.399999999999999,-34.69)) ;
#150840=CARTESIAN_POINT('',(6.97071067811865,-0.0585786437626952,-34.4192893218813)) ;
#150841=CARTESIAN_POINT('',(6.72928932188135,-0.300000000000001,-34.6607106781186)) ;
#150842=CARTESIAN_POINT('',(6.67642977396045,-0.352859547920898,-34.7135702260396)) ;
#150843=CARTESIAN_POINT('',(6.72928932188134,0.3,-34.6607106781187)) ;
#150844=CARTESIAN_POINT('',(6.72928932188135,-0.399999999999999,-34.6607106781186)) ;
#150845=CARTESIAN_POINT('',(6.97071067811865,0.0585786437626901,-34.4192893218813)) ;
#150846=CARTESIAN_POINT('',(6.94309644062711,0.0861928812542281,-34.4469035593729)) ;
#150847=CARTESIAN_POINT('',(6.97071067811865,-0.4,-34.4192893218813)) ;
#150848=CARTESIAN_POINT('Origin',(7.,-0.399999999999999,-34.19)) ;
#150849=CARTESIAN_POINT('',(6.97071067811866,0.0585786437626919,-34.1607106781187)) ;
#150850=CARTESIAN_POINT('',(6.72928932188134,0.300000000000006,-33.9192893218814)) ;
#150851=CARTESIAN_POINT('',(7.14309644062712,-0.113807118745768,-34.3330964406271)) ;
#150852=CARTESIAN_POINT('',(6.72928932188134,-0.300000000000007,-33.9192893218813)) ;
#150853=CARTESIAN_POINT('',(6.72928932188134,-0.399999999999999,-33.9192893218814)) ;
#150854=CARTESIAN_POINT('',(6.97071067811866,-0.058578643762684,-34.1607106781187)) ;
#150855=CARTESIAN_POINT('',(6.87642977396045,-0.152859547920894,-34.0664297739605)) ;
#150856=CARTESIAN_POINT('',(6.97071067811866,-0.399999999999999,-34.1607106781187)) ;
#150857=CARTESIAN_POINT('Origin',(6.7,-0.399999999999999,-30.88)) ;
#150858=CARTESIAN_POINT('',(6.97071067811866,-0.0585786437626901,-30.6092893218813)) ;
#150859=CARTESIAN_POINT('',(6.72928932188135,-0.299999999999997,-30.8507106781187)) ;
#150860=CARTESIAN_POINT('',(6.67642977396045,-0.352859547920897,-30.9035702260396)) ;
#150861=CARTESIAN_POINT('',(6.72928932188135,0.299999999999998,-30.8507106781187)) ;
#150862=CARTESIAN_POINT('',(6.72928932188135,-0.399999999999999,-30.8507106781187)) ;
#150863=CARTESIAN_POINT('',(6.97071067811866,0.0585786437626903,-30.6092893218813)) ;
#150864=CARTESIAN_POINT('',(6.94309644062712,0.0861928812542301,-30.6369035593729)) ;
#150865=CARTESIAN_POINT('',(6.97071067811866,-0.4,-30.6092893218813)) ;
#150866=CARTESIAN_POINT('Origin',(7.,-0.399999999999999,-30.38)) ;
#150867=CARTESIAN_POINT('',(6.97071067811865,0.058578643762691,-30.3507106781187)) ;
#150868=CARTESIAN_POINT('',(6.72928932188135,0.299999999999994,-30.1092893218813)) ;
#150869=CARTESIAN_POINT('',(7.14309644062712,-0.11380711874577,-30.5230964406271)) ;
#150870=CARTESIAN_POINT('',(6.72928932188135,-0.299999999999999,-30.1092893218813)) ;
#150871=CARTESIAN_POINT('',(6.72928932188135,-0.399999999999999,-30.1092893218813)) ;
#150872=CARTESIAN_POINT('',(6.97071067811865,-0.0585786437626907,-30.3507106781187)) ;
#150873=CARTESIAN_POINT('',(6.87642977396045,-0.152859547920896,-30.2564297739604)) ;
#150874=CARTESIAN_POINT('',(6.97071067811865,-0.399999999999999,-30.3507106781187)) ;
#150875=CARTESIAN_POINT('Origin',(6.7,-0.399999999999999,-27.07)) ;
#150876=CARTESIAN_POINT('',(6.97071067811866,-0.0585786437626901,-26.7992893218813)) ;
#150877=CARTESIAN_POINT('',(6.72928932188135,-0.299999999999997,-27.0407106781187)) ;
#150878=CARTESIAN_POINT('',(6.67642977396045,-0.352859547920897,-27.0935702260396)) ;
#150879=CARTESIAN_POINT('',(6.72928932188135,0.299999999999998,-27.0407106781187)) ;
#150880=CARTESIAN_POINT('',(6.72928932188135,-0.399999999999999,-27.0407106781187)) ;
#150881=CARTESIAN_POINT('',(6.97071067811866,0.0585786437626903,-26.7992893218813)) ;
#150882=CARTESIAN_POINT('',(6.94309644062712,0.0861928812542301,-26.8269035593729)) ;
#150883=CARTESIAN_POINT('',(6.97071067811866,-0.4,-26.7992893218813)) ;
#150884=CARTESIAN_POINT('Origin',(7.,-0.399999999999999,-26.57)) ;
#150885=CARTESIAN_POINT('',(6.97071067811865,0.058578643762691,-26.5407106781187)) ;
#150886=CARTESIAN_POINT('',(6.72928932188135,0.299999999999994,-26.2992893218813)) ;
#150887=CARTESIAN_POINT('',(7.14309644062712,-0.11380711874577,-26.7130964406271)) ;
#150888=CARTESIAN_POINT('',(6.72928932188135,-0.299999999999999,-26.2992893218813)) ;
#150889=CARTESIAN_POINT('',(6.72928932188135,-0.399999999999999,-26.2992893218813)) ;
#150890=CARTESIAN_POINT('',(6.97071067811865,-0.0585786437626907,-26.5407106781187)) ;
#150891=CARTESIAN_POINT('',(6.87642977396045,-0.152859547920896,-26.4464297739605)) ;
#150892=CARTESIAN_POINT('',(6.97071067811865,-0.399999999999999,-26.5407106781187)) ;
#150893=CARTESIAN_POINT('Origin',(6.7,-0.399999999999999,-23.26)) ;
#150894=CARTESIAN_POINT('',(6.97071067811866,-0.0585786437626901,-22.9892893218813)) ;
#150895=CARTESIAN_POINT('',(6.72928932188135,-0.299999999999997,-23.2307106781187)) ;
#150896=CARTESIAN_POINT('',(6.67642977396045,-0.352859547920897,-23.2835702260396)) ;
#150897=CARTESIAN_POINT('',(6.72928932188135,0.299999999999998,-23.2307106781187)) ;
#150898=CARTESIAN_POINT('',(6.72928932188135,-0.399999999999999,-23.2307106781187)) ;
#150899=CARTESIAN_POINT('',(6.97071067811866,0.0585786437626903,-22.9892893218813)) ;
#150900=CARTESIAN_POINT('',(6.94309644062712,0.0861928812542301,-23.0169035593729)) ;
#150901=CARTESIAN_POINT('',(6.97071067811866,-0.4,-22.9892893218813)) ;
#150902=CARTESIAN_POINT('Origin',(7.,-0.399999999999999,-22.76)) ;
#150903=CARTESIAN_POINT('',(6.97071067811865,0.058578643762691,-22.7307106781187)) ;
#150904=CARTESIAN_POINT('',(6.72928932188135,0.299999999999994,-22.4892893218814)) ;
#150905=CARTESIAN_POINT('',(7.14309644062712,-0.11380711874577,-22.9030964406271)) ;
#150906=CARTESIAN_POINT('',(6.72928932188135,-0.299999999999999,-22.4892893218813)) ;
#150907=CARTESIAN_POINT('',(6.72928932188135,-0.399999999999999,-22.4892893218814)) ;
#150908=CARTESIAN_POINT('',(6.97071067811865,-0.0585786437626907,-22.7307106781187)) ;
#150909=CARTESIAN_POINT('',(6.87642977396045,-0.152859547920896,-22.6364297739605)) ;
#150910=CARTESIAN_POINT('',(6.97071067811865,-0.399999999999999,-22.7307106781187)) ;
#150911=CARTESIAN_POINT('Origin',(6.7,-0.399999999999999,-19.45)) ;
#150912=CARTESIAN_POINT('',(6.97071067811866,-0.0585786437626901,-19.1792893218813)) ;
#150913=CARTESIAN_POINT('',(6.72928932188135,-0.299999999999997,-19.4207106781187)) ;
#150914=CARTESIAN_POINT('',(6.67642977396045,-0.352859547920897,-19.4735702260396)) ;
#150915=CARTESIAN_POINT('',(6.72928932188135,0.299999999999998,-19.4207106781187)) ;
#150916=CARTESIAN_POINT('',(6.72928932188135,-0.399999999999999,-19.4207106781187)) ;
#150917=CARTESIAN_POINT('',(6.97071067811866,0.0585786437626903,-19.1792893218813)) ;
#150918=CARTESIAN_POINT('',(6.94309644062712,0.0861928812542301,-19.2069035593729)) ;
#150919=CARTESIAN_POINT('',(6.97071067811866,-0.4,-19.1792893218813)) ;
#150920=CARTESIAN_POINT('Origin',(7.,-0.399999999999999,-18.95)) ;
#150921=CARTESIAN_POINT('',(6.97071067811865,0.058578643762691,-18.9207106781187)) ;
#150922=CARTESIAN_POINT('',(6.72928932188135,0.299999999999992,-18.6792893218814)) ;
#150923=CARTESIAN_POINT('',(7.14309644062712,-0.11380711874577,-19.0930964406271)) ;
#150924=CARTESIAN_POINT('',(6.72928932188135,-0.299999999999999,-18.6792893218813)) ;
#150925=CARTESIAN_POINT('',(6.72928932188135,-0.399999999999999,-18.6792893218813)) ;
#150926=CARTESIAN_POINT('',(6.97071067811865,-0.0585786437626907,-18.9207106781187)) ;
#150927=CARTESIAN_POINT('',(6.87642977396045,-0.152859547920896,-18.8264297739604)) ;
#150928=CARTESIAN_POINT('',(6.97071067811865,-0.399999999999999,-18.9207106781187)) ;
#150929=CARTESIAN_POINT('Origin',(6.7,-0.399999999999999,-15.64)) ;
#150930=CARTESIAN_POINT('',(6.97071067811866,-0.058578643762691,-15.3692893218813)) ;
#150931=CARTESIAN_POINT('',(6.72928932188135,-0.299999999999999,-15.6107106781187)) ;
#150932=CARTESIAN_POINT('',(6.67642977396045,-0.352859547920897,-15.6635702260396)) ;
#150933=CARTESIAN_POINT('',(6.72928932188134,0.300000000000003,-15.6107106781187)) ;
#150934=CARTESIAN_POINT('',(6.72928932188135,-0.399999999999999,-15.6107106781187)) ;
#150935=CARTESIAN_POINT('',(6.97071067811866,0.0585786437626913,-15.3692893218813)) ;
#150936=CARTESIAN_POINT('',(6.94309644062712,0.086192881254231,-15.3969035593729)) ;
#150937=CARTESIAN_POINT('',(6.97071067811866,-0.4,-15.3692893218813)) ;
#150938=CARTESIAN_POINT('Origin',(7.,-0.399999999999999,-15.14)) ;
#150939=CARTESIAN_POINT('',(6.97071067811865,0.0585786437626917,-15.1107106781187)) ;
#150940=CARTESIAN_POINT('',(6.72928932188135,0.3,-14.8692893218813)) ;
#150941=CARTESIAN_POINT('',(7.14309644062712,-0.11380711874577,-15.2830964406271)) ;
#150942=CARTESIAN_POINT('',(6.72928932188135,-0.299999999999999,-14.8692893218813)) ;
#150943=CARTESIAN_POINT('',(6.72928932188135,-0.399999999999999,-14.8692893218813)) ;
#150944=CARTESIAN_POINT('',(6.97071067811865,-0.0585786437626915,-15.1107106781187)) ;
#150945=CARTESIAN_POINT('',(6.87642977396045,-0.152859547920897,-15.0164297739605)) ;
#150946=CARTESIAN_POINT('',(6.97071067811865,-0.399999999999999,-15.1107106781187)) ;
#150947=CARTESIAN_POINT('Origin',(6.7,-0.399999999999999,-11.83)) ;
#150948=CARTESIAN_POINT('',(6.97071067811866,-0.058578643762691,-11.5592893218813)) ;
#150949=CARTESIAN_POINT('',(6.72928932188134,-0.300000000000002,-11.8007106781187)) ;
#150950=CARTESIAN_POINT('',(6.67642977396045,-0.352859547920897,-11.8535702260395)) ;
#150951=CARTESIAN_POINT('',(6.72928932188135,0.300000000000002,-11.8007106781187)) ;
#150952=CARTESIAN_POINT('',(6.72928932188135,-0.399999999999999,-11.8007106781187)) ;
#150953=CARTESIAN_POINT('',(6.97071067811866,0.0585786437626919,-11.5592893218813)) ;
#150954=CARTESIAN_POINT('',(6.94309644062712,0.0861928812542313,-11.5869035593729)) ;
#150955=CARTESIAN_POINT('',(6.97071067811866,-0.4,-11.5592893218813)) ;
#150956=CARTESIAN_POINT('Origin',(7.,-0.399999999999999,-11.33)) ;
#150957=CARTESIAN_POINT('',(6.97071067811865,0.0585786437626923,-11.3007106781187)) ;
#150958=CARTESIAN_POINT('',(6.72928932188135,0.300000000000001,-11.0592893218813)) ;
#150959=CARTESIAN_POINT('',(7.14309644062712,-0.113807118745769,-11.4730964406271)) ;
#150960=CARTESIAN_POINT('',(6.72928932188135,-0.300000000000002,-11.0592893218813)) ;
#150961=CARTESIAN_POINT('',(6.72928932188134,-0.399999999999999,-11.0592893218813)) ;
#150962=CARTESIAN_POINT('',(6.97071067811865,-0.0585786437626925,-11.3007106781187)) ;
#150963=CARTESIAN_POINT('',(6.87642977396045,-0.152859547920897,-11.2064297739604)) ;
#150964=CARTESIAN_POINT('',(6.97071067811865,-0.399999999999999,-11.3007106781187)) ;
#150965=CARTESIAN_POINT('Origin',(6.7,-0.399999999999999,-8.02)) ;
#150966=CARTESIAN_POINT('',(6.97071067811866,-0.0585786437626908,-7.74928932188134)) ;
#150967=CARTESIAN_POINT('',(6.72928932188134,-0.300000000000002,-7.99071067811866)) ;
#150968=CARTESIAN_POINT('',(6.67642977396045,-0.352859547920897,-8.04357022603955)) ;
#150969=CARTESIAN_POINT('',(6.72928932188135,0.300000000000002,-7.99071067811866)) ;
#150970=CARTESIAN_POINT('',(6.72928932188135,-0.399999999999999,-7.99071067811866)) ;
#150971=CARTESIAN_POINT('',(6.97071067811866,0.0585786437626916,-7.74928932188134)) ;
#150972=CARTESIAN_POINT('',(6.94309644062712,0.0861928812542312,-7.77690355937288)) ;
#150973=CARTESIAN_POINT('',(6.97071067811866,-0.4,-7.74928932188134)) ;
#150974=CARTESIAN_POINT('Origin',(7.,-0.399999999999999,-7.52)) ;
#150975=CARTESIAN_POINT('',(6.97071067811866,0.0585786437626905,-7.49071067811866)) ;
#150976=CARTESIAN_POINT('',(6.72928932188134,0.300000000000002,-7.24928932188134)) ;
#150977=CARTESIAN_POINT('',(7.14309644062712,-0.11380711874577,-7.66309644062712)) ;
#150978=CARTESIAN_POINT('',(6.72928932188135,-0.300000000000002,-7.24928932188134)) ;
#150979=CARTESIAN_POINT('',(6.72928932188135,-0.399999999999999,-7.24928932188134)) ;
#150980=CARTESIAN_POINT('',(6.97071067811866,-0.058578643762691,-7.49071067811866)) ;
#150981=CARTESIAN_POINT('',(6.87642977396045,-0.152859547920897,-7.39642977396045)) ;
#150982=CARTESIAN_POINT('',(6.97071067811866,-0.399999999999999,-7.49071067811866)) ;
#150983=CARTESIAN_POINT('Origin',(6.7,-0.399999999999999,-4.21)) ;
#150984=CARTESIAN_POINT('',(6.97071067811866,-0.058578643762691,-3.93928932188135)) ;
#150985=CARTESIAN_POINT('',(6.72928932188135,-0.300000000000001,-4.18071067811866)) ;
#150986=CARTESIAN_POINT('',(6.67642977396045,-0.352859547920897,-4.23357022603955)) ;
#150987=CARTESIAN_POINT('',(6.72928932188135,0.300000000000001,-4.18071067811866)) ;
#150988=CARTESIAN_POINT('',(6.72928932188135,-0.399999999999999,-4.18071067811866)) ;
#150989=CARTESIAN_POINT('',(6.97071067811866,0.0585786437626911,-3.93928932188135)) ;
#150990=CARTESIAN_POINT('',(6.94309644062712,0.0861928812542308,-3.96690355937289)) ;
#150991=CARTESIAN_POINT('',(6.97071067811866,-0.4,-3.93928932188135)) ;
#150992=CARTESIAN_POINT('Origin',(7.,-0.399999999999999,-3.71)) ;
#150993=CARTESIAN_POINT('',(6.97071067811866,0.058578643762691,-3.68071067811866)) ;
#150994=CARTESIAN_POINT('',(6.72928932188135,0.3,-3.43928932188135)) ;
#150995=CARTESIAN_POINT('',(7.14309644062712,-0.11380711874577,-3.85309644062712)) ;
#150996=CARTESIAN_POINT('',(6.72928932188135,-0.3,-3.43928932188135)) ;
#150997=CARTESIAN_POINT('',(6.72928932188135,-0.399999999999999,-3.43928932188135)) ;
#150998=CARTESIAN_POINT('',(6.97071067811866,-0.0585786437626913,-3.68071067811866)) ;
#150999=CARTESIAN_POINT('',(6.87642977396045,-0.152859547920897,-3.58642977396045)) ;
#151000=CARTESIAN_POINT('',(6.97071067811866,-0.399999999999999,-3.68071067811866)) ;
#151001=CARTESIAN_POINT('Origin',(-0.113807118745769,-6.47238576250846,
-3.69619288125423)) ;
#151002=CARTESIAN_POINT('Origin',(0.3,-6.05857864376269,-4.11)) ;
#151003=CARTESIAN_POINT('Origin',(0.0585786437626911,-6.3,-3.86857864376269)) ;
#151004=CARTESIAN_POINT('Origin',(0.3,-6.05857864376269,-3.41)) ;
#151005=CARTESIAN_POINT('Origin',(0.3,-6.05857864376269,-4.11)) ;
#151006=CARTESIAN_POINT('Origin',(0.3,-6.05857864376269,-3.51)) ;
#151007=CARTESIAN_POINT('Origin',(0.0585786437626908,-6.3,-3.86857864376269)) ;
#151008=CARTESIAN_POINT('Origin',(0.0585786437626908,-6.3,-3.86857864376269)) ;
#151009=CARTESIAN_POINT('Origin',(0.0585786437626908,-6.3,-3.86857864376269)) ;
#151010=CARTESIAN_POINT('Origin',(0.152859547920897,-6.20571909584179,-3.6571404520791)) ;
#151011=CARTESIAN_POINT('Origin',(0.3,-6.05857864376269,-3.51)) ;
#151012=CARTESIAN_POINT('Origin',(0.0585786437626908,-6.3,-3.75142135623731)) ;
#151013=CARTESIAN_POINT('Origin',(0.0585786437626908,-6.3,-3.41)) ;
#151014=CARTESIAN_POINT('Origin',(0.0585786437626908,-6.3,-3.75142135623731)) ;
#151015=CARTESIAN_POINT('Origin',(0.4,-6.3,-3.86857864376269)) ;
#151016=CARTESIAN_POINT('Origin',(-0.0585786437626904,-6.3,-3.86857864376269)) ;
#151017=CARTESIAN_POINT('Origin',(0.0585786437626908,-6.3,-3.75142135623731)) ;
#151018=CARTESIAN_POINT('Origin',(0.0585786437626907,-6.3,-3.75142135623731)) ;
#151019=CARTESIAN_POINT('Origin',(-0.0585786437626908,-6.3,-3.86857864376269)) ;
#151020=CARTESIAN_POINT('Origin',(-0.0585786437626908,-6.3,-3.86857864376269)) ;
#151021=CARTESIAN_POINT('Origin',(-0.0585786437626908,-6.3,-3.86857864376269)) ;
#151022=CARTESIAN_POINT('Origin',(-0.1,-6.3,-3.75142135623731)) ;
#151023=CARTESIAN_POINT('Origin',(-0.0585786437626908,-6.3,-3.75142135623731)) ;
#151024=CARTESIAN_POINT('Origin',(-0.0585786437626908,-6.3,-3.41)) ;
#151025=CARTESIAN_POINT('Origin',(-0.0585786437626908,-6.3,-3.75142135623731)) ;
#151026=CARTESIAN_POINT('Origin',(-0.0861928812542299,-6.27238576250846,
-3.89619288125423)) ;
#151027=CARTESIAN_POINT('Origin',(-0.3,-6.05857864376269,-4.11)) ;
#151028=CARTESIAN_POINT('Origin',(-0.0585786437626908,-6.3,-3.75142135623731)) ;
#151029=CARTESIAN_POINT('Origin',(-0.0585786437626909,-6.3,-3.75142135623731)) ;
#151030=CARTESIAN_POINT('Origin',(-0.3,-6.05857864376269,-3.41)) ;
#151031=CARTESIAN_POINT('Origin',(-0.3,-6.05857864376269,-4.11)) ;
#151032=CARTESIAN_POINT('Origin',(-0.3,-6.05857864376269,-3.51)) ;
#151033=CARTESIAN_POINT('Origin',(-0.352859547920897,-6.00571909584179,
-3.4571404520791)) ;
#151034=CARTESIAN_POINT('Origin',(-0.3,-6.05857864376269,-3.51)) ;
#151035=CARTESIAN_POINT('Origin',(7.07238576250846,-0.11380711874577,-3.69619288125423)) ;
#151036=CARTESIAN_POINT('Origin',(6.65857864376269,0.300000000000001,-4.11)) ;
#151037=CARTESIAN_POINT('Origin',(6.9,0.0585786437626911,-3.86857864376269)) ;
#151038=CARTESIAN_POINT('Origin',(6.65857864376269,0.300000000000001,-3.41)) ;
#151039=CARTESIAN_POINT('Origin',(6.65857864376269,0.300000000000001,-4.11)) ;
#151040=CARTESIAN_POINT('Origin',(6.65857864376269,0.300000000000001,-3.51)) ;
#151041=CARTESIAN_POINT('Origin',(6.9,0.0585786437626909,-3.86857864376269)) ;
#151042=CARTESIAN_POINT('Origin',(6.9,0.0585786437626909,-3.86857864376269)) ;
#151043=CARTESIAN_POINT('Origin',(6.9,0.0585786437626909,-3.86857864376269)) ;
#151044=CARTESIAN_POINT('Origin',(6.80571909584179,0.152859547920897,-3.6571404520791)) ;
#151045=CARTESIAN_POINT('Origin',(6.65857864376269,0.300000000000001,-3.51)) ;
#151046=CARTESIAN_POINT('Origin',(6.9,0.0585786437626909,-3.75142135623731)) ;
#151047=CARTESIAN_POINT('Origin',(6.9,0.0585786437626909,-3.41)) ;
#151048=CARTESIAN_POINT('Origin',(6.9,0.0585786437626909,-3.75142135623731)) ;
#151049=CARTESIAN_POINT('Origin',(6.9,-0.1,-3.86857864376269)) ;
#151050=CARTESIAN_POINT('Origin',(6.9,-0.058578643762691,-3.86857864376269)) ;
#151051=CARTESIAN_POINT('Origin',(6.9,0.0585786437626909,-3.75142135623731)) ;
#151052=CARTESIAN_POINT('Origin',(6.9,0.058578643762691,-3.75142135623731)) ;
#151053=CARTESIAN_POINT('Origin',(6.9,-0.0585786437626909,-3.86857864376269)) ;
#151054=CARTESIAN_POINT('Origin',(6.9,-0.0585786437626909,-3.86857864376269)) ;
#151055=CARTESIAN_POINT('Origin',(6.9,-0.0585786437626909,-3.86857864376269)) ;
#151056=CARTESIAN_POINT('Origin',(6.9,-0.399999999999999,-3.75142135623731)) ;
#151057=CARTESIAN_POINT('Origin',(6.9,-0.0585786437626909,-3.75142135623731)) ;
#151058=CARTESIAN_POINT('Origin',(6.9,-0.0585786437626909,-3.41)) ;
#151059=CARTESIAN_POINT('Origin',(6.9,-0.0585786437626909,-3.75142135623731)) ;
#151060=CARTESIAN_POINT('Origin',(6.87238576250846,-0.0861928812542305,
-3.89619288125423)) ;
#151061=CARTESIAN_POINT('Origin',(6.65857864376269,-0.3,-4.11)) ;
#151062=CARTESIAN_POINT('Origin',(6.9,-0.0585786437626909,-3.75142135623731)) ;
#151063=CARTESIAN_POINT('Origin',(6.9,-0.0585786437626913,-3.75142135623731)) ;
#151064=CARTESIAN_POINT('Origin',(6.65857864376269,-0.300000000000001,-3.41)) ;
#151065=CARTESIAN_POINT('Origin',(6.65857864376269,-0.300000000000001,-4.11)) ;
#151066=CARTESIAN_POINT('Origin',(6.65857864376269,-0.300000000000001,-3.51)) ;
#151067=CARTESIAN_POINT('Origin',(6.60571909584179,-0.352859547920897,-3.4571404520791)) ;
#151068=CARTESIAN_POINT('Origin',(6.65857864376269,-0.300000000000001,-3.51)) ;
#151069=CARTESIAN_POINT('Origin',(-0.11380711874577,-6.47238576250846,-7.50619288125423)) ;
#151070=CARTESIAN_POINT('Origin',(0.300000000000001,-6.05857864376269,-7.92)) ;
#151071=CARTESIAN_POINT('Origin',(0.0585786437626912,-6.3,-7.67857864376269)) ;
#151072=CARTESIAN_POINT('Origin',(0.3,-6.05857864376269,-7.22)) ;
#151073=CARTESIAN_POINT('Origin',(0.3,-6.05857864376269,-7.92)) ;
#151074=CARTESIAN_POINT('Origin',(0.3,-6.05857864376269,-7.32)) ;
#151075=CARTESIAN_POINT('Origin',(0.0585786437626908,-6.3,-7.67857864376269)) ;
#151076=CARTESIAN_POINT('Origin',(0.0585786437626908,-6.3,-7.67857864376269)) ;
#151077=CARTESIAN_POINT('Origin',(0.0585786437626908,-6.3,-7.67857864376269)) ;
#151078=CARTESIAN_POINT('Origin',(0.152859547920898,-6.20571909584179,-7.4671404520791)) ;
#151079=CARTESIAN_POINT('Origin',(0.300000000000001,-6.05857864376269,-7.32)) ;
#151080=CARTESIAN_POINT('Origin',(0.0585786437626908,-6.3,-7.56142135623731)) ;
#151081=CARTESIAN_POINT('Origin',(0.0585786437626908,-6.3,-7.22)) ;
#151082=CARTESIAN_POINT('Origin',(0.0585786437626908,-6.3,-7.56142135623731)) ;
#151083=CARTESIAN_POINT('Origin',(0.4,-6.3,-7.67857864376269)) ;
#151084=CARTESIAN_POINT('Origin',(-0.0585786437626906,-6.3,-7.67857864376269)) ;
#151085=CARTESIAN_POINT('Origin',(0.0585786437626908,-6.3,-7.56142135623731)) ;
#151086=CARTESIAN_POINT('Origin',(0.0585786437626908,-6.3,-7.56142135623731)) ;
#151087=CARTESIAN_POINT('Origin',(-0.0585786437626908,-6.3,-7.67857864376269)) ;
#151088=CARTESIAN_POINT('Origin',(-0.0585786437626907,-6.3,-7.67857864376269)) ;
#151089=CARTESIAN_POINT('Origin',(-0.0585786437626908,-6.3,-7.67857864376269)) ;
#151090=CARTESIAN_POINT('Origin',(-0.1,-6.3,-7.56142135623731)) ;
#151091=CARTESIAN_POINT('Origin',(-0.0585786437626908,-6.3,-7.56142135623731)) ;
#151092=CARTESIAN_POINT('Origin',(-0.0585786437626908,-6.3,-7.22)) ;
#151093=CARTESIAN_POINT('Origin',(-0.0585786437626908,-6.3,-7.56142135623731)) ;
#151094=CARTESIAN_POINT('Origin',(-0.0861928812542296,-6.27238576250846,
-7.70619288125423)) ;
#151095=CARTESIAN_POINT('Origin',(-0.3,-6.05857864376269,-7.92)) ;
#151096=CARTESIAN_POINT('Origin',(-0.0585786437626908,-6.3,-7.56142135623731)) ;
#151097=CARTESIAN_POINT('Origin',(-0.0585786437626907,-6.3,-7.56142135623731)) ;
#151098=CARTESIAN_POINT('Origin',(-0.3,-6.05857864376269,-7.22)) ;
#151099=CARTESIAN_POINT('Origin',(-0.3,-6.05857864376269,-7.92)) ;
#151100=CARTESIAN_POINT('Origin',(-0.3,-6.05857864376269,-7.32)) ;
#151101=CARTESIAN_POINT('Origin',(-0.352859547920897,-6.00571909584179,
-7.2671404520791)) ;
#151102=CARTESIAN_POINT('Origin',(-0.300000000000001,-6.05857864376269,
-7.32)) ;
#151103=CARTESIAN_POINT('Origin',(7.07238576250846,-0.11380711874577,-7.50619288125423)) ;
#151104=CARTESIAN_POINT('Origin',(6.65857864376269,0.300000000000002,-7.92)) ;
#151105=CARTESIAN_POINT('Origin',(6.9,0.0585786437626916,-7.67857864376269)) ;
#151106=CARTESIAN_POINT('Origin',(6.65857864376269,0.300000000000001,-7.22)) ;
#151107=CARTESIAN_POINT('Origin',(6.65857864376269,0.300000000000001,-7.92)) ;
#151108=CARTESIAN_POINT('Origin',(6.65857864376269,0.300000000000001,-7.32)) ;
#151109=CARTESIAN_POINT('Origin',(6.9,0.0585786437626909,-7.67857864376269)) ;
#151110=CARTESIAN_POINT('Origin',(6.9,0.0585786437626909,-7.67857864376269)) ;
#151111=CARTESIAN_POINT('Origin',(6.9,0.0585786437626909,-7.67857864376269)) ;
#151112=CARTESIAN_POINT('Origin',(6.80571909584179,0.152859547920898,-7.4671404520791)) ;
#151113=CARTESIAN_POINT('Origin',(6.65857864376269,0.300000000000002,-7.32)) ;
#151114=CARTESIAN_POINT('Origin',(6.9,0.0585786437626908,-7.56142135623731)) ;
#151115=CARTESIAN_POINT('Origin',(6.9,0.0585786437626909,-7.22)) ;
#151116=CARTESIAN_POINT('Origin',(6.9,0.0585786437626909,-7.56142135623731)) ;
#151117=CARTESIAN_POINT('Origin',(6.9,-0.1,-7.67857864376269)) ;
#151118=CARTESIAN_POINT('Origin',(6.9,-0.0585786437626908,-7.67857864376269)) ;
#151119=CARTESIAN_POINT('Origin',(6.9,0.0585786437626909,-7.56142135623731)) ;
#151120=CARTESIAN_POINT('Origin',(6.9,0.0585786437626905,-7.56142135623731)) ;
#151121=CARTESIAN_POINT('Origin',(6.9,-0.058578643762691,-7.67857864376269)) ;
#151122=CARTESIAN_POINT('Origin',(6.9,-0.058578643762691,-7.67857864376269)) ;
#151123=CARTESIAN_POINT('Origin',(6.9,-0.0585786437626909,-7.67857864376269)) ;
#151124=CARTESIAN_POINT('Origin',(6.9,-0.399999999999999,-7.56142135623731)) ;
#151125=CARTESIAN_POINT('Origin',(6.9,-0.0585786437626909,-7.56142135623731)) ;
#151126=CARTESIAN_POINT('Origin',(6.9,-0.0585786437626909,-7.22)) ;
#151127=CARTESIAN_POINT('Origin',(6.9,-0.0585786437626909,-7.56142135623731)) ;
#151128=CARTESIAN_POINT('Origin',(6.87238576250846,-0.0861928812542304,
-7.70619288125423)) ;
#151129=CARTESIAN_POINT('Origin',(6.65857864376269,-0.300000000000001,-7.92)) ;
#151130=CARTESIAN_POINT('Origin',(6.9,-0.058578643762691,-7.56142135623731)) ;
#151131=CARTESIAN_POINT('Origin',(6.9,-0.058578643762691,-7.56142135623731)) ;
#151132=CARTESIAN_POINT('Origin',(6.65857864376269,-0.300000000000001,-7.22)) ;
#151133=CARTESIAN_POINT('Origin',(6.65857864376269,-0.300000000000001,-7.92)) ;
#151134=CARTESIAN_POINT('Origin',(6.65857864376269,-0.300000000000001,-7.32)) ;
#151135=CARTESIAN_POINT('Origin',(6.60571909584179,-0.352859547920898,-7.2671404520791)) ;
#151136=CARTESIAN_POINT('Origin',(6.65857864376269,-0.300000000000001,-7.32)) ;
#151137=CARTESIAN_POINT('Origin',(-0.11380711874577,-6.47238576250846,-11.3161928812542)) ;
#151138=CARTESIAN_POINT('Origin',(0.299999999999999,-6.05857864376269,-11.73)) ;
#151139=CARTESIAN_POINT('Origin',(0.0585786437626907,-6.3,-11.4885786437627)) ;
#151140=CARTESIAN_POINT('Origin',(0.3,-6.05857864376269,-11.03)) ;
#151141=CARTESIAN_POINT('Origin',(0.3,-6.05857864376269,-11.73)) ;
#151142=CARTESIAN_POINT('Origin',(0.3,-6.05857864376269,-11.13)) ;
#151143=CARTESIAN_POINT('Origin',(0.0585786437626908,-6.3,-11.4885786437627)) ;
#151144=CARTESIAN_POINT('Origin',(0.0585786437626908,-6.3,-11.4885786437627)) ;
#151145=CARTESIAN_POINT('Origin',(0.0585786437626908,-6.3,-11.4885786437627)) ;
#151146=CARTESIAN_POINT('Origin',(0.152859547920898,-6.20571909584179,-11.2771404520791)) ;
#151147=CARTESIAN_POINT('Origin',(0.300000000000003,-6.05857864376269,-11.13)) ;
#151148=CARTESIAN_POINT('Origin',(0.0585786437626905,-6.3,-11.3714213562373)) ;
#151149=CARTESIAN_POINT('Origin',(0.0585786437626908,-6.3,-11.03)) ;
#151150=CARTESIAN_POINT('Origin',(0.0585786437626908,-6.3,-11.3714213562373)) ;
#151151=CARTESIAN_POINT('Origin',(0.4,-6.3,-11.4885786437627)) ;
#151152=CARTESIAN_POINT('Origin',(-0.0585786437626916,-6.3,-11.4885786437627)) ;
#151153=CARTESIAN_POINT('Origin',(0.0585786437626908,-6.3,-11.3714213562373)) ;
#151154=CARTESIAN_POINT('Origin',(0.0585786437626913,-6.3,-11.3714213562373)) ;
#151155=CARTESIAN_POINT('Origin',(-0.0585786437626908,-6.3,-11.4885786437627)) ;
#151156=CARTESIAN_POINT('Origin',(-0.0585786437626908,-6.3,-11.4885786437627)) ;
#151157=CARTESIAN_POINT('Origin',(-0.0585786437626908,-6.3,-11.4885786437627)) ;
#151158=CARTESIAN_POINT('Origin',(-0.1,-6.3,-11.3714213562373)) ;
#151159=CARTESIAN_POINT('Origin',(-0.0585786437626908,-6.3,-11.3714213562373)) ;
#151160=CARTESIAN_POINT('Origin',(-0.0585786437626908,-6.3,-11.03)) ;
#151161=CARTESIAN_POINT('Origin',(-0.0585786437626908,-6.3,-11.3714213562373)) ;
#151162=CARTESIAN_POINT('Origin',(-0.0861928812542293,-6.27238576250846,
-11.5161928812542)) ;
#151163=CARTESIAN_POINT('Origin',(-0.3,-6.05857864376269,-11.73)) ;
#151164=CARTESIAN_POINT('Origin',(-0.0585786437626908,-6.3,-11.3714213562373)) ;
#151165=CARTESIAN_POINT('Origin',(-0.0585786437626915,-6.3,-11.3714213562373)) ;
#151166=CARTESIAN_POINT('Origin',(-0.3,-6.05857864376269,-11.03)) ;
#151167=CARTESIAN_POINT('Origin',(-0.3,-6.05857864376269,-11.73)) ;
#151168=CARTESIAN_POINT('Origin',(-0.3,-6.05857864376269,-11.13)) ;
#151169=CARTESIAN_POINT('Origin',(-0.352859547920898,-6.00571909584179,
-11.0771404520791)) ;
#151170=CARTESIAN_POINT('Origin',(-0.300000000000003,-6.05857864376269,
-11.13)) ;
#151171=CARTESIAN_POINT('Origin',(7.07238576250846,-0.11380711874577,-11.3161928812542)) ;
#151172=CARTESIAN_POINT('Origin',(6.65857864376269,0.300000000000003,-11.73)) ;
#151173=CARTESIAN_POINT('Origin',(6.9,0.0585786437626919,-11.4885786437627)) ;
#151174=CARTESIAN_POINT('Origin',(6.65857864376269,0.300000000000001,-11.03)) ;
#151175=CARTESIAN_POINT('Origin',(6.65857864376269,0.300000000000001,-11.73)) ;
#151176=CARTESIAN_POINT('Origin',(6.65857864376269,0.300000000000001,-11.13)) ;
#151177=CARTESIAN_POINT('Origin',(6.9,0.0585786437626909,-11.4885786437627)) ;
#151178=CARTESIAN_POINT('Origin',(6.9,0.0585786437626909,-11.4885786437627)) ;
#151179=CARTESIAN_POINT('Origin',(6.9,0.0585786437626909,-11.4885786437627)) ;
#151180=CARTESIAN_POINT('Origin',(6.80571909584179,0.152859547920898,-11.2771404520791)) ;
#151181=CARTESIAN_POINT('Origin',(6.65857864376269,0.300000000000003,-11.13)) ;
#151182=CARTESIAN_POINT('Origin',(6.9,0.0585786437626911,-11.3714213562373)) ;
#151183=CARTESIAN_POINT('Origin',(6.9,0.0585786437626909,-11.03)) ;
#151184=CARTESIAN_POINT('Origin',(6.9,0.0585786437626909,-11.3714213562373)) ;
#151185=CARTESIAN_POINT('Origin',(6.9,-0.1,-11.4885786437627)) ;
#151186=CARTESIAN_POINT('Origin',(6.9,-0.058578643762691,-11.4885786437627)) ;
#151187=CARTESIAN_POINT('Origin',(6.9,0.0585786437626909,-11.3714213562373)) ;
#151188=CARTESIAN_POINT('Origin',(6.9,0.0585786437626923,-11.3714213562373)) ;
#151189=CARTESIAN_POINT('Origin',(6.9,-0.058578643762691,-11.4885786437627)) ;
#151190=CARTESIAN_POINT('Origin',(6.9,-0.0585786437626912,-11.4885786437627)) ;
#151191=CARTESIAN_POINT('Origin',(6.9,-0.0585786437626909,-11.4885786437627)) ;
#151192=CARTESIAN_POINT('Origin',(6.9,-0.399999999999999,-11.3714213562373)) ;
#151193=CARTESIAN_POINT('Origin',(6.9,-0.0585786437626909,-11.3714213562373)) ;
#151194=CARTESIAN_POINT('Origin',(6.9,-0.0585786437626909,-11.03)) ;
#151195=CARTESIAN_POINT('Origin',(6.9,-0.0585786437626909,-11.3714213562373)) ;
#151196=CARTESIAN_POINT('Origin',(6.87238576250846,-0.0861928812542304,
-11.5161928812542)) ;
#151197=CARTESIAN_POINT('Origin',(6.65857864376269,-0.300000000000002,-11.73)) ;
#151198=CARTESIAN_POINT('Origin',(6.9,-0.058578643762691,-11.3714213562373)) ;
#151199=CARTESIAN_POINT('Origin',(6.9,-0.0585786437626925,-11.3714213562373)) ;
#151200=CARTESIAN_POINT('Origin',(6.65857864376269,-0.300000000000001,-11.03)) ;
#151201=CARTESIAN_POINT('Origin',(6.65857864376269,-0.300000000000001,-11.73)) ;
#151202=CARTESIAN_POINT('Origin',(6.65857864376269,-0.300000000000001,-11.13)) ;
#151203=CARTESIAN_POINT('Origin',(6.60571909584179,-0.352859547920898,-11.0771404520791)) ;
#151204=CARTESIAN_POINT('Origin',(6.65857864376269,-0.300000000000003,-11.13)) ;
#151205=CARTESIAN_POINT('Origin',(-0.113807118745769,-6.47238576250846,
-15.1261928812542)) ;
#151206=CARTESIAN_POINT('Origin',(0.300000000000001,-6.05857864376269,-15.54)) ;
#151207=CARTESIAN_POINT('Origin',(0.0585786437626911,-6.3,-15.2985786437627)) ;
#151208=CARTESIAN_POINT('Origin',(0.3,-6.05857864376269,-14.84)) ;
#151209=CARTESIAN_POINT('Origin',(0.3,-6.05857864376269,-15.54)) ;
#151210=CARTESIAN_POINT('Origin',(0.3,-6.05857864376269,-14.94)) ;
#151211=CARTESIAN_POINT('Origin',(0.0585786437626908,-6.3,-15.2985786437627)) ;
#151212=CARTESIAN_POINT('Origin',(0.0585786437626908,-6.3,-15.2985786437627)) ;
#151213=CARTESIAN_POINT('Origin',(0.0585786437626908,-6.3,-15.2985786437627)) ;
#151214=CARTESIAN_POINT('Origin',(0.152859547920898,-6.20571909584179,-15.0871404520791)) ;
#151215=CARTESIAN_POINT('Origin',(0.300000000000001,-6.05857864376269,-14.94)) ;
#151216=CARTESIAN_POINT('Origin',(0.0585786437626911,-6.3,-15.1814213562373)) ;
#151217=CARTESIAN_POINT('Origin',(0.0585786437626908,-6.3,-14.84)) ;
#151218=CARTESIAN_POINT('Origin',(0.0585786437626908,-6.3,-15.1814213562373)) ;
#151219=CARTESIAN_POINT('Origin',(0.4,-6.3,-15.2985786437627)) ;
#151220=CARTESIAN_POINT('Origin',(-0.0585786437626904,-6.3,-15.2985786437627)) ;
#151221=CARTESIAN_POINT('Origin',(0.0585786437626908,-6.3,-15.1814213562373)) ;
#151222=CARTESIAN_POINT('Origin',(0.0585786437626904,-6.3,-15.1814213562373)) ;
#151223=CARTESIAN_POINT('Origin',(-0.0585786437626908,-6.3,-15.2985786437627)) ;
#151224=CARTESIAN_POINT('Origin',(-0.0585786437626908,-6.3,-15.2985786437627)) ;
#151225=CARTESIAN_POINT('Origin',(-0.0585786437626908,-6.3,-15.2985786437627)) ;
#151226=CARTESIAN_POINT('Origin',(-0.1,-6.3,-15.1814213562373)) ;
#151227=CARTESIAN_POINT('Origin',(-0.0585786437626908,-6.3,-15.1814213562373)) ;
#151228=CARTESIAN_POINT('Origin',(-0.0585786437626908,-6.3,-14.84)) ;
#151229=CARTESIAN_POINT('Origin',(-0.0585786437626908,-6.3,-15.1814213562373)) ;
#151230=CARTESIAN_POINT('Origin',(-0.0861928812542299,-6.27238576250846,
-15.3261928812542)) ;
#151231=CARTESIAN_POINT('Origin',(-0.300000000000001,-6.05857864376269,
-15.54)) ;
#151232=CARTESIAN_POINT('Origin',(-0.0585786437626908,-6.3,-15.1814213562373)) ;
#151233=CARTESIAN_POINT('Origin',(-0.0585786437626914,-6.3,-15.1814213562373)) ;
#151234=CARTESIAN_POINT('Origin',(-0.3,-6.05857864376269,-14.84)) ;
#151235=CARTESIAN_POINT('Origin',(-0.3,-6.05857864376269,-15.54)) ;
#151236=CARTESIAN_POINT('Origin',(-0.3,-6.05857864376269,-14.94)) ;
#151237=CARTESIAN_POINT('Origin',(-0.352859547920897,-6.00571909584179,
-14.8871404520791)) ;
#151238=CARTESIAN_POINT('Origin',(-0.3,-6.05857864376269,-14.94)) ;
#151239=CARTESIAN_POINT('Origin',(7.07238576250846,-0.11380711874577,-15.1261928812542)) ;
#151240=CARTESIAN_POINT('Origin',(6.65857864376269,0.300000000000003,-15.54)) ;
#151241=CARTESIAN_POINT('Origin',(6.9,0.0585786437626913,-15.2985786437627)) ;
#151242=CARTESIAN_POINT('Origin',(6.65857864376269,0.300000000000001,-14.84)) ;
#151243=CARTESIAN_POINT('Origin',(6.65857864376269,0.300000000000001,-15.54)) ;
#151244=CARTESIAN_POINT('Origin',(6.65857864376269,0.300000000000001,-14.94)) ;
#151245=CARTESIAN_POINT('Origin',(6.9,0.0585786437626909,-15.2985786437627)) ;
#151246=CARTESIAN_POINT('Origin',(6.9,0.0585786437626909,-15.2985786437627)) ;
#151247=CARTESIAN_POINT('Origin',(6.9,0.0585786437626909,-15.2985786437627)) ;
#151248=CARTESIAN_POINT('Origin',(6.80571909584179,0.152859547920897,-15.0871404520791)) ;
#151249=CARTESIAN_POINT('Origin',(6.65857864376269,0.300000000000001,-14.94)) ;
#151250=CARTESIAN_POINT('Origin',(6.9,0.0585786437626909,-15.1814213562373)) ;
#151251=CARTESIAN_POINT('Origin',(6.9,0.0585786437626909,-14.84)) ;
#151252=CARTESIAN_POINT('Origin',(6.9,0.0585786437626909,-15.1814213562373)) ;
#151253=CARTESIAN_POINT('Origin',(6.9,-0.1,-15.2985786437627)) ;
#151254=CARTESIAN_POINT('Origin',(6.9,-0.058578643762691,-15.2985786437627)) ;
#151255=CARTESIAN_POINT('Origin',(6.9,0.0585786437626909,-15.1814213562373)) ;
#151256=CARTESIAN_POINT('Origin',(6.9,0.0585786437626917,-15.1814213562373)) ;
#151257=CARTESIAN_POINT('Origin',(6.9,-0.0585786437626909,-15.2985786437627)) ;
#151258=CARTESIAN_POINT('Origin',(6.9,-0.058578643762691,-15.2985786437627)) ;
#151259=CARTESIAN_POINT('Origin',(6.9,-0.0585786437626909,-15.2985786437627)) ;
#151260=CARTESIAN_POINT('Origin',(6.9,-0.399999999999999,-15.1814213562373)) ;
#151261=CARTESIAN_POINT('Origin',(6.9,-0.0585786437626909,-15.1814213562373)) ;
#151262=CARTESIAN_POINT('Origin',(6.9,-0.0585786437626909,-14.84)) ;
#151263=CARTESIAN_POINT('Origin',(6.9,-0.0585786437626909,-15.1814213562373)) ;
#151264=CARTESIAN_POINT('Origin',(6.87238576250846,-0.0861928812542304,
-15.3261928812542)) ;
#151265=CARTESIAN_POINT('Origin',(6.65857864376269,-0.300000000000002,-15.54)) ;
#151266=CARTESIAN_POINT('Origin',(6.9,-0.058578643762691,-15.1814213562373)) ;
#151267=CARTESIAN_POINT('Origin',(6.9,-0.0585786437626915,-15.1814213562373)) ;
#151268=CARTESIAN_POINT('Origin',(6.65857864376269,-0.300000000000001,-14.84)) ;
#151269=CARTESIAN_POINT('Origin',(6.65857864376269,-0.300000000000001,-15.54)) ;
#151270=CARTESIAN_POINT('Origin',(6.65857864376269,-0.300000000000001,-14.94)) ;
#151271=CARTESIAN_POINT('Origin',(6.60571909584179,-0.352859547920897,-14.8871404520791)) ;
#151272=CARTESIAN_POINT('Origin',(6.65857864376269,-0.300000000000001,-14.94)) ;
#151273=CARTESIAN_POINT('Origin',(-0.113807118745769,-6.47238576250846,
-18.9361928812542)) ;
#151274=CARTESIAN_POINT('Origin',(0.300000000000001,-6.05857864376269,-19.35)) ;
#151275=CARTESIAN_POINT('Origin',(0.058578643762692,-6.3,-19.1085786437627)) ;
#151276=CARTESIAN_POINT('Origin',(0.3,-6.05857864376269,-18.65)) ;
#151277=CARTESIAN_POINT('Origin',(0.3,-6.05857864376269,-19.35)) ;
#151278=CARTESIAN_POINT('Origin',(0.3,-6.05857864376269,-18.75)) ;
#151279=CARTESIAN_POINT('Origin',(0.0585786437626908,-6.3,-19.1085786437627)) ;
#151280=CARTESIAN_POINT('Origin',(0.0585786437626908,-6.3,-19.1085786437627)) ;
#151281=CARTESIAN_POINT('Origin',(0.0585786437626908,-6.3,-19.1085786437627)) ;
#151282=CARTESIAN_POINT('Origin',(0.152859547920896,-6.2057190958418,-18.8971404520791)) ;
#151283=CARTESIAN_POINT('Origin',(0.299999999999995,-6.0585786437627,-18.75)) ;
#151284=CARTESIAN_POINT('Origin',(0.0585786437626908,-6.3,-18.9914213562373)) ;
#151285=CARTESIAN_POINT('Origin',(0.0585786437626908,-6.3,-18.65)) ;
#151286=CARTESIAN_POINT('Origin',(0.0585786437626908,-6.3,-18.9914213562373)) ;
#151287=CARTESIAN_POINT('Origin',(0.4,-6.3,-19.1085786437627)) ;
#151288=CARTESIAN_POINT('Origin',(-0.0585786437626899,-6.3,-19.1085786437627)) ;
#151289=CARTESIAN_POINT('Origin',(0.0585786437626908,-6.3,-18.9914213562373)) ;
#151290=CARTESIAN_POINT('Origin',(0.0585786437626916,-6.3,-18.9914213562373)) ;
#151291=CARTESIAN_POINT('Origin',(-0.0585786437626908,-6.3,-19.1085786437627)) ;
#151292=CARTESIAN_POINT('Origin',(-0.0585786437626905,-6.3,-19.1085786437627)) ;
#151293=CARTESIAN_POINT('Origin',(-0.0585786437626908,-6.3,-19.1085786437627)) ;
#151294=CARTESIAN_POINT('Origin',(-0.1,-6.3,-18.9914213562373)) ;
#151295=CARTESIAN_POINT('Origin',(-0.0585786437626908,-6.3,-18.9914213562373)) ;
#151296=CARTESIAN_POINT('Origin',(-0.0585786437626908,-6.3,-18.65)) ;
#151297=CARTESIAN_POINT('Origin',(-0.0585786437626908,-6.3,-18.9914213562373)) ;
#151298=CARTESIAN_POINT('Origin',(-0.0861928812542299,-6.27238576250846,
-19.1361928812542)) ;
#151299=CARTESIAN_POINT('Origin',(-0.299999999999999,-6.05857864376269,
-19.35)) ;
#151300=CARTESIAN_POINT('Origin',(-0.0585786437626908,-6.3,-18.9914213562373)) ;
#151301=CARTESIAN_POINT('Origin',(-0.0585786437626909,-6.3,-18.9914213562373)) ;
#151302=CARTESIAN_POINT('Origin',(-0.3,-6.05857864376269,-18.65)) ;
#151303=CARTESIAN_POINT('Origin',(-0.3,-6.05857864376269,-19.35)) ;
#151304=CARTESIAN_POINT('Origin',(-0.3,-6.05857864376269,-18.75)) ;
#151305=CARTESIAN_POINT('Origin',(-0.352859547920895,-6.00571909584179,
-18.6971404520791)) ;
#151306=CARTESIAN_POINT('Origin',(-0.299999999999997,-6.05857864376269,
-18.75)) ;
#151307=CARTESIAN_POINT('Origin',(7.07238576250846,-0.11380711874577,-18.9361928812542)) ;
#151308=CARTESIAN_POINT('Origin',(6.65857864376269,0.299999999999999,-19.35)) ;
#151309=CARTESIAN_POINT('Origin',(6.9,0.0585786437626903,-19.1085786437627)) ;
#151310=CARTESIAN_POINT('Origin',(6.65857864376269,0.300000000000001,-18.65)) ;
#151311=CARTESIAN_POINT('Origin',(6.65857864376269,0.300000000000001,-19.35)) ;
#151312=CARTESIAN_POINT('Origin',(6.65857864376269,0.300000000000001,-18.75)) ;
#151313=CARTESIAN_POINT('Origin',(6.9,0.0585786437626909,-19.1085786437627)) ;
#151314=CARTESIAN_POINT('Origin',(6.9,0.0585786437626909,-19.1085786437627)) ;
#151315=CARTESIAN_POINT('Origin',(6.9,0.0585786437626909,-19.1085786437627)) ;
#151316=CARTESIAN_POINT('Origin',(6.8057190958418,0.152859547920896,-18.8971404520791)) ;
#151317=CARTESIAN_POINT('Origin',(6.6585786437627,0.299999999999996,-18.75)) ;
#151318=CARTESIAN_POINT('Origin',(6.9,0.0585786437626908,-18.9914213562373)) ;
#151319=CARTESIAN_POINT('Origin',(6.9,0.0585786437626909,-18.65)) ;
#151320=CARTESIAN_POINT('Origin',(6.9,0.0585786437626909,-18.9914213562373)) ;
#151321=CARTESIAN_POINT('Origin',(6.9,-0.1,-19.1085786437627)) ;
#151322=CARTESIAN_POINT('Origin',(6.9,-0.0585786437626902,-19.1085786437627)) ;
#151323=CARTESIAN_POINT('Origin',(6.9,0.0585786437626909,-18.9914213562373)) ;
#151324=CARTESIAN_POINT('Origin',(6.9,0.058578643762691,-18.9914213562373)) ;
#151325=CARTESIAN_POINT('Origin',(6.9,-0.0585786437626909,-19.1085786437627)) ;
#151326=CARTESIAN_POINT('Origin',(6.9,-0.0585786437626907,-19.1085786437627)) ;
#151327=CARTESIAN_POINT('Origin',(6.9,-0.0585786437626909,-19.1085786437627)) ;
#151328=CARTESIAN_POINT('Origin',(6.9,-0.399999999999999,-18.9914213562373)) ;
#151329=CARTESIAN_POINT('Origin',(6.9,-0.0585786437626909,-18.9914213562373)) ;
#151330=CARTESIAN_POINT('Origin',(6.9,-0.0585786437626909,-18.65)) ;
#151331=CARTESIAN_POINT('Origin',(6.9,-0.058578643762691,-18.9914213562373)) ;
#151332=CARTESIAN_POINT('Origin',(6.87238576250846,-0.0861928812542304,
-19.1361928812542)) ;
#151333=CARTESIAN_POINT('Origin',(6.65857864376269,-0.3,-19.35)) ;
#151334=CARTESIAN_POINT('Origin',(6.9,-0.0585786437626909,-18.9914213562373)) ;
#151335=CARTESIAN_POINT('Origin',(6.9,-0.0585786437626907,-18.9914213562373)) ;
#151336=CARTESIAN_POINT('Origin',(6.65857864376269,-0.300000000000001,-18.65)) ;
#151337=CARTESIAN_POINT('Origin',(6.65857864376269,-0.300000000000001,-19.35)) ;
#151338=CARTESIAN_POINT('Origin',(6.65857864376269,-0.300000000000001,-18.75)) ;
#151339=CARTESIAN_POINT('Origin',(6.6057190958418,-0.352859547920896,-18.6971404520791)) ;
#151340=CARTESIAN_POINT('Origin',(6.65857864376269,-0.299999999999998,-18.75)) ;
#151341=CARTESIAN_POINT('Origin',(-0.113807118745769,-6.47238576250846,
-22.7461928812542)) ;
#151342=CARTESIAN_POINT('Origin',(0.300000000000001,-6.05857864376269,-23.16)) ;
#151343=CARTESIAN_POINT('Origin',(0.058578643762692,-6.3,-22.9185786437627)) ;
#151344=CARTESIAN_POINT('Origin',(0.3,-6.05857864376269,-22.46)) ;
#151345=CARTESIAN_POINT('Origin',(0.3,-6.05857864376269,-23.16)) ;
#151346=CARTESIAN_POINT('Origin',(0.3,-6.05857864376269,-22.56)) ;
#151347=CARTESIAN_POINT('Origin',(0.0585786437626908,-6.3,-22.9185786437627)) ;
#151348=CARTESIAN_POINT('Origin',(0.0585786437626908,-6.3,-22.9185786437627)) ;
#151349=CARTESIAN_POINT('Origin',(0.0585786437626908,-6.3,-22.9185786437627)) ;
#151350=CARTESIAN_POINT('Origin',(0.152859547920896,-6.2057190958418,-22.7071404520791)) ;
#151351=CARTESIAN_POINT('Origin',(0.299999999999995,-6.0585786437627,-22.56)) ;
#151352=CARTESIAN_POINT('Origin',(0.0585786437626908,-6.3,-22.8014213562373)) ;
#151353=CARTESIAN_POINT('Origin',(0.0585786437626908,-6.3,-22.46)) ;
#151354=CARTESIAN_POINT('Origin',(0.0585786437626908,-6.3,-22.8014213562373)) ;
#151355=CARTESIAN_POINT('Origin',(0.4,-6.3,-22.9185786437627)) ;
#151356=CARTESIAN_POINT('Origin',(-0.0585786437626899,-6.3,-22.9185786437627)) ;
#151357=CARTESIAN_POINT('Origin',(0.0585786437626908,-6.3,-22.8014213562373)) ;
#151358=CARTESIAN_POINT('Origin',(0.0585786437626916,-6.3,-22.8014213562373)) ;
#151359=CARTESIAN_POINT('Origin',(-0.0585786437626908,-6.3,-22.9185786437627)) ;
#151360=CARTESIAN_POINT('Origin',(-0.0585786437626905,-6.3,-22.9185786437627)) ;
#151361=CARTESIAN_POINT('Origin',(-0.0585786437626908,-6.3,-22.9185786437627)) ;
#151362=CARTESIAN_POINT('Origin',(-0.1,-6.3,-22.8014213562373)) ;
#151363=CARTESIAN_POINT('Origin',(-0.0585786437626908,-6.3,-22.8014213562373)) ;
#151364=CARTESIAN_POINT('Origin',(-0.0585786437626908,-6.3,-22.46)) ;
#151365=CARTESIAN_POINT('Origin',(-0.0585786437626908,-6.3,-22.8014213562373)) ;
#151366=CARTESIAN_POINT('Origin',(-0.0861928812542299,-6.27238576250846,
-22.9461928812542)) ;
#151367=CARTESIAN_POINT('Origin',(-0.299999999999999,-6.05857864376269,
-23.16)) ;
#151368=CARTESIAN_POINT('Origin',(-0.0585786437626908,-6.3,-22.8014213562373)) ;
#151369=CARTESIAN_POINT('Origin',(-0.0585786437626909,-6.3,-22.8014213562373)) ;
#151370=CARTESIAN_POINT('Origin',(-0.3,-6.05857864376269,-22.46)) ;
#151371=CARTESIAN_POINT('Origin',(-0.3,-6.05857864376269,-23.16)) ;
#151372=CARTESIAN_POINT('Origin',(-0.3,-6.05857864376269,-22.56)) ;
#151373=CARTESIAN_POINT('Origin',(-0.352859547920895,-6.00571909584179,
-22.5071404520791)) ;
#151374=CARTESIAN_POINT('Origin',(-0.299999999999997,-6.05857864376269,
-22.56)) ;
#151375=CARTESIAN_POINT('Origin',(7.07238576250846,-0.11380711874577,-22.7461928812542)) ;
#151376=CARTESIAN_POINT('Origin',(6.65857864376269,0.299999999999999,-23.16)) ;
#151377=CARTESIAN_POINT('Origin',(6.9,0.0585786437626903,-22.9185786437627)) ;
#151378=CARTESIAN_POINT('Origin',(6.65857864376269,0.300000000000001,-22.46)) ;
#151379=CARTESIAN_POINT('Origin',(6.65857864376269,0.300000000000001,-23.16)) ;
#151380=CARTESIAN_POINT('Origin',(6.65857864376269,0.300000000000001,-22.56)) ;
#151381=CARTESIAN_POINT('Origin',(6.9,0.0585786437626909,-22.9185786437627)) ;
#151382=CARTESIAN_POINT('Origin',(6.9,0.0585786437626909,-22.9185786437627)) ;
#151383=CARTESIAN_POINT('Origin',(6.9,0.0585786437626909,-22.9185786437627)) ;
#151384=CARTESIAN_POINT('Origin',(6.8057190958418,0.152859547920896,-22.7071404520791)) ;
#151385=CARTESIAN_POINT('Origin',(6.6585786437627,0.299999999999996,-22.56)) ;
#151386=CARTESIAN_POINT('Origin',(6.9,0.0585786437626908,-22.8014213562373)) ;
#151387=CARTESIAN_POINT('Origin',(6.9,0.0585786437626909,-22.46)) ;
#151388=CARTESIAN_POINT('Origin',(6.9,0.0585786437626909,-22.8014213562373)) ;
#151389=CARTESIAN_POINT('Origin',(6.9,-0.1,-22.9185786437627)) ;
#151390=CARTESIAN_POINT('Origin',(6.9,-0.0585786437626902,-22.9185786437627)) ;
#151391=CARTESIAN_POINT('Origin',(6.9,0.0585786437626909,-22.8014213562373)) ;
#151392=CARTESIAN_POINT('Origin',(6.9,0.058578643762691,-22.8014213562373)) ;
#151393=CARTESIAN_POINT('Origin',(6.9,-0.0585786437626909,-22.9185786437627)) ;
#151394=CARTESIAN_POINT('Origin',(6.9,-0.0585786437626907,-22.9185786437627)) ;
#151395=CARTESIAN_POINT('Origin',(6.9,-0.0585786437626909,-22.9185786437627)) ;
#151396=CARTESIAN_POINT('Origin',(6.9,-0.399999999999999,-22.8014213562373)) ;
#151397=CARTESIAN_POINT('Origin',(6.9,-0.0585786437626909,-22.8014213562373)) ;
#151398=CARTESIAN_POINT('Origin',(6.9,-0.0585786437626909,-22.46)) ;
#151399=CARTESIAN_POINT('Origin',(6.9,-0.058578643762691,-22.8014213562373)) ;
#151400=CARTESIAN_POINT('Origin',(6.87238576250846,-0.0861928812542304,
-22.9461928812542)) ;
#151401=CARTESIAN_POINT('Origin',(6.65857864376269,-0.3,-23.16)) ;
#151402=CARTESIAN_POINT('Origin',(6.9,-0.0585786437626909,-22.8014213562373)) ;
#151403=CARTESIAN_POINT('Origin',(6.9,-0.0585786437626907,-22.8014213562373)) ;
#151404=CARTESIAN_POINT('Origin',(6.65857864376269,-0.300000000000001,-22.46)) ;
#151405=CARTESIAN_POINT('Origin',(6.65857864376269,-0.300000000000001,-23.16)) ;
#151406=CARTESIAN_POINT('Origin',(6.65857864376269,-0.300000000000001,-22.56)) ;
#151407=CARTESIAN_POINT('Origin',(6.6057190958418,-0.352859547920896,-22.5071404520791)) ;
#151408=CARTESIAN_POINT('Origin',(6.65857864376269,-0.299999999999998,-22.56)) ;
#151409=CARTESIAN_POINT('Origin',(-0.113807118745769,-6.47238576250846,
-26.5561928812542)) ;
#151410=CARTESIAN_POINT('Origin',(0.300000000000001,-6.05857864376269,-26.97)) ;
#151411=CARTESIAN_POINT('Origin',(0.058578643762692,-6.3,-26.7285786437627)) ;
#151412=CARTESIAN_POINT('Origin',(0.3,-6.05857864376269,-26.27)) ;
#151413=CARTESIAN_POINT('Origin',(0.3,-6.05857864376269,-26.97)) ;
#151414=CARTESIAN_POINT('Origin',(0.3,-6.05857864376269,-26.37)) ;
#151415=CARTESIAN_POINT('Origin',(0.0585786437626908,-6.3,-26.7285786437627)) ;
#151416=CARTESIAN_POINT('Origin',(0.0585786437626908,-6.3,-26.7285786437627)) ;
#151417=CARTESIAN_POINT('Origin',(0.0585786437626908,-6.3,-26.7285786437627)) ;
#151418=CARTESIAN_POINT('Origin',(0.152859547920896,-6.2057190958418,-26.5171404520791)) ;
#151419=CARTESIAN_POINT('Origin',(0.299999999999995,-6.0585786437627,-26.37)) ;
#151420=CARTESIAN_POINT('Origin',(0.0585786437626908,-6.3,-26.6114213562373)) ;
#151421=CARTESIAN_POINT('Origin',(0.0585786437626908,-6.3,-26.27)) ;
#151422=CARTESIAN_POINT('Origin',(0.0585786437626908,-6.3,-26.6114213562373)) ;
#151423=CARTESIAN_POINT('Origin',(0.4,-6.3,-26.7285786437627)) ;
#151424=CARTESIAN_POINT('Origin',(-0.0585786437626899,-6.3,-26.7285786437627)) ;
#151425=CARTESIAN_POINT('Origin',(0.0585786437626908,-6.3,-26.6114213562373)) ;
#151426=CARTESIAN_POINT('Origin',(0.0585786437626916,-6.3,-26.6114213562373)) ;
#151427=CARTESIAN_POINT('Origin',(-0.0585786437626908,-6.3,-26.7285786437627)) ;
#151428=CARTESIAN_POINT('Origin',(-0.0585786437626905,-6.3,-26.7285786437627)) ;
#151429=CARTESIAN_POINT('Origin',(-0.0585786437626908,-6.3,-26.7285786437627)) ;
#151430=CARTESIAN_POINT('Origin',(-0.1,-6.3,-26.6114213562373)) ;
#151431=CARTESIAN_POINT('Origin',(-0.0585786437626908,-6.3,-26.6114213562373)) ;
#151432=CARTESIAN_POINT('Origin',(-0.0585786437626908,-6.3,-26.27)) ;
#151433=CARTESIAN_POINT('Origin',(-0.0585786437626908,-6.3,-26.6114213562373)) ;
#151434=CARTESIAN_POINT('Origin',(-0.0861928812542299,-6.27238576250846,
-26.7561928812542)) ;
#151435=CARTESIAN_POINT('Origin',(-0.299999999999999,-6.05857864376269,
-26.97)) ;
#151436=CARTESIAN_POINT('Origin',(-0.0585786437626908,-6.3,-26.6114213562373)) ;
#151437=CARTESIAN_POINT('Origin',(-0.0585786437626909,-6.3,-26.6114213562373)) ;
#151438=CARTESIAN_POINT('Origin',(-0.3,-6.05857864376269,-26.27)) ;
#151439=CARTESIAN_POINT('Origin',(-0.3,-6.05857864376269,-26.97)) ;
#151440=CARTESIAN_POINT('Origin',(-0.3,-6.05857864376269,-26.37)) ;
#151441=CARTESIAN_POINT('Origin',(-0.352859547920895,-6.00571909584179,
-26.3171404520791)) ;
#151442=CARTESIAN_POINT('Origin',(-0.299999999999997,-6.05857864376269,
-26.37)) ;
#151443=CARTESIAN_POINT('Origin',(7.07238576250846,-0.11380711874577,-26.5561928812542)) ;
#151444=CARTESIAN_POINT('Origin',(6.65857864376269,0.299999999999999,-26.97)) ;
#151445=CARTESIAN_POINT('Origin',(6.9,0.0585786437626903,-26.7285786437627)) ;
#151446=CARTESIAN_POINT('Origin',(6.65857864376269,0.300000000000001,-26.27)) ;
#151447=CARTESIAN_POINT('Origin',(6.65857864376269,0.300000000000001,-26.97)) ;
#151448=CARTESIAN_POINT('Origin',(6.65857864376269,0.300000000000001,-26.37)) ;
#151449=CARTESIAN_POINT('Origin',(6.9,0.0585786437626909,-26.7285786437627)) ;
#151450=CARTESIAN_POINT('Origin',(6.9,0.0585786437626909,-26.7285786437627)) ;
#151451=CARTESIAN_POINT('Origin',(6.9,0.0585786437626909,-26.7285786437627)) ;
#151452=CARTESIAN_POINT('Origin',(6.8057190958418,0.152859547920896,-26.5171404520791)) ;
#151453=CARTESIAN_POINT('Origin',(6.6585786437627,0.299999999999996,-26.37)) ;
#151454=CARTESIAN_POINT('Origin',(6.9,0.0585786437626908,-26.6114213562373)) ;
#151455=CARTESIAN_POINT('Origin',(6.9,0.0585786437626909,-26.27)) ;
#151456=CARTESIAN_POINT('Origin',(6.9,0.0585786437626909,-26.6114213562373)) ;
#151457=CARTESIAN_POINT('Origin',(6.9,-0.1,-26.7285786437627)) ;
#151458=CARTESIAN_POINT('Origin',(6.9,-0.0585786437626902,-26.7285786437627)) ;
#151459=CARTESIAN_POINT('Origin',(6.9,0.0585786437626909,-26.6114213562373)) ;
#151460=CARTESIAN_POINT('Origin',(6.9,0.058578643762691,-26.6114213562373)) ;
#151461=CARTESIAN_POINT('Origin',(6.9,-0.0585786437626909,-26.7285786437627)) ;
#151462=CARTESIAN_POINT('Origin',(6.9,-0.0585786437626907,-26.7285786437627)) ;
#151463=CARTESIAN_POINT('Origin',(6.9,-0.0585786437626909,-26.7285786437627)) ;
#151464=CARTESIAN_POINT('Origin',(6.9,-0.399999999999999,-26.6114213562373)) ;
#151465=CARTESIAN_POINT('Origin',(6.9,-0.0585786437626909,-26.6114213562373)) ;
#151466=CARTESIAN_POINT('Origin',(6.9,-0.0585786437626909,-26.27)) ;
#151467=CARTESIAN_POINT('Origin',(6.9,-0.058578643762691,-26.6114213562373)) ;
#151468=CARTESIAN_POINT('Origin',(6.87238576250846,-0.0861928812542304,
-26.7561928812542)) ;
#151469=CARTESIAN_POINT('Origin',(6.65857864376269,-0.3,-26.97)) ;
#151470=CARTESIAN_POINT('Origin',(6.9,-0.0585786437626909,-26.6114213562373)) ;
#151471=CARTESIAN_POINT('Origin',(6.9,-0.0585786437626907,-26.6114213562373)) ;
#151472=CARTESIAN_POINT('Origin',(6.65857864376269,-0.300000000000001,-26.27)) ;
#151473=CARTESIAN_POINT('Origin',(6.65857864376269,-0.300000000000001,-26.97)) ;
#151474=CARTESIAN_POINT('Origin',(6.65857864376269,-0.300000000000001,-26.37)) ;
#151475=CARTESIAN_POINT('Origin',(6.6057190958418,-0.352859547920896,-26.3171404520791)) ;
#151476=CARTESIAN_POINT('Origin',(6.65857864376269,-0.299999999999998,-26.37)) ;
#151477=CARTESIAN_POINT('Origin',(-0.113807118745769,-6.47238576250846,
-30.3661928812542)) ;
#151478=CARTESIAN_POINT('Origin',(0.300000000000001,-6.05857864376269,-30.78)) ;
#151479=CARTESIAN_POINT('Origin',(0.058578643762692,-6.3,-30.5385786437627)) ;
#151480=CARTESIAN_POINT('Origin',(0.3,-6.05857864376269,-30.08)) ;
#151481=CARTESIAN_POINT('Origin',(0.3,-6.05857864376269,-30.78)) ;
#151482=CARTESIAN_POINT('Origin',(0.3,-6.05857864376269,-30.18)) ;
#151483=CARTESIAN_POINT('Origin',(0.0585786437626908,-6.3,-30.5385786437627)) ;
#151484=CARTESIAN_POINT('Origin',(0.0585786437626908,-6.3,-30.5385786437627)) ;
#151485=CARTESIAN_POINT('Origin',(0.0585786437626908,-6.3,-30.5385786437627)) ;
#151486=CARTESIAN_POINT('Origin',(0.152859547920896,-6.2057190958418,-30.3271404520791)) ;
#151487=CARTESIAN_POINT('Origin',(0.299999999999995,-6.0585786437627,-30.18)) ;
#151488=CARTESIAN_POINT('Origin',(0.0585786437626908,-6.3,-30.4214213562373)) ;
#151489=CARTESIAN_POINT('Origin',(0.0585786437626908,-6.3,-30.08)) ;
#151490=CARTESIAN_POINT('Origin',(0.0585786437626908,-6.3,-30.4214213562373)) ;
#151491=CARTESIAN_POINT('Origin',(0.4,-6.3,-30.5385786437627)) ;
#151492=CARTESIAN_POINT('Origin',(-0.0585786437626899,-6.3,-30.5385786437627)) ;
#151493=CARTESIAN_POINT('Origin',(0.0585786437626908,-6.3,-30.4214213562373)) ;
#151494=CARTESIAN_POINT('Origin',(0.0585786437626916,-6.3,-30.4214213562373)) ;
#151495=CARTESIAN_POINT('Origin',(-0.0585786437626908,-6.3,-30.5385786437627)) ;
#151496=CARTESIAN_POINT('Origin',(-0.0585786437626905,-6.3,-30.5385786437627)) ;
#151497=CARTESIAN_POINT('Origin',(-0.0585786437626908,-6.3,-30.5385786437627)) ;
#151498=CARTESIAN_POINT('Origin',(-0.1,-6.3,-30.4214213562373)) ;
#151499=CARTESIAN_POINT('Origin',(-0.0585786437626908,-6.3,-30.4214213562373)) ;
#151500=CARTESIAN_POINT('Origin',(-0.0585786437626908,-6.3,-30.08)) ;
#151501=CARTESIAN_POINT('Origin',(-0.0585786437626908,-6.3,-30.4214213562373)) ;
#151502=CARTESIAN_POINT('Origin',(-0.0861928812542299,-6.27238576250846,
-30.5661928812542)) ;
#151503=CARTESIAN_POINT('Origin',(-0.299999999999999,-6.05857864376269,
-30.78)) ;
#151504=CARTESIAN_POINT('Origin',(-0.0585786437626908,-6.3,-30.4214213562373)) ;
#151505=CARTESIAN_POINT('Origin',(-0.0585786437626909,-6.3,-30.4214213562373)) ;
#151506=CARTESIAN_POINT('Origin',(-0.3,-6.05857864376269,-30.08)) ;
#151507=CARTESIAN_POINT('Origin',(-0.3,-6.05857864376269,-30.78)) ;
#151508=CARTESIAN_POINT('Origin',(-0.3,-6.05857864376269,-30.18)) ;
#151509=CARTESIAN_POINT('Origin',(-0.352859547920895,-6.00571909584179,
-30.1271404520791)) ;
#151510=CARTESIAN_POINT('Origin',(-0.299999999999997,-6.05857864376269,
-30.18)) ;
#151511=CARTESIAN_POINT('Origin',(7.07238576250846,-0.11380711874577,-30.3661928812542)) ;
#151512=CARTESIAN_POINT('Origin',(6.65857864376269,0.299999999999999,-30.78)) ;
#151513=CARTESIAN_POINT('Origin',(6.9,0.0585786437626903,-30.5385786437627)) ;
#151514=CARTESIAN_POINT('Origin',(6.65857864376269,0.300000000000001,-30.08)) ;
#151515=CARTESIAN_POINT('Origin',(6.65857864376269,0.300000000000001,-30.78)) ;
#151516=CARTESIAN_POINT('Origin',(6.65857864376269,0.300000000000001,-30.18)) ;
#151517=CARTESIAN_POINT('Origin',(6.9,0.0585786437626909,-30.5385786437627)) ;
#151518=CARTESIAN_POINT('Origin',(6.9,0.0585786437626909,-30.5385786437627)) ;
#151519=CARTESIAN_POINT('Origin',(6.9,0.0585786437626909,-30.5385786437627)) ;
#151520=CARTESIAN_POINT('Origin',(6.8057190958418,0.152859547920896,-30.3271404520791)) ;
#151521=CARTESIAN_POINT('Origin',(6.6585786437627,0.299999999999996,-30.18)) ;
#151522=CARTESIAN_POINT('Origin',(6.9,0.0585786437626908,-30.4214213562373)) ;
#151523=CARTESIAN_POINT('Origin',(6.9,0.0585786437626909,-30.08)) ;
#151524=CARTESIAN_POINT('Origin',(6.9,0.0585786437626909,-30.4214213562373)) ;
#151525=CARTESIAN_POINT('Origin',(6.9,-0.1,-30.5385786437627)) ;
#151526=CARTESIAN_POINT('Origin',(6.9,-0.0585786437626902,-30.5385786437627)) ;
#151527=CARTESIAN_POINT('Origin',(6.9,0.0585786437626909,-30.4214213562373)) ;
#151528=CARTESIAN_POINT('Origin',(6.9,0.058578643762691,-30.4214213562373)) ;
#151529=CARTESIAN_POINT('Origin',(6.9,-0.0585786437626909,-30.5385786437627)) ;
#151530=CARTESIAN_POINT('Origin',(6.9,-0.0585786437626907,-30.5385786437627)) ;
#151531=CARTESIAN_POINT('Origin',(6.9,-0.0585786437626909,-30.5385786437627)) ;
#151532=CARTESIAN_POINT('Origin',(6.9,-0.399999999999999,-30.4214213562373)) ;
#151533=CARTESIAN_POINT('Origin',(6.9,-0.0585786437626909,-30.4214213562373)) ;
#151534=CARTESIAN_POINT('Origin',(6.9,-0.0585786437626909,-30.08)) ;
#151535=CARTESIAN_POINT('Origin',(6.9,-0.058578643762691,-30.4214213562373)) ;
#151536=CARTESIAN_POINT('Origin',(6.87238576250846,-0.0861928812542304,
-30.5661928812542)) ;
#151537=CARTESIAN_POINT('Origin',(6.65857864376269,-0.3,-30.78)) ;
#151538=CARTESIAN_POINT('Origin',(6.9,-0.0585786437626909,-30.4214213562373)) ;
#151539=CARTESIAN_POINT('Origin',(6.9,-0.0585786437626907,-30.4214213562373)) ;
#151540=CARTESIAN_POINT('Origin',(6.65857864376269,-0.300000000000001,-30.08)) ;
#151541=CARTESIAN_POINT('Origin',(6.65857864376269,-0.300000000000001,-30.78)) ;
#151542=CARTESIAN_POINT('Origin',(6.65857864376269,-0.300000000000001,-30.18)) ;
#151543=CARTESIAN_POINT('Origin',(6.6057190958418,-0.352859547920896,-30.1271404520791)) ;
#151544=CARTESIAN_POINT('Origin',(6.65857864376269,-0.299999999999998,-30.18)) ;
#151545=CARTESIAN_POINT('Origin',(-0.113807118745771,-6.47238576250846,
-34.1761928812542)) ;
#151546=CARTESIAN_POINT('Origin',(0.299999999999993,-6.0585786437627,-34.59)) ;
#151547=CARTESIAN_POINT('Origin',(0.0585786437626844,-6.3,-34.3485786437627)) ;
#151548=CARTESIAN_POINT('Origin',(0.3,-6.05857864376269,-33.89)) ;
#151549=CARTESIAN_POINT('Origin',(0.3,-6.05857864376269,-34.59)) ;
#151550=CARTESIAN_POINT('Origin',(0.3,-6.05857864376269,-33.99)) ;
#151551=CARTESIAN_POINT('Origin',(0.0585786437626887,-6.3,-34.3485786437627)) ;
#151552=CARTESIAN_POINT('Origin',(0.0585786437626908,-6.3,-34.3485786437627)) ;
#151553=CARTESIAN_POINT('Origin',(0.0585786437626908,-6.3,-34.3485786437627)) ;
#151554=CARTESIAN_POINT('Origin',(0.152859547920899,-6.20571909584179,-34.1371404520791)) ;
#151555=CARTESIAN_POINT('Origin',(0.300000000000006,-6.05857864376268,-33.99)) ;
#151556=CARTESIAN_POINT('Origin',(0.0585786437626911,-6.3,-34.2314213562373)) ;
#151557=CARTESIAN_POINT('Origin',(0.0585786437626908,-6.3,-33.89)) ;
#151558=CARTESIAN_POINT('Origin',(0.0585786437626908,-6.3,-34.2314213562373)) ;
#151559=CARTESIAN_POINT('Origin',(0.4,-6.3,-34.3485786437627)) ;
#151560=CARTESIAN_POINT('Origin',(-0.0585786437626895,-6.3,-34.3485786437627)) ;
#151561=CARTESIAN_POINT('Origin',(0.0585786437626903,-6.3,-34.2314213562373)) ;
#151562=CARTESIAN_POINT('Origin',(0.058578643762689,-6.3,-34.2314213562373)) ;
#151563=CARTESIAN_POINT('Origin',(-0.0585786437626902,-6.3,-34.3485786437627)) ;
#151564=CARTESIAN_POINT('Origin',(-0.0585786437626905,-6.3,-34.3485786437627)) ;
#151565=CARTESIAN_POINT('Origin',(-0.0585786437626908,-6.3,-34.3485786437627)) ;
#151566=CARTESIAN_POINT('Origin',(-0.1,-6.3,-34.2314213562373)) ;
#151567=CARTESIAN_POINT('Origin',(-0.0585786437626908,-6.3,-34.2314213562373)) ;
#151568=CARTESIAN_POINT('Origin',(-0.0585786437626908,-6.3,-33.89)) ;
#151569=CARTESIAN_POINT('Origin',(-0.0585786437626908,-6.3,-34.2314213562373)) ;
#151570=CARTESIAN_POINT('Origin',(-0.0861928812542287,-6.27238576250846,
-34.3761928812542)) ;
#151571=CARTESIAN_POINT('Origin',(-0.299999999999994,-6.0585786437627,-34.59)) ;
#151572=CARTESIAN_POINT('Origin',(-0.0585786437626908,-6.3,-34.2314213562373)) ;
#151573=CARTESIAN_POINT('Origin',(-0.0585786437626846,-6.3,-34.2314213562373)) ;
#151574=CARTESIAN_POINT('Origin',(-0.3,-6.05857864376269,-33.89)) ;
#151575=CARTESIAN_POINT('Origin',(-0.3,-6.05857864376269,-34.59)) ;
#151576=CARTESIAN_POINT('Origin',(-0.3,-6.05857864376269,-33.99)) ;
#151577=CARTESIAN_POINT('Origin',(-0.352859547920899,-6.00571909584179,
-33.9371404520791)) ;
#151578=CARTESIAN_POINT('Origin',(-0.3,-6.05857864376269,-33.99)) ;
#151579=CARTESIAN_POINT('Origin',(7.07238576250846,-0.113807118745771,-34.1761928812542)) ;
#151580=CARTESIAN_POINT('Origin',(6.6585786437627,0.299999999999994,-34.59)) ;
#151581=CARTESIAN_POINT('Origin',(6.9,0.0585786437626901,-34.3485786437627)) ;
#151582=CARTESIAN_POINT('Origin',(6.65857864376269,0.300000000000001,-33.89)) ;
#151583=CARTESIAN_POINT('Origin',(6.65857864376269,0.300000000000001,-34.59)) ;
#151584=CARTESIAN_POINT('Origin',(6.65857864376269,0.300000000000001,-33.99)) ;
#151585=CARTESIAN_POINT('Origin',(6.9,0.0585786437626906,-34.3485786437627)) ;
#151586=CARTESIAN_POINT('Origin',(6.9,0.0585786437626909,-34.3485786437627)) ;
#151587=CARTESIAN_POINT('Origin',(6.9,0.0585786437626909,-34.3485786437627)) ;
#151588=CARTESIAN_POINT('Origin',(6.80571909584179,0.1528595479209,-34.1371404520791)) ;
#151589=CARTESIAN_POINT('Origin',(6.65857864376268,0.300000000000007,-33.99)) ;
#151590=CARTESIAN_POINT('Origin',(6.9,0.0585786437626911,-34.2314213562373)) ;
#151591=CARTESIAN_POINT('Origin',(6.9,0.0585786437626909,-33.89)) ;
#151592=CARTESIAN_POINT('Origin',(6.9,0.0585786437626909,-34.2314213562373)) ;
#151593=CARTESIAN_POINT('Origin',(6.9,-0.1,-34.3485786437627)) ;
#151594=CARTESIAN_POINT('Origin',(6.9,-0.0585786437626952,-34.3485786437627)) ;
#151595=CARTESIAN_POINT('Origin',(6.9,0.0585786437626913,-34.2314213562373)) ;
#151596=CARTESIAN_POINT('Origin',(6.9,0.0585786437626919,-34.2314213562373)) ;
#151597=CARTESIAN_POINT('Origin',(6.9,-0.0585786437626923,-34.3485786437627)) ;
#151598=CARTESIAN_POINT('Origin',(6.9,-0.0585786437626907,-34.3485786437627)) ;
#151599=CARTESIAN_POINT('Origin',(6.9,-0.0585786437626909,-34.3485786437627)) ;
#151600=CARTESIAN_POINT('Origin',(6.9,-0.399999999999999,-34.2314213562373)) ;
#151601=CARTESIAN_POINT('Origin',(6.9,-0.0585786437626909,-34.2314213562373)) ;
#151602=CARTESIAN_POINT('Origin',(6.9,-0.0585786437626909,-33.89)) ;
#151603=CARTESIAN_POINT('Origin',(6.9,-0.058578643762691,-34.2314213562373)) ;
#151604=CARTESIAN_POINT('Origin',(6.87238576250846,-0.0861928812542292,
-34.3761928812542)) ;
#151605=CARTESIAN_POINT('Origin',(6.6585786437627,-0.299999999999995,-34.59)) ;
#151606=CARTESIAN_POINT('Origin',(6.9,-0.0585786437626886,-34.2314213562373)) ;
#151607=CARTESIAN_POINT('Origin',(6.9,-0.058578643762684,-34.2314213562373)) ;
#151608=CARTESIAN_POINT('Origin',(6.65857864376269,-0.300000000000001,-33.89)) ;
#151609=CARTESIAN_POINT('Origin',(6.65857864376269,-0.300000000000001,-34.59)) ;
#151610=CARTESIAN_POINT('Origin',(6.65857864376269,-0.300000000000001,-33.99)) ;
#151611=CARTESIAN_POINT('Origin',(6.60571909584179,-0.3528595479209,-33.9371404520791)) ;
#151612=CARTESIAN_POINT('Origin',(6.65857864376269,-0.300000000000001,-33.99)) ;
#151613=CARTESIAN_POINT('Origin',(0.6,-0.6,-4.11)) ;
#151614=CARTESIAN_POINT('Origin',(0.3,-0.6,-4.11)) ;
#151615=CARTESIAN_POINT('Origin',(0.3,-6.1,-4.11)) ;
#151616=CARTESIAN_POINT('Origin',(0.3,-6.05857864376269,-4.11)) ;
#151617=CARTESIAN_POINT('Origin',(0.3,-6.05857864376269,-4.11)) ;
#151618=CARTESIAN_POINT('Origin',(0.3,-6.05857864376269,-4.11)) ;
#151619=CARTESIAN_POINT('Origin',(0.4,-6.05857864376269,-4.11)) ;
#151620=CARTESIAN_POINT('Origin',(-0.300000000000001,-6.05857864376269,
-4.11)) ;
#151621=CARTESIAN_POINT('Origin',(-0.3,-6.05857864376269,-4.11)) ;
#151622=CARTESIAN_POINT('Origin',(-0.3,-6.05857864376269,-4.11)) ;
#151623=CARTESIAN_POINT('Origin',(-0.3,-0.600000000000001,-4.11)) ;
#151624=CARTESIAN_POINT('Origin',(-0.3,-0.600000000000001,-4.11)) ;
#151625=CARTESIAN_POINT('Origin',(0.6,-0.600000000000001,-4.11)) ;
#151626=CARTESIAN_POINT('Origin',(0.6,-0.600000000000001,-3.51)) ;
#151627=CARTESIAN_POINT('Origin',(-0.3,-0.600000000000001,-3.51)) ;
#151628=CARTESIAN_POINT('Origin',(-0.3,-0.600000000000001,-3.51)) ;
#151629=CARTESIAN_POINT('Origin',(-0.3,-6.05857864376269,-3.51)) ;
#151630=CARTESIAN_POINT('Origin',(-0.3,-6.05857864376269,-3.51)) ;
#151631=CARTESIAN_POINT('Origin',(-0.299999999999999,-6.05857864376269,
-3.51)) ;
#151632=CARTESIAN_POINT('Origin',(0.4,-6.05857864376269,-3.51)) ;
#151633=CARTESIAN_POINT('Origin',(0.299999999999999,-6.05857864376269,-3.51)) ;
#151634=CARTESIAN_POINT('Origin',(0.3,-6.05857864376269,-3.51)) ;
#151635=CARTESIAN_POINT('Origin',(0.3,-6.05857864376269,-3.51)) ;
#151636=CARTESIAN_POINT('Origin',(0.3,-0.600000000000001,-3.51)) ;
#151637=CARTESIAN_POINT('Origin',(0.3,-0.6,-3.51)) ;
#151638=CARTESIAN_POINT('Origin',(0.6,-0.6,-3.51)) ;
#151639=CARTESIAN_POINT('Origin',(6.7,0.300000000000001,-4.11)) ;
#151640=CARTESIAN_POINT('Origin',(6.65857864376269,0.300000000000001,-4.11)) ;
#151641=CARTESIAN_POINT('Origin',(6.65857864376269,0.300000000000001,-4.11)) ;
#151642=CARTESIAN_POINT('Origin',(6.65857864376269,0.300000000000001,-4.11)) ;
#151643=CARTESIAN_POINT('Origin',(6.65857864376269,-0.399999999999999,-4.11)) ;
#151644=CARTESIAN_POINT('Origin',(6.65857864376269,-0.300000000000001,-4.11)) ;
#151645=CARTESIAN_POINT('Origin',(6.65857864376269,-0.3,-4.11)) ;
#151646=CARTESIAN_POINT('Origin',(6.65857864376269,-0.300000000000001,-4.11)) ;
#151647=CARTESIAN_POINT('Origin',(0.6,-0.3,-4.11)) ;
#151648=CARTESIAN_POINT('Origin',(0.6,0.299999999999999,-3.51)) ;
#151649=CARTESIAN_POINT('Origin',(6.65857864376269,0.300000000000001,-3.51)) ;
#151650=CARTESIAN_POINT('Origin',(6.65857864376269,0.300000000000001,-3.51)) ;
#151651=CARTESIAN_POINT('Origin',(6.65857864376269,0.3,-3.51)) ;
#151652=CARTESIAN_POINT('Origin',(6.65857864376269,-0.399999999999999,-3.51)) ;
#151653=CARTESIAN_POINT('Origin',(6.65857864376269,-0.3,-3.51)) ;
#151654=CARTESIAN_POINT('Origin',(0.6,-0.3,-3.51)) ;
#151655=CARTESIAN_POINT('Origin',(6.65857864376269,-0.300000000000001,-3.51)) ;
#151656=CARTESIAN_POINT('Origin',(6.65857864376269,-0.300000000000001,-3.51)) ;
#151657=CARTESIAN_POINT('Origin',(0.6,-0.6,-7.92)) ;
#151658=CARTESIAN_POINT('Origin',(0.3,-0.6,-7.92)) ;
#151659=CARTESIAN_POINT('Origin',(0.3,-6.1,-7.92)) ;
#151660=CARTESIAN_POINT('Origin',(0.3,-6.05857864376269,-7.92)) ;
#151661=CARTESIAN_POINT('Origin',(0.3,-6.05857864376269,-7.92)) ;
#151662=CARTESIAN_POINT('Origin',(0.3,-6.05857864376269,-7.92)) ;
#151663=CARTESIAN_POINT('Origin',(0.4,-6.05857864376269,-7.92)) ;
#151664=CARTESIAN_POINT('Origin',(-0.299999999999999,-6.05857864376269,
-7.92)) ;
#151665=CARTESIAN_POINT('Origin',(-0.3,-6.05857864376269,-7.92)) ;
#151666=CARTESIAN_POINT('Origin',(-0.3,-6.05857864376269,-7.92)) ;
#151667=CARTESIAN_POINT('Origin',(-0.3,-0.600000000000001,-7.92)) ;
#151668=CARTESIAN_POINT('Origin',(-0.3,-0.600000000000001,-7.92)) ;
#151669=CARTESIAN_POINT('Origin',(0.6,-0.600000000000001,-7.92)) ;
#151670=CARTESIAN_POINT('Origin',(0.6,-0.600000000000001,-7.32)) ;
#151671=CARTESIAN_POINT('Origin',(-0.3,-0.600000000000001,-7.32)) ;
#151672=CARTESIAN_POINT('Origin',(-0.3,-0.600000000000001,-7.32)) ;
#151673=CARTESIAN_POINT('Origin',(-0.3,-6.05857864376269,-7.32)) ;
#151674=CARTESIAN_POINT('Origin',(-0.3,-6.05857864376269,-7.32)) ;
#151675=CARTESIAN_POINT('Origin',(-0.300000000000001,-6.05857864376269,
-7.32)) ;
#151676=CARTESIAN_POINT('Origin',(0.4,-6.05857864376269,-7.32)) ;
#151677=CARTESIAN_POINT('Origin',(0.300000000000002,-6.05857864376269,-7.32)) ;
#151678=CARTESIAN_POINT('Origin',(0.300000000000001,-6.05857864376269,-7.32)) ;
#151679=CARTESIAN_POINT('Origin',(0.3,-6.05857864376269,-7.32)) ;
#151680=CARTESIAN_POINT('Origin',(0.3,-0.600000000000001,-7.32)) ;
#151681=CARTESIAN_POINT('Origin',(0.3,-0.6,-7.32)) ;
#151682=CARTESIAN_POINT('Origin',(0.6,-0.6,-7.32)) ;
#151683=CARTESIAN_POINT('Origin',(6.7,0.300000000000001,-7.92)) ;
#151684=CARTESIAN_POINT('Origin',(6.65857864376269,0.300000000000001,-7.92)) ;
#151685=CARTESIAN_POINT('Origin',(6.65857864376269,0.300000000000001,-7.92)) ;
#151686=CARTESIAN_POINT('Origin',(6.65857864376269,0.300000000000002,-7.92)) ;
#151687=CARTESIAN_POINT('Origin',(6.65857864376269,-0.399999999999999,-7.92)) ;
#151688=CARTESIAN_POINT('Origin',(6.65857864376269,-0.300000000000002,-7.92)) ;
#151689=CARTESIAN_POINT('Origin',(6.65857864376269,-0.300000000000001,-7.92)) ;
#151690=CARTESIAN_POINT('Origin',(6.65857864376269,-0.300000000000001,-7.92)) ;
#151691=CARTESIAN_POINT('Origin',(0.6,-0.3,-7.92)) ;
#151692=CARTESIAN_POINT('Origin',(0.6,0.299999999999999,-7.32)) ;
#151693=CARTESIAN_POINT('Origin',(6.65857864376269,0.300000000000001,-7.32)) ;
#151694=CARTESIAN_POINT('Origin',(6.65857864376269,0.300000000000001,-7.32)) ;
#151695=CARTESIAN_POINT('Origin',(6.65857864376269,0.300000000000002,-7.32)) ;
#151696=CARTESIAN_POINT('Origin',(6.65857864376269,-0.399999999999999,-7.32)) ;
#151697=CARTESIAN_POINT('Origin',(6.65857864376269,-0.300000000000002,-7.32)) ;
#151698=CARTESIAN_POINT('Origin',(0.6,-0.3,-7.32)) ;
#151699=CARTESIAN_POINT('Origin',(6.65857864376269,-0.300000000000001,-7.32)) ;
#151700=CARTESIAN_POINT('Origin',(6.65857864376269,-0.300000000000001,-7.32)) ;
#151701=CARTESIAN_POINT('Origin',(0.6,-0.6,-11.73)) ;
#151702=CARTESIAN_POINT('Origin',(0.3,-0.6,-11.73)) ;
#151703=CARTESIAN_POINT('Origin',(0.3,-6.1,-11.73)) ;
#151704=CARTESIAN_POINT('Origin',(0.3,-6.05857864376269,-11.73)) ;
#151705=CARTESIAN_POINT('Origin',(0.3,-6.05857864376269,-11.73)) ;
#151706=CARTESIAN_POINT('Origin',(0.299999999999998,-6.05857864376269,-11.73)) ;
#151707=CARTESIAN_POINT('Origin',(0.4,-6.05857864376269,-11.73)) ;
#151708=CARTESIAN_POINT('Origin',(-0.299999999999999,-6.05857864376269,
-11.73)) ;
#151709=CARTESIAN_POINT('Origin',(-0.3,-6.05857864376269,-11.73)) ;
#151710=CARTESIAN_POINT('Origin',(-0.3,-6.05857864376269,-11.73)) ;
#151711=CARTESIAN_POINT('Origin',(-0.3,-0.600000000000001,-11.73)) ;
#151712=CARTESIAN_POINT('Origin',(-0.3,-0.600000000000001,-11.73)) ;
#151713=CARTESIAN_POINT('Origin',(0.6,-0.600000000000001,-11.73)) ;
#151714=CARTESIAN_POINT('Origin',(0.6,-0.600000000000001,-11.13)) ;
#151715=CARTESIAN_POINT('Origin',(-0.3,-0.600000000000001,-11.13)) ;
#151716=CARTESIAN_POINT('Origin',(-0.3,-0.600000000000001,-11.13)) ;
#151717=CARTESIAN_POINT('Origin',(-0.3,-6.05857864376269,-11.13)) ;
#151718=CARTESIAN_POINT('Origin',(-0.3,-6.05857864376269,-11.13)) ;
#151719=CARTESIAN_POINT('Origin',(-0.300000000000002,-6.05857864376269,
-11.13)) ;
#151720=CARTESIAN_POINT('Origin',(0.4,-6.05857864376269,-11.13)) ;
#151721=CARTESIAN_POINT('Origin',(0.300000000000001,-6.05857864376269,-11.13)) ;
#151722=CARTESIAN_POINT('Origin',(0.300000000000003,-6.05857864376269,-11.13)) ;
#151723=CARTESIAN_POINT('Origin',(0.3,-6.05857864376269,-11.13)) ;
#151724=CARTESIAN_POINT('Origin',(0.3,-0.600000000000001,-11.13)) ;
#151725=CARTESIAN_POINT('Origin',(0.3,-0.6,-11.13)) ;
#151726=CARTESIAN_POINT('Origin',(0.6,-0.6,-11.13)) ;
#151727=CARTESIAN_POINT('Origin',(6.7,0.300000000000001,-11.73)) ;
#151728=CARTESIAN_POINT('Origin',(6.65857864376269,0.300000000000001,-11.73)) ;
#151729=CARTESIAN_POINT('Origin',(6.65857864376269,0.300000000000001,-11.73)) ;
#151730=CARTESIAN_POINT('Origin',(6.65857864376269,0.300000000000001,-11.73)) ;
#151731=CARTESIAN_POINT('Origin',(6.65857864376269,-0.399999999999999,-11.73)) ;
#151732=CARTESIAN_POINT('Origin',(6.65857864376269,-0.300000000000002,-11.73)) ;
#151733=CARTESIAN_POINT('Origin',(6.65857864376269,-0.300000000000002,-11.73)) ;
#151734=CARTESIAN_POINT('Origin',(6.65857864376269,-0.300000000000001,-11.73)) ;
#151735=CARTESIAN_POINT('Origin',(0.6,-0.3,-11.73)) ;
#151736=CARTESIAN_POINT('Origin',(0.6,0.299999999999999,-11.13)) ;
#151737=CARTESIAN_POINT('Origin',(6.65857864376269,0.300000000000001,-11.13)) ;
#151738=CARTESIAN_POINT('Origin',(6.65857864376269,0.300000000000001,-11.13)) ;
#151739=CARTESIAN_POINT('Origin',(6.65857864376269,0.300000000000001,-11.13)) ;
#151740=CARTESIAN_POINT('Origin',(6.65857864376269,-0.399999999999999,-11.13)) ;
#151741=CARTESIAN_POINT('Origin',(6.65857864376269,-0.300000000000002,-11.13)) ;
#151742=CARTESIAN_POINT('Origin',(0.6,-0.3,-11.13)) ;
#151743=CARTESIAN_POINT('Origin',(6.65857864376269,-0.300000000000001,-11.13)) ;
#151744=CARTESIAN_POINT('Origin',(6.65857864376269,-0.300000000000003,-11.13)) ;
#151745=CARTESIAN_POINT('Origin',(0.6,-0.6,-15.54)) ;
#151746=CARTESIAN_POINT('Origin',(0.3,-0.6,-15.54)) ;
#151747=CARTESIAN_POINT('Origin',(0.3,-6.1,-15.54)) ;
#151748=CARTESIAN_POINT('Origin',(0.3,-6.05857864376269,-15.54)) ;
#151749=CARTESIAN_POINT('Origin',(0.3,-6.05857864376269,-15.54)) ;
#151750=CARTESIAN_POINT('Origin',(0.3,-6.05857864376269,-15.54)) ;
#151751=CARTESIAN_POINT('Origin',(0.4,-6.05857864376269,-15.54)) ;
#151752=CARTESIAN_POINT('Origin',(-0.299999999999999,-6.05857864376269,
-15.54)) ;
#151753=CARTESIAN_POINT('Origin',(-0.300000000000001,-6.05857864376269,
-15.54)) ;
#151754=CARTESIAN_POINT('Origin',(-0.3,-6.05857864376269,-15.54)) ;
#151755=CARTESIAN_POINT('Origin',(-0.3,-0.600000000000001,-15.54)) ;
#151756=CARTESIAN_POINT('Origin',(-0.3,-0.600000000000001,-15.54)) ;
#151757=CARTESIAN_POINT('Origin',(0.6,-0.600000000000001,-15.54)) ;
#151758=CARTESIAN_POINT('Origin',(0.6,-0.600000000000001,-14.94)) ;
#151759=CARTESIAN_POINT('Origin',(-0.3,-0.600000000000001,-14.94)) ;
#151760=CARTESIAN_POINT('Origin',(-0.3,-0.600000000000001,-14.94)) ;
#151761=CARTESIAN_POINT('Origin',(-0.3,-6.05857864376269,-14.94)) ;
#151762=CARTESIAN_POINT('Origin',(-0.3,-6.05857864376269,-14.94)) ;
#151763=CARTESIAN_POINT('Origin',(-0.3,-6.05857864376269,-14.94)) ;
#151764=CARTESIAN_POINT('Origin',(0.4,-6.05857864376269,-14.94)) ;
#151765=CARTESIAN_POINT('Origin',(0.299999999999999,-6.05857864376269,-14.94)) ;
#151766=CARTESIAN_POINT('Origin',(0.300000000000001,-6.05857864376269,-14.94)) ;
#151767=CARTESIAN_POINT('Origin',(0.3,-6.05857864376269,-14.94)) ;
#151768=CARTESIAN_POINT('Origin',(0.3,-0.600000000000001,-14.94)) ;
#151769=CARTESIAN_POINT('Origin',(0.3,-0.6,-14.94)) ;
#151770=CARTESIAN_POINT('Origin',(0.6,-0.6,-14.94)) ;
#151771=CARTESIAN_POINT('Origin',(6.7,0.300000000000001,-15.54)) ;
#151772=CARTESIAN_POINT('Origin',(6.65857864376269,0.300000000000001,-15.54)) ;
#151773=CARTESIAN_POINT('Origin',(6.65857864376269,0.300000000000001,-15.54)) ;
#151774=CARTESIAN_POINT('Origin',(6.65857864376269,0.300000000000003,-15.54)) ;
#151775=CARTESIAN_POINT('Origin',(6.65857864376269,-0.399999999999999,-15.54)) ;
#151776=CARTESIAN_POINT('Origin',(6.65857864376269,-0.3,-15.54)) ;
#151777=CARTESIAN_POINT('Origin',(6.65857864376269,-0.300000000000002,-15.54)) ;
#151778=CARTESIAN_POINT('Origin',(6.65857864376269,-0.300000000000001,-15.54)) ;
#151779=CARTESIAN_POINT('Origin',(0.6,-0.3,-15.54)) ;
#151780=CARTESIAN_POINT('Origin',(0.6,0.299999999999999,-14.94)) ;
#151781=CARTESIAN_POINT('Origin',(6.65857864376269,0.300000000000001,-14.94)) ;
#151782=CARTESIAN_POINT('Origin',(6.65857864376269,0.300000000000001,-14.94)) ;
#151783=CARTESIAN_POINT('Origin',(6.65857864376269,0.3,-14.94)) ;
#151784=CARTESIAN_POINT('Origin',(6.65857864376269,-0.399999999999999,-14.94)) ;
#151785=CARTESIAN_POINT('Origin',(6.65857864376269,-0.299999999999999,-14.94)) ;
#151786=CARTESIAN_POINT('Origin',(0.6,-0.3,-14.94)) ;
#151787=CARTESIAN_POINT('Origin',(6.65857864376269,-0.300000000000001,-14.94)) ;
#151788=CARTESIAN_POINT('Origin',(6.65857864376269,-0.300000000000001,-14.94)) ;
#151789=CARTESIAN_POINT('Origin',(0.6,-0.6,-19.35)) ;
#151790=CARTESIAN_POINT('Origin',(0.3,-0.6,-19.35)) ;
#151791=CARTESIAN_POINT('Origin',(0.3,-6.1,-19.35)) ;
#151792=CARTESIAN_POINT('Origin',(0.3,-6.05857864376269,-19.35)) ;
#151793=CARTESIAN_POINT('Origin',(0.3,-6.05857864376269,-19.35)) ;
#151794=CARTESIAN_POINT('Origin',(0.299999999999999,-6.05857864376269,-19.35)) ;
#151795=CARTESIAN_POINT('Origin',(0.4,-6.05857864376269,-19.35)) ;
#151796=CARTESIAN_POINT('Origin',(-0.299999999999994,-6.0585786437627,-19.35)) ;
#151797=CARTESIAN_POINT('Origin',(-0.299999999999999,-6.05857864376269,
-19.35)) ;
#151798=CARTESIAN_POINT('Origin',(-0.3,-6.05857864376269,-19.35)) ;
#151799=CARTESIAN_POINT('Origin',(-0.3,-0.600000000000001,-19.35)) ;
#151800=CARTESIAN_POINT('Origin',(-0.3,-0.600000000000001,-19.35)) ;
#151801=CARTESIAN_POINT('Origin',(0.6,-0.600000000000001,-19.35)) ;
#151802=CARTESIAN_POINT('Origin',(0.6,-0.600000000000001,-18.75)) ;
#151803=CARTESIAN_POINT('Origin',(-0.3,-0.600000000000001,-18.75)) ;
#151804=CARTESIAN_POINT('Origin',(-0.3,-0.600000000000001,-18.75)) ;
#151805=CARTESIAN_POINT('Origin',(-0.3,-6.05857864376269,-18.75)) ;
#151806=CARTESIAN_POINT('Origin',(-0.3,-6.05857864376269,-18.75)) ;
#151807=CARTESIAN_POINT('Origin',(-0.299999999999994,-6.0585786437627,-18.75)) ;
#151808=CARTESIAN_POINT('Origin',(0.4,-6.0585786437627,-18.75)) ;
#151809=CARTESIAN_POINT('Origin',(0.299999999999993,-6.0585786437627,-18.75)) ;
#151810=CARTESIAN_POINT('Origin',(0.299999999999996,-6.0585786437627,-18.75)) ;
#151811=CARTESIAN_POINT('Origin',(0.3,-6.05857864376269,-18.75)) ;
#151812=CARTESIAN_POINT('Origin',(0.3,-0.600000000000001,-18.75)) ;
#151813=CARTESIAN_POINT('Origin',(0.3,-0.6,-18.75)) ;
#151814=CARTESIAN_POINT('Origin',(0.6,-0.6,-18.75)) ;
#151815=CARTESIAN_POINT('Origin',(6.7,0.300000000000001,-19.35)) ;
#151816=CARTESIAN_POINT('Origin',(6.65857864376269,0.300000000000001,-19.35)) ;
#151817=CARTESIAN_POINT('Origin',(6.65857864376269,0.300000000000001,-19.35)) ;
#151818=CARTESIAN_POINT('Origin',(6.65857864376269,0.299999999999997,-19.35)) ;
#151819=CARTESIAN_POINT('Origin',(6.65857864376269,-0.399999999999999,-19.35)) ;
#151820=CARTESIAN_POINT('Origin',(6.65857864376269,-0.299999999999997,-19.35)) ;
#151821=CARTESIAN_POINT('Origin',(6.65857864376269,-0.3,-19.35)) ;
#151822=CARTESIAN_POINT('Origin',(6.65857864376269,-0.300000000000001,-19.35)) ;
#151823=CARTESIAN_POINT('Origin',(0.6,-0.3,-19.35)) ;
#151824=CARTESIAN_POINT('Origin',(0.6,0.299999999999999,-18.75)) ;
#151825=CARTESIAN_POINT('Origin',(6.65857864376269,0.300000000000001,-18.75)) ;
#151826=CARTESIAN_POINT('Origin',(6.65857864376269,0.300000000000001,-18.75)) ;
#151827=CARTESIAN_POINT('Origin',(6.6585786437627,0.299999999999995,-18.75)) ;
#151828=CARTESIAN_POINT('Origin',(6.6585786437627,-0.399999999999999,-18.75)) ;
#151829=CARTESIAN_POINT('Origin',(6.6585786437627,-0.299999999999994,-18.75)) ;
#151830=CARTESIAN_POINT('Origin',(0.6,-0.3,-18.75)) ;
#151831=CARTESIAN_POINT('Origin',(6.65857864376269,-0.300000000000001,-18.75)) ;
#151832=CARTESIAN_POINT('Origin',(6.65857864376269,-0.299999999999998,-18.75)) ;
#151833=CARTESIAN_POINT('Origin',(0.6,-0.6,-23.16)) ;
#151834=CARTESIAN_POINT('Origin',(0.3,-0.6,-23.16)) ;
#151835=CARTESIAN_POINT('Origin',(0.3,-6.1,-23.16)) ;
#151836=CARTESIAN_POINT('Origin',(0.3,-6.05857864376269,-23.16)) ;
#151837=CARTESIAN_POINT('Origin',(0.3,-6.05857864376269,-23.16)) ;
#151838=CARTESIAN_POINT('Origin',(0.299999999999999,-6.05857864376269,-23.16)) ;
#151839=CARTESIAN_POINT('Origin',(0.4,-6.05857864376269,-23.16)) ;
#151840=CARTESIAN_POINT('Origin',(-0.299999999999994,-6.0585786437627,-23.16)) ;
#151841=CARTESIAN_POINT('Origin',(-0.299999999999999,-6.05857864376269,
-23.16)) ;
#151842=CARTESIAN_POINT('Origin',(-0.3,-6.05857864376269,-23.16)) ;
#151843=CARTESIAN_POINT('Origin',(-0.3,-0.600000000000001,-23.16)) ;
#151844=CARTESIAN_POINT('Origin',(-0.3,-0.600000000000001,-23.16)) ;
#151845=CARTESIAN_POINT('Origin',(0.6,-0.600000000000001,-23.16)) ;
#151846=CARTESIAN_POINT('Origin',(0.6,-0.600000000000001,-22.56)) ;
#151847=CARTESIAN_POINT('Origin',(-0.3,-0.600000000000001,-22.56)) ;
#151848=CARTESIAN_POINT('Origin',(-0.3,-0.600000000000001,-22.56)) ;
#151849=CARTESIAN_POINT('Origin',(-0.3,-6.05857864376269,-22.56)) ;
#151850=CARTESIAN_POINT('Origin',(-0.3,-6.05857864376269,-22.56)) ;
#151851=CARTESIAN_POINT('Origin',(-0.299999999999994,-6.0585786437627,-22.56)) ;
#151852=CARTESIAN_POINT('Origin',(0.4,-6.0585786437627,-22.56)) ;
#151853=CARTESIAN_POINT('Origin',(0.299999999999993,-6.0585786437627,-22.56)) ;
#151854=CARTESIAN_POINT('Origin',(0.299999999999996,-6.0585786437627,-22.56)) ;
#151855=CARTESIAN_POINT('Origin',(0.3,-6.05857864376269,-22.56)) ;
#151856=CARTESIAN_POINT('Origin',(0.3,-0.600000000000001,-22.56)) ;
#151857=CARTESIAN_POINT('Origin',(0.3,-0.6,-22.56)) ;
#151858=CARTESIAN_POINT('Origin',(0.6,-0.6,-22.56)) ;
#151859=CARTESIAN_POINT('Origin',(6.7,0.300000000000001,-23.16)) ;
#151860=CARTESIAN_POINT('Origin',(6.65857864376269,0.300000000000001,-23.16)) ;
#151861=CARTESIAN_POINT('Origin',(6.65857864376269,0.300000000000001,-23.16)) ;
#151862=CARTESIAN_POINT('Origin',(6.65857864376269,0.299999999999997,-23.16)) ;
#151863=CARTESIAN_POINT('Origin',(6.65857864376269,-0.399999999999999,-23.16)) ;
#151864=CARTESIAN_POINT('Origin',(6.65857864376269,-0.299999999999997,-23.16)) ;
#151865=CARTESIAN_POINT('Origin',(6.65857864376269,-0.3,-23.16)) ;
#151866=CARTESIAN_POINT('Origin',(6.65857864376269,-0.300000000000001,-23.16)) ;
#151867=CARTESIAN_POINT('Origin',(0.6,-0.3,-23.16)) ;
#151868=CARTESIAN_POINT('Origin',(0.6,0.299999999999999,-22.56)) ;
#151869=CARTESIAN_POINT('Origin',(6.65857864376269,0.300000000000001,-22.56)) ;
#151870=CARTESIAN_POINT('Origin',(6.65857864376269,0.300000000000001,-22.56)) ;
#151871=CARTESIAN_POINT('Origin',(6.6585786437627,0.299999999999995,-22.56)) ;
#151872=CARTESIAN_POINT('Origin',(6.6585786437627,-0.399999999999999,-22.56)) ;
#151873=CARTESIAN_POINT('Origin',(6.6585786437627,-0.299999999999994,-22.56)) ;
#151874=CARTESIAN_POINT('Origin',(0.6,-0.3,-22.56)) ;
#151875=CARTESIAN_POINT('Origin',(6.65857864376269,-0.300000000000001,-22.56)) ;
#151876=CARTESIAN_POINT('Origin',(6.65857864376269,-0.299999999999998,-22.56)) ;
#151877=CARTESIAN_POINT('Origin',(0.6,-0.6,-26.97)) ;
#151878=CARTESIAN_POINT('Origin',(0.3,-0.6,-26.97)) ;
#151879=CARTESIAN_POINT('Origin',(0.3,-6.1,-26.97)) ;
#151880=CARTESIAN_POINT('Origin',(0.3,-6.05857864376269,-26.97)) ;
#151881=CARTESIAN_POINT('Origin',(0.3,-6.05857864376269,-26.97)) ;
#151882=CARTESIAN_POINT('Origin',(0.299999999999999,-6.05857864376269,-26.97)) ;
#151883=CARTESIAN_POINT('Origin',(0.4,-6.05857864376269,-26.97)) ;
#151884=CARTESIAN_POINT('Origin',(-0.299999999999994,-6.0585786437627,-26.97)) ;
#151885=CARTESIAN_POINT('Origin',(-0.299999999999999,-6.05857864376269,
-26.97)) ;
#151886=CARTESIAN_POINT('Origin',(-0.3,-6.05857864376269,-26.97)) ;
#151887=CARTESIAN_POINT('Origin',(-0.3,-0.600000000000001,-26.97)) ;
#151888=CARTESIAN_POINT('Origin',(-0.3,-0.600000000000001,-26.97)) ;
#151889=CARTESIAN_POINT('Origin',(0.6,-0.600000000000001,-26.97)) ;
#151890=CARTESIAN_POINT('Origin',(0.6,-0.600000000000001,-26.37)) ;
#151891=CARTESIAN_POINT('Origin',(-0.3,-0.600000000000001,-26.37)) ;
#151892=CARTESIAN_POINT('Origin',(-0.3,-0.600000000000001,-26.37)) ;
#151893=CARTESIAN_POINT('Origin',(-0.3,-6.05857864376269,-26.37)) ;
#151894=CARTESIAN_POINT('Origin',(-0.3,-6.05857864376269,-26.37)) ;
#151895=CARTESIAN_POINT('Origin',(-0.299999999999994,-6.0585786437627,-26.37)) ;
#151896=CARTESIAN_POINT('Origin',(0.4,-6.0585786437627,-26.37)) ;
#151897=CARTESIAN_POINT('Origin',(0.299999999999993,-6.0585786437627,-26.37)) ;
#151898=CARTESIAN_POINT('Origin',(0.299999999999996,-6.0585786437627,-26.37)) ;
#151899=CARTESIAN_POINT('Origin',(0.3,-6.05857864376269,-26.37)) ;
#151900=CARTESIAN_POINT('Origin',(0.3,-0.600000000000001,-26.37)) ;
#151901=CARTESIAN_POINT('Origin',(0.3,-0.6,-26.37)) ;
#151902=CARTESIAN_POINT('Origin',(0.6,-0.6,-26.37)) ;
#151903=CARTESIAN_POINT('Origin',(6.7,0.300000000000001,-26.97)) ;
#151904=CARTESIAN_POINT('Origin',(6.65857864376269,0.300000000000001,-26.97)) ;
#151905=CARTESIAN_POINT('Origin',(6.65857864376269,0.300000000000001,-26.97)) ;
#151906=CARTESIAN_POINT('Origin',(6.65857864376269,0.299999999999997,-26.97)) ;
#151907=CARTESIAN_POINT('Origin',(6.65857864376269,-0.399999999999999,-26.97)) ;
#151908=CARTESIAN_POINT('Origin',(6.65857864376269,-0.299999999999997,-26.97)) ;
#151909=CARTESIAN_POINT('Origin',(6.65857864376269,-0.3,-26.97)) ;
#151910=CARTESIAN_POINT('Origin',(6.65857864376269,-0.300000000000001,-26.97)) ;
#151911=CARTESIAN_POINT('Origin',(0.6,-0.3,-26.97)) ;
#151912=CARTESIAN_POINT('Origin',(0.6,0.299999999999999,-26.37)) ;
#151913=CARTESIAN_POINT('Origin',(6.65857864376269,0.300000000000001,-26.37)) ;
#151914=CARTESIAN_POINT('Origin',(6.65857864376269,0.300000000000001,-26.37)) ;
#151915=CARTESIAN_POINT('Origin',(6.6585786437627,0.299999999999995,-26.37)) ;
#151916=CARTESIAN_POINT('Origin',(6.6585786437627,-0.399999999999999,-26.37)) ;
#151917=CARTESIAN_POINT('Origin',(6.6585786437627,-0.299999999999994,-26.37)) ;
#151918=CARTESIAN_POINT('Origin',(0.6,-0.3,-26.37)) ;
#151919=CARTESIAN_POINT('Origin',(6.65857864376269,-0.300000000000001,-26.37)) ;
#151920=CARTESIAN_POINT('Origin',(6.65857864376269,-0.299999999999998,-26.37)) ;
#151921=CARTESIAN_POINT('Origin',(0.6,-0.6,-30.78)) ;
#151922=CARTESIAN_POINT('Origin',(0.3,-0.6,-30.78)) ;
#151923=CARTESIAN_POINT('Origin',(0.3,-6.1,-30.78)) ;
#151924=CARTESIAN_POINT('Origin',(0.3,-6.05857864376269,-30.78)) ;
#151925=CARTESIAN_POINT('Origin',(0.3,-6.05857864376269,-30.78)) ;
#151926=CARTESIAN_POINT('Origin',(0.299999999999999,-6.05857864376269,-30.78)) ;
#151927=CARTESIAN_POINT('Origin',(0.4,-6.05857864376269,-30.78)) ;
#151928=CARTESIAN_POINT('Origin',(-0.299999999999994,-6.0585786437627,-30.78)) ;
#151929=CARTESIAN_POINT('Origin',(-0.299999999999999,-6.05857864376269,
-30.78)) ;
#151930=CARTESIAN_POINT('Origin',(-0.3,-6.05857864376269,-30.78)) ;
#151931=CARTESIAN_POINT('Origin',(-0.3,-0.600000000000001,-30.78)) ;
#151932=CARTESIAN_POINT('Origin',(-0.3,-0.600000000000001,-30.78)) ;
#151933=CARTESIAN_POINT('Origin',(0.6,-0.600000000000001,-30.78)) ;
#151934=CARTESIAN_POINT('Origin',(0.6,-0.600000000000001,-30.18)) ;
#151935=CARTESIAN_POINT('Origin',(-0.3,-0.600000000000001,-30.18)) ;
#151936=CARTESIAN_POINT('Origin',(-0.3,-0.600000000000001,-30.18)) ;
#151937=CARTESIAN_POINT('Origin',(-0.3,-6.05857864376269,-30.18)) ;
#151938=CARTESIAN_POINT('Origin',(-0.3,-6.05857864376269,-30.18)) ;
#151939=CARTESIAN_POINT('Origin',(-0.299999999999994,-6.0585786437627,-30.18)) ;
#151940=CARTESIAN_POINT('Origin',(0.4,-6.0585786437627,-30.18)) ;
#151941=CARTESIAN_POINT('Origin',(0.299999999999993,-6.0585786437627,-30.18)) ;
#151942=CARTESIAN_POINT('Origin',(0.299999999999996,-6.0585786437627,-30.18)) ;
#151943=CARTESIAN_POINT('Origin',(0.3,-6.05857864376269,-30.18)) ;
#151944=CARTESIAN_POINT('Origin',(0.3,-0.600000000000001,-30.18)) ;
#151945=CARTESIAN_POINT('Origin',(0.3,-0.6,-30.18)) ;
#151946=CARTESIAN_POINT('Origin',(0.6,-0.6,-30.18)) ;
#151947=CARTESIAN_POINT('Origin',(6.7,0.300000000000001,-30.78)) ;
#151948=CARTESIAN_POINT('Origin',(6.65857864376269,0.300000000000001,-30.78)) ;
#151949=CARTESIAN_POINT('Origin',(6.65857864376269,0.300000000000001,-30.78)) ;
#151950=CARTESIAN_POINT('Origin',(6.65857864376269,0.299999999999997,-30.78)) ;
#151951=CARTESIAN_POINT('Origin',(6.65857864376269,-0.399999999999999,-30.78)) ;
#151952=CARTESIAN_POINT('Origin',(6.65857864376269,-0.299999999999997,-30.78)) ;
#151953=CARTESIAN_POINT('Origin',(6.65857864376269,-0.3,-30.78)) ;
#151954=CARTESIAN_POINT('Origin',(6.65857864376269,-0.300000000000001,-30.78)) ;
#151955=CARTESIAN_POINT('Origin',(0.6,-0.3,-30.78)) ;
#151956=CARTESIAN_POINT('Origin',(0.6,0.299999999999999,-30.18)) ;
#151957=CARTESIAN_POINT('Origin',(6.65857864376269,0.300000000000001,-30.18)) ;
#151958=CARTESIAN_POINT('Origin',(6.65857864376269,0.300000000000001,-30.18)) ;
#151959=CARTESIAN_POINT('Origin',(6.6585786437627,0.299999999999995,-30.18)) ;
#151960=CARTESIAN_POINT('Origin',(6.6585786437627,-0.399999999999999,-30.18)) ;
#151961=CARTESIAN_POINT('Origin',(6.6585786437627,-0.299999999999994,-30.18)) ;
#151962=CARTESIAN_POINT('Origin',(0.6,-0.3,-30.18)) ;
#151963=CARTESIAN_POINT('Origin',(6.65857864376269,-0.300000000000001,-30.18)) ;
#151964=CARTESIAN_POINT('Origin',(6.65857864376269,-0.299999999999998,-30.18)) ;
#151965=CARTESIAN_POINT('Origin',(0.6,-0.6,-34.59)) ;
#151966=CARTESIAN_POINT('Origin',(0.3,-0.6,-34.59)) ;
#151967=CARTESIAN_POINT('Origin',(0.3,-6.1,-34.59)) ;
#151968=CARTESIAN_POINT('Origin',(0.3,-6.05857864376269,-34.59)) ;
#151969=CARTESIAN_POINT('Origin',(0.3,-6.05857864376269,-34.59)) ;
#151970=CARTESIAN_POINT('Origin',(0.3,-6.05857864376269,-34.59)) ;
#151971=CARTESIAN_POINT('Origin',(0.4,-6.05857864376269,-34.59)) ;
#151972=CARTESIAN_POINT('Origin',(-0.299999999999998,-6.05857864376269,
-34.59)) ;
#151973=CARTESIAN_POINT('Origin',(-0.299999999999994,-6.0585786437627,-34.59)) ;
#151974=CARTESIAN_POINT('Origin',(-0.3,-6.05857864376269,-34.59)) ;
#151975=CARTESIAN_POINT('Origin',(-0.3,-0.600000000000001,-34.59)) ;
#151976=CARTESIAN_POINT('Origin',(-0.3,-0.600000000000001,-34.59)) ;
#151977=CARTESIAN_POINT('Origin',(0.6,-0.600000000000001,-34.59)) ;
#151978=CARTESIAN_POINT('Origin',(0.6,-0.600000000000001,-33.99)) ;
#151979=CARTESIAN_POINT('Origin',(-0.3,-0.600000000000001,-33.99)) ;
#151980=CARTESIAN_POINT('Origin',(-0.3,-0.600000000000001,-33.99)) ;
#151981=CARTESIAN_POINT('Origin',(-0.3,-6.05857864376269,-33.99)) ;
#151982=CARTESIAN_POINT('Origin',(-0.3,-6.05857864376269,-33.99)) ;
#151983=CARTESIAN_POINT('Origin',(-0.300000000000007,-6.05857864376268,
-33.99)) ;
#151984=CARTESIAN_POINT('Origin',(0.4,-6.05857864376269,-33.99)) ;
#151985=CARTESIAN_POINT('Origin',(0.30000000000001,-6.05857864376268,-33.99)) ;
#151986=CARTESIAN_POINT('Origin',(0.300000000000006,-6.05857864376268,-33.99)) ;
#151987=CARTESIAN_POINT('Origin',(0.3,-6.05857864376269,-33.99)) ;
#151988=CARTESIAN_POINT('Origin',(0.3,-0.600000000000001,-33.99)) ;
#151989=CARTESIAN_POINT('Origin',(0.3,-0.6,-33.99)) ;
#151990=CARTESIAN_POINT('Origin',(0.6,-0.6,-33.99)) ;
#151991=CARTESIAN_POINT('Origin',(6.7,0.300000000000001,-34.59)) ;
#151992=CARTESIAN_POINT('Origin',(6.65857864376269,0.300000000000001,-34.59)) ;
#151993=CARTESIAN_POINT('Origin',(6.65857864376269,0.300000000000001,-34.59)) ;
#151994=CARTESIAN_POINT('Origin',(6.65857864376269,0.300000000000001,-34.59)) ;
#151995=CARTESIAN_POINT('Origin',(6.6585786437627,-0.399999999999999,-34.59)) ;
#151996=CARTESIAN_POINT('Origin',(6.65857864376269,-0.300000000000002,-34.59)) ;
#151997=CARTESIAN_POINT('Origin',(6.6585786437627,-0.299999999999996,-34.59)) ;
#151998=CARTESIAN_POINT('Origin',(6.65857864376269,-0.300000000000001,-34.59)) ;
#151999=CARTESIAN_POINT('Origin',(0.6,-0.3,-34.59)) ;
#152000=CARTESIAN_POINT('Origin',(0.6,0.299999999999999,-33.99)) ;
#152001=CARTESIAN_POINT('Origin',(6.65857864376269,0.300000000000001,-33.99)) ;
#152002=CARTESIAN_POINT('Origin',(6.65857864376269,0.300000000000001,-33.99)) ;
#152003=CARTESIAN_POINT('Origin',(6.65857864376269,0.300000000000005,-33.99)) ;
#152004=CARTESIAN_POINT('Origin',(6.65857864376269,-0.399999999999999,-33.99)) ;
#152005=CARTESIAN_POINT('Origin',(6.65857864376268,-0.300000000000006,-33.99)) ;
#152006=CARTESIAN_POINT('Origin',(0.6,-0.3,-33.99)) ;
#152007=CARTESIAN_POINT('Origin',(6.65857864376269,-0.300000000000001,-33.99)) ;
#152008=CARTESIAN_POINT('Origin',(6.65857864376269,-0.300000000000001,-33.99)) ;
#170120=UNCERTAINTY_MEASURE_WITH_UNIT(LENGTH_MEASURE(0.01),#170128,
'DISTANCE_ACCURACY_VALUE',
'Maximum model space distance between geometric entities at asserted c
onnectivities') ;
#170122=UNCERTAINTY_MEASURE_WITH_UNIT(LENGTH_MEASURE(0.01),#170128,
'DISTANCE_ACCURACY_VALUE',
'Maximum model space distance between geometric entities at asserted c
onnectivities') ;
#170125=(
GEOMETRIC_REPRESENTATION_CONTEXT(3)
GLOBAL_UNCERTAINTY_ASSIGNED_CONTEXT((#170120))
GLOBAL_UNIT_ASSIGNED_CONTEXT((#170128,#170130,#170131))
REPRESENTATION_CONTEXT('','3D')
) ;
#170127=(
GEOMETRIC_REPRESENTATION_CONTEXT(3)
GLOBAL_UNCERTAINTY_ASSIGNED_CONTEXT((#170122))
GLOBAL_UNIT_ASSIGNED_CONTEXT((#170128,#170130,#170131))
REPRESENTATION_CONTEXT('','3D')
) ;
#170128=(
LENGTH_UNIT()
NAMED_UNIT(*)
SI_UNIT(.MILLI.,.METRE.)
) ;
#170130=(
NAMED_UNIT(*)
PLANE_ANGLE_UNIT()
SI_UNIT($,.RADIAN.)
) ;
#170131=(
NAMED_UNIT(*)
SI_UNIT($,.STERADIAN.)
SOLID_ANGLE_UNIT()
) ;
#170134=SHAPE_DEFINITION_REPRESENTATION(#170138,#170145) ;
#170138=PRODUCT_DEFINITION_SHAPE('',$,#170150) ;
#170145=SHAPE_REPRESENTATION('',(#93348),#170125) ;
#170147=PRODUCT_DEFINITION_CONTEXT('part definition',#170161,'design') ;
#170150=PRODUCT_DEFINITION('Terminal_Block_Header',
'Terminal_Block_Header',#170154,#170147) ;
#170154=PRODUCT_DEFINITION_FORMATION('',$,#170165) ;
#170161=APPLICATION_CONTEXT(
'Core Data for Automotive Mechanical Design Process') ;
#170162=PRODUCT_CONTEXT('part definition',#170161,'mechanical') ;
#170165=PRODUCT('Terminal_Block_Header','Terminal_Block_Header',$,(#170162)) ;
#170168=PRESENTATION_STYLE_ASSIGNMENT((#170174)) ;
#170169=PRESENTATION_STYLE_ASSIGNMENT((#170175)) ;
#170171=PRESENTATION_STYLE_ASSIGNMENT((#170177)) ;
#170174=SURFACE_STYLE_USAGE(.BOTH.,#170180) ;
#170175=SURFACE_STYLE_USAGE(.BOTH.,#170181) ;
#170177=SURFACE_STYLE_USAGE(.BOTH.,#170183) ;
#170180=SURFACE_SIDE_STYLE('',(#170186)) ;
#170181=SURFACE_SIDE_STYLE('',(#170187)) ;
#170183=SURFACE_SIDE_STYLE('',(#170189)) ;
#170186=SURFACE_STYLE_FILL_AREA(#170192) ;
#170187=SURFACE_STYLE_FILL_AREA(#170193) ;
#170189=SURFACE_STYLE_FILL_AREA(#170195) ;
#170192=FILL_AREA_STYLE('Opaque(202,209,238)',(#170198)) ;
#170193=FILL_AREA_STYLE('Opaque(128,255,128)',(#170199)) ;
#170195=FILL_AREA_STYLE('Opaque(204,207,204)',(#170201)) ;
#170198=FILL_AREA_STYLE_COLOUR('Opaque(202,209,238)',#170204) ;
#170199=FILL_AREA_STYLE_COLOUR('Opaque(128,255,128)',#170205) ;
#170201=FILL_AREA_STYLE_COLOUR('Opaque(204,207,204)',#170207) ;
#170204=COLOUR_RGB('Opaque(202,209,238)', 0.09019608, 0.27058824, 0.51372549) ;
#170205=COLOUR_RGB('Opaque(128,255,128)', 0.09019608, 0.27058824, 0.51372549) ;
#170207=COLOUR_RGB('Opaque(204,207,204)', 0.09019608, 0.27058824, 0.51372549) ;
ENDSEC;
END-ISO-10303-21;
